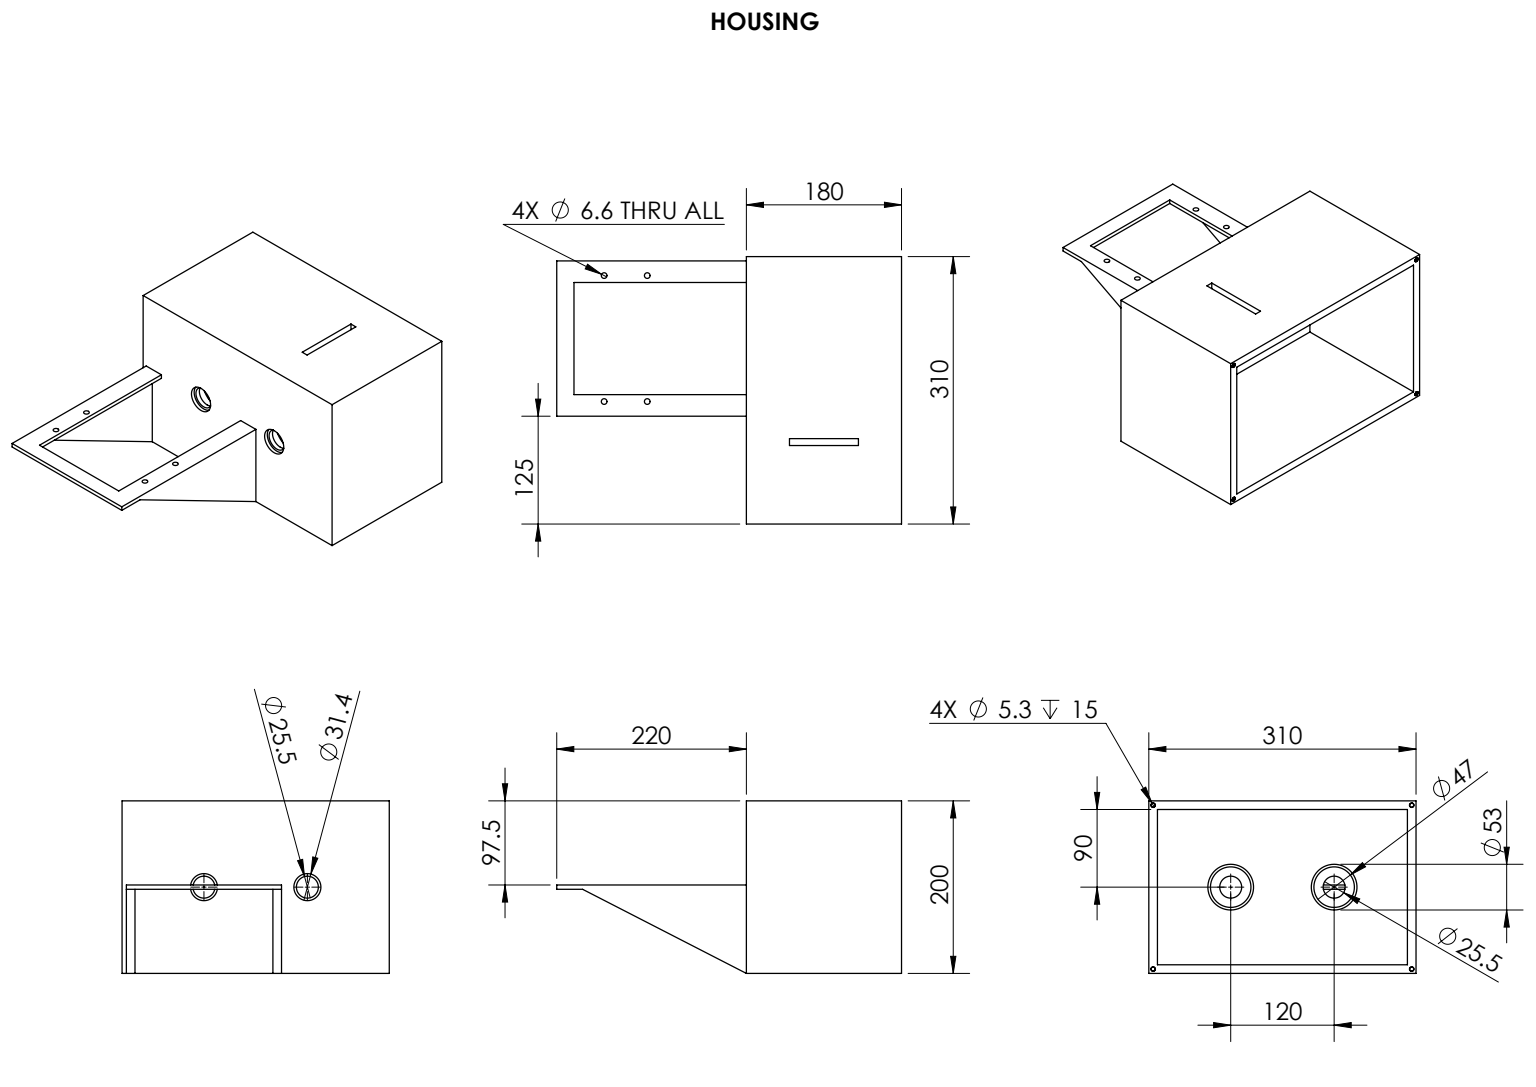
ISO-10303-21;
HEADER;
FILE_DESCRIPTION (('STEP AP214'),
    '1' );
FILE_NAME ('housing.step',
    '2026-10-08T09:53:37',
    ( '' ),
    ( '' ),
    'SwSTEP 2.0',
    'SolidWorks 2026',
    '' );
FILE_SCHEMA (( 'AUTOMOTIVE_DESIGN' ));
ENDSEC;

DATA;
#1=ORIENTED_EDGE ( 'NONE', *, *, #51679, .F. ) ;
#2=CARTESIAN_POINT ( 'NONE',  ( -96.15314808468745866, -211.9973110713294489, 75.77864583420047495 ) ) ;
#6=DIRECTION ( 'NONE',  ( -0.000000000000000000, -0.000000000000000000, 1.000000000000000000 ) ) ;
#9=CARTESIAN_POINT ( 'NONE',  ( -92.34999999999999432, -209.9999999999999716, 90.00000000000000000 ) ) ;
#10=CARTESIAN_POINT ( 'NONE',  ( 96.15314808468748708, 91.99731107132950569, 84.98614583420047097 ) ) ;
#18=CARTESIAN_POINT ( 'NONE',  ( 99.99999999999998579, 90.00000000000000000, -90.00000000000000000 ) ) ;
#23=CARTESIAN_POINT ( 'NONE',  ( -92.69370383062505425, 91.33154071421968467, 89.37822916753378877 ) ) ;
#27=CARTESIAN_POINT ( 'NONE',  ( -93.07557990970633455, 88.17815826261617929, 75.00000000000001421 ) ) ;
#29=CARTESIAN_POINT ( 'NONE',  ( -92.35000000000005116, 91.52997821335253548, 77.03541666666666288 ) ) ;
#32=DIRECTION ( 'NONE',  ( 0.4565542962317865050, 0.000000000000000000, 0.8896955516311735312 ) ) ;
#37=CARTESIAN_POINT ( 'NONE',  ( 97.30629616937498838, -208.6684592857803011, 84.45697916753383083 ) ) ;
#47=CARTESIAN_POINT ( 'NONE',  ( 96.15314808468750130, -211.9973110713294489, 77.78947916753381264 ) ) ;
#49=CARTESIAN_POINT ( 'NONE',  ( 95.00000000000000000, -212.6630814284392557, 84.24531250086715772 ) ) ;
#52=ORIENTED_EDGE ( 'NONE', *, *, #54649, .T. ) ;
#53=CARTESIAN_POINT ( 'NONE',  ( -92.35000000000005116, -211.5299782133524786, 88.35958333333334735 ) ) ;
#54=ORIENTED_EDGE ( 'NONE', *, *, #5365, .T. ) ;
#56=CARTESIAN_POINT ( 'NONE',  ( -97.30629616937501680, 88.66845928578038638, 75.24947916753383481 ) ) ;
#60=CARTESIAN_POINT ( 'NONE',  ( 97.64999999999997726, -211.5299782133524502, 87.16895833506762870 ) ) ;
#78=CARTESIAN_POINT ( 'NONE',  ( 95.00000000000000000, -213.0599564267049857, 76.18874999999999886 ) ) ;
#79=CARTESIAN_POINT ( 'NONE',  ( -97.64999999960622290, -209.9999706925929672, 76.74344264316562203 ) ) ;
#80=CARTESIAN_POINT ( 'NONE',  ( -97.65000000000001990, 90.00000000000004263, 86.82500000000000284 ) ) ;
#85=LINE ( 'NONE', #57553, #61145 ) ;
#86=CARTESIAN_POINT ( 'NONE',  ( -92.69370383062498320, -209.9999999999999716, 84.88031250086713442 ) ) ;
#87=ORIENTED_EDGE ( 'NONE', *, *, #45061, .F. ) ;
#90=CARTESIAN_POINT ( 'NONE',  ( 93.89144186338218390, -212.3693961632864955, 74.97612907457772735 ) ) ;
#91=CARTESIAN_POINT ( 'NONE',  ( -2.499999999999970690, 73.00000000000001421, -201.6999999999999602 ) ) ;
#92=CARTESIAN_POINT ( 'NONE',  ( -97.30629616937497417, -208.6684592857803295, 76.25489583420049655 ) ) ;
#95=CARTESIAN_POINT ( 'NONE',  ( 94.99999999999998579, 90.00000000000002842, 90.00000000000000000 ) ) ;
#101=CARTESIAN_POINT ( 'NONE',  ( -96.15314808468752972, 91.99731107132950569, 78.74197916753381321 ) ) ;
#104=( BOUNDED_CURVE ( )  B_SPLINE_CURVE ( 2, ( #36888, #19593, #59840, #8323, #31250, #71460, #19961 ),
 .UNSPECIFIED., .F., .F. ) 
 B_SPLINE_CURVE_WITH_KNOTS ( ( 3, 2, 2, 3 ),
 ( 0.2291666666666663521, 0.2361111111111107719, 0.2430555555555551639, 0.2499999999999995837 ),
 .UNSPECIFIED. ) 
 CURVE ( )  GEOMETRIC_REPRESENTATION_ITEM ( )  RATIONAL_B_SPLINE_CURVE ( ( 1.000000000000005995, 0.8660254037844328234, 1.000000000000000000, 0.8660254037844387076, 1.000000000000000000, 0.8660254037844467012, 0.9999999999999920064 ) ) 
 REPRESENTATION_ITEM ( '' )  );
#106=DIRECTION ( 'NONE',  ( -1.000000000000000000, 0.000000000000000000, -0.000000000000000000 ) ) ;
#108=CARTESIAN_POINT ( 'NONE',  ( 97.64999999999999147, 90.00000015433757028, 79.60187500750917877 ) ) ;
#112=CARTESIAN_POINT ( 'NONE',  ( -93.84685191531248449, -208.0026889286704943, 80.06489583420048461 ) ) ;
#113=LINE ( 'NONE', #11332, #2116 ) ;
#129=CARTESIAN_POINT ( 'NONE',  ( 92.69370383062501162, -208.6684592857803295, 89.58989583420047609 ) ) ;
#134=EDGE_CURVE ( 'NONE', #23470, #67171, #321, .T. ) ;
#135=ORIENTED_EDGE ( 'NONE', *, *, #35787, .T. ) ;
#145=ORIENTED_EDGE ( 'NONE', *, *, #39730, .F. ) ;
#146=CYLINDRICAL_SURFACE ( 'NONE', #33227, 26.50000000000000355 ) ;
#156=CARTESIAN_POINT ( 'NONE',  ( 97.30629616937498838, 91.33154071421968467, 85.56822916753380071 ) ) ;
#157=EDGE_CURVE ( 'NONE', #60576, #23470, #28588, .T. ) ;
#159=CARTESIAN_POINT ( 'NONE',  ( 96.15314808468750130, -211.9973110713294489, 82.23447916753380582 ) ) ;
#163=CARTESIAN_POINT ( 'NONE',  ( -2.500000000000015543, -73.00000000000001421, -255.0000000000000000 ) ) ;
#164=CARTESIAN_POINT ( 'NONE',  ( -94.99999999999997158, -206.9400435732949575, 89.20624999999999716 ) ) ;
#165=CARTESIAN_POINT ( 'NONE',  ( -97.65000000000001990, 90.00000000000004263, 79.20499999999999829 ) ) ;
#166=CARTESIAN_POINT ( 'NONE',  ( 97.65000000000000568, 88.47002178664752137, 85.26395833506762756 ) ) ;
#167=CARTESIAN_POINT ( 'NONE',  ( -93.84685191531248449, -208.0026889286704943, 84.98614583420047097 ) ) ;
#168=CARTESIAN_POINT ( 'NONE',  ( -92.69370383062502583, 91.33154071421968467, 85.72697916753381264 ) ) ;
#169=EDGE_CURVE ( 'NONE', #3345, #5520, #11254, .T. ) ;
#171=CARTESIAN_POINT ( 'NONE',  ( 96.15314808468748708, 91.99731107132950569, 84.98614583420047097 ) ) ;
#172=CARTESIAN_POINT ( 'NONE',  ( -95.00000000000002842, 92.66308142843932671, 85.03906250086714635 ) ) ;
#175=CARTESIAN_POINT ( 'NONE',  ( 96.32499999999998863, -212.2949673200287179, 76.32104166840096582 ) ) ;
#178=CARTESIAN_POINT ( 'NONE',  ( -96.15314808468745866, -211.9973110713294489, 86.57364583420047666 ) ) ;
#187=CARTESIAN_POINT ( 'NONE',  ( -97.65000000000001990, 90.00000000000004263, 77.29999999999999716 ) ) ;
#188=LINE ( 'NONE', #23080, #53533 ) ;
#190=LINE ( 'NONE', #46749, #7538 ) ;
#191=CARTESIAN_POINT ( 'NONE',  ( -92.35000000000000853, -208.4700217866474929, 89.73541666666663730 ) ) ;
#193=ORIENTED_EDGE ( 'NONE', *, *, #19096, .F. ) ;
#194=CARTESIAN_POINT ( 'NONE',  ( -97.30629616937501680, 88.66845928578038638, 76.99572916753380980 ) ) ;
#205=CARTESIAN_POINT ( 'NONE',  ( 97.30629616937498838, 90.00000000000002842, 78.68906250086715204 ) ) ;
#206=ADVANCED_FACE ( 'NONE', ( #58175 ), #28481, .T. ) ;
#207=CARTESIAN_POINT ( 'NONE',  ( -97.30629616937497417, -211.3315407142195852, 79.05947916753382287 ) ) ;
#211=CARTESIAN_POINT ( 'NONE',  ( -93.09170270117411405, -211.8387227684710012, 74.99909419456534465 ) ) ;
#214=EDGE_CURVE ( 'NONE', #50169, #71079, #46057, .T. ) ;
#216=CARTESIAN_POINT ( 'NONE',  ( -92.69370383062505425, 91.33154071421968467, 76.20197916753382117 ) ) ;
#217=CARTESIAN_POINT ( 'NONE',  ( 97.30629616937498838, -208.6684592857803011, 81.75822916753381264 ) ) ;
#219=CARTESIAN_POINT ( 'NONE',  ( -93.67500000000003979, 92.29496732002878900, 75.18333333333332291 ) ) ;
#221=ADVANCED_FACE ( 'NONE', ( #63104 ), #33867, .F. ) ;
#222=CYLINDRICAL_SURFACE ( 'NONE', #63992, 2.649999999999999467 ) ;
#228=ORIENTED_EDGE ( 'NONE', *, *, #5227, .F. ) ;
#230=EDGE_LOOP ( 'NONE', ( #33493, #51216, #41523, #73402, #35685 ) ) ;
#234=CARTESIAN_POINT ( 'NONE',  ( 94.99999999999998579, 92.66308142843935514, 83.92781250086716227 ) ) ;
#243=EDGE_CURVE ( 'NONE', #20441, #46588, #25658, .T. ) ;
#250=VECTOR ( 'NONE', #46862, 1000.000000000000000 ) ;
#251=FACE_OUTER_BOUND ( 'NONE', #1348, .T. ) ;
#255=CARTESIAN_POINT ( 'NONE',  ( -96.32499999999996021, -212.2949673200287179, 82.56520833506762358 ) ) ;
#256=ORIENTED_EDGE ( 'NONE', *, *, #21571, .T. ) ;
#260=CARTESIAN_POINT ( 'NONE',  ( 93.67499999999998295, 92.29496732002878900, 80.44854166840097776 ) ) ;
#261=CARTESIAN_POINT ( 'NONE',  ( -97.65000000000001990, 90.00000000000004263, 81.18937500173430521 ) ) ;
#263=CARTESIAN_POINT ( 'NONE',  ( 92.69370383062498320, 90.00000000000002842, 81.54656250086715374 ) ) ;
#269=CARTESIAN_POINT ( 'NONE',  ( -97.65000000000001990, 90.00000000000004263, 80.47499999999999432 ) ) ;
#273=ORIENTED_EDGE ( 'NONE', *, *, #31155, .T. ) ;
#276=FACE_OUTER_BOUND ( 'NONE', #73498, .T. ) ;
#277=CARTESIAN_POINT ( 'NONE',  ( -92.69370383062498320, -208.6684592857803011, 80.01197916753380923 ) ) ;
#284=CARTESIAN_POINT ( 'NONE',  ( 93.84685191531248449, 91.99731107132950569, 74.93197916753379673 ) ) ;
#288=DIRECTION ( 'NONE',  ( -0.000000000000000000, -0.000000000000000000, 1.000000000000000000 ) ) ;
#293=CARTESIAN_POINT ( 'NONE',  ( 97.30629616937498838, 88.66845928578035796, 88.79614583420048746 ) ) ;
#295=CARTESIAN_POINT ( 'NONE',  ( 94.99999999999998579, 86.94004357329502852, 82.53874999999999318 ) ) ;
#298=CARTESIAN_POINT ( 'NONE',  ( -95.00000000000002842, 92.66308142843932671, 81.22906250086714408 ) ) ;
#306=( BOUNDED_CURVE ( )  B_SPLINE_CURVE ( 2, ( #42487, #60161, #54139, #60884, #2672, #20658, #32290, #43244, #36830 ),
 .UNSPECIFIED., .F., .F. ) 
 B_SPLINE_CURVE_WITH_KNOTS ( ( 3, 2, 2, 2, 3 ),
 ( 0.3810111478265176821, 0.3810113392076479033, 0.3880671047485306224, 0.3951228702894133971, 0.4021785743327781493 ),
 .UNSPECIFIED. ) 
 CURVE ( )  GEOMETRIC_REPRESENTATION_ITEM ( )  RATIONAL_B_SPLINE_CURVE ( ( 0.9999927323225166198, 0.9999963660626911555, 1.000000000000000000, 0.8660254037844387076, 1.000000000000000000, 0.8660254037844387076, 1.000000000000000000, 0.8660265714968713446, 0.9999976645954902210 ) ) 
 REPRESENTATION_ITEM ( '' )  );
#307=CARTESIAN_POINT ( 'NONE',  ( 92.34999999999999432, 90.00000000000002842, 90.00000000000000000 ) ) ;
#314=ORIENTED_EDGE ( 'NONE', *, *, #27692, .F. ) ;
#316=CARTESIAN_POINT ( 'NONE',  ( 97.30629616937498838, -208.6684592857803295, 81.28197916753381946 ) ) ;
#321=( BOUNDED_CURVE ( )  B_SPLINE_CURVE ( 2, ( #16099, #50676, #20629, #43944, #66860, #72847, #67236, #38290, #61237 ),
 .UNSPECIFIED., .F., .F. ) 
 B_SPLINE_CURVE_WITH_KNOTS ( ( 3, 2, 2, 2, 3 ),
 ( 0.3386766260338263668, 0.3386767459623536980, 0.3457325115032360840, 0.3527882770441184701, 0.3598440426530882807 ),
 .UNSPECIFIED. ) 
 CURVE ( )  GEOMETRIC_REPRESENTATION_ITEM ( )  RATIONAL_B_SPLINE_CURVE ( ( 0.9999954456811732673, 0.9999977228018805953, 1.000000000000000000, 0.8660254037844387076, 1.000000000000000000, 0.8660254037844387076, 1.000000000000000000, 0.8660254037844387076, 1.000000000000000000 ) ) 
 REPRESENTATION_ITEM ( '' )  );
#322=CARTESIAN_POINT ( 'NONE',  ( 92.35000000049315361, 89.99996796133687837, 83.73041644179049570 ) ) ;
#324=CARTESIAN_POINT ( 'NONE',  ( 97.64999999999999147, -209.9999999999999716, 87.77749999999998920 ) ) ;
#329=ORIENTED_EDGE ( 'NONE', *, *, #65370, .T. ) ;
#331=EDGE_CURVE ( 'NONE', #62654, #68271, #27501, .T. ) ;
#333=CARTESIAN_POINT ( 'NONE',  ( -96.15314808468752972, 91.99731107132950569, 89.06072916753382174 ) ) ;
#336=CARTESIAN_POINT ( 'NONE',  ( 92.35000000000000853, -209.9999999999999716, 75.47437500173430180 ) ) ;
#337=CARTESIAN_POINT ( 'NONE',  ( 92.34999999999999432, 90.00000000000002842, 79.83999999999998920 ) ) ;
#338=EDGE_LOOP ( 'NONE', ( #19478, #31271, #53427, #16608 ) ) ;
#343=ORIENTED_EDGE ( 'NONE', *, *, #47596, .F. ) ;
#344=CARTESIAN_POINT ( 'NONE',  ( -97.65000000000001990, 91.52997821335253548, 89.39145833506763950 ) ) ;
#346=CARTESIAN_POINT ( 'NONE',  ( -97.30629616937501680, 91.33154071421968467, 82.76364583420048859 ) ) ;
#347=CARTESIAN_POINT ( 'NONE',  ( 94.99999999999998579, 92.66308142843935514, 89.64281250086715147 ) ) ;
#351=CARTESIAN_POINT ( 'NONE',  ( 96.32499999999998863, -212.2949673200287179, 85.76666666666665151 ) ) ;
#357=CARTESIAN_POINT ( 'NONE',  ( -92.69370383062498320, -209.9999999999999716, 77.89531250086714920 ) ) ;
#360=DIRECTION ( 'NONE',  ( -0.000000000000000000, -0.000000000000000000, 1.000000000000000000 ) ) ;
#362=CARTESIAN_POINT ( 'NONE',  ( 92.34999999999990905, 88.47002178664757821, 77.98791666666667766 ) ) ;
#363=CARTESIAN_POINT ( 'NONE',  ( -96.32499999999996021, -212.2949673200287179, 78.04083333333333883 ) ) ;
#365=CARTESIAN_POINT ( 'NONE',  ( -96.15314808468745866, -211.9973110713294489, 75.14364583420046984 ) ) ;
#373=CARTESIAN_POINT ( 'NONE',  ( 92.69370383062498320, 91.33154071421968467, 83.23989583420048177 ) ) ;
#397=DIRECTION ( 'NONE',  ( -0.000000000000000000, -0.000000000000000000, 1.000000000000000000 ) ) ;
#400=CARTESIAN_POINT ( 'NONE',  ( 95.00000000000000000, -207.3369185715606307, 85.83281250086714920 ) ) ;
#405=CARTESIAN_POINT ( 'NONE',  ( -97.64999999999996305, -209.9999999999999716, 86.18999999999999773 ) ) ;
#408=CARTESIAN_POINT ( 'NONE',  ( 95.00000000000000000, -212.6630814284392557, 76.46656250086712703 ) ) ;
#409=ORIENTED_EDGE ( 'NONE', *, *, #48240, .T. ) ;
#410=CARTESIAN_POINT ( 'NONE',  ( 93.84685191531249870, -208.0026889286704943, 83.98072916753382344 ) ) ;
#413=ORIENTED_EDGE ( 'NONE', *, *, #7216, .F. ) ;
#414=EDGE_LOOP ( 'NONE', ( #16035, #20964, #13795, #59926 ) ) ;
#418=DIRECTION ( 'NONE',  ( 1.000000000000000000, 0.000000000000000000, 0.000000000000000000 ) ) ;
#419=CARTESIAN_POINT ( 'NONE',  ( 97.64999999999997726, -211.5299782133524502, 86.53395833506763779 ) ) ;
#422=VECTOR ( 'NONE', #39738, 1000.000000000000000 ) ;
#423=VERTEX_POINT ( 'NONE', #26756 ) ;
#428=VERTEX_POINT ( 'NONE', #4227 ) ;
#429=CARTESIAN_POINT ( 'NONE',  ( -92.35001786638896704, -211.5299885285169523, 78.27895762153575276 ) ) ;
#437=CARTESIAN_POINT ( 'NONE',  ( 94.99999999999998579, 93.05995642670504253, 81.58624999999999261 ) ) ;
#438=CARTESIAN_POINT ( 'NONE',  ( -93.67500000000003979, 92.29496732002878900, 85.97833333333332462 ) ) ;
#443=DIRECTION ( 'NONE',  ( -1.000000000000000000, 0.000000000000000000, 0.000000000000000000 ) ) ;
#444=CARTESIAN_POINT ( 'NONE',  ( -96.15314808468745866, -211.9973110713294489, 86.57364583420047666 ) ) ;
#448=CARTESIAN_POINT ( 'NONE',  ( 94.70433044324006744, -212.6272429001183752, 74.99300273738302280 ) ) ;
#449=CARTESIAN_POINT ( 'NONE',  ( 97.64999999999999147, -209.9999999999999716, 87.77749999999998920 ) ) ;
#450=CARTESIAN_POINT ( 'NONE',  ( -94.99999999999997158, -212.6630814284392557, 77.10156250086711793 ) ) ;
#460=CARTESIAN_POINT ( 'NONE',  ( 94.99999999999998579, 86.94004357329502852, 88.25374999999999659 ) ) ;
#461=CARTESIAN_POINT ( 'NONE',  ( -96.15314808468751551, 88.00268892867056536, 78.31864583420048120 ) ) ;
#465=CARTESIAN_POINT ( 'NONE',  ( -97.64998201403183486, -208.4700114024439301, 80.50145761676010636 ) ) ;
#466=ADVANCED_FACE ( 'NONE', ( #10577, #5342 ), #11324, .T. ) ;
#472=CARTESIAN_POINT ( 'NONE',  ( -97.30629616937497417, -211.3315407142195852, 77.15447916753382174 ) ) ;
#475=ORIENTED_EDGE ( 'NONE', *, *, #13669, .T. ) ;
#491=CARTESIAN_POINT ( 'NONE',  ( 92.69370383062501162, -209.9999999999999716, 87.73781250086713612 ) ) ;
#492=CARTESIAN_POINT ( 'NONE',  ( -96.32499999999996021, -207.7050326799711968, 83.62354166840097491 ) ) ;
#496=CARTESIAN_POINT ( 'NONE',  ( 92.35000000000000853, -209.9999999999999716, 89.36499999999999488 ) ) ;
#502=CARTESIAN_POINT ( 'NONE',  ( -96.15314808468752972, 91.99731107132950569, 80.80572916753382628 ) ) ;
#508=ORIENTED_EDGE ( 'NONE', *, *, #49231, .F. ) ;
#510=B_SPLINE_CURVE_WITH_KNOTS ( 'NONE', 3,
 ( #3394, #26294, #49227, #66535, #39824, #742 ),
 .UNSPECIFIED., .F., .F.,
 ( 4, 2, 4 ),
 ( 0.7528176110416364697, 0.8153862273022683960, 0.8779548435629003222 ),
 .UNSPECIFIED. ) ;
#513=VECTOR ( 'NONE', #18864, 1000.000000000000000 ) ;
#515=CARTESIAN_POINT ( 'NONE',  ( 97.30629616937498838, 88.66845928578037217, 84.19239583420046813 ) ) ;
#517=CARTESIAN_POINT ( 'NONE',  ( 92.69370383062501162, -208.6684592857803011, 82.60489583420047666 ) ) ;
#519=CARTESIAN_POINT ( 'NONE',  ( -94.99999999999997158, -213.0599564267049857, 81.34812500173430294 ) ) ;
#520=CARTESIAN_POINT ( 'NONE',  ( -93.33265519076724104, -212.0887925413172184, 75.00000000000000000 ) ) ;
#525=CARTESIAN_POINT ( 'NONE',  ( -96.15314808468747287, -208.0026889286704943, 83.82197916753381151 ) ) ;
#526=CARTESIAN_POINT ( 'NONE',  ( -92.69370383062502583, 88.66845928578038638, 81.17614583420048291 ) ) ;
#528=CARTESIAN_POINT ( 'NONE',  ( 94.99999999999998579, 92.66308142843935514, 83.76906250086713612 ) ) ;
#529=( BOUNDED_CURVE ( )  B_SPLINE_CURVE ( 2, ( #47805, #72207, #66588, #9060, #20711, #13586, #71832, #43301, #43665 ),
 .UNSPECIFIED., .F., .F. ) 
 B_SPLINE_CURVE_WITH_KNOTS ( ( 3, 2, 2, 2, 3 ),
 ( 0.5291824299508934848, 0.5362381811070600079, 0.5432939466479423940, 0.5503497121888247801, 0.5503499107226622611 ),
 .UNSPECIFIED. ) 
 CURVE ( )  GEOMETRIC_REPRESENTATION_ITEM ( )  RATIONAL_B_SPLINE_CURVE ( ( 1.000000000000000000, 0.8660254037844387076, 1.000000000000000000, 0.8660254037844387076, 1.000000000000000000, 0.8660254037844387076, 1.000000000000000000, 0.9999962302473691667, 0.9999924607068835236 ) ) 
 REPRESENTATION_ITEM ( '' )  );
#532=CARTESIAN_POINT ( 'NONE',  ( 97.64999999999602665, -210.0000045800691737, 76.42687486206342840 ) ) ;
#534=LINE ( 'NONE', #6511, #45287 ) ;
#535=CARTESIAN_POINT ( 'NONE',  ( -97.30629616937495996, -209.9999999999999716, 86.46781250086714010 ) ) ;
#541=ORIENTED_EDGE ( 'NONE', *, *, #46124, .F. ) ;
#545=CARTESIAN_POINT ( 'NONE',  ( -97.65000000000001990, 91.52997821335253548, 77.24708333333332178 ) ) ;
#555=CARTESIAN_POINT ( 'NONE',  ( -92.69370383062504004, 90.00000000000004263, 79.80031250086713612 ) ) ;
#556=ADVANCED_FACE ( 'NONE', ( #33503 ), #45931, .F. ) ;
#558=AXIS2_PLACEMENT_3D ( 'NONE', #43819, #60369, #66736 ) ;
#561=CARTESIAN_POINT ( 'NONE',  ( 92.35000000039373447, 90.00002930740642171, 76.74344264317738862 ) ) ;
#563=CARTESIAN_POINT ( 'NONE',  ( -96.15314808468745866, -211.9973110713294489, 87.36739583420049371 ) ) ;
#566=CARTESIAN_POINT ( 'NONE',  ( 97.30629616937498838, 88.66845928578035796, 76.73114583420048973 ) ) ;
#568=CARTESIAN_POINT ( 'NONE',  ( -96.15314808468747287, -208.0026889286704943, 78.90072916753382515 ) ) ;
#570=ORIENTED_EDGE ( 'NONE', *, *, #37192, .T. ) ;
#572=DIRECTION ( 'NONE',  ( -0.000000000000000000, -0.000000000000000000, 1.000000000000000000 ) ) ;
#573=CYLINDRICAL_SURFACE ( 'NONE', #58202, 2.649999999999985700 ) ;
#575=CARTESIAN_POINT ( 'NONE',  ( 97.30629616937498838, -208.6684592857803011, 78.58322916753381548 ) ) ;
#577=EDGE_CURVE ( 'NONE', #43302, #35704, #70298, .T. ) ;
#578=EDGE_CURVE ( 'NONE', #23298, #25333, #62669, .T. ) ;
#587=ORIENTED_EDGE ( 'NONE', *, *, #27135, .F. ) ;
#589=CARTESIAN_POINT ( 'NONE',  ( 96.92442009029420547, -211.8218417373832096, 75.00000000000001421 ) ) ;
#593=CARTESIAN_POINT ( 'NONE',  ( 97.30629616937498838, 90.00000000000002842, 83.76906250086716454 ) ) ;
#596=CARTESIAN_POINT ( 'NONE',  ( 96.32499999999998863, -212.2949673200287179, 76.24166666666666003 ) ) ;
#597=ORIENTED_EDGE ( 'NONE', *, *, #35391, .T. ) ;
#603=CARTESIAN_POINT ( 'NONE',  ( -92.34999999999999432, -209.9999999999999716, 85.23749999999999716 ) ) ;
#605=CYLINDRICAL_SURFACE ( 'NONE', #65079, 2.649999999999985700 ) ;
#610=ORIENTED_EDGE ( 'NONE', *, *, #1325, .T. ) ;
#611=CARTESIAN_POINT ( 'NONE',  ( -93.67499999999998295, -212.2949673200287179, 79.49604166840096298 ) ) ;
#617=CARTESIAN_POINT ( 'NONE',  ( 94.99999999999998579, 86.94004357329500010, 80.71312500173431204 ) ) ;
#618=CARTESIAN_POINT ( 'NONE',  ( -95.00000000000002842, 93.05995642670501411, 81.03062500173430749 ) ) ;
#619=ORIENTED_EDGE ( 'NONE', *, *, #26416, .F. ) ;
#620=CARTESIAN_POINT ( 'NONE',  ( 97.30629616937498838, 91.33154071421968467, 79.37697916753381833 ) ) ;
#621=CARTESIAN_POINT ( 'NONE',  ( -93.67499999999998295, -207.7050326799711968, 82.16833333333332234 ) ) ;
#625=CYLINDRICAL_SURFACE ( 'NONE', #23007, 2.649999999999999467 ) ;
#626=CARTESIAN_POINT ( 'NONE',  ( 92.35000000000000853, -209.9999999999999716, 84.28499999999999659 ) ) ;
#628=CARTESIAN_POINT ( 'NONE',  ( -92.35000000000003695, 90.00000000000004263, 80.15749999999999886 ) ) ;
#636=FACE_OUTER_BOUND ( 'NONE', #73794, .T. ) ;
#638=CARTESIAN_POINT ( 'NONE',  ( -92.69370383062498320, -208.6684592857803011, 76.20197916753382117 ) ) ;
#644=FACE_BOUND ( 'NONE', #53061, .T. ) ;
#645=CARTESIAN_POINT ( 'NONE',  ( 94.99999999999998579, 87.33691857156068750, 75.83156250086715033 ) ) ;
#655=CARTESIAN_POINT ( 'NONE',  ( 97.30629616937498838, 88.66845928578035796, 85.62114583420047609 ) ) ;
#659=ORIENTED_EDGE ( 'NONE', *, *, #57378, .T. ) ;
#661=CARTESIAN_POINT ( 'NONE',  ( -92.69370383062505425, 88.66845928578038638, 81.01739583420048518 ) ) ;
#666=CARTESIAN_POINT ( 'NONE',  ( 97.30629616937498838, -209.9999999999999716, 86.78531250086714977 ) ) ;
#668=ORIENTED_EDGE ( 'NONE', *, *, #18506, .T. ) ;
#669=CARTESIAN_POINT ( 'NONE',  ( -92.35000000000003695, 89.99999996655868983, 87.85687500050293863 ) ) ;
#672=ORIENTED_EDGE ( 'NONE', *, *, #52995, .F. ) ;
#673=EDGE_CURVE ( 'NONE', #53082, #50612, #29711, .T. ) ;
#674=CARTESIAN_POINT ( 'NONE',  ( 7.103376864691351012E-17, -120.0000000000000000, -64.00000000000000000 ) ) ;
#678=ORIENTED_EDGE ( 'NONE', *, *, #36155, .F. ) ;
#679=CARTESIAN_POINT ( 'NONE',  ( 97.30629616937498838, -209.9999999999999716, 81.86406250086714920 ) ) ;
#680=CYLINDRICAL_SURFACE ( 'NONE', #59674, 2.649999999999985700 ) ;
#681=DIRECTION ( 'NONE',  ( -0.000000000000000000, -0.000000000000000000, 1.000000000000000000 ) ) ;
#683=CARTESIAN_POINT ( 'NONE',  ( 97.64999999989933599, 90.00002309722570715, 83.41187580057898288 ) ) ;
#685=CARTESIAN_POINT ( 'NONE',  ( 95.00000000000000000, -206.9400435732949575, 84.12625000000001307 ) ) ;
#693=CARTESIAN_POINT ( 'NONE',  ( -93.84685191531252713, 88.00268892867056536, 88.74322916753382628 ) ) ;
#696=CARTESIAN_POINT ( 'NONE',  ( 92.35000000000000853, -209.9999999999999716, 76.74437500173429783 ) ) ;
#697=CARTESIAN_POINT ( 'NONE',  ( 97.64999999999997726, 91.52997821335252127, 78.30541666666668732 ) ) ;
#698=ORIENTED_EDGE ( 'NONE', *, *, #67370, .F. ) ;
#699=CARTESIAN_POINT ( 'NONE',  ( -93.67499999999998295, -207.7050326799711968, 89.23270833506762756 ) ) ;
#700=ORIENTED_EDGE ( 'NONE', *, *, #70526, .F. ) ;
#702=ORIENTED_EDGE ( 'NONE', *, *, #35715, .T. ) ;
#703=CARTESIAN_POINT ( 'NONE',  ( -97.65000000000001990, 90.00000000000004263, 88.17437500173430465 ) ) ;
#704=CARTESIAN_POINT ( 'NONE',  ( -92.69370383062505425, 88.66845928578038638, 82.44614583420049314 ) ) ;
#705=CARTESIAN_POINT ( 'NONE',  ( 97.30629616937498838, 91.33154071421968467, 76.04322916753380923 ) ) ;
#710=CARTESIAN_POINT ( 'NONE',  ( 95.00000000000000000, -213.0599564267049857, 85.71374999999999034 ) ) ;
#715=AXIS2_PLACEMENT_3D ( 'NONE', #66827, #15314, #46127 ) ;
#716=CARTESIAN_POINT ( 'NONE',  ( -97.30629616937497417, -208.6684592857803011, 76.88989583420047325 ) ) ;
#721=CARTESIAN_POINT ( 'NONE',  ( 97.64999999946594755, 90.00005320149050192, 78.96687695417308817 ) ) ;
#724=ORIENTED_EDGE ( 'NONE', *, *, #39012, .T. ) ;
#728=CARTESIAN_POINT ( 'NONE',  ( -97.30629616937497417, -211.3315407142195852, 87.94947916753382344 ) ) ;
#730=CARTESIAN_POINT ( 'NONE',  ( 97.64999999994533653, 89.99998298270493535, 88.49187441316099978 ) ) ;
#732=ORIENTED_EDGE ( 'NONE', *, *, #49373, .F. ) ;
#735=CARTESIAN_POINT ( 'NONE',  ( -97.65000000000001990, 90.00000000000004263, 83.72937500173429726 ) ) ;
#738=CARTESIAN_POINT ( 'NONE',  ( 94.99999999999998579, 87.33691857156068750, 85.99156250086714692 ) ) ;
#742=CARTESIAN_POINT ( 'NONE',  ( 96.90829729882862864, -211.8387227684681591, 74.99954709728268654 ) ) ;
#745=CARTESIAN_POINT ( 'NONE',  ( 95.00000000000000000, -213.0599564267049857, 87.69812500173429726 ) ) ;
#747=( BOUNDED_CURVE ( )  B_SPLINE_CURVE ( 2, ( #24289, #12255, #25012, #14741, #18627, #40847, #41566, #47953, #70870 ),
 .UNSPECIFIED., .F., .F. ) 
 B_SPLINE_CURVE_WITH_KNOTS ( ( 3, 2, 2, 2, 3 ),
 ( 0.2751748541917909407, 0.2822306216366805010, 0.2892863871775971929, 0.2963421527185139959, 0.2963422021995995026 ),
 .UNSPECIFIED. ) 
 CURVE ( )  GEOMETRIC_REPRESENTATION_ITEM ( )  RATIONAL_B_SPLINE_CURVE ( ( 1.000000000000000000, 0.8660254037844387076, 1.000000000000000000, 0.8660254037844387076, 1.000000000000000000, 0.8660254037844387076, 1.000000000000000000, 0.9999990604551106665, 0.9999981209233991253 ) ) 
 REPRESENTATION_ITEM ( '' )  );
#756=( BOUNDED_CURVE ( )  B_SPLINE_CURVE ( 2, ( #59486, #48574, #47465, #64762, #25279, #41816, #36176, #7978, #48203 ),
 .UNSPECIFIED., .F., .F. ) 
 B_SPLINE_CURVE_WITH_KNOTS ( ( 3, 2, 2, 2, 3 ),
 ( 0.4021785743347534581, 0.4021786358322713695, 0.4092344013731880059, 0.4162901669141046423, 0.4233457466706606609 ),
 .UNSPECIFIED. ) 
 CURVE ( )  GEOMETRIC_REPRESENTATION_ITEM ( )  RATIONAL_B_SPLINE_CURVE ( ( 0.9999976645954944399, 0.9999988322875694724, 1.000000000000000000, 0.8660254037844387076, 1.000000000000000000, 0.8660254037844387076, 1.000000000000000000, 0.8660289314505091873, 0.9999929448536319931 ) ) 
 REPRESENTATION_ITEM ( '' )  );
#757=DIRECTION ( 'NONE',  ( 0.000000000000000000, 0.000000000000000000, 1.000000000000000000 ) ) ;
#761=CARTESIAN_POINT ( 'NONE',  ( -93.67500000000003979, 87.70503267997129626, 77.59104166840097605 ) ) ;
#764=CARTESIAN_POINT ( 'NONE',  ( 96.15314808468748708, -208.0026889286704943, 83.87489583420048689 ) ) ;
#769=VERTEX_POINT ( 'NONE', #31569 ) ;
#773=CARTESIAN_POINT ( 'NONE',  ( 96.15314808468748708, -208.0026889286704943, 75.46114583420047950 ) ) ;
#775=CARTESIAN_POINT ( 'NONE',  ( 92.69370383062501162, -208.6684592857803011, 80.85864583420048746 ) ) ;
#785=CARTESIAN_POINT ( 'NONE',  ( 96.32499999999998863, -207.7050326799711968, 87.96270833506763154 ) ) ;
#786=ORIENTED_EDGE ( 'NONE', *, *, #5639, .T. ) ;
#791=EDGE_CURVE ( 'NONE', #29550, #48269, #72525, .T. ) ;
#792=CARTESIAN_POINT ( 'NONE',  ( 97.64999999999997726, 91.52997821335252127, 87.27479166840096525 ) ) ;
#805=FACE_OUTER_BOUND ( 'NONE', #65981, .T. ) ;
#806=ADVANCED_FACE ( 'NONE', ( #54514 ), #43981, .F. ) ;
#807=CARTESIAN_POINT ( 'NONE',  ( -95.00000000000002842, 86.94004357329504273, 86.98374999999998636 ) ) ;
#812=CARTESIAN_POINT ( 'NONE',  ( -96.15314808468747287, -208.0026889286704943, 85.72697916753379843 ) ) ;
#815=CARTESIAN_POINT ( 'NONE',  ( -97.64999999992174651, -209.9999869687493685, 79.28395951166956479 ) ) ;
#819=CARTESIAN_POINT ( 'NONE',  ( -93.84685191531248449, -208.0026889286704943, 74.82614583420047438 ) ) ;
#826=DIRECTION ( 'NONE',  ( -0.000000000000000000, -0.000000000000000000, 1.000000000000000000 ) ) ;
#827=ADVANCED_FACE ( 'NONE', ( #55624 ), #60537, .F. ) ;
#829=EDGE_CURVE ( 'NONE', #43747, #51185, #3600, .T. ) ;
#830=CARTESIAN_POINT ( 'NONE',  ( -96.15314808468752972, 91.99731107132950569, 77.47197916753380298 ) ) ;
#844=CARTESIAN_POINT ( 'NONE',  ( -96.15314808468747287, -208.0026889286704943, 76.99572916753382401 ) ) ;
#845=FACE_OUTER_BOUND ( 'NONE', #61404, .T. ) ;
#856=CARTESIAN_POINT ( 'NONE',  ( 97.30629616937498838, -208.6684592857803295, 83.66322916753381378 ) ) ;
#865=CARTESIAN_POINT ( 'NONE',  ( -92.69370383062502583, 91.33154071421968467, 80.01197916753380923 ) ) ;
#869=EDGE_CURVE ( 'NONE', #18817, #10724, #10128, .T. ) ;
#871=( BOUNDED_CURVE ( )  B_SPLINE_CURVE ( 2, ( #24028, #46957, #18006, #63886, #69869, #12357, #35300 ),
 .UNSPECIFIED., .F., .F. ) 
 B_SPLINE_CURVE_WITH_KNOTS ( ( 3, 2, 2, 3 ),
 ( 0.8333333333333334814, 0.8402777777777779011, 0.8472222222222222099, 0.8541666666666666297 ),
 .UNSPECIFIED. ) 
 CURVE ( )  GEOMETRIC_REPRESENTATION_ITEM ( )  RATIONAL_B_SPLINE_CURVE ( ( 0.9999999999999978906, 0.8660254037844408170, 1.000000000000000000, 0.8660254037844387076, 1.000000000000000000, 0.8660254037844387076, 1.000000000000000000 ) ) 
 REPRESENTATION_ITEM ( '' )  );
#881=CARTESIAN_POINT ( 'NONE',  ( 96.32499999999998863, -212.2949673200287179, 80.76604166840097321 ) ) ;
#886=CARTESIAN_POINT ( 'NONE',  ( 96.15314808468750130, -211.9973110713294489, 81.59947916753381492 ) ) ;
#891=CARTESIAN_POINT ( 'NONE',  ( 97.64999999999999147, 89.99999999755287661, 75.15687493081163950 ) ) ;
#893=CARTESIAN_POINT ( 'NONE',  ( -97.65000000000003411, -208.4700217866475214, 89.31208333333333371 ) ) ;
#895=CARTESIAN_POINT ( 'NONE',  ( 96.32499999999998863, -207.7050326799711968, 76.45333333333333314 ) ) ;
#896=CARTESIAN_POINT ( 'NONE',  ( -97.30629616937497417, -211.3315407142195852, 85.88572916753382458 ) ) ;
#898=CARTESIAN_POINT ( 'NONE',  ( -96.15314808468751551, 88.00268892867056536, 82.28739583420048120 ) ) ;
#900=CARTESIAN_POINT ( 'NONE',  ( 97.30629616937498838, 88.66845928578037217, 85.46239583420047836 ) ) ;
#907=CARTESIAN_POINT ( 'NONE',  ( -94.99999999999997158, -212.6630814284392557, 85.35656250086714181 ) ) ;
#911=CARTESIAN_POINT ( 'NONE',  ( 92.35000000000005116, 91.52997821335254969, 80.42208333333330472 ) ) ;
#912=ORIENTED_EDGE ( 'NONE', *, *, #73582, .T. ) ;
#914=CARTESIAN_POINT ( 'NONE',  ( -93.67500000000003979, 87.70503267997129626, 78.78166666666666629 ) ) ;
#918=CARTESIAN_POINT ( 'NONE',  ( -97.30629616937501680, 91.33154071421968467, 87.68489583420047495 ) ) ;
#919=CARTESIAN_POINT ( 'NONE',  ( 97.64999999999999147, -209.9999999999999716, 80.79249999999998977 ) ) ;
#922=CARTESIAN_POINT ( 'NONE',  ( 97.65000000000000568, -208.4700217866474645, 77.74979166840097378 ) ) ;
#925=CARTESIAN_POINT ( 'NONE',  ( -97.30629616937501680, 91.33154071421968467, 76.88989583420047325 ) ) ;
#928=FACE_OUTER_BOUND ( 'NONE', #18946, .T. ) ;
#933=CARTESIAN_POINT ( 'NONE',  ( -94.99999999999997158, -212.6630814284392557, 84.88031250086714863 ) ) ;
#935=CARTESIAN_POINT ( 'NONE',  ( 97.64999999946594755, -209.9999467985095976, 78.96687695417307395 ) ) ;
#936=CARTESIAN_POINT ( 'NONE',  ( 92.69370383062498320, 90.00000000000002842, 76.46656250086715545 ) ) ;
#937=CARTESIAN_POINT ( 'NONE',  ( -97.30629616937497417, -211.3315407142195852, 75.24947916753383481 ) ) ;
#945=CARTESIAN_POINT ( 'NONE',  ( 97.30629616937498838, -211.3315407142195852, 77.20739583420046870 ) ) ;
#948=EDGE_CURVE ( 'NONE', #66194, #44844, #36716, .T. ) ;
#951=DIRECTION ( 'NONE',  ( 1.000000000000000000, 0.000000000000000000, 0.000000000000000000 ) ) ;
#953=CARTESIAN_POINT ( 'NONE',  ( -92.35000000053409508, 90.00005320149026034, 78.96687695417308817 ) ) ;
#954=EDGE_LOOP ( 'NONE', ( #39042, #25241, #27298, #50210 ) ) ;
#962=( BOUNDED_CURVE ( )  B_SPLINE_CURVE ( 2, ( #1157, #42080, #42445, #59365, #65383, #65016, #54102 ),
 .UNSPECIFIED., .F., .F. ) 
 B_SPLINE_CURVE_WITH_KNOTS ( ( 3, 2, 2, 3 ),
 ( 0.4583333333333335924, 0.4652777777777780122, 0.4722222222222224319, 0.4791666666666668517 ),
 .UNSPECIFIED. ) 
 CURVE ( )  GEOMETRIC_REPRESENTATION_ITEM ( )  RATIONAL_B_SPLINE_CURVE ( ( 0.9999999999999946709, 0.8660254037844440367, 1.000000000000000000, 0.8660254037844387076, 1.000000000000000000, 0.8660254037844354880, 1.000000000000003109 ) ) 
 REPRESENTATION_ITEM ( '' )  );
#963=CARTESIAN_POINT ( 'NONE',  ( 94.99999999999998579, 92.66308142843935514, 83.29281250086717137 ) ) ;
#977=CARTESIAN_POINT ( 'NONE',  ( -92.34999999999999432, -208.4700217866474645, 75.20979166840096752 ) ) ;
#981=CARTESIAN_POINT ( 'NONE',  ( 92.35000000039364920, -209.9999706968037287, 82.45844277051352833 ) ) ;
#985=CARTESIAN_POINT ( 'NONE',  ( -93.67499999999998295, -207.7050326799711968, 77.80270833506763495 ) ) ;
#989=CARTESIAN_POINT ( 'NONE',  ( 92.34999999999999432, 91.52997821335252127, 79.86645833506761960 ) ) ;
#990=CARTESIAN_POINT ( 'NONE',  ( -97.65000000000001990, 88.47002178664754979, 78.70229166840096013 ) ) ;
#992=CARTESIAN_POINT ( 'NONE',  ( 92.69370383062498320, 90.00000000000002842, 78.37156250086715659 ) ) ;
#995=CARTESIAN_POINT ( 'NONE',  ( -92.35000000000003695, 89.99999997928479445, 80.87187500099602744 ) ) ;
#999=CARTESIAN_POINT ( 'NONE',  ( 92.35000000000003695, -208.4700217866474929, 77.24708333333332178 ) ) ;
#1001=ORIENTED_EDGE ( 'NONE', *, *, #65099, .T. ) ;
#1008=DIRECTION ( 'NONE',  ( -0.000000000000000000, -0.000000000000000000, 1.000000000000000000 ) ) ;
#1010=CARTESIAN_POINT ( 'NONE',  ( -93.84685191531247028, -211.9973110713294489, 77.94822916753382458 ) ) ;
#1013=ORIENTED_EDGE ( 'NONE', *, *, #51838, .T. ) ;
#1021=CARTESIAN_POINT ( 'NONE',  ( 92.34999999999999432, 90.00000000000002842, 86.26937500173430351 ) ) ;
#1024=AXIS2_PLACEMENT_3D ( 'NONE', #8514, #65658, #64924 ) ;
#1025=CARTESIAN_POINT ( 'NONE',  ( 92.69370383062498320, 88.66845928578035796, 87.94947916753382344 ) ) ;
#1028=CARTESIAN_POINT ( 'NONE',  ( -96.15314808468745866, -211.9973110713294489, 86.09739583420049769 ) ) ;
#1030=ORIENTED_EDGE ( 'NONE', *, *, #64700, .F. ) ;
#1031=CARTESIAN_POINT ( 'NONE',  ( -97.65000000000006253, 91.52997821335252127, 81.69208333333332916 ) ) ;
#1032=CARTESIAN_POINT ( 'NONE',  ( -92.34999999999999432, -208.4700217866474645, 80.21041666666666003 ) ) ;
#1033=CARTESIAN_POINT ( 'NONE',  ( -93.26027265873601380, 91.51405112163766375, 74.79348190356853365 ) ) ;
#1034=AXIS2_PLACEMENT_3D ( 'NONE', #51639, #52754, #57661 ) ;
#1036=CARTESIAN_POINT ( 'NONE',  ( 92.69370383062501162, -209.9999999999999716, 86.46781250086714010 ) ) ;
#1041=DIRECTION ( 'NONE',  ( -0.000000000000000000, -0.000000000000000000, -1.000000000000000000 ) ) ;
#1051=CARTESIAN_POINT ( 'NONE',  ( 97.30629616937498838, -208.6684592857803295, 80.64697916753382856 ) ) ;
#1053=CYLINDRICAL_SURFACE ( 'NONE', #39955, 2.649999999999985700 ) ;
#1054=COLOUR_RGB ( '', 0.66274510, 0.83137255, 0.94901961) ;
#1058=CARTESIAN_POINT ( 'NONE',  ( 95.00000000000000000, -206.9400435732949575, 86.03125000000000000 ) ) ;
#1066=CARTESIAN_POINT ( 'NONE',  ( -95.00000000000002842, 92.66308142843932671, 87.73781250086715033 ) ) ;
#1069=CARTESIAN_POINT ( 'NONE',  ( 93.67500000000001137, -207.7050326799711968, 74.73354166840096013 ) ) ;
#1070=CARTESIAN_POINT ( 'NONE',  ( 96.32499999999998863, 87.70503267997126784, 77.51166666666665606 ) ) ;
#1072=CARTESIAN_POINT ( 'NONE',  ( -97.64999999999994884, -211.5299782133524502, 88.22729166840096582 ) ) ;
#1074=CARTESIAN_POINT ( 'NONE',  ( -97.64999999999999147, -211.5299782133525071, 84.97291666666667709 ) ) ;
#1077=CARTESIAN_POINT ( 'NONE',  ( -95.00000000000002842, 86.94004357329504273, 88.33312500173428816 ) ) ;
#1078=CARTESIAN_POINT ( 'NONE',  ( -93.84685191531254134, 91.99731107132950569, 82.60489583420049087 ) ) ;
#1080=CARTESIAN_POINT ( 'NONE',  ( 97.30629616937498838, 90.00000000000002842, 74.72031250086713783 ) ) ;
#1086=DIRECTION ( 'NONE',  ( 0.000000000000000000, -0.000000000000000000, -1.000000000000000000 ) ) ;
#1088=CARTESIAN_POINT ( 'NONE',  ( -97.64999999999996305, -209.9999999999999716, 86.26937500173430351 ) ) ;
#1091=EDGE_CURVE ( 'NONE', #44704, #27953, #35640, .T. ) ;
#1099=CARTESIAN_POINT ( 'NONE',  ( -92.34999999999999432, -209.9999999999999716, 89.04749999999999943 ) ) ;
#1102=CARTESIAN_POINT ( 'NONE',  ( -93.84685191531248449, -208.0026889286704943, 87.04989583420048405 ) ) ;
#1106=ORIENTED_EDGE ( 'NONE', *, *, #17167, .T. ) ;
#1107=AXIS2_PLACEMENT_3D ( 'NONE', #20105, #19733, #37790 ) ;
#1112=CARTESIAN_POINT ( 'NONE',  ( 92.69370383062498320, 88.66845928578035796, 81.44072916753380298 ) ) ;
#1115=CARTESIAN_POINT ( 'NONE',  ( -96.32500000000001705, 92.29496732002878900, 85.44916666666665606 ) ) ;
#1120=CARTESIAN_POINT ( 'NONE',  ( 94.99999999999998579, 90.00000000000002842, 90.00000000000000000 ) ) ;
#1122=CARTESIAN_POINT ( 'NONE',  ( -92.69370383062505425, 91.33154071421968467, 88.10822916753380696 ) ) ;
#1123=LINE ( 'NONE', #17998, #61089 ) ;
#1126=VERTEX_POINT ( 'NONE', #23638 ) ;
#1130=CARTESIAN_POINT ( 'NONE',  ( 92.35000000046503033, 89.99996900126896548, 83.09538598081184091 ) ) ;
#1131=AXIS2_PLACEMENT_3D ( 'NONE', #52664, #1217, #24110 ) ;
#1135=CARTESIAN_POINT ( 'NONE',  ( 96.15314808468750130, -211.9973110713294489, 81.12322916753382174 ) ) ;
#1137=EDGE_CURVE ( 'NONE', #25853, #74080, #3155, .T. ) ;
#1143=CARTESIAN_POINT ( 'NONE',  ( 95.00000000000000000, -206.9400435732949575, 88.57124999999999204 ) ) ;
#1147=CARTESIAN_POINT ( 'NONE',  ( 95.00000000000000000, -207.3369185715606307, 80.75281250086715090 ) ) ;
#1151=CARTESIAN_POINT ( 'NONE',  ( 97.64999999999999147, 89.99999990163419739, 80.23687499810812085 ) ) ;
#1157=CARTESIAN_POINT ( 'NONE',  ( -97.65000000000001990, 90.00000000000004263, 83.01499999999998636 ) ) ;
#1161=CARTESIAN_POINT ( 'NONE',  ( 92.35000000000000853, -209.9999999999999716, 86.26937500173430351 ) ) ;
#1162=CARTESIAN_POINT ( 'NONE',  ( 94.99999999999998579, 86.94004357329500010, 87.61875000000000568 ) ) ;
#1165=CARTESIAN_POINT ( 'NONE',  ( 92.35001072950491618, 91.52998440803509084, 84.94645790656223028 ) ) ;
#1169=CARTESIAN_POINT ( 'NONE',  ( -97.30629616937501680, 90.00000000000004263, 89.80156250086714920 ) ) ;
#1171=CARTESIAN_POINT ( 'NONE',  ( 97.64999999999997726, 88.47002178664753558, 86.53395833506763779 ) ) ;
#1178=ORIENTED_EDGE ( 'NONE', *, *, #31971, .T. ) ;
#1180=EDGE_LOOP ( 'NONE', ( #3896, #18215, #17497, #47321 ) ) ;
#1183=CARTESIAN_POINT ( 'NONE',  ( -92.35000000000005116, 88.47002178664754979, 88.35958333333333314 ) ) ;
#1185=ADVANCED_FACE ( 'NONE', ( #52568 ), #1489, .F. ) ;
#1187=( BOUNDED_CURVE ( )  B_SPLINE_CURVE ( 2, ( #53628, #31794, #37083, #54740, #54373, #2170, #25056 ),
 .UNSPECIFIED., .F., .F. ) 
 B_SPLINE_CURVE_WITH_KNOTS ( ( 3, 2, 2, 3 ),
 ( 0.1905056698846566698, 0.1975614351456765616, 0.2046172006865936144, 0.2116728463017078510 ),
 .UNSPECIFIED. ) 
 CURVE ( )  GEOMETRIC_REPRESENTATION_ITEM ( )  RATIONAL_B_SPLINE_CURVE ( ( 1.000000000000000000, 0.8660254037844387076, 1.000000000000000000, 0.8660254037844387076, 1.000000000000000000, 0.8660276809308252721, 0.9999954457846356171 ) ) 
 REPRESENTATION_ITEM ( '' )  );
#1191=CARTESIAN_POINT ( 'NONE',  ( -97.30629616937497417, -208.6684592857803011, 82.60489583420047666 ) ) ;
#1195=CARTESIAN_POINT ( 'NONE',  ( 93.74200686866063847, -212.2877248121147034, 74.97309184317512631 ) ) ;
#1197=CARTESIAN_POINT ( 'NONE',  ( -92.69370383062498320, -211.3315407142195852, 77.84239583420047381 ) ) ;
#1200=VECTOR ( 'NONE', #13246, 1000.000000000000000 ) ;
#1207=CARTESIAN_POINT ( 'NONE',  ( -95.00000000000002842, 87.33691857156074434, 77.10156250086711793 ) ) ;
#1213=CARTESIAN_POINT ( 'NONE',  ( 97.65000000000000568, -208.4700217866474645, 89.17979166840096639 ) ) ;
#1217=DIRECTION ( 'NONE',  ( -0.000000000000000000, -0.000000000000000000, 1.000000000000000000 ) ) ;
#1220=CARTESIAN_POINT ( 'NONE',  ( -97.30629616937495996, -209.9999999999999716, 77.10156250086714635 ) ) ;
#1223=DIRECTION ( 'NONE',  ( 1.000000000000000000, 0.000000000000000000, -0.000000000000000000 ) ) ;
#1226=LINE ( 'NONE', #70684, #62292 ) ;
#1227=CARTESIAN_POINT ( 'NONE',  ( -97.65000000000001990, 90.00000000000004263, 90.00000000000000000 ) ) ;
#1237=CARTESIAN_POINT ( 'NONE',  ( 93.84685191531249870, -208.0026889286704943, 86.36197916753381776 ) ) ;
#1238=CARTESIAN_POINT ( 'NONE',  ( -92.35000000010064980, -209.9999769027738239, 83.41187580057901130 ) ) ;
#1239=ORIENTED_EDGE ( 'NONE', *, *, #62083, .F. ) ;
#1240=CARTESIAN_POINT ( 'NONE',  ( -92.35000000000005116, 91.52997821335253548, 79.57541666666666913 ) ) ;
#1242=ORIENTED_EDGE ( 'NONE', *, *, #57164, .F. ) ;
#1245=CARTESIAN_POINT ( 'NONE',  ( -97.30629616937501680, 88.66845928578038638, 80.96447916753382401 ) ) ;
#1252=DIRECTION ( 'NONE',  ( -0.000000000000000000, -0.000000000000000000, 1.000000000000000000 ) ) ;
#1262=VERTEX_POINT ( 'NONE', #37880 ) ;
#1263=CARTESIAN_POINT ( 'NONE',  ( 93.84685191531251292, -211.9973110713294489, 82.76364583420047438 ) ) ;
#1265=ADVANCED_FACE ( 'NONE', ( #71698 ), #68476, .F. ) ;
#1271=CARTESIAN_POINT ( 'NONE',  ( 92.35000000000000853, -209.9999999999999716, 79.20499999999999829 ) ) ;
#1272=CARTESIAN_POINT ( 'NONE',  ( -97.64999999999996305, -209.9999999999999716, 89.36499999999999488 ) ) ;
#1274=VECTOR ( 'NONE', #31612, 1000.000000000000000 ) ;
#1277=CARTESIAN_POINT ( 'NONE',  ( -97.30629616937495996, -209.9999999999999716, 85.83281250086714920 ) ) ;
#1278=CARTESIAN_POINT ( 'NONE',  ( -92.69370383062504004, 90.00000000000004263, 81.22906250086715829 ) ) ;
#1280=CARTESIAN_POINT ( 'NONE',  ( 93.84685191531248449, 91.99731107132950569, 82.55197916753380127 ) ) ;
#1282=CARTESIAN_POINT ( 'NONE',  ( -95.00000000000002842, 86.94004357329504273, 78.80812500173429669 ) ) ;
#1287=CARTESIAN_POINT ( 'NONE',  ( -92.69370383062498320, -211.3315407142195852, 88.00239583420047040 ) ) ;
#1293=ORIENTED_EDGE ( 'NONE', *, *, #14537, .T. ) ;
#1295=CARTESIAN_POINT ( 'NONE',  ( -97.65000000000001990, 88.47002178664754979, 78.62291666666668277 ) ) ;
#1297=CARTESIAN_POINT ( 'NONE',  ( -97.30629616937501680, 90.00000000000004263, 89.00781250086714635 ) ) ;
#1299=CARTESIAN_POINT ( 'NONE',  ( 92.34999999999999432, 90.00000000000002842, 76.66499999999999204 ) ) ;
#1302=ORIENTED_EDGE ( 'NONE', *, *, #61731, .T. ) ;
#1307=CARTESIAN_POINT ( 'NONE',  ( -97.64999999999996305, -209.9999999999999716, 90.00000000000000000 ) ) ;
#1310=CARTESIAN_POINT ( 'NONE',  ( -94.99999999999997158, -212.6630814284392557, 87.42031250086715488 ) ) ;
#1312=EDGE_CURVE ( 'NONE', #51311, #11086, #32593, .T. ) ;
#1317=CARTESIAN_POINT ( 'NONE',  ( -96.15314808468745866, -211.9973110713294489, 75.30239583420048177 ) ) ;
#1325=EDGE_CURVE ( 'NONE', #15992, #50254, #26586, .T. ) ;
#1326=AXIS2_PLACEMENT_3D ( 'NONE', #48969, #48614, #71528 ) ;
#1327=CARTESIAN_POINT ( 'NONE',  ( -92.69370383062504004, 90.00000000000004263, 75.51406250086715488 ) ) ;
#1328=CARTESIAN_POINT ( 'NONE',  ( 95.00000000000000000, -212.6630814284392557, 76.46656250086712703 ) ) ;
#1333=EDGE_CURVE ( 'NONE', #6700, #65764, #21417, .T. ) ;
#1345=CARTESIAN_POINT ( 'NONE',  ( 92.69370383062498320, 91.33154071421968467, 84.66864583420047552 ) ) ;
#1347=CARTESIAN_POINT ( 'NONE',  ( 97.64999999999997726, -211.5299782133524502, 76.29458333333333542 ) ) ;
#1348=EDGE_LOOP ( 'NONE', ( #12482, #25821, #42433, #73861 ) ) ;
#1356=CARTESIAN_POINT ( 'NONE',  ( -97.64999999999996305, -210.0000123297513142, 75.47437542817786493 ) ) ;
#1360=CYLINDRICAL_SURFACE ( 'NONE', #49182, 2.649999999999985700 ) ;
#1362=CARTESIAN_POINT ( 'NONE',  ( -92.34999999999999432, -208.4700217866474645, 80.28979166840098003 ) ) ;
#1366=CARTESIAN_POINT ( 'NONE',  ( 96.32499999999998863, 87.70503267997126784, 80.13104166840095388 ) ) ;
#1367=CARTESIAN_POINT ( 'NONE',  ( -97.65000000000001990, 88.47002178664754979, 75.52729166840099140 ) ) ;
#1368=ORIENTED_EDGE ( 'NONE', *, *, #26702, .T. ) ;
#1369=CARTESIAN_POINT ( 'NONE',  ( 92.69370383062498320, 90.00000000000002842, 80.27656250086714351 ) ) ;
#1383=CYLINDRICAL_SURFACE ( 'NONE', #67856, 2.649999999999999467 ) ;
#1385=CARTESIAN_POINT ( 'NONE',  ( -97.30629616937495996, -209.9999999999999716, 78.37156250086715659 ) ) ;
#1389=CARTESIAN_POINT ( 'NONE',  ( -94.99999999999997158, -209.9999999999999716, 90.00000000000000000 ) ) ;
#1390=CARTESIAN_POINT ( 'NONE',  ( -92.34999999999999432, -209.9999999999999716, 90.00000000000000000 ) ) ;
#1399=DIRECTION ( 'NONE',  ( -0.000000000000000000, -0.000000000000000000, 1.000000000000000000 ) ) ;
#1400=CARTESIAN_POINT ( 'NONE',  ( 93.84685191531248449, 88.00268892867053694, 86.09739583420049769 ) ) ;
#1402=CARTESIAN_POINT ( 'NONE',  ( -92.69370383062498320, -211.3315407142195852, 86.25614583420048120 ) ) ;
#1404=VECTOR ( 'NONE', #49786, 1000.000000000000000 ) ;
#1405=CARTESIAN_POINT ( 'NONE',  ( 96.32499999999998863, -212.2949673200287179, 83.30604166840096525 ) ) ;
#1407=CARTESIAN_POINT ( 'NONE',  ( -92.34999999999999432, -208.4700217866474645, 82.75041666666665208 ) ) ;
#1408=CARTESIAN_POINT ( 'NONE',  ( -92.69370383062505425, 88.66845928578038638, 77.20739583420046870 ) ) ;
#1411=CARTESIAN_POINT ( 'NONE',  ( 95.00000000000000000, -207.3369185715606307, 85.67406250086715147 ) ) ;
#1415=( BOUNDED_CURVE ( )  B_SPLINE_CURVE ( 2, ( #55247, #62014, #10879, #21026, #50342, #61269, #73272 ),
 .UNSPECIFIED., .F., .F. ) 
 B_SPLINE_CURVE_WITH_KNOTS ( ( 3, 2, 2, 3 ),
 ( 0.8125000000000002220, 0.8194444444444446418, 0.8263888888888889506, 0.8333333333333334814 ),
 .UNSPECIFIED. ) 
 CURVE ( )  GEOMETRIC_REPRESENTATION_ITEM ( )  RATIONAL_B_SPLINE_CURVE ( ( 0.9999999999999956701, 0.8660254037844430375, 1.000000000000000000, 0.8660254037844387076, 1.000000000000000000, 0.8660254037844365982, 1.000000000000002220 ) ) 
 REPRESENTATION_ITEM ( '' )  );
#1421=CARTESIAN_POINT ( 'NONE',  ( 97.64999999999999147, 90.00000000000002842, 90.00000000000000000 ) ) ;
#1424=ORIENTED_EDGE ( 'NONE', *, *, #33606, .T. ) ;
#1425=CARTESIAN_POINT ( 'NONE',  ( 95.00000000000000000, -207.3369185715606307, 83.29281250086715715 ) ) ;
#1435=CARTESIAN_POINT ( 'NONE',  ( 93.67500000000001137, -212.2949673200287179, 85.02583333333332405 ) ) ;
#1441=CARTESIAN_POINT ( 'NONE',  ( -97.30629616937501680, 90.00000000000004263, 88.53156250086716739 ) ) ;
#1442=CARTESIAN_POINT ( 'NONE',  ( -0.0004442498525516064278, 0.001194404164626844313, -80.00000000000000000 ) ) ;
#1443=CARTESIAN_POINT ( 'NONE',  ( 97.65000000000000568, -210.0000154727341055, 78.33187446658581621 ) ) ;
#1444=CARTESIAN_POINT ( 'NONE',  ( 93.84685191531249870, -208.0026889286704943, 88.90197916753380980 ) ) ;
#1445=CARTESIAN_POINT ( 'NONE',  ( 97.64999999999997726, 88.47002178664753558, 79.46958333333333258 ) ) ;
#1447=CARTESIAN_POINT ( 'NONE',  ( -97.64999999999996305, -209.9999999999999716, 89.44437500173430067 ) ) ;
#1451=CARTESIAN_POINT ( 'NONE',  ( -92.35000000000005116, 91.52997821335253548, 87.27479166840096525 ) ) ;
#1452=CARTESIAN_POINT ( 'NONE',  ( 94.99999999999998579, 87.33691857156068750, 75.19656250086714522 ) ) ;
#1456=DIRECTION ( 'NONE',  ( 0.000000000000000000, 0.000000000000000000, 1.000000000000000000 ) ) ;
#1461=CARTESIAN_POINT ( 'NONE',  ( -94.99999999999997158, -207.3369185715606307, 75.51406250086714067 ) ) ;
#1469=CARTESIAN_POINT ( 'NONE',  ( -97.30629616937497417, -208.6684592857803011, 86.57364583420047666 ) ) ;
#1470=ORIENTED_EDGE ( 'NONE', *, *, #28367, .T. ) ;
#1478=CARTESIAN_POINT ( 'NONE',  ( 94.99999999999998579, 92.66308142843932671, 81.86406250086713499 ) ) ;
#1483=CYLINDRICAL_SURFACE ( 'NONE', #12026, 2.649999999999999467 ) ;
#1486=EDGE_CURVE ( 'NONE', #13338, #50169, #7947, .T. ) ;
#1489=CYLINDRICAL_SURFACE ( 'NONE', #8409, 2.649999999999999467 ) ;
#1490=EDGE_CURVE ( 'NONE', #73251, #73292, #52095, .T. ) ;
#1492=CARTESIAN_POINT ( 'NONE',  ( -93.84685191531252713, 88.00268892867056536, 87.94947916753380923 ) ) ;
#1497=CARTESIAN_POINT ( 'NONE',  ( 97.64999999999987779, -208.4700217866473793, 83.38541666666667140 ) ) ;
#1501=STYLED_ITEM ( 'NONE', ( #59364 ), #59777 ) ;
#1504=CARTESIAN_POINT ( 'NONE',  ( 97.30629616937498838, -208.6684592857803011, 83.18697916753382060 ) ) ;
#1517=CARTESIAN_POINT ( 'NONE',  ( 96.15314808468750130, -211.9973110713294489, 80.48822916753381662 ) ) ;
#1525=FILL_AREA_STYLE ('',( #52986 ) ) ;
#1529=CARTESIAN_POINT ( 'NONE',  ( 97.64999999999997726, -211.5299782133524502, 83.35895833506762642 ) ) ;
#1530=CARTESIAN_POINT ( 'NONE',  ( 92.34999999999999432, 90.00000000000002842, 90.00000000000000000 ) ) ;
#1533=CARTESIAN_POINT ( 'NONE',  ( -92.35000000000003695, 90.00000000000004263, 78.88750000000000284 ) ) ;
#1538=CARTESIAN_POINT ( 'NONE',  ( 92.34999999999999432, 88.47002178664753558, 87.59229166840096070 ) ) ;
#1548=CARTESIAN_POINT ( 'NONE',  ( -97.65000000000001990, 90.00000000000004263, 86.18999999999999773 ) ) ;
#1554=CARTESIAN_POINT ( 'NONE',  ( -92.69370383062498320, -208.6684592857803011, 82.39322916753381776 ) ) ;
#1558=CARTESIAN_POINT ( 'NONE',  ( 93.67499999999998295, 92.29496732002878900, 89.33854166840096411 ) ) ;
#1566=CARTESIAN_POINT ( 'NONE',  ( 96.85456758451090309, -211.3788240028427765, 74.79348190356850523 ) ) ;
#1571=CARTESIAN_POINT ( 'NONE',  ( -96.15314808468752972, 91.99731107132950569, 79.37697916753380412 ) ) ;
#1575=DIRECTION ( 'NONE',  ( 0.000000000000000000, -0.000000000000000000, -1.000000000000000000 ) ) ;
#1582=CARTESIAN_POINT ( 'NONE',  ( 95.00000000000000000, -209.9999999999999716, 90.00000000000000000 ) ) ;
#1583=CARTESIAN_POINT ( 'NONE',  ( -92.69370383062498320, -210.9303121318040155, 74.84209103131394158 ) ) ;
#1586=ORIENTED_EDGE ( 'NONE', *, *, #57493, .F. ) ;
#1594=CARTESIAN_POINT ( 'NONE',  ( 97.64999999999999147, 90.00001154861291752, 83.41187540116095533 ) ) ;
#1595=EDGE_LOOP ( 'NONE', ( #4910, #24656 ) ) ;
#1596=DIRECTION ( 'NONE',  ( -0.000000000000000000, -0.000000000000000000, 1.000000000000000000 ) ) ;
#1600=CARTESIAN_POINT ( 'NONE',  ( 93.84685191531251292, -211.9973110713294489, 85.93864583420048575 ) ) ;
#1601=CARTESIAN_POINT ( 'NONE',  ( 92.69370383062501162, -209.9999999999999716, 87.89656250086714806 ) ) ;
#1609=CARTESIAN_POINT ( 'NONE',  ( -93.84685191531254134, 91.99731107132950569, 81.33489583420049485 ) ) ;
#1613=CYLINDRICAL_SURFACE ( 'NONE', #24485, 3.299999999999969624 ) ;
#1617=ORIENTED_EDGE ( 'NONE', *, *, #51959, .T. ) ;
#1619=AXIS2_PLACEMENT_3D ( 'NONE', #13758, #25425, #3623 ) ;
#1621=( BOUNDED_CURVE ( )  B_SPLINE_CURVE ( 2, ( #67884, #27269, #44959, #20901, #21253, #16375, #39317 ),
 .UNSPECIFIED., .F., .F. ) 
 B_SPLINE_CURVE_WITH_KNOTS ( ( 3, 2, 2, 3 ),
 ( 0.06350193517771154927, 0.07055765540916983380, 0.07761342095008726127, 0.08466915177933910519 ),
 .UNSPECIFIED. ) 
 CURVE ( )  GEOMETRIC_REPRESENTATION_ITEM ( )  RATIONAL_B_SPLINE_CURVE ( ( 0.9999982793426236416, 0.8660262641186515786, 1.000000000000000000, 0.8660254037844387076, 1.000000000000000000, 0.8660260628881676359, 0.9999986817990271781 ) ) 
 REPRESENTATION_ITEM ( '' )  );
#1622=CARTESIAN_POINT ( 'NONE',  ( 94.70433044323989691, 87.37275709988163896, 74.99300273738302280 ) ) ;
#1628=CARTESIAN_POINT ( 'NONE',  ( 95.00000000000000000, -212.6630814284392557, 82.18156250086714465 ) ) ;
#1632=LINE ( 'NONE', #2734, #4166 ) ;
#1636=DIRECTION ( 'NONE',  ( 0.4565542962317865050, 0.000000000000000000, 0.8896955516311735312 ) ) ;
#1637=CARTESIAN_POINT ( 'NONE',  ( -96.15314808468745866, -211.9973110713294489, 85.93864583420048575 ) ) ;
#1638=CARTESIAN_POINT ( 'NONE',  ( -95.00000000000002842, 92.66308142843932671, 83.29281250086717137 ) ) ;
#1640=CARTESIAN_POINT ( 'NONE',  ( 92.69370383062498320, 88.66845928578037217, 79.53572916753380184 ) ) ;
#1647=CARTESIAN_POINT ( 'NONE',  ( -97.30629616937495996, -209.9999999999999716, 84.56281250086713897 ) ) ;
#1649=EDGE_CURVE ( 'NONE', #6687, #39397, #29244, .T. ) ;
#1650=CARTESIAN_POINT ( 'NONE',  ( 92.35000000003287823, 90.00000839536618003, 84.99910573348789455 ) ) ;
#1658=CARTESIAN_POINT ( 'NONE',  ( -97.65000000000001990, 91.52997821335253548, 75.97708333333333997 ) ) ;
#1660=CARTESIAN_POINT ( 'NONE',  ( -97.30629616937501680, 90.00000000000004263, 88.37281250086715545 ) ) ;
#1666=ORIENTED_EDGE ( 'NONE', *, *, #39550, .T. ) ;
#1667=CARTESIAN_POINT ( 'NONE',  ( -95.00000000000002842, 87.33691857156074434, 75.83156250086715033 ) ) ;
#1670=CARTESIAN_POINT ( 'NONE',  ( 93.67500000000001137, -207.7050326799711968, 84.25854166840096582 ) ) ;
#1671=CARTESIAN_POINT ( 'NONE',  ( -15.70000000000000284, -120.0000000000000000, -90.00000000000000000 ) ) ;
#1672=CARTESIAN_POINT ( 'NONE',  ( -92.69370383062498320, -209.9999999999999716, 85.67406250086715147 ) ) ;
#1678=CARTESIAN_POINT ( 'NONE',  ( 2.500000000000029754, 73.00000000000001421, -258.2999999999999545 ) ) ;
#1679=CARTESIAN_POINT ( 'NONE',  ( -97.30629616937495996, -209.9999999999999716, 77.73656250086715147 ) ) ;
#1680=CARTESIAN_POINT ( 'NONE',  ( 93.67499999999998295, 92.29496732002878900, 88.62416666666665321 ) ) ;
#1684=CARTESIAN_POINT ( 'NONE',  ( 96.32499999999997442, 92.29496732002878900, 85.42270833506762528 ) ) ;
#1686=VECTOR ( 'NONE', #33317, 1000.000000000000000 ) ;
#1689=CARTESIAN_POINT ( 'NONE',  ( 92.69370383062501162, -209.9999999999999716, 77.57781250086713953 ) ) ;
#1697=CARTESIAN_POINT ( 'NONE',  ( -97.64998344411506537, 91.52998777189718282, 79.23145767387349281 ) ) ;
#1701=CARTESIAN_POINT ( 'NONE',  ( -97.64999999996712177, 90.00000839536629371, 84.99910573348492449 ) ) ;
#1702=ORIENTED_EDGE ( 'NONE', *, *, #65557, .T. ) ;
#1705=CARTESIAN_POINT ( 'NONE',  ( 92.69370383062498320, 91.33154071421968467, 79.58864583420047722 ) ) ;
#1711=DIRECTION ( 'NONE',  ( -0.000000000000000000, -0.000000000000000000, 1.000000000000000000 ) ) ;
#1718=CARTESIAN_POINT ( 'NONE',  ( -0.0004442498525516064278, 0.001194404164626844313, -90.00000000000000000 ) ) ;
#1720=CARTESIAN_POINT ( 'NONE',  ( 94.99999999999998579, 93.05995642670504253, 77.77624999999999034 ) ) ;
#1721=CARTESIAN_POINT ( 'NONE',  ( -94.99999999999997158, -206.9400435732949575, 79.76062500173429726 ) ) ;
#1724=CARTESIAN_POINT ( 'NONE',  ( 92.69370383062498320, 90.00000000000002842, 89.64281250086713726 ) ) ;
#1725=CARTESIAN_POINT ( 'NONE',  ( -95.00000000000002842, 86.94004357329504273, 75.63312500173429953 ) ) ;
#1728=CARTESIAN_POINT ( 'NONE',  ( 94.99999999999998579, 87.33691857156068750, 79.80031250086715033 ) ) ;
#1729=VECTOR ( 'NONE', #24933, 1000.000000000000000 ) ;
#1730=CARTESIAN_POINT ( 'NONE',  ( -97.64999999999996305, -209.9999999999999716, 82.37999999999999545 ) ) ;
#1741=ORIENTED_EDGE ( 'NONE', *, *, #25450, .T. ) ;
#1742=EDGE_CURVE ( 'NONE', #2166, #43747, #62203, .T. ) ;
#1744=EDGE_CURVE ( 'NONE', #52184, #4841, #67009, .T. ) ;
#1749=CARTESIAN_POINT ( 'NONE',  ( -93.84685191531248449, -208.0026889286704943, 77.52489583420047836 ) ) ;
#1759=CYLINDRICAL_SURFACE ( 'NONE', #69719, 2.649999999999999467 ) ;
#1761=FACE_OUTER_BOUND ( 'NONE', #45328, .T. ) ;
#1766=CARTESIAN_POINT ( 'NONE',  ( 97.30629616937498838, 91.33154071421968467, 85.09197916753380753 ) ) ;
#1767=CARTESIAN_POINT ( 'NONE',  ( -92.69370383062498320, -208.6684592857803295, 86.99697916753382287 ) ) ;
#1770=CARTESIAN_POINT ( 'NONE',  ( -96.32500000000001705, 92.29496732002878900, 81.63916666666666799 ) ) ;
#1771=CARTESIAN_POINT ( 'NONE',  ( -97.64999999999996305, -209.9999999999999716, 81.10999999999999943 ) ) ;
#1772=CARTESIAN_POINT ( 'NONE',  ( -97.30629616937501680, 90.00000000000004263, 76.30781250086714351 ) ) ;
#1776=CARTESIAN_POINT ( 'NONE',  ( 97.30629616937498838, -211.3315407142195852, 86.73239583420047438 ) ) ;
#1787=VERTEX_POINT ( 'NONE', #50807 ) ;
#1790=CARTESIAN_POINT ( 'NONE',  ( 92.69370383062501162, -208.6684592857803295, 82.12864583420048348 ) ) ;
#1792=CARTESIAN_POINT ( 'NONE',  ( 92.34999999999999432, 90.00000000000002842, 81.10999999999999943 ) ) ;
#1795=CARTESIAN_POINT ( 'NONE',  ( 92.35000000000000853, -209.9999999999999716, 85.55499999999999261 ) ) ;
#1798=ORIENTED_EDGE ( 'NONE', *, *, #2824, .T. ) ;
#1800=VERTEX_POINT ( 'NONE', #51930 ) ;
#1802=CARTESIAN_POINT ( 'NONE',  ( -93.84685191531252713, 88.00268892867056536, 88.10822916753382117 ) ) ;
#1806=CARTESIAN_POINT ( 'NONE',  ( 93.84685191531251292, -211.9973110713294489, 87.84364583420047268 ) ) ;
#1807=CARTESIAN_POINT ( 'NONE',  ( 93.67499999999999716, 87.70503267997126784, 79.31083333333333485 ) ) ;
#1810=CARTESIAN_POINT ( 'NONE',  ( -96.32499999999996021, -207.7050326799711968, 88.06854166840095388 ) ) ;
#1814=CARTESIAN_POINT ( 'NONE',  ( -97.65000000000001990, 88.47002178664754979, 86.32229166840097889 ) ) ;
#1815=CARTESIAN_POINT ( 'NONE',  ( 93.84685191531248449, 91.99731107132950569, 89.69572916753382685 ) ) ;
#1818=ADVANCED_FACE ( 'NONE', ( #69598 ), #6092, .F. ) ;
#1820=CARTESIAN_POINT ( 'NONE',  ( 95.00000000000000000, -209.9999999999999716, 90.00000000000000000 ) ) ;
#1824=CARTESIAN_POINT ( 'NONE',  ( -97.64999999993855795, 90.00001182123732235, 81.82400613091868991 ) ) ;
#1825=AXIS2_PLACEMENT_3D ( 'NONE', #50580, #21252, #39316 ) ;
#1831=CARTESIAN_POINT ( 'NONE',  ( -97.30629616937497417, -211.3315407142195852, 88.58447916753382856 ) ) ;
#1834=EDGE_CURVE ( 'NONE', #56117, #3345, #113, .T. ) ;
#1843=CARTESIAN_POINT ( 'NONE',  ( 93.84685191531248449, 91.99731107132950569, 80.01197916753380923 ) ) ;
#1853=( BOUNDED_CURVE ( )  B_SPLINE_CURVE ( 2, ( #56734, #57097, #61995, #5234, #68384, #362, #28133 ),
 .UNSPECIFIED., .F., .F. ) 
 B_SPLINE_CURVE_WITH_KNOTS ( ( 3, 2, 2, 3 ),
 ( 0.7708333333333328152, 0.7777777777777775681, 0.7847222222222222099, 0.7916666666666669627 ),
 .UNSPECIFIED. ) 
 CURVE ( )  GEOMETRIC_REPRESENTATION_ITEM ( )  RATIONAL_B_SPLINE_CURVE ( ( 1.000000000000010658, 0.8660254037844280495, 1.000000000000000000, 0.8660254037844387076, 1.000000000000000000, 0.8660254037844322683, 1.000000000000006439 ) ) 
 REPRESENTATION_ITEM ( '' )  );
#1859=CARTESIAN_POINT ( 'NONE',  ( -96.15314808468751551, 88.00268892867056536, 87.20864583420046756 ) ) ;
#1869=CARTESIAN_POINT ( 'NONE',  ( 96.15314808468748708, -208.0026889286704943, 81.96989583420048575 ) ) ;
#1871=ORIENTED_EDGE ( 'NONE', *, *, #11857, .F. ) ;
#1873=DIRECTION ( 'NONE',  ( -0.000000000000000000, -0.000000000000000000, -1.000000000000000000 ) ) ;
#1875=CARTESIAN_POINT ( 'NONE',  ( 92.35000000000000853, -209.9999999999999716, 88.73000000000000398 ) ) ;
#1876=CARTESIAN_POINT ( 'NONE',  ( 92.69370383062501162, -208.6684592857803295, 76.25489583420049655 ) ) ;
#1878=ORIENTED_EDGE ( 'NONE', *, *, #4867, .T. ) ;
#1880=CARTESIAN_POINT ( 'NONE',  ( 95.00000000000000000, -212.6630814284392557, 79.80031250086715033 ) ) ;
#1886=CARTESIAN_POINT ( 'NONE',  ( 97.65000000000000568, -208.4700217866474645, 86.63979166840096013 ) ) ;
#1888=ADVANCED_FACE ( 'NONE', ( #34637 ), #56842, .F. ) ;
#1891=CARTESIAN_POINT ( 'NONE',  ( 93.67500000000001137, -207.7050326799711968, 83.62354166840097491 ) ) ;
#1892=CARTESIAN_POINT ( 'NONE',  ( 94.99999999999998579, 93.05995642670504253, 89.20624999999999716 ) ) ;
#1899=ORIENTED_EDGE ( 'NONE', *, *, #7386, .T. ) ;
#1900=CARTESIAN_POINT ( 'NONE',  ( -92.69370383062505425, 88.66845928578038638, 89.43114583420049257 ) ) ;
#1901=CARTESIAN_POINT ( 'NONE',  ( 94.99999999999998579, 87.33691857156068750, 84.08656250086713158 ) ) ;
#1904=CARTESIAN_POINT ( 'NONE',  ( 96.32499999999998863, 87.70503267997126784, 87.11604166840096752 ) ) ;
#1915=CARTESIAN_POINT ( 'NONE',  ( 92.34999999999999432, 91.52997821335252127, 75.42145833506764063 ) ) ;
#1916=CARTESIAN_POINT ( 'NONE',  ( -97.65000000000001990, 88.47002178664754979, 84.97291666666666288 ) ) ;
#1919=DIRECTION ( 'NONE',  ( 1.000000000000000000, 0.000000000000000000, 0.000000000000000000 ) ) ;
#1922=CARTESIAN_POINT ( 'NONE',  ( -96.15314808468747287, -208.0026889286704943, 83.82197916753381151 ) ) ;
#1923=ORIENTED_EDGE ( 'NONE', *, *, #36567, .F. ) ;
#1927=CARTESIAN_POINT ( 'NONE',  ( -92.35000000000003695, 90.00000000000004263, 90.00000000000000000 ) ) ;
#1929=CARTESIAN_POINT ( 'NONE',  ( 97.64999999999447766, 89.99999459739470353, 81.50687481489491404 ) ) ;
#1937=CARTESIAN_POINT ( 'NONE',  ( -92.69370383062504004, 90.00000000000004263, 89.48406250086715374 ) ) ;
#1940=ADVANCED_FACE ( 'NONE', ( #845 ), #22253, .F. ) ;
#1950=CARTESIAN_POINT ( 'NONE',  ( -96.15314808468747287, -208.0026889286704943, 76.36072916753381890 ) ) ;
#1962=ORIENTED_EDGE ( 'NONE', *, *, #51424, .T. ) ;
#1964=CARTESIAN_POINT ( 'NONE',  ( 93.84685191531251292, -211.9973110713294489, 86.57364583420047666 ) ) ;
#1965=CARTESIAN_POINT ( 'NONE',  ( 92.69370383062501162, -208.6684592857803295, 89.74864583420048803 ) ) ;
#1967=ADVANCED_FACE ( 'NONE', ( #36117 ), #41392, .F. ) ;
#1970=CARTESIAN_POINT ( 'NONE',  ( -92.34999999999999432, -209.9999999999999716, 80.79249999999998977 ) ) ;
#1972=CARTESIAN_POINT ( 'NONE',  ( -92.69370383062504004, 90.00000000000004263, 81.22906250086715829 ) ) ;
#1976=DIRECTION ( 'NONE',  ( -1.000000000000000000, -0.000000000000000000, -0.000000000000000000 ) ) ;
#1982=ORIENTED_EDGE ( 'NONE', *, *, #9744, .F. ) ;
#1986=ADVANCED_FACE ( 'NONE', ( #71421 ), #24117, .F. ) ;
#1987=ORIENTED_EDGE ( 'NONE', *, *, #10454, .T. ) ;
#1989=CARTESIAN_POINT ( 'NONE',  ( 95.00000000000000000, -207.3369185715606307, 79.95906250086713385 ) ) ;
#1993=LINE ( 'NONE', #8337, #11259 ) ;
#2000=CARTESIAN_POINT ( 'NONE',  ( -94.99999999999997158, -212.6630814284392557, 80.27656250086714351 ) ) ;
#2001=CARTESIAN_POINT ( 'NONE',  ( -95.00000000000002842, 87.33691857156074434, 80.43531250086715545 ) ) ;
#2005=CARTESIAN_POINT ( 'NONE',  ( 97.30629616937498838, 90.00000000000002842, 82.34031250086714238 ) ) ;
#2014=CARTESIAN_POINT ( 'NONE',  ( -94.99999999999997158, -207.3369185715606307, 82.49906250086715431 ) ) ;
#2026=CARTESIAN_POINT ( 'NONE',  ( -95.00000000000002842, 87.33691857156074434, 85.99156250086714692 ) ) ;
#2032=CARTESIAN_POINT ( 'NONE',  ( -97.30629616937501680, 90.00000000000004263, 75.67281250086713840 ) ) ;
#2039=CARTESIAN_POINT ( 'NONE',  ( -93.84685191531248449, -208.0026889286704943, 86.41489583420049314 ) ) ;
#2044=CARTESIAN_POINT ( 'NONE',  ( -96.15314808468747287, -208.0026889286704943, 76.36072916753381890 ) ) ;
#2048=CARTESIAN_POINT ( 'NONE',  ( -97.64999999999996305, -209.9999999999999716, 81.82437500173429612 ) ) ;
#2049=CARTESIAN_POINT ( 'NONE',  ( 92.34999999999990905, 91.52997821335249284, 75.97708333333333997 ) ) ;
#2050=CARTESIAN_POINT ( 'NONE',  ( 97.64999999999990621, 90.00000071509185773, 85.31687502647973531 ) ) ;
#2054=CARTESIAN_POINT ( 'NONE',  ( 96.15314808468750130, -211.9973110713294489, 76.51947916753380241 ) ) ;
#2060=( BOUNDED_CURVE ( )  B_SPLINE_CURVE ( 2, ( #61830, #44538, #55436, #21584, #72349, #38141, #38891 ),
 .UNSPECIFIED., .F., .F. ) 
 B_SPLINE_CURVE_WITH_KNOTS ( ( 3, 2, 2, 3 ),
 ( 0.2708333333333337034, 0.2777777777777781232, 0.2847222222222224874, 0.2916666666666669072 ),
 .UNSPECIFIED. ) 
 CURVE ( )  GEOMETRIC_REPRESENTATION_ITEM ( )  RATIONAL_B_SPLINE_CURVE ( ( 0.9999999999999924505, 0.8660254037844462571, 1.000000000000000000, 0.8660254037844387076, 1.000000000000000000, 0.8660254037844343777, 1.000000000000004219 ) ) 
 REPRESENTATION_ITEM ( '' )  );
#2064=DIRECTION ( 'NONE',  ( -0.000000000000000000, 0.000000000000000000, 1.000000000000000000 ) ) ;
#2069=ADVANCED_FACE ( 'NONE', ( #30464 ), #53413, .F. ) ;
#2071=FACE_OUTER_BOUND ( 'NONE', #69092, .T. ) ;
#2073=ORIENTED_EDGE ( 'NONE', *, *, #17898, .F. ) ;
#2075=CARTESIAN_POINT ( 'NONE',  ( 93.84685191531248449, 91.99731107132950569, 80.17072916753382117 ) ) ;
#2076=CARTESIAN_POINT ( 'NONE',  ( 97.64999999964365429, -210.0000434577794408, 89.12687334326047051 ) ) ;
#2080=VERTEX_POINT ( 'NONE', #31216 ) ;
#2088=DIRECTION ( 'NONE',  ( 1.000000000000000000, 0.000000000000000000, 0.000000000000000000 ) ) ;
#2091=CARTESIAN_POINT ( 'NONE',  ( -97.64999999999996305, -209.9999999999999716, 80.55437500173430010 ) ) ;
#2093=CARTESIAN_POINT ( 'NONE',  ( 94.99999999999998579, 93.05995642670504253, 75.95062500173428077 ) ) ;
#2094=CARTESIAN_POINT ( 'NONE',  ( -93.67500000000003979, 92.29496732002878900, 74.62770833506762358 ) ) ;
#2096=CARTESIAN_POINT ( 'NONE',  ( 92.69370383062498320, 91.33154071421968467, 75.14364583420049826 ) ) ;
#2115=PLANE ( 'NONE',  #73532 ) ;
#2116=VECTOR ( 'NONE', #18095, 1000.000000000000000 ) ;
#2118=CARTESIAN_POINT ( 'NONE',  ( -93.67499999999998295, -207.7050326799711968, 75.81833333333332803 ) ) ;
#2119=CARTESIAN_POINT ( 'NONE',  ( -92.69370383062498320, -209.9999999999999716, 76.78406250086715090 ) ) ;
#2120=VERTEX_POINT ( 'NONE', #32682 ) ;
#2133=CARTESIAN_POINT ( 'NONE',  ( 93.84685191531248449, 91.99731107132950569, 85.25072916753381946 ) ) ;
#2134=CARTESIAN_POINT ( 'NONE',  ( -97.30629616937495996, -209.9999999999999716, 87.26156250086715715 ) ) ;
#2138=CARTESIAN_POINT ( 'NONE',  ( -92.34999999999999432, -209.9999999999999716, 82.06250000000000000 ) ) ;
#2139=CARTESIAN_POINT ( 'NONE',  ( -96.15314808468752972, 91.99731107132950569, 75.56697916753381605 ) ) ;
#2140=CARTESIAN_POINT ( 'NONE',  ( 92.69370383062501162, -208.6684592857803011, 85.77989583420048803 ) ) ;
#2151=EDGE_CURVE ( 'NONE', #37629, #51617, #36609, .T. ) ;
#2157=CARTESIAN_POINT ( 'NONE',  ( 96.15314808468750130, -211.9973110713294489, 77.31322916753381946 ) ) ;
#2164=CARTESIAN_POINT ( 'NONE',  ( 95.00000000000000000, -213.0599564267049857, 83.17374999999999829 ) ) ;
#2166=VERTEX_POINT ( 'NONE', #31947 ) ;
#2170=CARTESIAN_POINT ( 'NONE',  ( -97.64997399525502431, -211.5299932271988723, 86.32229270695523837 ) ) ;
#2172=CARTESIAN_POINT ( 'NONE',  ( -96.15314808468752972, 91.99731107132950569, 84.61572916753381435 ) ) ;
#2179=DIRECTION ( 'NONE',  ( -1.000000000000000000, -0.000000000000000000, -0.000000000000000000 ) ) ;
#2180=ORIENTED_EDGE ( 'NONE', *, *, #58720, .T. ) ;
#2184=CARTESIAN_POINT ( 'NONE',  ( -96.32500000000001705, 92.29496732002878900, 86.79854166840097207 ) ) ;
#2186=CARTESIAN_POINT ( 'NONE',  ( 96.15314808468748708, 91.99731107132950569, 86.41489583420049314 ) ) ;
#2187=PLANE ( 'NONE',  #44209 ) ;
#2191=ORIENTED_EDGE ( 'NONE', *, *, #47228, .T. ) ;
#2200=CARTESIAN_POINT ( 'NONE',  ( -97.65000000000001990, 90.00000000000004263, 75.47437500173430180 ) ) ;
#2201=CARTESIAN_POINT ( 'NONE',  ( -92.69370383062498320, -208.6684592857803011, 88.26697916753381890 ) ) ;
#2207=VECTOR ( 'NONE', #33319, 1000.000000000000000 ) ;
#2210=CARTESIAN_POINT ( 'NONE',  ( 94.99999999999998579, 93.05995642670504253, 86.66624999999999091 ) ) ;
#2213=CARTESIAN_POINT ( 'NONE',  ( 97.30629616937498838, 90.00000000000002842, 82.97531250086714749 ) ) ;
#2216=DIRECTION ( 'NONE',  ( -0.000000000000000000, -0.000000000000000000, 1.000000000000000000 ) ) ;
#2218=CARTESIAN_POINT ( 'NONE',  ( -92.35000000000005116, 88.47002178664754979, 77.00895833506763211 ) ) ;
#2220=DIRECTION ( 'NONE',  ( 1.000000000000000000, 0.000000000000000000, 0.000000000000000000 ) ) ;
#2221=CARTESIAN_POINT ( 'NONE',  ( 92.35000000000000853, -208.4700217866474645, 85.58145833506763722 ) ) ;
#2223=ORIENTED_EDGE ( 'NONE', *, *, #63704, .T. ) ;
#2224=CARTESIAN_POINT ( 'NONE',  ( -93.84685191531254134, 91.99731107132950569, 86.89114583420047211 ) ) ;
#2225=DIRECTION ( 'NONE',  ( -1.000000000000000000, -0.000000000000000000, -0.000000000000000000 ) ) ;
#2226=ADVANCED_FACE ( 'NONE', ( #72533 ), #60186, .F. ) ;
#2229=EDGE_CURVE ( 'NONE', #46998, #14970, #33054, .T. ) ;
#2231=EDGE_CURVE ( 'NONE', #25802, #52184, #66907, .T. ) ;
#2237=EDGE_CURVE ( 'NONE', #44790, #71356, #42871, .T. ) ;
#2238=CARTESIAN_POINT ( 'NONE',  ( 93.84685191531251292, -211.9973110713294489, 83.55739583420049144 ) ) ;
#2242=CYLINDRICAL_SURFACE ( 'NONE', #47591, 2.649999999999985700 ) ;
#2245=DIRECTION ( 'NONE',  ( -0.000000000000000000, -0.000000000000000000, 1.000000000000000000 ) ) ;
#2249=CARTESIAN_POINT ( 'NONE',  ( 92.69370383062501162, -209.9999999999999716, 79.64156250086715261 ) ) ;
#2250=VECTOR ( 'NONE', #24283, 1000.000000000000000 ) ;
#2253=CARTESIAN_POINT ( 'NONE',  ( 96.32499999999998863, 87.70503267997126784, 79.41666666666665719 ) ) ;
#2258=CARTESIAN_POINT ( 'NONE',  ( 96.32499999999998863, -207.7050326799711968, 80.26333333333332121 ) ) ;
#2259=ORIENTED_EDGE ( 'NONE', *, *, #58765, .T. ) ;
#2260=CARTESIAN_POINT ( 'NONE',  ( -96.32500000000001705, 92.29496732002878900, 84.17916666666666003 ) ) ;
#2261=CARTESIAN_POINT ( 'NONE',  ( 97.64999999999997726, -208.4700217866474645, 82.82979166840095786 ) ) ;
#2262=CARTESIAN_POINT ( 'NONE',  ( 94.99999999999998579, 93.05995642670504253, 84.12625000000001307 ) ) ;
#2269=VERTEX_POINT ( 'NONE', #23284 ) ;
#2270=CARTESIAN_POINT ( 'NONE',  ( -97.30629616937501680, 91.33154071421968467, 89.11364583420049712 ) ) ;
#2271=CARTESIAN_POINT ( 'NONE',  ( 92.69370383062498320, 88.66845928578037217, 81.44072916753381719 ) ) ;
#2273=CARTESIAN_POINT ( 'NONE',  ( 97.64999999999997726, 88.47002178664753558, 85.89895833506764689 ) ) ;
#2279=ORIENTED_EDGE ( 'NONE', *, *, #8294, .F. ) ;
#2282=CARTESIAN_POINT ( 'NONE',  ( 96.32499999999997442, 92.29496732002878900, 75.26270833506764291 ) ) ;
#2285=CARTESIAN_POINT ( 'NONE',  ( -95.00000000000002842, 93.05995642670501411, 83.49125000000000796 ) ) ;
#2287=CARTESIAN_POINT ( 'NONE',  ( 96.73972734126401463, 91.51405112163766375, 74.79348190356853365 ) ) ;
#2291=( BOUNDED_CURVE ( )  B_SPLINE_CURVE ( 2, ( #27012, #72860, #38309, #31916, #49574, #20265, #44324 ),
 .UNSPECIFIED., .F., .F. ) 
 B_SPLINE_CURVE_WITH_KNOTS ( ( 3, 2, 2, 3 ),
 ( 0.5503499107253647660, 0.5574054777324447540, 0.5644612432733617791, 0.5715170088694363493 ),
 .UNSPECIFIED. ) 
 CURVE ( )  GEOMETRIC_REPRESENTATION_ITEM ( )  RATIONAL_B_SPLINE_CURVE ( ( 0.9999924607068964022, 0.8660291735370631017, 1.000000000000000000, 0.8660254037844387076, 1.000000000000000000, 0.8660254037844387076, 1.000000000000000000 ) ) 
 REPRESENTATION_ITEM ( '' )  );
#2293=CARTESIAN_POINT ( 'NONE',  ( -92.69370383062498320, -211.3315407142195852, 83.55739583420047722 ) ) ;
#2294=VERTEX_POINT ( 'NONE', #16906 ) ;
#2301=CARTESIAN_POINT ( 'NONE',  ( 97.01450244679210755, -211.1324117838501877, 74.79348190356851944 ) ) ;
#2306=CARTESIAN_POINT ( 'NONE',  ( -97.30629616937501680, 90.00000000000004263, 76.30781250086714351 ) ) ;
#2316=CARTESIAN_POINT ( 'NONE',  ( 92.35000000000000853, -209.9999999999999716, 77.29999999999999716 ) ) ;
#2318=CARTESIAN_POINT ( 'NONE',  ( 97.64999999999999147, 90.00000000000002842, 90.00000000000000000 ) ) ;
#2319=CARTESIAN_POINT ( 'NONE',  ( -92.34999999999999432, -211.5299782133524502, 89.62958333333332916 ) ) ;
#2323=DIRECTION ( 'NONE',  ( -0.000000000000000000, -0.000000000000000000, 1.000000000000000000 ) ) ;
#2327=CARTESIAN_POINT ( 'NONE',  ( 97.64999999999999147, -209.9999999999999716, 76.34749999999999659 ) ) ;
#2341=CARTESIAN_POINT ( 'NONE',  ( 93.84685191531249870, -208.0026889286704943, 83.18697916753382060 ) ) ;
#2342=CARTESIAN_POINT ( 'NONE',  ( 97.30629616937498838, -209.9999999999999716, 87.57906250086715261 ) ) ;
#2343=EDGE_CURVE ( 'NONE', #62638, #43916, #41555, .T. ) ;
#2348=CARTESIAN_POINT ( 'NONE',  ( -95.00000000000002842, 87.33691857156074434, 77.26031250086714408 ) ) ;
#2356=VERTEX_POINT ( 'NONE', #5634 ) ;
#2357=PLANE ( 'NONE',  #10599 ) ;
#2368=CARTESIAN_POINT ( 'NONE',  ( 93.84685191531249870, -208.0026889286704943, 76.83697916753381207 ) ) ;
#2376=CARTESIAN_POINT ( 'NONE',  ( -92.34999999999999432, -209.9999999999999716, 75.71250000000000568 ) ) ;
#2379=CARTESIAN_POINT ( 'NONE',  ( -92.69370383062498320, -211.3315407142195852, 80.38239583420049428 ) ) ;
#2380=CARTESIAN_POINT ( 'NONE',  ( -92.69370383062502583, 91.33154071421968467, 79.37697916753381833 ) ) ;
#2382=CARTESIAN_POINT ( 'NONE',  ( 94.99999999999998579, 92.66308142843935514, 80.59406250086715318 ) ) ;
#2384=CARTESIAN_POINT ( 'NONE',  ( 93.67499999999998295, 92.29496732002878900, 78.54354166840096241 ) ) ;
#2389=CARTESIAN_POINT ( 'NONE',  ( -93.84685191531247028, -211.9973110713294489, 83.50447916753381605 ) ) ;
#2403=CARTESIAN_POINT ( 'NONE',  ( -96.15314808468751551, 88.00268892867056536, 86.57364583420047666 ) ) ;
#2408=CARTESIAN_POINT ( 'NONE',  ( -92.69370383062504004, 90.00000000000004263, 74.72031250086713783 ) ) ;
#2409=EDGE_CURVE ( 'NONE', #19936, #50232, #5563, .T. ) ;
#2414=CARTESIAN_POINT ( 'NONE',  ( -97.64999999999996305, -209.9999999999999716, 76.03000000000000114 ) ) ;
#2415=CARTESIAN_POINT ( 'NONE',  ( -93.84685191531247028, -211.9973110713294489, 82.39322916753381776 ) ) ;
#2417=EDGE_CURVE ( 'NONE', #23688, #40782, #10815, .T. ) ;
#2421=CARTESIAN_POINT ( 'NONE',  ( 94.99999999999998579, 92.66308142843932671, 75.03781250086714749 ) ) ;
#2422=AXIS2_PLACEMENT_3D ( 'NONE', #44885, #32469, #32835 ) ;
#2423=CARTESIAN_POINT ( 'NONE',  ( -92.69370383062498320, -208.6684592857803295, 76.20197916753382117 ) ) ;
#2433=CARTESIAN_POINT ( 'NONE',  ( 92.69370383062501162, -209.9999999999999716, 88.53156250086716739 ) ) ;
#2434=EDGE_LOOP ( 'NONE', ( #65330, #60143, #52415, #7736 ) ) ;
#2441=EDGE_CURVE ( 'NONE', #8621, #33107, #31119, .T. ) ;
#2445=CARTESIAN_POINT ( 'NONE',  ( 0.000000000000000000, 0.000000000000000000, -90.00000000000000000 ) ) ;
#2450=EDGE_LOOP ( 'NONE', ( #72929, #48162 ) ) ;
#2454=LINE ( 'NONE', #24953, #27482 ) ;
#2455=ADVANCED_FACE ( 'NONE', ( #13821 ), #70220, .F. ) ;
#2458=CARTESIAN_POINT ( 'NONE',  ( 97.30629616937498838, 90.00000000000002842, 80.59406250086715318 ) ) ;
#2471=CYLINDRICAL_SURFACE ( 'NONE', #41864, 2.649999999999985700 ) ;
#2472=CARTESIAN_POINT ( 'NONE',  ( -96.32499999999996021, -207.7050326799711968, 76.63854166840096127 ) ) ;
#2473=CARTESIAN_POINT ( 'NONE',  ( -97.30629616937501680, 90.00000000000004263, 89.80156250086714920 ) ) ;
#2474=CARTESIAN_POINT ( 'NONE',  ( 92.34999999999999432, 88.47002178664753558, 75.52729166840099140 ) ) ;
#2475=CARTESIAN_POINT ( 'NONE',  ( -96.32500000000001705, 87.70503267997129626, 76.21520833506762926 ) ) ;
#2478=CARTESIAN_POINT ( 'NONE',  ( 97.30629616937498838, 91.33154071421968467, 76.20197916753382117 ) ) ;
#2479=CARTESIAN_POINT ( 'NONE',  ( 93.67499999999998295, 92.29496732002878900, 82.27416666666665890 ) ) ;
#2486=CARTESIAN_POINT ( 'NONE',  ( -97.64999999999996305, -209.9999999999999716, 87.45999999999999375 ) ) ;
#2488=CYLINDRICAL_SURFACE ( 'NONE', #61222, 2.649999999999999467 ) ;
#2490=ORIENTED_EDGE ( 'NONE', *, *, #28162, .F. ) ;
#2497=CARTESIAN_POINT ( 'NONE',  ( -97.30629616937497417, -208.6684592857803011, 75.77864583420048916 ) ) ;
#2504=LINE ( 'NONE', #12977, #33234 ) ;
#2516=( BOUNDED_CURVE ( )  B_SPLINE_CURVE ( 2, ( #11798, #69329, #5825, #17096, #219, #23471, #21985 ),
 .UNSPECIFIED., .F., .F. ) 
 B_SPLINE_CURVE_WITH_KNOTS ( ( 3, 2, 2, 3 ),
 ( 0.9583333333333337034, 0.9652777777777781232, 0.9722222222222225430, 0.9791666666666669627 ),
 .UNSPECIFIED. ) 
 CURVE ( )  GEOMETRIC_REPRESENTATION_ITEM ( )  RATIONAL_B_SPLINE_CURVE ( ( 0.9999999999999935607, 0.8660254037844451469, 1.000000000000000000, 0.8660254037844387076, 1.000000000000000000, 0.8660254037844322683, 1.000000000000006439 ) ) 
 REPRESENTATION_ITEM ( '' )  );
#2517=CARTESIAN_POINT ( 'NONE',  ( 97.30629616937498838, 91.33154071421968467, 84.45697916753383083 ) ) ;
#2518=CARTESIAN_POINT ( 'NONE',  ( -94.99999999999997158, -207.3369185715606307, 86.46781250086714010 ) ) ;
#2523=CARTESIAN_POINT ( 'NONE',  ( -94.99999999999997158, -213.0599564267049857, 81.26874999999999716 ) ) ;
#2524=CARTESIAN_POINT ( 'NONE',  ( -92.69370383062505425, 88.66845928578038638, 76.57239583420046358 ) ) ;
#2525=CARTESIAN_POINT ( 'NONE',  ( 92.69370383062501162, -211.3315407142195852, 84.61572916753380014 ) ) ;
#2538=CARTESIAN_POINT ( 'NONE',  ( 95.00000000000000000, -212.6630814284392557, 78.53031250086715431 ) ) ;
#2542=CARTESIAN_POINT ( 'NONE',  ( 97.64999999999999147, -209.9999999999999716, 80.79249999999998977 ) ) ;
#2544=CARTESIAN_POINT ( 'NONE',  ( -95.00000000000002842, 86.94004357329504273, 83.25312500173430408 ) ) ;
#2545=CARTESIAN_POINT ( 'NONE',  ( 97.64999999999999147, -209.9999999999999716, 82.69749999999999091 ) ) ;
#2547=ORIENTED_EDGE ( 'NONE', *, *, #55991, .F. ) ;
#2550=CARTESIAN_POINT ( 'NONE',  ( 2.500000000000035083, 90.00000000000000000, -279.9999999999999432 ) ) ;
#2553=CARTESIAN_POINT ( 'NONE',  ( -93.84685191531252713, 88.00268892867056536, 83.66322916753382799 ) ) ;
#2554=CARTESIAN_POINT ( 'NONE',  ( -93.67499999999998295, -207.7050326799711968, 77.08833333333332405 ) ) ;
#2557=CARTESIAN_POINT ( 'NONE',  ( 96.32499999999998863, 87.70503267997126784, 75.60666666666665492 ) ) ;
#2559=CARTESIAN_POINT ( 'NONE',  ( -96.32499999999996021, -207.7050326799711968, 84.89354166840095672 ) ) ;
#2563=CARTESIAN_POINT ( 'NONE',  ( -92.35000000000003695, 90.00000000000004263, 87.22187500173430408 ) ) ;
#2564=CARTESIAN_POINT ( 'NONE',  ( 94.99999999999998579, 87.33691857156068750, 86.15031250086714465 ) ) ;
#2570=CARTESIAN_POINT ( 'NONE',  ( 94.99999999999998579, 90.00000000000002842, 90.00000000000000000 ) ) ;
#2576=CARTESIAN_POINT ( 'NONE',  ( -97.65000000000004832, -211.5299782133524218, 83.06791666666666174 ) ) ;
#2577=CARTESIAN_POINT ( 'NONE',  ( -97.30629616937497417, -208.6684592857803011, 85.30364583420048064 ) ) ;
#2587=CARTESIAN_POINT ( 'NONE',  ( 94.99999999999998579, 87.33691857156068750, 88.69031250086716511 ) ) ;
#2589=CARTESIAN_POINT ( 'NONE',  ( 92.69370383062498320, 91.33154071421968467, 82.60489583420049087 ) ) ;
#2595=CARTESIAN_POINT ( 'NONE',  ( -97.65000000000001990, 90.00003217427526181, 76.74437388893713319 ) ) ;
#2600=CARTESIAN_POINT ( 'NONE',  ( -97.64999999953592180, 89.99996903277666149, 77.38038495128051864 ) ) ;
#2602=CARTESIAN_POINT ( 'NONE',  ( -92.69370383062505425, 88.66845928578038638, 88.00239583420047040 ) ) ;
#2604=FACE_OUTER_BOUND ( 'NONE', #63993, .T. ) ;
#2606=VECTOR ( 'NONE', #50629, 1000.000000000000000 ) ;
#2612=CARTESIAN_POINT ( 'NONE',  ( -26.50000000000000355, -120.0000000000000000, -80.00000000000000000 ) ) ;
#2616=CARTESIAN_POINT ( 'NONE',  ( 96.15314808468748708, -208.0026889286704943, 80.69989583420047552 ) ) ;
#2625=CARTESIAN_POINT ( 'NONE',  ( 97.30629616937498838, -208.6684592857803011, 77.47197916753381719 ) ) ;
#2627=ORIENTED_EDGE ( 'NONE', *, *, #62325, .T. ) ;
#2629=VERTEX_POINT ( 'NONE', #20206 ) ;
#2636=CARTESIAN_POINT ( 'NONE',  ( 97.64999999999997726, -211.5299782133524502, 83.99395833506763154 ) ) ;
#2637=CARTESIAN_POINT ( 'NONE',  ( 97.64999999999999147, 90.00000000000002842, 83.96750000000000114 ) ) ;
#2644=CARTESIAN_POINT ( 'NONE',  ( -93.84685191531254134, 91.99731107132950569, 88.31989583420048007 ) ) ;
#2645=CARTESIAN_POINT ( 'NONE',  ( 94.99999999999998579, 87.33691857156068750, 80.27656250086714351 ) ) ;
#2647=CARTESIAN_POINT ( 'NONE',  ( 94.99999999999998579, 93.05995642670504253, 82.30062500173428930 ) ) ;
#2650=CARTESIAN_POINT ( 'NONE',  ( -92.34999999999999432, -209.9999999999999716, 86.50750000000000739 ) ) ;
#2659=CARTESIAN_POINT ( 'NONE',  ( -95.00000000000002842, 86.94004357329504273, 85.07874999999999943 ) ) ;
#2663=ORIENTED_EDGE ( 'NONE', *, *, #20184, .T. ) ;
#2665=CARTESIAN_POINT ( 'NONE',  ( -92.69370383062498320, -208.6684592857803011, 78.58322916753381548 ) ) ;
#2672=CARTESIAN_POINT ( 'NONE',  ( 93.67500000000001137, -207.7050326799711968, 83.62354166840097491 ) ) ;
#2678=EDGE_CURVE ( 'NONE', #23574, #16444, #67840, .T. ) ;
#2679=CARTESIAN_POINT ( 'NONE',  ( -95.00000000000002842, 87.33691857156074434, 89.32531250086715602 ) ) ;
#2688=CARTESIAN_POINT ( 'NONE',  ( 93.84685191531248449, 91.99731107132950569, 89.06072916753382174 ) ) ;
#2693=CARTESIAN_POINT ( 'NONE',  ( -92.34999999999999432, -209.9999999999999716, 88.41249999999999432 ) ) ;
#2701=CARTESIAN_POINT ( 'NONE',  ( 92.35001072685611234, -211.5299844065056902, 78.06729209680055703 ) ) ;
#2705=DIRECTION ( 'NONE',  ( 0.000000000000000000, -1.000000000000000000, 0.000000000000000000 ) ) ;
#2707=CARTESIAN_POINT ( 'NONE',  ( 95.00000000000000000, -207.3369185715606307, 82.49906250086715431 ) ) ;
#2708=CARTESIAN_POINT ( 'NONE',  ( 92.69370383062501162, -209.9999999999999716, 89.80156250086714920 ) ) ;
#2714=CARTESIAN_POINT ( 'NONE',  ( -96.15314808468752972, 91.99731107132950569, 78.26572916753382003 ) ) ;
#2724=( BOUNDED_CURVE ( )  B_SPLINE_CURVE ( 2, ( #35371, #52653, #41380, #460, #58665, #17703, #12062 ),
 .UNSPECIFIED., .F., .F. ) 
 B_SPLINE_CURVE_WITH_KNOTS ( ( 3, 2, 2, 3 ),
 ( 0.1041666666666670182, 0.1111111111111114103, 0.1180555555555558161, 0.1250000000000002220 ),
 .UNSPECIFIED. ) 
 CURVE ( )  GEOMETRIC_REPRESENTATION_ITEM ( )  RATIONAL_B_SPLINE_CURVE ( ( 0.9999999999999933387, 0.8660254037844453689, 1.000000000000000000, 0.8660254037844387076, 1.000000000000000000, 0.8660254037844343777, 1.000000000000004219 ) ) 
 REPRESENTATION_ITEM ( '' )  );
#2731=CARTESIAN_POINT ( 'NONE',  ( 92.69370383062501162, -209.9999999999999716, 78.21281250086714465 ) ) ;
#2734=CARTESIAN_POINT ( 'NONE',  ( 97.64999999999999147, 90.00000000000002842, 90.00000000000000000 ) ) ;
#2737=CARTESIAN_POINT ( 'NONE',  ( -92.34999999999999432, -211.5299782133524218, 78.91395833506763324 ) ) ;
#2740=CYLINDRICAL_SURFACE ( 'NONE', #69209, 2.649999999999999467 ) ;
#2744=CARTESIAN_POINT ( 'NONE',  ( -94.99999999999997158, -207.3369185715606307, 80.59406250086715318 ) ) ;
#2746=CARTESIAN_POINT ( 'NONE',  ( -92.69370383062502583, 88.66845928578038638, 80.54114583420049200 ) ) ;
#2749=CARTESIAN_POINT ( 'NONE',  ( 92.69370383062498320, 91.33154071421968467, 81.33489583420048064 ) ) ;
#2754=CARTESIAN_POINT ( 'NONE',  ( -96.32499999999996021, -212.2949673200287179, 76.77083333333332860 ) ) ;
#2757=CARTESIAN_POINT ( 'NONE',  ( -97.30629616937497417, -211.3315407142195852, 81.44072916753380298 ) ) ;
#2765=CARTESIAN_POINT ( 'NONE',  ( -97.65000000000001990, 88.47002178664754979, 75.44791666666667140 ) ) ;
#2767=CARTESIAN_POINT ( 'NONE',  ( -93.84685191531254134, 91.99731107132950569, 83.71614583420047495 ) ) ;
#2768=CARTESIAN_POINT ( 'NONE',  ( -97.19210266091309336, -208.8322938842643168, 74.89296886168689582 ) ) ;
#2773=CARTESIAN_POINT ( 'NONE',  ( -92.69370383062504004, 89.06968361095763953, 74.68334086212732359 ) ) ;
#2776=CYLINDRICAL_SURFACE ( 'NONE', #58571, 2.649999999999985700 ) ;
#2778=FACE_OUTER_BOUND ( 'NONE', #230, .T. ) ;
#2779=CARTESIAN_POINT ( 'NONE',  ( -92.69370383062498320, -209.9999999999999716, 81.22906250086715829 ) ) ;
#2793=CARTESIAN_POINT ( 'NONE',  ( 93.84685191531249870, -208.0026889286704943, 87.79072916753381151 ) ) ;
#2794=VERTEX_POINT ( 'NONE', #45392 ) ;
#2806=ORIENTED_EDGE ( 'NONE', *, *, #57155, .T. ) ;
#2809=ORIENTED_EDGE ( 'NONE', *, *, #26416, .T. ) ;
#2810=CARTESIAN_POINT ( 'NONE',  ( 93.84685191531248449, 88.00268892867053694, 79.74739583420048916 ) ) ;
#2813=ORIENTED_EDGE ( 'NONE', *, *, #40858, .F. ) ;
#2816=ORIENTED_EDGE ( 'NONE', *, *, #74295, .F. ) ;
#2818=ORIENTED_EDGE ( 'NONE', *, *, #7831, .F. ) ;
#2824=EDGE_CURVE ( 'NONE', #9802, #55839, #28443, .T. ) ;
#2827=CARTESIAN_POINT ( 'NONE',  ( -92.34999999999999432, -208.4700217866474645, 76.47979166840096354 ) ) ;
#2831=CARTESIAN_POINT ( 'NONE',  ( 94.99999999999998579, 93.05995642670504253, 76.58562500173430010 ) ) ;
#2832=CARTESIAN_POINT ( 'NONE',  ( -93.67500000000003979, 87.70503267997129626, 77.59104166840097605 ) ) ;
#2833=ORIENTED_EDGE ( 'NONE', *, *, #52136, .T. ) ;
#2834=CARTESIAN_POINT ( 'NONE',  ( 96.15314808468748708, 88.00268892867053694, 76.04322916753382344 ) ) ;
#2838=CARTESIAN_POINT ( 'NONE',  ( -96.32500000000001705, 92.29496732002878900, 78.54354166840096241 ) ) ;
#2840=EDGE_CURVE ( 'NONE', #58070, #55829, #4811, .T. ) ;
#2862=CARTESIAN_POINT ( 'NONE',  ( 97.64999999999999147, -210.0000000983658026, 80.23687499810812085 ) ) ;
#2863=CARTESIAN_POINT ( 'NONE',  ( -93.67499999999998295, -207.7050326799711968, 77.80270833506763495 ) ) ;
#2866=ADVANCED_FACE ( 'NONE', ( #16432 ), #65068, .F. ) ;
#2867=CARTESIAN_POINT ( 'NONE',  ( 92.69370383062498320, 90.00000000000002842, 85.35656250086715602 ) ) ;
#2869=CARTESIAN_POINT ( 'NONE',  ( -93.84685191531247028, -211.9973110713294489, 83.02822916753380866 ) ) ;
#2873=CARTESIAN_POINT ( 'NONE',  ( -96.32499999999996021, -212.2949673200287179, 76.77083333333332860 ) ) ;
#2875=CARTESIAN_POINT ( 'NONE',  ( 92.69370383062501162, -211.3315407142195852, 82.71072916753379900 ) ) ;
#2880=ORIENTED_EDGE ( 'NONE', *, *, #9602, .T. ) ;
#2887=CARTESIAN_POINT ( 'NONE',  ( 92.69370383062501162, -209.9999999999999716, 78.37156250086715659 ) ) ;
#2889=CARTESIAN_POINT ( 'NONE',  ( -96.32500000000001705, 92.29496732002878900, 76.63854166840096127 ) ) ;
#2890=EDGE_CURVE ( 'NONE', #61621, #67171, #39759, .T. ) ;
#2895=CARTESIAN_POINT ( 'NONE',  ( 97.64999999999999147, 89.99999999755287661, 75.15687493081163950 ) ) ;
#2896=CARTESIAN_POINT ( 'NONE',  ( 95.00000000000000000, -206.9400435732949575, 82.85625000000000284 ) ) ;
#2906=CARTESIAN_POINT ( 'NONE',  ( -92.69370383062502583, 88.66845928578038638, 82.44614583420049314 ) ) ;
#2910=CARTESIAN_POINT ( 'NONE',  ( 96.32499999999997442, 92.29496732002878900, 75.81833333333332803 ) ) ;
#2913=CARTESIAN_POINT ( 'NONE',  ( -97.64999999999994884, -211.5299782133524502, 86.32229166840097889 ) ) ;
#2916=ORIENTED_EDGE ( 'NONE', *, *, #5879, .T. ) ;
#2917=CARTESIAN_POINT ( 'NONE',  ( -93.67500000000003979, 87.70503267997129626, 85.21104166840096639 ) ) ;
#2919=CARTESIAN_POINT ( 'NONE',  ( 96.15314808468748708, 88.00268892867053694, 86.20322916753382003 ) ) ;
#2925=ORIENTED_EDGE ( 'NONE', *, *, #72549, .F. ) ;
#2928=VERTEX_POINT ( 'NONE', #61981 ) ;
#2935=( BOUNDED_CURVE ( )  B_SPLINE_CURVE ( 2, ( #23444, #41110, #34342, #46748, #18167, #12147, #919 ),
 .UNSPECIFIED., .F., .F. ) 
 B_SPLINE_CURVE_WITH_KNOTS ( ( 3, 2, 2, 3 ),
 ( 0.5833333333333329263, 0.5902777777777776791, 0.5972222222222223209, 0.6041666666666670737 ),
 .UNSPECIFIED. ) 
 CURVE ( )  GEOMETRIC_REPRESENTATION_ITEM ( )  RATIONAL_B_SPLINE_CURVE ( ( 1.000000000000008660, 0.8660254037844301589, 1.000000000000000000, 0.8660254037844387076, 1.000000000000000000, 0.8660254037844301589, 1.000000000000008660 ) ) 
 REPRESENTATION_ITEM ( '' )  );
#2936=CARTESIAN_POINT ( 'NONE',  ( -97.30629616937497417, -211.3315407142195852, 84.77447916753381207 ) ) ;
#2937=ORIENTED_EDGE ( 'NONE', *, *, #64890, .F. ) ;
#2938=DIRECTION ( 'NONE',  ( -0.000000000000000000, -0.000000000000000000, 1.000000000000000000 ) ) ;
#2940=ORIENTED_EDGE ( 'NONE', *, *, #44122, .T. ) ;
#2946=CARTESIAN_POINT ( 'NONE',  ( 93.84685191531248449, 91.99731107132950569, 76.83697916753381207 ) ) ;
#2950=CARTESIAN_POINT ( 'NONE',  ( 92.80789733908675032, 91.16770611573555527, 74.89296886168688161 ) ) ;
#2953=ADVANCED_FACE ( 'NONE', ( #68365 ), #22877, .F. ) ;
#2961=CARTESIAN_POINT ( 'NONE',  ( -93.84685191531252713, 88.00268892867056536, 82.86947916753379673 ) ) ;
#2971=CARTESIAN_POINT ( 'NONE',  ( 92.69370383062501162, -211.3315407142195852, 79.69447916753381378 ) ) ;
#2979=CARTESIAN_POINT ( 'NONE',  ( 96.15314808468748708, -208.0026889286704943, 75.61989583420049144 ) ) ;
#2991=CARTESIAN_POINT ( 'NONE',  ( 96.32499999999998863, -212.2949673200287179, 82.03604166840096923 ) ) ;
#2993=CARTESIAN_POINT ( 'NONE',  ( 94.99999999999998579, 93.05995642670504253, 86.03125000000000000 ) ) ;
#2997=CARTESIAN_POINT ( 'NONE',  ( -93.67499999999998295, -212.2949673200287179, 89.02104166840096866 ) ) ;
#3000=CARTESIAN_POINT ( 'NONE',  ( -93.84685191531254134, 91.99731107132950569, 89.58989583420049030 ) ) ;
#3002=CARTESIAN_POINT ( 'NONE',  ( 97.30629616937498838, 90.00000000000002842, 82.97531250086714749 ) ) ;
#3005=CARTESIAN_POINT ( 'NONE',  ( 92.34999999999999432, 91.52997821335252127, 81.13645833506764404 ) ) ;
#3013=ORIENTED_EDGE ( 'NONE', *, *, #7066, .F. ) ;
#3017=CARTESIAN_POINT ( 'NONE',  ( -95.00000000000002842, 86.94004357329504273, 85.71374999999997613 ) ) ;
#3020=AXIS2_PLACEMENT_3D ( 'NONE', #39598, #9160, #44501 ) ;
#3024=CARTESIAN_POINT ( 'NONE',  ( -92.69370383062498320, -209.9999999999999716, 78.53031250086714010 ) ) ;
#3033=ADVANCED_FACE ( 'NONE', ( #24341 ), #2187, .T. ) ;
#3035=CARTESIAN_POINT ( 'NONE',  ( 92.69370383062498320, 88.66845928578035796, 89.06072916753382174 ) ) ;
#3038=CARTESIAN_POINT ( 'NONE',  ( -92.34999999999999432, -208.4700217866474645, 86.63979166840096013 ) ) ;
#3039=CARTESIAN_POINT ( 'NONE',  ( -92.69370383062502583, 88.66845928578038638, 75.93739583420047268 ) ) ;
#3044=CARTESIAN_POINT ( 'NONE',  ( -93.67499999999998295, -212.2949673200287179, 84.57604166840096127 ) ) ;
#3048=CARTESIAN_POINT ( 'NONE',  ( 97.65000000000000568, 88.47002178664752137, 75.73895833506765030 ) ) ;
#3049=CARTESIAN_POINT ( 'NONE',  ( -93.67499999999998295, -212.2949673200287179, 88.94166666666666288 ) ) ;
#3062=FACE_OUTER_BOUND ( 'NONE', #13368, .T. ) ;
#3063=ORIENTED_EDGE ( 'NONE', *, *, #48240, .F. ) ;
#3064=CARTESIAN_POINT ( 'NONE',  ( 93.84685191531251292, -211.9973110713294489, 82.12864583420046927 ) ) ;
#3065=CARTESIAN_POINT ( 'NONE',  ( 92.69370383062501162, -208.6684592857803295, 89.11364583420049712 ) ) ;
#3067=VECTOR ( 'NONE', #17136, 1000.000000000000000 ) ;
#3068=CARTESIAN_POINT ( 'NONE',  ( 96.15314808468750130, -211.9973110713294489, 86.83822916753382515 ) ) ;
#3073=CARTESIAN_POINT ( 'NONE',  ( -97.30629616937501680, 90.00000000000004263, 77.10156250086714635 ) ) ;
#3074=EDGE_LOOP ( 'NONE', ( #36887, #53165, #62381, #13225 ) ) ;
#3079=VERTEX_POINT ( 'NONE', #23601 ) ;
#3086=CYLINDRICAL_SURFACE ( 'NONE', #33629, 2.649999999999985700 ) ;
#3091=CARTESIAN_POINT ( 'NONE',  ( 95.00000000000000000, -212.6630814284392557, 78.37156250086714238 ) ) ;
#3098=ORIENTED_EDGE ( 'NONE', *, *, #3316, .T. ) ;
#3102=CARTESIAN_POINT ( 'NONE',  ( -92.69370383062502583, 88.66845928578038638, 79.27114583420048177 ) ) ;
#3105=CARTESIAN_POINT ( 'NONE',  ( 96.15314808468748708, 91.99731107132950569, 78.63614583420047666 ) ) ;
#3112=CARTESIAN_POINT ( 'NONE',  ( -96.15314808468745866, -211.9973110713294489, 82.76364583420047438 ) ) ;
#3122=CARTESIAN_POINT ( 'NONE',  ( -96.32500000000001705, 92.29496732002878900, 75.92416666666666458 ) ) ;
#3123=CARTESIAN_POINT ( 'NONE',  ( -92.35000000000003695, 89.99999988321006583, 84.68187499741277691 ) ) ;
#3124=CARTESIAN_POINT ( 'NONE',  ( -97.30629616937501680, 88.66845928578038638, 84.61572916753380014 ) ) ;
#3135=CARTESIAN_POINT ( 'NONE',  ( 94.99999999999998579, 86.94004357329502852, 86.34874999999999545 ) ) ;
#3136=CARTESIAN_POINT ( 'NONE',  ( -92.69370383062498320, -211.3315407142195852, 82.44614583420049314 ) ) ;
#3139=( BOUNDED_CURVE ( )  B_SPLINE_CURVE ( 2, ( #61169, #31830, #50234, #73168, #26935, #3303, #72783 ),
 .UNSPECIFIED., .F., .F. ) 
 B_SPLINE_CURVE_WITH_KNOTS ( ( 3, 2, 2, 3 ),
 ( 0.5624999999999997780, 0.5694444444444440867, 0.5763888888888885065, 0.5833333333333329263 ),
 .UNSPECIFIED. ) 
 CURVE ( )  GEOMETRIC_REPRESENTATION_ITEM ( )  RATIONAL_B_SPLINE_CURVE ( ( 1.000000000000004219, 0.8660254037844343777, 1.000000000000000000, 0.8660254037844387076, 1.000000000000000000, 0.8660254037844472563, 0.9999999999999914513 ) ) 
 REPRESENTATION_ITEM ( '' )  );
#3148=DIRECTION ( 'NONE',  ( 1.000000000000000000, 0.000000000000000000, 0.000000000000000000 ) ) ;
#3155=( BOUNDED_CURVE ( )  B_SPLINE_CURVE ( 2, ( #18720, #47669, #41300, #2221, #24740, #58580, #64598, #11979, #36019 ),
 .UNSPECIFIED., .F., .F. ) 
 B_SPLINE_CURVE_WITH_KNOTS ( ( 3, 2, 2, 2, 3 ),
 ( 0.2540073681283129825, 0.2540075594717653429, 0.2610633250126476734, 0.2681190905535301150, 0.2751748541904411316 ),
 .UNSPECIFIED. ) 
 CURVE ( )  GEOMETRIC_REPRESENTATION_ITEM ( )  RATIONAL_B_SPLINE_CURVE ( ( 0.9999927337532901195, 0.9999963667781166521, 1.000000000000000000, 0.8660254037844387076, 1.000000000000000000, 0.8660254037844387076, 1.000000000000000000, 0.8660254037844387076, 1.000000000000000000 ) ) 
 REPRESENTATION_ITEM ( '' )  );
#3161=ORIENTED_EDGE ( 'NONE', *, *, #62752, .T. ) ;
#3162=AXIS2_PLACEMENT_3D ( 'NONE', #12087, #72814, #66832 ) ;
#3164=ORIENTED_EDGE ( 'NONE', *, *, #5446, .F. ) ;
#3166=ORIENTED_EDGE ( 'NONE', *, *, #69522, .F. ) ;
#3169=VERTEX_POINT ( 'NONE', #35609 ) ;
#3173=CARTESIAN_POINT ( 'NONE',  ( 94.99999999999998579, 92.66308142843935514, 75.67281250086716682 ) ) ;
#3178=ORIENTED_EDGE ( 'NONE', *, *, #39219, .F. ) ;
#3182=CARTESIAN_POINT ( 'NONE',  ( 95.00000000000000000, -212.6630814284392557, 87.89656250086713385 ) ) ;
#3187=DIRECTION ( 'NONE',  ( -0.000000000000000000, 0.000000000000000000, 1.000000000000000000 ) ) ;
#3190=CARTESIAN_POINT ( 'NONE',  ( -97.64999999999994884, -208.4700217866474645, 76.05645833506761733 ) ) ;
#3192=CARTESIAN_POINT ( 'NONE',  ( -95.00000000000002842, 92.66308142843932671, 89.00781250086716057 ) ) ;
#3195=CARTESIAN_POINT ( 'NONE',  ( 96.32499999999997442, 92.29496732002878900, 75.26270833506764291 ) ) ;
#3196=CARTESIAN_POINT ( 'NONE',  ( -96.15314808468752972, 91.99731107132950569, 88.90197916753380980 ) ) ;
#3197=B_SPLINE_CURVE_WITH_KNOTS ( 'NONE', 1,
 ( #32318, #48878 ),
 .UNSPECIFIED., .F., .F.,
 ( 2, 2 ),
 ( 0.000000000000000000, 1.000000000000000000 ),
 .UNSPECIFIED. ) ;
#3199=CARTESIAN_POINT ( 'NONE',  ( 96.15314808468748708, 91.99731107132950569, 74.98489583420048632 ) ) ;
#3201=DIRECTION ( 'NONE',  ( -1.000000000000000000, 0.000000000000000000, -0.000000000000000000 ) ) ;
#3206=CARTESIAN_POINT ( 'NONE',  ( -97.64999999999994884, -211.5299782133524218, 87.51291666666666913 ) ) ;
#3215=CARTESIAN_POINT ( 'NONE',  ( 92.35000000009272014, 90.00001381026685010, 80.55392363656929433 ) ) ;
#3216=CARTESIAN_POINT ( 'NONE',  ( -92.69370383062499741, -210.9303297190751891, 74.84209033237941355 ) ) ;
#3219=CARTESIAN_POINT ( 'NONE',  ( -95.00000000000002842, 92.66308142843932671, 82.49906250086714010 ) ) ;
#3222=CARTESIAN_POINT ( 'NONE',  ( -97.65000000000007674, 91.52997821335250705, 79.15208333333333712 ) ) ;
#3229=DIRECTION ( 'NONE',  ( -0.000000000000000000, -0.000000000000000000, 1.000000000000000000 ) ) ;
#3233=CARTESIAN_POINT ( 'NONE',  ( 97.30629616937498838, 88.66845928578035796, 84.98614583420047097 ) ) ;
#3234=CARTESIAN_POINT ( 'NONE',  ( -97.30629616937495996, -209.9999999999999716, 81.54656250086715374 ) ) ;
#3238=CARTESIAN_POINT ( 'NONE',  ( -92.34999999999999432, -211.5299782133524502, 78.83458333333334167 ) ) ;
#3242=CARTESIAN_POINT ( 'NONE',  ( 92.69370383062501162, -208.6684592857803011, 82.60489583420047666 ) ) ;
#3246=EDGE_LOOP ( 'NONE', ( #22765, #11489, #8962, #73622, #29290, #732 ) ) ;
#3251=CARTESIAN_POINT ( 'NONE',  ( -97.65000000000001990, 90.00001433786178495, 79.28437450583712121 ) ) ;
#3252=ORIENTED_EDGE ( 'NONE', *, *, #64700, .T. ) ;
#3253=CARTESIAN_POINT ( 'NONE',  ( 96.15314808468750130, -211.9973110713294489, 77.94822916753382458 ) ) ;
#3260=CARTESIAN_POINT ( 'NONE',  ( 93.67500000000001137, -207.7050326799711968, 81.63916666666666799 ) ) ;
#3262=ORIENTED_EDGE ( 'NONE', *, *, #15719, .T. ) ;
#3267=CARTESIAN_POINT ( 'NONE',  ( -93.84685191531254134, 91.99731107132950569, 83.87489583420048689 ) ) ;
#3268=AXIS2_PLACEMENT_3D ( 'NONE', #46731, #17775, #6153 ) ;
#3269=CARTESIAN_POINT ( 'NONE',  ( 97.64999999994533653, 89.99998298270493535, 88.49187441316099978 ) ) ;
#3272=( BOUNDED_CURVE ( )  B_SPLINE_CURVE ( 2, ( #8654, #66178, #71783, #55248, #21028, #66899, #38331 ),
 .UNSPECIFIED., .F., .F. ) 
 B_SPLINE_CURVE_WITH_KNOTS ( ( 3, 2, 2, 3 ),
 ( 0.9583333333333337034, 0.9652777777777781232, 0.9722222222222225430, 0.9791666666666669627 ),
 .UNSPECIFIED. ) 
 CURVE ( )  GEOMETRIC_REPRESENTATION_ITEM ( )  RATIONAL_B_SPLINE_CURVE ( ( 0.9999999999999935607, 0.8660254037844451469, 1.000000000000000000, 0.8660254037844387076, 1.000000000000000000, 0.8660254037844322683, 1.000000000000006439 ) ) 
 REPRESENTATION_ITEM ( '' )  );
#3273=CARTESIAN_POINT ( 'NONE',  ( 92.34999999999999432, 91.52997821335252127, 75.97708333333333997 ) ) ;
#3276=CARTESIAN_POINT ( 'NONE',  ( -97.64999999999994884, -211.5299782133524502, 87.59229166840096070 ) ) ;
#3278=VERTEX_POINT ( 'NONE', #48374 ) ;
#3281=EDGE_LOOP ( 'NONE', ( #56265, #48763, #11453, #36038 ) ) ;
#3282=CARTESIAN_POINT ( 'NONE',  ( -97.65000000000001990, 91.52997821335253548, 82.40645833506762585 ) ) ;
#3285=CARTESIAN_POINT ( 'NONE',  ( 97.30629616937498838, 90.00000000000002842, 88.21406250086714351 ) ) ;
#3288=CARTESIAN_POINT ( 'NONE',  ( -97.64995850092664398, 88.46999782714635785, 83.78229332575388355 ) ) ;
#3291=ORIENTED_EDGE ( 'NONE', *, *, #48064, .T. ) ;
#3292=CARTESIAN_POINT ( 'NONE',  ( 95.00000000000000000, -206.9400435732949575, 77.77624999999999034 ) ) ;
#3296=ORIENTED_EDGE ( 'NONE', *, *, #13435, .F. ) ;
#3301=CARTESIAN_POINT ( 'NONE',  ( -93.84685191531248449, -208.0026889286704943, 85.14489583420048291 ) ) ;
#3303=CARTESIAN_POINT ( 'NONE',  ( 92.35000000000012221, -211.5299782133525071, 81.16291666666667481 ) ) ;
#3306=CARTESIAN_POINT ( 'NONE',  ( 93.84685191531248449, 88.00268892867053694, 89.27239583420049485 ) ) ;
#3308=CARTESIAN_POINT ( 'NONE',  ( 94.99999999999998579, 87.33691857156068750, 76.46656250086712703 ) ) ;
#3316=EDGE_CURVE ( 'NONE', #56423, #51311, #48011, .T. ) ;
#3320=CARTESIAN_POINT ( 'NONE',  ( 92.34999999999999432, 90.00000000000002842, 89.36499999999999488 ) ) ;
#3322=CARTESIAN_POINT ( 'NONE',  ( -92.69370383062504004, 90.00000000000004263, 81.70531250086713726 ) ) ;
#3335=CARTESIAN_POINT ( 'NONE',  ( 96.15314808468750130, -211.9973110713294489, 79.85322916753381151 ) ) ;
#3345=VERTEX_POINT ( 'NONE', #42375 ) ;
#3346=CARTESIAN_POINT ( 'NONE',  ( 93.84685191531249870, -208.0026889286704943, 75.72572916753382799 ) ) ;
#3349=ORIENTED_EDGE ( 'NONE', *, *, #46529, .F. ) ;
#3356=CARTESIAN_POINT ( 'NONE',  ( 95.00000000000000000, -213.0599564267049857, 79.44312500173428759 ) ) ;
#3357=CARTESIAN_POINT ( 'NONE',  ( 94.99999999999998579, 86.94004357329500010, 85.07874999999999943 ) ) ;
#3364=( BOUNDED_CURVE ( )  B_SPLINE_CURVE ( 2, ( #47605, #11536, #51773, #53613, #37070, #42712, #26143 ),
 .UNSPECIFIED., .F., .F. ) 
 B_SPLINE_CURVE_WITH_KNOTS ( ( 3, 2, 2, 3 ),
 ( 0.5833333333333329263, 0.5902777777777776791, 0.5972222222222223209, 0.6041666666666670737 ),
 .UNSPECIFIED. ) 
 CURVE ( )  GEOMETRIC_REPRESENTATION_ITEM ( )  RATIONAL_B_SPLINE_CURVE ( ( 1.000000000000008660, 0.8660254037844301589, 1.000000000000000000, 0.8660254037844387076, 1.000000000000000000, 0.8660254037844301589, 1.000000000000008660 ) ) 
 REPRESENTATION_ITEM ( '' )  );
#3365=CARTESIAN_POINT ( 'NONE',  ( -92.69370383062504004, 90.00000000000004263, 88.84906250086716284 ) ) ;
#3366=CARTESIAN_POINT ( 'NONE',  ( 93.84685191531248449, 88.00268892867053694, 82.76364583420047438 ) ) ;
#3371=ORIENTED_EDGE ( 'NONE', *, *, #21136, .T. ) ;
#3372=ORIENTED_EDGE ( 'NONE', *, *, #26905, .F. ) ;
#3380=CARTESIAN_POINT ( 'NONE',  ( -96.15314808468747287, -208.0026889286704943, 78.74197916753381321 ) ) ;
#3382=DIRECTION ( 'NONE',  ( -0.000000000000000000, -0.000000000000000000, 1.000000000000000000 ) ) ;
#3384=CARTESIAN_POINT ( 'NONE',  ( 97.64999999999997726, 89.99997826787402744, 89.12687425009507081 ) ) ;
#3389=CARTESIAN_POINT ( 'NONE',  ( 94.99999999999998579, 92.66308142843932671, 86.94406250086714749 ) ) ;
#3394=CARTESIAN_POINT ( 'NONE',  ( 95.04693102382874770, -212.6495843973424940, 75.00000002508419072 ) ) ;
#3396=CARTESIAN_POINT ( 'NONE',  ( -92.35000000000000853, -210.0000001051137701, 86.58687499784845443 ) ) ;
#3400=DIRECTION ( 'NONE',  ( -0.000000000000000000, -0.000000000000000000, 1.000000000000000000 ) ) ;
#3401=CARTESIAN_POINT ( 'NONE',  ( 97.64999999999821512, 90.00000306648260562, 75.79187510780352000 ) ) ;
#3405=CARTESIAN_POINT ( 'NONE',  ( 97.30629616937498838, 90.00000000000002842, 89.48406250086715374 ) ) ;
#3407=EDGE_CURVE ( 'NONE', #14315, #53082, #7509, .T. ) ;
#3409=CARTESIAN_POINT ( 'NONE',  ( -94.99999999999997158, -213.0599564267049857, 88.88875000000000171 ) ) ;
#3410=EDGE_CURVE ( 'NONE', #58605, #30791, #29028, .T. ) ;
#3413=EDGE_LOOP ( 'NONE', ( #10470, #25244, #45684, #45485 ) ) ;
#3425=CARTESIAN_POINT ( 'NONE',  ( 97.30629616937498838, -208.6684592857803295, 82.39322916753381776 ) ) ;
#3426=CARTESIAN_POINT ( 'NONE',  ( 95.00000000000000000, -207.3369185715606307, 83.92781250086716227 ) ) ;
#3428=CARTESIAN_POINT ( 'NONE',  ( 92.69370383062501162, -211.3315407142195852, 85.40947916753380298 ) ) ;
#3433=EDGE_CURVE ( 'NONE', #52810, #22408, #54512, .T. ) ;
#3435=CARTESIAN_POINT ( 'NONE',  ( -97.30629616937501680, 91.33154071421968467, 78.31864583420050963 ) ) ;
#3444=CARTESIAN_POINT ( 'NONE',  ( -92.35000000010070664, 90.00002309722640348, 83.41187580057902551 ) ) ;
#3447=DIRECTION ( 'NONE',  ( -0.000000000000000000, -0.000000000000000000, 1.000000000000000000 ) ) ;
#3450=FACE_OUTER_BOUND ( 'NONE', #20245, .T. ) ;
#3454=CARTESIAN_POINT ( 'NONE',  ( 92.69370383062501162, -208.6684592857803011, 78.15989583420048348 ) ) ;
#3459=CARTESIAN_POINT ( 'NONE',  ( -94.99999999999997158, -213.0599564267049857, 84.44374999999999432 ) ) ;
#3461=CARTESIAN_POINT ( 'NONE',  ( -93.84685191531254134, 91.99731107132950569, 78.15989583420049769 ) ) ;
#3463=CARTESIAN_POINT ( 'NONE',  ( 94.99999999999998579, 87.33691857156068750, 76.46656250086712703 ) ) ;
#3466=CARTESIAN_POINT ( 'NONE',  ( -96.15314808468747287, -208.0026889286704943, 89.53697916753381492 ) ) ;
#3467=AXIS2_PLACEMENT_3D ( 'NONE', #13316, #1711, #24598 ) ;
#3470=DIRECTION ( 'NONE',  ( -0.000000000000000000, -0.000000000000000000, 1.000000000000000000 ) ) ;
#3471=CARTESIAN_POINT ( 'NONE',  ( -94.99999999999997158, -207.3369185715606307, 79.32406250086714294 ) ) ;
#3482=CARTESIAN_POINT ( 'NONE',  ( -92.69370383062504004, 90.00000000000004263, 85.51531250086713953 ) ) ;
#3490=CARTESIAN_POINT ( 'NONE',  ( -97.64999999999996305, -209.9999999999999716, 90.00000000000000000 ) ) ;
#3496=CARTESIAN_POINT ( 'NONE',  ( -93.84685191531248449, -208.0026889286704943, 82.60489583420049087 ) ) ;
#3502=EDGE_CURVE ( 'NONE', #31031, #23968, #72707, .T. ) ;
#3505=FACE_OUTER_BOUND ( 'NONE', #33164, .T. ) ;
#3506=ORIENTED_EDGE ( 'NONE', *, *, #243, .F. ) ;
#3510=DIRECTION ( 'NONE',  ( -0.000000000000000000, -0.000000000000000000, 1.000000000000000000 ) ) ;
#3511=ADVANCED_FACE ( 'NONE', ( #73892 ), #39706, .F. ) ;
#3515=CARTESIAN_POINT ( 'NONE',  ( -93.67500000000003979, 92.29496732002878900, 75.89770833506763381 ) ) ;
#3532=ORIENTED_EDGE ( 'NONE', *, *, #62824, .T. ) ;
#3538=CARTESIAN_POINT ( 'NONE',  ( 92.69370383062498320, 91.33154071421968467, 77.04864583420048518 ) ) ;
#3545=CARTESIAN_POINT ( 'NONE',  ( 97.30629616937498838, 91.33154071421968467, 87.47322916753381605 ) ) ;
#3547=CARTESIAN_POINT ( 'NONE',  ( 95.00000000000000000, -212.6630814284392557, 89.16656250086712987 ) ) ;
#3553=CARTESIAN_POINT ( 'NONE',  ( 94.99999999999998579, 93.05995642670504253, 77.85562500173431033 ) ) ;
#3554=CARTESIAN_POINT ( 'NONE',  ( -92.34999999999999432, -208.4700217866474645, 84.09979166840098230 ) ) ;
#3555=FACE_OUTER_BOUND ( 'NONE', #56420, .T. ) ;
#3558=CARTESIAN_POINT ( 'NONE',  ( -96.32499999999996021, -212.2949673200287179, 76.85020833506763438 ) ) ;
#3559=CARTESIAN_POINT ( 'NONE',  ( -92.69370383062502583, 91.33154071421968467, 88.26697916753381890 ) ) ;
#3561=CARTESIAN_POINT ( 'NONE',  ( 93.84685191531248449, 91.99731107132950569, 88.26697916753380468 ) ) ;
#3562=CARTESIAN_POINT ( 'NONE',  ( -93.84685191531252713, 88.00268892867056536, 87.94947916753380923 ) ) ;
#3566=CYLINDRICAL_SURFACE ( 'NONE', #43922, 2.649999999999985700 ) ;
#3567=FACE_OUTER_BOUND ( 'NONE', #46877, .T. ) ;
#3572=ORIENTED_EDGE ( 'NONE', *, *, #2231, .F. ) ;
#3573=ORIENTED_EDGE ( 'NONE', *, *, #24608, .F. ) ;
#3574=CARTESIAN_POINT ( 'NONE',  ( -96.32500000000001705, 92.29496732002878900, 82.90916666666666401 ) ) ;
#3581=( BOUNDED_CURVE ( )  B_SPLINE_CURVE ( 2, ( #8612, #61597, #2997, #25889, #72845, #21344, #20627 ),
 .UNSPECIFIED., .F., .F. ) 
 B_SPLINE_CURVE_WITH_KNOTS ( ( 3, 2, 2, 3 ),
 ( 0.02116741234835334273, 0.02822306216366812434, 0.03527882770458510425, 0.04233441017615420521 ),
 .UNSPECIFIED. ) 
 CURVE ( )  GEOMETRIC_REPRESENTATION_ITEM ( )  RATIONAL_B_SPLINE_CURVE ( ( 0.9999956052857933431, 0.8660276011775827065, 1.000000000000000000, 0.8660254037844387076, 1.000000000000000000, 0.8660288798979544067, 0.9999930479533516436 ) ) 
 REPRESENTATION_ITEM ( '' )  );
#3586=CARTESIAN_POINT ( 'NONE',  ( -92.69370383062502583, 91.33154071421968467, 83.02822916753379445 ) ) ;
#3587=EDGE_CURVE ( 'NONE', #51903, #72660, #70099, .T. ) ;
#3589=CARTESIAN_POINT ( 'NONE',  ( 92.34999999999999432, 90.00000000000002842, 82.45937500173430124 ) ) ;
#3599=EDGE_CURVE ( 'NONE', #30760, #39726, #45765, .T. ) ;
#3600=( BOUNDED_CURVE ( )  B_SPLINE_CURVE ( 2, ( #32303, #38333, #61271, #9760, #61641, #27034, #3401 ),
 .UNSPECIFIED., .F., .F. ) 
 B_SPLINE_CURVE_WITH_KNOTS ( ( 3, 2, 2, 3 ),
 ( 0.8890265259358468564, 0.8960822236920598094, 0.9031379892329426395, 0.9101937466091534201 ),
 .UNSPECIFIED. ) 
 CURVE ( )  GEOMETRIC_REPRESENTATION_ITEM ( )  RATIONAL_B_SPLINE_CURVE ( ( 0.9999974258394828119, 0.8660266908770624106, 1.000000000000000000, 0.8660254037844387076, 1.000000000000000000, 0.8660254037844387076, 1.000000000000000000 ) ) 
 REPRESENTATION_ITEM ( '' )  );
#3601=EDGE_CURVE ( 'NONE', #22350, #20056, #59793, .T. ) ;
#3602=CARTESIAN_POINT ( 'NONE',  ( 92.69370383062498320, 90.00000000000002842, 80.91156250086716284 ) ) ;
#3603=CARTESIAN_POINT ( 'NONE',  ( -92.69370383062498320, -211.3315407142195852, 82.44614583420049314 ) ) ;
#3604=CARTESIAN_POINT ( 'NONE',  ( 97.64999999999999147, 90.00000000000002842, 90.00000000000000000 ) ) ;
#3608=CARTESIAN_POINT ( 'NONE',  ( -97.64999999999994884, -211.5299782133524502, 77.35291666666665833 ) ) ;
#3612=CARTESIAN_POINT ( 'NONE',  ( 92.69370383062501162, -208.6684592857803011, 83.87489583420047268 ) ) ;
#3613=ADVANCED_FACE ( 'NONE', ( #69014 ), #6599, .T. ) ;
#3617=VERTEX_POINT ( 'NONE', #6240 ) ;
#3621=CARTESIAN_POINT ( 'NONE',  ( 92.69370383062501162, -211.3315407142195852, 77.15447916753382174 ) ) ;
#3623=DIRECTION ( 'NONE',  ( 1.000000000000000000, 0.000000000000000000, 0.000000000000000000 ) ) ;
#3624=CARTESIAN_POINT ( 'NONE',  ( -95.79297114439312111, 87.49569407151190603, 74.98272308147875265 ) ) ;
#3625=CARTESIAN_POINT ( 'NONE',  ( 92.69370383062498320, 88.66845928578037217, 87.94947916753382344 ) ) ;
#3627=CARTESIAN_POINT ( 'NONE',  ( 92.35000000000002274, -208.4700217866474645, 82.96208333333333940 ) ) ;
#3635=CARTESIAN_POINT ( 'NONE',  ( -93.84685191531252713, 88.00268892867056536, 84.29822916753381890 ) ) ;
#3636=FACE_OUTER_BOUND ( 'NONE', #71266, .T. ) ;
#3639=CARTESIAN_POINT ( 'NONE',  ( 92.34999999999999432, 91.52997821335252127, 76.61208333333333087 ) ) ;
#3642=CARTESIAN_POINT ( 'NONE',  ( -93.67499999999998295, -207.7050326799711968, 86.05770833506763040 ) ) ;
#3643=ORIENTED_EDGE ( 'NONE', *, *, #24107, .F. ) ;
#3645=ORIENTED_EDGE ( 'NONE', *, *, #8579, .F. ) ;
#3646=CARTESIAN_POINT ( 'NONE',  ( -96.32500000000001705, 92.29496732002878900, 81.71854166840095957 ) ) ;
#3648=CARTESIAN_POINT ( 'NONE',  ( 94.99999999999998579, 87.33691857156068750, 88.05531250086716000 ) ) ;
#3652=CARTESIAN_POINT ( 'NONE',  ( -93.67500000000003979, 87.70503267997129626, 83.94104166840097037 ) ) ;
#3655=CARTESIAN_POINT ( 'NONE',  ( -94.99999999999997158, -209.9999999999999716, 90.00000000000000000 ) ) ;
#3657=CARTESIAN_POINT ( 'NONE',  ( -93.67500000000003979, 92.29496732002878900, 80.97770833506763211 ) ) ;
#3660=VECTOR ( 'NONE', #51991, 1000.000000000000000 ) ;
#3670=CARTESIAN_POINT ( 'NONE',  ( -92.35000000000003695, 89.99999999755290503, 75.15687493081163950 ) ) ;
#3671=CARTESIAN_POINT ( 'NONE',  ( -97.30629616937495996, -209.9999999999999716, 84.08656250086716000 ) ) ;
#3679=CARTESIAN_POINT ( 'NONE',  ( 97.30629616937498838, 91.33154071421968467, 77.31322916753380525 ) ) ;
#3683=CARTESIAN_POINT ( 'NONE',  ( 94.99999999999998579, 90.00000000000002842, 90.00000000000000000 ) ) ;
#3690=CARTESIAN_POINT ( 'NONE',  ( -92.69370383062505425, 91.33154071421968467, 83.02822916753379445 ) ) ;
#3695=EDGE_CURVE ( 'NONE', #35038, #69246, #13220, .T. ) ;
#3704=FACE_OUTER_BOUND ( 'NONE', #37853, .T. ) ;
#3705=CARTESIAN_POINT ( 'NONE',  ( 96.15314808468748708, -208.0026889286704943, 77.52489583420047836 ) ) ;
#3709=( BOUNDED_CURVE ( )  B_SPLINE_CURVE ( 2, ( #41441, #19244, #12856, #52347, #895, #42196, #41086 ),
 .UNSPECIFIED., .F., .F. ) 
 B_SPLINE_CURVE_WITH_KNOTS ( ( 3, 2, 2, 3 ),
 ( 0.8749999999999997780, 0.8819444444444441977, 0.8888888888888886175, 0.8958333333333331483 ),
 .UNSPECIFIED. ) 
 CURVE ( )  GEOMETRIC_REPRESENTATION_ITEM ( )  RATIONAL_B_SPLINE_CURVE ( ( 1.000000000000004219, 0.8660254037844343777, 1.000000000000000000, 0.8660254037844387076, 1.000000000000000000, 0.8660254037844430375, 0.9999999999999956701 ) ) 
 REPRESENTATION_ITEM ( '' )  );
#3715=CARTESIAN_POINT ( 'NONE',  ( 96.15314808468750130, -211.9973110713294489, 75.40822916753381833 ) ) ;
#3716=ORIENTED_EDGE ( 'NONE', *, *, #32088, .F. ) ;
#3717=CARTESIAN_POINT ( 'NONE',  ( -92.34999999999999432, -209.9999999999999716, 87.77749999999998920 ) ) ;
#3722=EDGE_LOOP ( 'NONE', ( #73607, #73304, #12847, #40772 ) ) ;
#3724=CARTESIAN_POINT ( 'NONE',  ( 97.64999999999997726, -211.5299782133524502, 80.81895833506764859 ) ) ;
#3725=CARTESIAN_POINT ( 'NONE',  ( 92.34999999999999432, 90.00000000000002842, 86.82500000000000284 ) ) ;
#3730=CARTESIAN_POINT ( 'NONE',  ( -97.30629616937501680, 88.66845928578038638, 84.13947916753383538 ) ) ;
#3731=CARTESIAN_POINT ( 'NONE',  ( 93.84685191531248449, 91.99731107132950569, 83.18697916753382060 ) ) ;
#3732=ORIENTED_EDGE ( 'NONE', *, *, #10251, .T. ) ;
#3733=EDGE_CURVE ( 'NONE', #71136, #42455, #6009, .T. ) ;
#3737=VERTEX_POINT ( 'NONE', #60694 ) ;
#3739=AXIS2_PLACEMENT_3D ( 'NONE', #53575, #25001, #63769 ) ;
#3747=CARTESIAN_POINT ( 'NONE',  ( 96.32499999999997442, 92.29496732002878900, 88.59770833506763665 ) ) ;
#3750=CARTESIAN_POINT ( 'NONE',  ( -93.84685191531247028, -211.9973110713294489, 78.42447916753381776 ) ) ;
#3757=ADVANCED_FACE ( 'NONE', ( #25365 ), #8809, .F. ) ;
#3761=CARTESIAN_POINT ( 'NONE',  ( -96.32500000000001705, 87.70503267997129626, 89.47083333333333144 ) ) ;
#3762=CARTESIAN_POINT ( 'NONE',  ( 97.30629616937498838, 88.66845928578035796, 87.36739583420047950 ) ) ;
#3766=CARTESIAN_POINT ( 'NONE',  ( -93.67500000000003979, 87.70503267997129626, 87.03666666666666174 ) ) ;
#3769=CARTESIAN_POINT ( 'NONE',  ( -97.64999999998390479, 89.99999393654049129, 88.17456390440148084 ) ) ;
#3777=CARTESIAN_POINT ( 'NONE',  ( -92.34999999999999432, -209.9999999999999716, 89.04749999999999943 ) ) ;
#3788=VECTOR ( 'NONE', #44721, 1000.000000000000000 ) ;
#3795=( BOUNDED_CURVE ( )  B_SPLINE_CURVE ( 2, ( #4462, #21725, #44681, #39028, #46899, #63823, #70167, #1443, #17572 ),
 .UNSPECIFIED., .F., .F. ) 
 B_SPLINE_CURVE_WITH_KNOTS ( ( 3, 2, 2, 2, 3 ),
 ( 0.7196881748034549275, 0.7267438507108832102, 0.7337996162517648191, 0.7408553817926463170, 0.7408554641864679713 ),
 .UNSPECIFIED. ) 
 CURVE ( )  GEOMETRIC_REPRESENTATION_ITEM ( )  RATIONAL_B_SPLINE_CURVE ( ( 0.9999965961303334261, 0.8660271057408929218, 1.000000000000000000, 0.8660254037844387076, 1.000000000000000000, 0.8660254037844387076, 1.000000000000000000, 0.9999984355093834987, 0.9999968710553057694 ) ) 
 REPRESENTATION_ITEM ( '' )  );
#3796=CARTESIAN_POINT ( 'NONE',  ( 92.69370383062501162, -211.3315407142195852, 81.44072916753380298 ) ) ;
#3797=CARTESIAN_POINT ( 'NONE',  ( 95.00000000000000000, -212.6630814284392557, 83.61031250086715261 ) ) ;
#3799=CARTESIAN_POINT ( 'NONE',  ( 97.30629616937498838, -211.3315407142195852, 84.98614583420047097 ) ) ;
#3804=CARTESIAN_POINT ( 'NONE',  ( -93.84685191531254134, 91.99731107132950569, 76.88989583420048746 ) ) ;
#3805=VECTOR ( 'NONE', #34128, 1000.000000000000000 ) ;
#3807=ORIENTED_EDGE ( 'NONE', *, *, #11540, .T. ) ;
#3813=ORIENTED_EDGE ( 'NONE', *, *, #56366, .T. ) ;
#3817=EDGE_LOOP ( 'NONE', ( #39411, #48534, #33782, #25634 ) ) ;
#3821=CARTESIAN_POINT ( 'NONE',  ( 92.69370383062501162, -208.6684592857803011, 74.98489583420048632 ) ) ;
#3822=FACE_OUTER_BOUND ( 'NONE', #9408, .T. ) ;
#3823=ORIENTED_EDGE ( 'NONE', *, *, #1137, .F. ) ;
#3830=CARTESIAN_POINT ( 'NONE',  ( -96.15314808468752972, 91.99731107132950569, 76.36072916753381890 ) ) ;
#3832=CARTESIAN_POINT ( 'NONE',  ( 97.30629616937498838, 90.00000000000002842, 75.99031250086714806 ) ) ;
#3839=CARTESIAN_POINT ( 'NONE',  ( -96.15314808468745866, -211.9973110713294489, 80.22364583420046813 ) ) ;
#3842=CARTESIAN_POINT ( 'NONE',  ( 97.64999999999999147, -209.9999999999999716, 90.00000000000000000 ) ) ;
#3849=DIRECTION ( 'NONE',  ( 0.000000000000000000, -1.000000000000000000, 0.000000000000000000 ) ) ;
#3851=CARTESIAN_POINT ( 'NONE',  ( -96.15314808468751551, 88.00268892867056536, 82.76364583420047438 ) ) ;
#3863=CARTESIAN_POINT ( 'NONE',  ( -92.34999999999999432, -209.9999999999999716, 90.00000000000000000 ) ) ;
#3866=CARTESIAN_POINT ( 'NONE',  ( -92.35003071824209542, -208.4700040514621264, 79.01979289519869099 ) ) ;
#3867=CARTESIAN_POINT ( 'NONE',  ( -94.99999999999997158, -207.3369185715606307, 83.29281250086717137 ) ) ;
#3871=ORIENTED_EDGE ( 'NONE', *, *, #25873, .T. ) ;
#3884=CARTESIAN_POINT ( 'NONE',  ( -92.35000000000012221, 90.00000071509187194, 85.31687502647973531 ) ) ;
#3890=ORIENTED_EDGE ( 'NONE', *, *, #10454, .F. ) ;
#3894=ORIENTED_EDGE ( 'NONE', *, *, #59094, .F. ) ;
#3896=ORIENTED_EDGE ( 'NONE', *, *, #65370, .F. ) ;
#3902=CARTESIAN_POINT ( 'NONE',  ( 92.69370383062498320, 91.33154071421968467, 76.41364583420049428 ) ) ;
#3903=CARTESIAN_POINT ( 'NONE',  ( 96.32499999999998863, -212.2949673200287179, 89.02104166840096866 ) ) ;
#3909=CARTESIAN_POINT ( 'NONE',  ( 92.69370383062498320, 90.00000000000002842, 89.64281250086713726 ) ) ;
#3912=CARTESIAN_POINT ( 'NONE',  ( 93.84685191531251292, -211.9973110713294489, 85.30364583420046642 ) ) ;
#3917=CYLINDRICAL_SURFACE ( 'NONE', #6593, 2.649999999999985700 ) ;
#3918=DIRECTION ( 'NONE',  ( -0.000000000000000000, -0.000000000000000000, 1.000000000000000000 ) ) ;
#3923=ADVANCED_FACE ( 'NONE', ( #5415 ), #50876, .F. ) ;
#3924=CARTESIAN_POINT ( 'NONE',  ( -93.67499999999998295, -212.2949673200287179, 76.32104166840096582 ) ) ;
#3928=CARTESIAN_POINT ( 'NONE',  ( 96.15314808468748708, 91.99731107132950569, 88.79614583420047325 ) ) ;
#3929=CARTESIAN_POINT ( 'NONE',  ( -95.00000000000002842, 92.66308142843932671, 87.57906250086713840 ) ) ;
#3942=EDGE_CURVE ( 'NONE', #37865, #23298, #67465, .T. ) ;
#3943=CARTESIAN_POINT ( 'NONE',  ( -93.67500000000003979, 92.29496732002878900, 82.80333333333332746 ) ) ;
#3951=CARTESIAN_POINT ( 'NONE',  ( -96.15314808468752972, 91.99731107132950569, 80.64697916753381435 ) ) ;
#3958=DIRECTION ( 'NONE',  ( -0.000000000000000000, -0.000000000000000000, 1.000000000000000000 ) ) ;
#3964=CARTESIAN_POINT ( 'NONE',  ( 92.69370383062498320, 90.00000000000002842, 80.27656250086714351 ) ) ;
#3965=CARTESIAN_POINT ( 'NONE',  ( -93.84685191531247028, -211.9973110713294489, 82.39322916753381776 ) ) ;
#3967=ORIENTED_EDGE ( 'NONE', *, *, #55706, .T. ) ;
#3968=CARTESIAN_POINT ( 'NONE',  ( 97.64999999999999147, -210.0000000207152198, 80.87187500099602744 ) ) ;
#3969=CARTESIAN_POINT ( 'NONE',  ( -97.64999999999994884, -208.4700217866474645, 78.51708333333334622 ) ) ;
#3973=CARTESIAN_POINT ( 'NONE',  ( -97.30629616937501680, 88.66845928578038638, 77.78947916753381264 ) ) ;
#3974=CARTESIAN_POINT ( 'NONE',  ( 97.30629616937498838, -209.9999999999999716, 83.61031250086713840 ) ) ;
#3980=CARTESIAN_POINT ( 'NONE',  ( -92.35000000000010800, -208.4700217866473793, 83.38541666666667140 ) ) ;
#3984=CARTESIAN_POINT ( 'NONE',  ( 95.00000000000000000, -209.9999999999999716, 90.00000000000000000 ) ) ;
#3987=CARTESIAN_POINT ( 'NONE',  ( 96.15314808468748708, 91.99731107132950569, 88.31989583420048007 ) ) ;
#3988=CARTESIAN_POINT ( 'NONE',  ( -96.32500000000001705, 87.70503267997129626, 83.20020833506764291 ) ) ;
#3989=CARTESIAN_POINT ( 'NONE',  ( 96.32499999999998863, -212.2949673200287179, 82.59166666666665435 ) ) ;
#3996=ORIENTED_EDGE ( 'NONE', *, *, #50257, .T. ) ;
#4003=CARTESIAN_POINT ( 'NONE',  ( 97.64999322989702080, -211.5299821220732213, 82.72395806468929891 ) ) ;
#4008=CARTESIAN_POINT ( 'NONE',  ( -97.64999999999994884, -211.5299782133524502, 85.68729166840097378 ) ) ;
#4009=VERTEX_POINT ( 'NONE', #6150 ) ;
#4012=CARTESIAN_POINT ( 'NONE',  ( -97.65000000000001990, 91.52997821335253548, 84.31145833506762699 ) ) ;
#4014=( BOUNDED_CURVE ( )  B_SPLINE_CURVE ( 2, ( #14802, #64844, #65958, #36624, #54301, #70448, #71570 ),
 .UNSPECIFIED., .F., .F. ) 
 B_SPLINE_CURVE_WITH_KNOTS ( ( 3, 2, 2, 3 ),
 ( 0.7708333333333328152, 0.7777777777777775681, 0.7847222222222222099, 0.7916666666666669627 ),
 .UNSPECIFIED. ) 
 CURVE ( )  GEOMETRIC_REPRESENTATION_ITEM ( )  RATIONAL_B_SPLINE_CURVE ( ( 1.000000000000010658, 0.8660254037844280495, 1.000000000000000000, 0.8660254037844387076, 1.000000000000000000, 0.8660254037844322683, 1.000000000000006439 ) ) 
 REPRESENTATION_ITEM ( '' )  );
#4015=EDGE_CURVE ( 'NONE', #55000, #14315, #42727, .T. ) ;
#4017=CARTESIAN_POINT ( 'NONE',  ( 92.69370383062498320, 91.33154071421968467, 84.66864583420047552 ) ) ;
#4020=CARTESIAN_POINT ( 'NONE',  ( -97.64999999999996305, -209.9999999999999716, 75.39499999999999602 ) ) ;
#4022=LINE ( 'NONE', #20916, #29433 ) ;
#4026=CARTESIAN_POINT ( 'NONE',  ( -97.64999999947052345, 90.00003365185393989, 81.18829462297244959 ) ) ;
#4028=CONICAL_SURFACE ( 'NONE', #24450, 2.649999999999999467, 1.029744258676654312 ) ;
#4037=CARTESIAN_POINT ( 'NONE',  ( -97.30629616937495996, -209.9999999999999716, 84.72156250086715090 ) ) ;
#4046=CARTESIAN_POINT ( 'NONE',  ( 92.69370383062498320, 88.66845928578035796, 79.53572916753380184 ) ) ;
#4057=CARTESIAN_POINT ( 'NONE',  ( -95.00000000000002842, 87.33691857156074434, 84.72156250086713669 ) ) ;
#4069=VECTOR ( 'NONE', #43982, 1000.000000000000000 ) ;
#4070=CARTESIAN_POINT ( 'NONE',  ( 92.69370383062501162, -211.3315407142195852, 77.15447916753382174 ) ) ;
#4073=ORIENTED_EDGE ( 'NONE', *, *, #21116, .T. ) ;
#4074=EDGE_CURVE ( 'NONE', #428, #4451, #59340, .T. ) ;
#4075=CARTESIAN_POINT ( 'NONE',  ( 97.25633982090076302, -209.4495095149827364, 74.79348190356850523 ) ) ;
#4077=EDGE_CURVE ( 'NONE', #61415, #47972, #12865, .T. ) ;
#4081=CARTESIAN_POINT ( 'NONE',  ( 95.00000000000000000, -207.3369185715606307, 77.57781250086715374 ) ) ;
#4086=ORIENTED_EDGE ( 'NONE', *, *, #48411, .T. ) ;
#4093=CARTESIAN_POINT ( 'NONE',  ( 96.32499999999998863, -212.2949673200287179, 79.49604166840096298 ) ) ;
#4094=CARTESIAN_POINT ( 'NONE',  ( 94.99999999999998579, 93.05995642670504253, 80.31624999999998238 ) ) ;
#4102=CARTESIAN_POINT ( 'NONE',  ( -97.30629616937501680, 90.00000000000004263, 83.45156250086715488 ) ) ;
#4104=CARTESIAN_POINT ( 'NONE',  ( 93.84685191531248449, 88.00268892867053694, 79.58864583420047722 ) ) ;
#4106=CARTESIAN_POINT ( 'NONE',  ( -94.99999999999997158, -213.0599564267049857, 78.80812500173429669 ) ) ;
#4110=CARTESIAN_POINT ( 'NONE',  ( -94.99999999999997158, -207.3369185715606307, 79.32406250086714294 ) ) ;
#4122=CARTESIAN_POINT ( 'NONE',  ( -92.69370383062498320, -209.9999999999999716, 79.16531250086714522 ) ) ;
#4133=CARTESIAN_POINT ( 'NONE',  ( 93.67500000000001137, -207.7050326799711968, 82.35354166840096468 ) ) ;
#4134=CARTESIAN_POINT ( 'NONE',  ( 96.15314808468748708, 88.00268892867053694, 89.21947916753380525 ) ) ;
#4139=CARTESIAN_POINT ( 'NONE',  ( -96.32500000000001705, 87.70503267997129626, 87.64520833506762187 ) ) ;
#4142=DIRECTION ( 'NONE',  ( 1.000000000000000000, 0.000000000000000000, 0.000000000000000000 ) ) ;
#4146=CARTESIAN_POINT ( 'NONE',  ( -97.64999999999996305, -209.9999999999999716, 83.01499999999998636 ) ) ;
#4154=CARTESIAN_POINT ( 'NONE',  ( 92.69370383062501162, -211.3315407142195852, 87.94947916753382344 ) ) ;
#4162=CARTESIAN_POINT ( 'NONE',  ( 93.84685191531251292, -211.9973110713294489, 77.68364583420047609 ) ) ;
#4163=CARTESIAN_POINT ( 'NONE',  ( 92.69370383062501162, -211.3315407142195852, 83.50447916753383026 ) ) ;
#4166=VECTOR ( 'NONE', #8705, 1000.000000000000000 ) ;
#4167=CARTESIAN_POINT ( 'NONE',  ( 96.15314808468748708, -208.0026889286704943, 87.68489583420048916 ) ) ;
#4168=EDGE_CURVE ( 'NONE', #19312, #6682, #16079, .T. ) ;
#4180=CARTESIAN_POINT ( 'NONE',  ( 96.32499999999998863, -207.7050326799711968, 89.23270833506762756 ) ) ;
#4191=CARTESIAN_POINT ( 'NONE',  ( 95.00000000000000000, -207.3369185715606307, 74.87906250086713555 ) ) ;
#4196=CARTESIAN_POINT ( 'NONE',  ( -92.34999999999996589, -211.5299782133524502, 84.54958333333334508 ) ) ;
#4197=CARTESIAN_POINT ( 'NONE',  ( -92.34999999999990905, -208.4700217866474929, 88.46541666666664128 ) ) ;
#4198=CARTESIAN_POINT ( 'NONE',  ( -96.15314808468751551, 88.00268892867056536, 75.93739583420048689 ) ) ;
#4199=EDGE_CURVE ( 'NONE', #32740, #72643, #756, .T. ) ;
#4201=EDGE_LOOP ( 'NONE', ( #10088, #15057 ) ) ;
#4202=CARTESIAN_POINT ( 'NONE',  ( 92.69370383062498320, 88.66845928578037217, 77.63072916753380071 ) ) ;
#4205=CARTESIAN_POINT ( 'NONE',  ( -93.84685191531248449, -208.0026889286704943, 88.79614583420047325 ) ) ;
#4211=CARTESIAN_POINT ( 'NONE',  ( -93.84685191531248449, -208.0026889286704943, 78.63614583420047666 ) ) ;
#4214=CARTESIAN_POINT ( 'NONE',  ( -97.64999999999996305, -209.9999999999999716, 84.28499999999999659 ) ) ;
#4215=EDGE_LOOP ( 'NONE', ( #56432, #33445, #45255, #50926 ) ) ;
#4220=DIRECTION ( 'NONE',  ( -0.000000000000000000, -0.000000000000000000, 1.000000000000000000 ) ) ;
#4221=CARTESIAN_POINT ( 'NONE',  ( -95.00000000000002842, 92.66308142843932671, 82.49906250086714010 ) ) ;
#4227=CARTESIAN_POINT ( 'NONE',  ( 97.64999999999602665, -210.0000045800691737, 76.42687486206342840 ) ) ;
#4232=CARTESIAN_POINT ( 'NONE',  ( 93.67500000000001137, -207.7050326799711968, 88.70354166840097321 ) ) ;
#4233=CARTESIAN_POINT ( 'NONE',  ( -93.84685191531248449, -208.0026889286704943, 79.42989583420049371 ) ) ;
#4235=CARTESIAN_POINT ( 'NONE',  ( -92.34999999999999432, -209.9999999999999716, 87.22187500173430408 ) ) ;
#4237=( BOUNDED_CURVE ( )  B_SPLINE_CURVE ( 2, ( #23300, #40581, #34562, #46226, #39102, #63529, #62427 ),
 .UNSPECIFIED., .F., .F. ) 
 B_SPLINE_CURVE_WITH_KNOTS ( ( 3, 2, 2, 3 ),
 ( 0.6350190250602294473, 0.6420746642234487211, 0.6491304297643658572, 0.6561861948943049638 ),
 .UNSPECIFIED. ) 
 CURVE ( )  GEOMETRIC_REPRESENTATION_ITEM ( )  RATIONAL_B_SPLINE_CURVE ( ( 0.9999952007765371409, 0.8660278034391509783, 1.000000000000000000, 0.8660254037844387076, 1.000000000000000000, 0.8660254037844387076, 1.000000000000000000 ) ) 
 REPRESENTATION_ITEM ( '' )  );
#4241=EDGE_CURVE ( 'NONE', #66971, #59392, #8403, .T. ) ;
#4247=EDGE_CURVE ( 'NONE', #42384, #68050, #23768, .T. ) ;
#4254=CARTESIAN_POINT ( 'NONE',  ( -92.35000000000003695, 90.00000000000004263, 80.15749999999999886 ) ) ;
#4256=VERTEX_POINT ( 'NONE', #62466 ) ;
#4262=CARTESIAN_POINT ( 'NONE',  ( 26.50000000000000355, -120.0000000000000000, -64.00000000000000000 ) ) ;
#4263=ORIENTED_EDGE ( 'NONE', *, *, #22560, .F. ) ;
#4270=CARTESIAN_POINT ( 'NONE',  ( 97.30629616937498838, 91.33154071421968467, 74.93197916753381094 ) ) ;
#4279=CARTESIAN_POINT ( 'NONE',  ( 92.69370383062498320, 91.33154071421968467, 89.58989583420047609 ) ) ;
#4280=EDGE_CURVE ( 'NONE', #62636, #53174, #70531, .T. ) ;
#4283=CARTESIAN_POINT ( 'NONE',  ( 97.30629616937498838, -211.3315407142195852, 86.73239583420047438 ) ) ;
#4286=CARTESIAN_POINT ( 'NONE',  ( -96.32499999999996021, -207.7050326799711968, 80.36916666666665776 ) ) ;
#4290=CARTESIAN_POINT ( 'NONE',  ( -92.34999999999999432, -209.9999999999999716, 82.69749999999999091 ) ) ;
#4292=CARTESIAN_POINT ( 'NONE',  ( -94.99999999999997158, -207.3369185715606307, 87.57906250086713840 ) ) ;
#4293=CARTESIAN_POINT ( 'NONE',  ( -93.84685191531252713, 88.00268892867056536, 84.29822916753381890 ) ) ;
#4296=CARTESIAN_POINT ( 'NONE',  ( 94.99999999999998579, 87.33691857156068750, 89.16656250086712987 ) ) ;
#4297=CARTESIAN_POINT ( 'NONE',  ( -95.00000000000002842, 92.66308142843932671, 86.94406250086714749 ) ) ;
#4300=CARTESIAN_POINT ( 'NONE',  ( 97.30629616937498838, 89.06967028092473981, 74.84209033237942776 ) ) ;
#4303=CARTESIAN_POINT ( 'NONE',  ( -95.00000000000002842, 90.00000000000004263, 90.00000000000000000 ) ) ;
#4306=CARTESIAN_POINT ( 'NONE',  ( -96.15314808468745866, -211.9973110713294489, 89.11364583420048291 ) ) ;
#4308=CARTESIAN_POINT ( 'NONE',  ( -95.00000000000002842, 90.00000000000004263, 90.00000000000000000 ) ) ;
#4313=CARTESIAN_POINT ( 'NONE',  ( -97.65000000000001990, 90.00000000000004263, 80.47499999999999432 ) ) ;
#4315=CARTESIAN_POINT ( 'NONE',  ( 97.64999999999989200, -208.4700217866474077, 75.76541666666668107 ) ) ;
#4322=CARTESIAN_POINT ( 'NONE',  ( -96.15314808468752972, 91.99731107132950569, 81.91697916753381037 ) ) ;
#4328=CARTESIAN_POINT ( 'NONE',  ( -93.84685191531247028, -211.9973110713294489, 89.37822916753381719 ) ) ;
#4330=CARTESIAN_POINT ( 'NONE',  ( 96.15314808468748708, 88.00268892867053694, 79.21822916753382060 ) ) ;
#4331=CARTESIAN_POINT ( 'NONE',  ( -92.69370383062498320, -209.9999999999999716, 83.13406250086715943 ) ) ;
#4335=CARTESIAN_POINT ( 'NONE',  ( -97.64999999999994884, -211.5299782133524502, 77.98791666666664923 ) ) ;
#4340=CIRCLE ( 'NONE', #30712, 2.649999999999985700 ) ;
#4341=EDGE_CURVE ( 'NONE', #69813, #62636, #18489, .T. ) ;
#4342=CARTESIAN_POINT ( 'NONE',  ( -97.30629616937501680, 88.66845928578038638, 79.05947916753382287 ) ) ;
#4343=CARTESIAN_POINT ( 'NONE',  ( 93.84685191531249870, -208.0026889286704943, 80.64697916753381435 ) ) ;
#4344=VERTEX_POINT ( 'NONE', #50783 ) ;
#4348=EDGE_LOOP ( 'NONE', ( #29664, #31807, #63172, #69094 ) ) ;
#4349=FACE_OUTER_BOUND ( 'NONE', #73662, .T. ) ;
#4352=ORIENTED_EDGE ( 'NONE', *, *, #36729, .F. ) ;
#4353=CARTESIAN_POINT ( 'NONE',  ( 92.69370383062501162, -208.6684592857803295, 76.41364583420049428 ) ) ;
#4357=CARTESIAN_POINT ( 'NONE',  ( 97.30629616937498838, 91.33154071421968467, 86.99697916753382287 ) ) ;
#4358=CARTESIAN_POINT ( 'NONE',  ( 2.499999999999988454, -65.00000000000000000, -290.0000000000000568 ) ) ;
#4359=CARTESIAN_POINT ( 'NONE',  ( 95.00000000000000000, -213.0599564267049857, 76.82374999999998977 ) ) ;
#4361=ORIENTED_EDGE ( 'NONE', *, *, #67415, .T. ) ;
#4370=CARTESIAN_POINT ( 'NONE',  ( 95.00000000000000000, -213.0599564267049857, 82.61812500173428475 ) ) ;
#4374=CARTESIAN_POINT ( 'NONE',  ( -94.99999999999997158, -213.0599564267049857, 81.34812500173430294 ) ) ;
#4379=CARTESIAN_POINT ( 'NONE',  ( 93.67499999999999716, 87.70503267997126784, 82.56520833506762358 ) ) ;
#4380=CARTESIAN_POINT ( 'NONE',  ( -96.32500000000001705, 92.29496732002878900, 83.62354166840097491 ) ) ;
#4382=CARTESIAN_POINT ( 'NONE',  ( 96.15314808468748708, 91.99731107132950569, 84.50989583420049200 ) ) ;
#4393=ORIENTED_EDGE ( 'NONE', *, *, #68628, .F. ) ;
#4401=CARTESIAN_POINT ( 'NONE',  ( -97.65000000000001990, 90.00000000000004263, 79.91937500173429498 ) ) ;
#4403=CARTESIAN_POINT ( 'NONE',  ( -93.84685191531248449, -208.0026889286704943, 81.33489583420049485 ) ) ;
#4406=ORIENTED_EDGE ( 'NONE', *, *, #30646, .T. ) ;
#4407=CARTESIAN_POINT ( 'NONE',  ( -92.35000000000000853, -209.9999996502046429, 77.69687501385436690 ) ) ;
#4411=CARTESIAN_POINT ( 'NONE',  ( 96.15314808468748708, 91.99731107132950569, 78.00114583420048575 ) ) ;
#4412=CARTESIAN_POINT ( 'NONE',  ( 97.64999999999999147, -209.9999999999999716, 90.00000000000000000 ) ) ;
#4417=CARTESIAN_POINT ( 'NONE',  ( 93.67500000000001137, -212.2949673200287179, 84.39083333333333314 ) ) ;
#4420=CARTESIAN_POINT ( 'NONE',  ( 94.99999999999998579, 86.94004357329502852, 76.90312500173429555 ) ) ;
#4423=CARTESIAN_POINT ( 'NONE',  ( -97.30629616937501680, 90.00000000000004263, 82.65781250086713783 ) ) ;
#4426=EDGE_CURVE ( 'NONE', #43916, #51617, #15649, .T. ) ;
#4430=DIRECTION ( 'NONE',  ( -0.000000000000000000, -0.000000000000000000, 1.000000000000000000 ) ) ;
#4431=CARTESIAN_POINT ( 'NONE',  ( 99.99999999999998579, 95.00000000000002842, -90.00000000000000000 ) ) ;
#4436=CARTESIAN_POINT ( 'NONE',  ( 93.84685191531251292, -211.9973110713294489, 77.20739583420048291 ) ) ;
#4444=DIRECTION ( 'NONE',  ( -0.000000000000000000, -0.000000000000000000, 1.000000000000000000 ) ) ;
#4445=( BOUNDED_CURVE ( )  B_SPLINE_CURVE ( 2, ( #30532, #911, #12141, #46738, #53115, #29791, #11758 ),
 .UNSPECIFIED., .F., .T. ) 
 B_SPLINE_CURVE_WITH_KNOTS ( ( 3, 2, 2, 3 ),
 ( 0.6250000000000003331, 0.6319444444444446418, 0.6388888888888890616, 0.6458333333333334814 ),
 .UNSPECIFIED. ) 
 CURVE ( )  GEOMETRIC_REPRESENTATION_ITEM ( )  RATIONAL_B_SPLINE_CURVE ( ( 0.9999999999999935607, 0.8660254037844451469, 1.000000000000000000, 0.8660254037844387076, 1.000000000000000000, 0.8660254037844365982, 1.000000000000002220 ) ) 
 REPRESENTATION_ITEM ( '' )  );
#4450=CARTESIAN_POINT ( 'NONE',  ( 95.00000000000000000, -213.0599564267049857, 86.98374999999998636 ) ) ;
#4451=VERTEX_POINT ( 'NONE', #11667 ) ;
#4457=EDGE_CURVE ( 'NONE', #8687, #55876, #23340, .T. ) ;
#4462=CARTESIAN_POINT ( 'NONE',  ( 92.35000000010806787, -209.9999848944895007, 78.64888723592486031 ) ) ;
#4463=CARTESIAN_POINT ( 'NONE',  ( 92.35000000000000853, -209.9999999999999716, 80.55437500173430010 ) ) ;
#4464=CARTESIAN_POINT ( 'NONE',  ( 93.67499999999998295, 92.29496732002878900, 82.27416666666665890 ) ) ;
#4471=CARTESIAN_POINT ( 'NONE',  ( -97.30629616937501680, 88.66845928578038638, 82.86947916753379673 ) ) ;
#4472=CARTESIAN_POINT ( 'NONE',  ( 93.84685191531248449, 88.00268892867053694, 77.68364583420047609 ) ) ;
#4480=CARTESIAN_POINT ( 'NONE',  ( -94.99999999999997158, -207.3369185715606307, 81.86406250086714920 ) ) ;
#4483=DIRECTION ( 'NONE',  ( 0.000000000000000000, -0.000000000000000000, -1.000000000000000000 ) ) ;
#4488=CARTESIAN_POINT ( 'NONE',  ( -92.69370383062498320, -208.6684592857803011, 74.77322916753379900 ) ) ;
#4498=CARTESIAN_POINT ( 'NONE',  ( -97.65000000000001990, 90.00000000000004263, 89.36499999999999488 ) ) ;
#4499=CARTESIAN_POINT ( 'NONE',  ( 92.69370383062498320, 88.66845928578035796, 88.42572916753381662 ) ) ;
#4501=VECTOR ( 'NONE', #45288, 1000.000000000000000 ) ;
#4503=CARTESIAN_POINT ( 'NONE',  ( 96.32499999999998863, 87.70503267997126784, 81.40104166840096411 ) ) ;
#4506=EDGE_CURVE ( 'NONE', #71815, #43675, #27859, .T. ) ;
#4519=CARTESIAN_POINT ( 'NONE',  ( -97.64999999999994884, -211.5299782133524502, 84.97291666666666288 ) ) ;
#4526=CARTESIAN_POINT ( 'NONE',  ( 97.64999999999999147, -209.9999999999999716, 85.23749999999999716 ) ) ;
#4527=CARTESIAN_POINT ( 'NONE',  ( 93.84685191531249870, -208.0026889286704943, 89.69572916753382685 ) ) ;
#4536=CARTESIAN_POINT ( 'NONE',  ( 92.69370383062501162, -209.9999999999999716, 78.84781250086714977 ) ) ;
#4537=VECTOR ( 'NONE', #73302, 1000.000000000000000 ) ;
#4539=CARTESIAN_POINT ( 'NONE',  ( 97.30629616937498838, -209.9999999999999716, 86.30906250086715659 ) ) ;
#4541=ORIENTED_EDGE ( 'NONE', *, *, #18001, .F. ) ;
#4544=CARTESIAN_POINT ( 'NONE',  ( -92.69370383062502583, 88.66845928578038638, 75.46114583420049371 ) ) ;
#4550=CARTESIAN_POINT ( 'NONE',  ( -97.65000000000001990, 90.00000000000004263, 77.29999999999999716 ) ) ;
#4551=CARTESIAN_POINT ( 'NONE',  ( 93.67500000000001137, -207.7050326799711968, 88.70354166840097321 ) ) ;
#4559=CARTESIAN_POINT ( 'NONE',  ( 95.00000000000000000, -207.3369185715606307, 75.51406250086714067 ) ) ;
#4568=DIRECTION ( 'NONE',  ( -0.000000000000000000, -1.000000000000000000, -0.000000000000000000 ) ) ;
#4569=AXIS2_PLACEMENT_3D ( 'NONE', #6286, #1041, #34845 ) ;
#4571=CARTESIAN_POINT ( 'NONE',  ( -93.33920801875069628, 88.39975876321990711, 74.80065669543250806 ) ) ;
#4573=VERTEX_POINT ( 'NONE', #25186 ) ;
#4574=CARTESIAN_POINT ( 'NONE',  ( 97.30629616937498838, 91.33154071421968467, 78.58322916753381548 ) ) ;
#4581=CARTESIAN_POINT ( 'NONE',  ( -92.34999999999999432, -210.0000000255707278, 84.04687500080852658 ) ) ;
#4582=CARTESIAN_POINT ( 'NONE',  ( -97.30629616937497417, -208.6684592857803295, 79.42989583420047950 ) ) ;
#4589=EDGE_CURVE ( 'NONE', #32411, #35173, #59400, .T. ) ;
#4590=CARTESIAN_POINT ( 'NONE',  ( 93.67499999999998295, 92.29496732002878900, 84.81416666666666515 ) ) ;
#4592=CARTESIAN_POINT ( 'NONE',  ( 92.69400202757779539, -209.0535479562711600, 74.89836836546776055 ) ) ;
#4593=CARTESIAN_POINT ( 'NONE',  ( -93.84685191531252713, 88.00268892867056536, 80.32947916753380468 ) ) ;
#4596=VECTOR ( 'NONE', #57520, 1000.000000000000000 ) ;
#4600=ADVANCED_FACE ( 'NONE', ( #41727 ), #43237, .F. ) ;
#4603=DIRECTION ( 'NONE',  ( -0.000000000000000000, -0.000000000000000000, 1.000000000000000000 ) ) ;
#4607=CARTESIAN_POINT ( 'NONE',  ( -93.67499999999998295, -207.7050326799711968, 79.07270833506763097 ) ) ;
#4608=CARTESIAN_POINT ( 'NONE',  ( -92.69370383062498320, -209.9999999999999716, 78.05406250086716113 ) ) ;
#4614=CARTESIAN_POINT ( 'NONE',  ( -96.32500000000001705, 87.70503267997129626, 80.66020833506763665 ) ) ;
#4627=LINE ( 'NONE', #33531, #46307 ) ;
#4630=CARTESIAN_POINT ( 'NONE',  ( 93.84685191531251292, -211.9973110713294489, 87.84364583420047268 ) ) ;
#4639=ORIENTED_EDGE ( 'NONE', *, *, #25137, .F. ) ;
#4644=CARTESIAN_POINT ( 'NONE',  ( 94.99999999999998579, 87.33691857156068750, 77.26031250086714408 ) ) ;
#4646=CARTESIAN_POINT ( 'NONE',  ( 95.00000000000000000, -209.9999999999999716, 90.00000000000000000 ) ) ;
#4652=CARTESIAN_POINT ( 'NONE',  ( 94.99999999999998579, 92.66308142843935514, 88.21406250086714351 ) ) ;
#4654=CARTESIAN_POINT ( 'NONE',  ( 96.15314808468748708, -208.0026889286704943, 84.98614583420047097 ) ) ;
#4657=CARTESIAN_POINT ( 'NONE',  ( -93.67500000000003979, 92.29496732002878900, 77.16770833506762983 ) ) ;
#4663=CARTESIAN_POINT ( 'NONE',  ( -97.30629616937497417, -208.6684592857803011, 87.04989583420048405 ) ) ;
#4664=CARTESIAN_POINT ( 'NONE',  ( -97.30629616937501680, 91.33154071421968467, 85.93864583420048575 ) ) ;
#4666=CARTESIAN_POINT ( 'NONE',  ( 97.30629616937498838, 91.33154071421968467, 89.37822916753381719 ) ) ;
#4667=CARTESIAN_POINT ( 'NONE',  ( -97.30629616937501680, 91.33154071421968467, 85.77989583420048803 ) ) ;
#4670=CARTESIAN_POINT ( 'NONE',  ( -92.34999999999999432, -211.5299782133524218, 80.81895833506763438 ) ) ;
#4673=CARTESIAN_POINT ( 'NONE',  ( -92.69370383062498320, -209.9999999999999716, 88.69031250086715090 ) ) ;
#4674=CARTESIAN_POINT ( 'NONE',  ( -97.65000000000001990, 90.00000000000004263, 90.00000000000000000 ) ) ;
#4675=EDGE_CURVE ( 'NONE', #52450, #18128, #7523, .T. ) ;
#4683=CARTESIAN_POINT ( 'NONE',  ( -95.00000000000002842, 93.05995642670501411, 82.22124999999999773 ) ) ;
#4685=FACE_OUTER_BOUND ( 'NONE', #13111, .T. ) ;
#4692=( BOUNDED_CURVE ( )  B_SPLINE_CURVE ( 2, ( #58874, #6981, #64145, #14093, #37043, #70128, #19371 ),
 .UNSPECIFIED., .F., .F. ) 
 B_SPLINE_CURVE_WITH_KNOTS ( ( 3, 2, 2, 3 ),
 ( 0.8958333333333331483, 0.9027777777777775681, 0.9097222222222218768, 0.9166666666666662966 ),
 .UNSPECIFIED. ) 
 CURVE ( )  GEOMETRIC_REPRESENTATION_ITEM ( )  RATIONAL_B_SPLINE_CURVE ( ( 1.000000000000004219, 0.8660254037844343777, 1.000000000000000000, 0.8660254037844387076, 1.000000000000000000, 0.8660254037844451469, 0.9999999999999935607 ) ) 
 REPRESENTATION_ITEM ( '' )  );
#4694=CARTESIAN_POINT ( 'NONE',  ( -92.69370383062502583, 91.33154071421968467, 80.48822916753383083 ) ) ;
#4701=CARTESIAN_POINT ( 'NONE',  ( -93.84685191531248449, -208.0026889286704943, 88.95489583420049939 ) ) ;
#4706=CARTESIAN_POINT ( 'NONE',  ( 92.69370383062498320, 91.33154071421968467, 80.85864583420048746 ) ) ;
#4710=CARTESIAN_POINT ( 'NONE',  ( -93.84685191531248449, -208.0026889286704943, 78.79489583420048859 ) ) ;
#4718=CARTESIAN_POINT ( 'NONE',  ( -92.69370383062504004, 90.00000000000004263, 78.05406250086716113 ) ) ;
#4719=CARTESIAN_POINT ( 'NONE',  ( 97.30629616937498838, -211.3315407142195852, 80.38239583420049428 ) ) ;
#4724=DIRECTION ( 'NONE',  ( 1.000000000000000000, 0.000000000000000000, 0.000000000000000000 ) ) ;
#4725=ORIENTED_EDGE ( 'NONE', *, *, #35646, .T. ) ;
#4727=CARTESIAN_POINT ( 'NONE',  ( -97.65000000000004832, -208.4700217866475214, 83.59708333333334451 ) ) ;
#4734=CARTESIAN_POINT ( 'NONE',  ( 93.84685191531249870, -208.0026889286704943, 76.36072916753381890 ) ) ;
#4739=CARTESIAN_POINT ( 'NONE',  ( 97.30629616937498838, 91.33154071421968467, 86.36197916753383197 ) ) ;
#4741=CARTESIAN_POINT ( 'NONE',  ( 92.35000000000002274, -208.4700217866474645, 78.51708333333334622 ) ) ;
#4753=CARTESIAN_POINT ( 'NONE',  ( -97.64999999999996305, -209.9999999999999716, 81.18937500173430521 ) ) ;
#4757=CARTESIAN_POINT ( 'NONE',  ( 97.64999999999997726, 91.52997821335252127, 84.09979166840095388 ) ) ;
#4758=CARTESIAN_POINT ( 'NONE',  ( -97.65000000000001990, 90.00000000000004263, 83.72937500173429726 ) ) ;
#4761=CARTESIAN_POINT ( 'NONE',  ( 92.69370383062498320, 88.66845928578037217, 83.50447916753383026 ) ) ;
#4762=CARTESIAN_POINT ( 'NONE',  ( -96.32499999999996021, -207.7050326799711968, 86.71916666666666629 ) ) ;
#4764=CARTESIAN_POINT ( 'NONE',  ( -89.99999999999998579, -124.0000000000000142, -40.00000000000002132 ) ) ;
#4767=CARTESIAN_POINT ( 'NONE',  ( -95.00000000000002842, 90.00000000000004263, 90.00000000000000000 ) ) ;
#4768=CARTESIAN_POINT ( 'NONE',  ( 97.65000000000000568, 91.52997821335252127, 81.55979166840097605 ) ) ;
#4774=DIRECTION ( 'NONE',  ( 1.000000000000000000, 0.000000000000000000, 0.000000000000000000 ) ) ;
#4777=ORIENTED_EDGE ( 'NONE', *, *, #38167, .T. ) ;
#4778=EDGE_CURVE ( 'NONE', #22408, #58433, #16125, .T. ) ;
#4781=DIRECTION ( 'NONE',  ( -0.000000000000000000, -0.000000000000000000, 1.000000000000000000 ) ) ;
#4782=CARTESIAN_POINT ( 'NONE',  ( -96.32500000000001705, 87.70503267997129626, 80.02520833506763154 ) ) ;
#4785=CARTESIAN_POINT ( 'NONE',  ( -97.30629616937497417, -211.3315407142195852, 81.59947916753381492 ) ) ;
#4788=ORIENTED_EDGE ( 'NONE', *, *, #64050, .T. ) ;
#4800=CARTESIAN_POINT ( 'NONE',  ( 2.499999999999984457, -73.00000000000001421, -208.2999999999999261 ) ) ;
#4806=CARTESIAN_POINT ( 'NONE',  ( 92.34999999999993747, 91.52997821335250705, 89.31208333333333371 ) ) ;
#4808=CARTESIAN_POINT ( 'NONE',  ( -92.69370383062504004, 90.00000000000004263, 79.80031250086713612 ) ) ;
#4809=EDGE_CURVE ( 'NONE', #30790, #33107, #61758, .T. ) ;
#4811=LINE ( 'NONE', #44653, #21320 ) ;
#4820=CARTESIAN_POINT ( 'NONE',  ( 97.64999999999999147, -210.0000000198592716, 85.95187500101400246 ) ) ;
#4821=CARTESIAN_POINT ( 'NONE',  ( 97.30629616937498838, -209.9999999999999716, 76.14906250086716000 ) ) ;
#4826=CARTESIAN_POINT ( 'NONE',  ( -97.64999999950698850, -210.0000320324311076, 85.63541623677365067 ) ) ;
#4830=CARTESIAN_POINT ( 'NONE',  ( 96.32499999999998863, -207.7050326799711968, 87.88333333333332575 ) ) ;
#4832=CARTESIAN_POINT ( 'NONE',  ( 92.34999999999999432, 90.00000000000002842, 90.00000000000000000 ) ) ;
#4840=AXIS2_PLACEMENT_3D ( 'NONE', #39585, #62532, #67026 ) ;
#4841=VERTEX_POINT ( 'NONE', #33787 ) ;
#4842=CARTESIAN_POINT ( 'NONE',  ( -92.34999999999999432, -210.0000000983656605, 80.23687499810813506 ) ) ;
#4843=CARTESIAN_POINT ( 'NONE',  ( 95.00000000000000000, -206.9400435732949575, 80.39562500173431658 ) ) ;
#4844=CARTESIAN_POINT ( 'NONE',  ( 94.99999999999998579, 86.94004357329500010, 81.26874999999999716 ) ) ;
#4852=CARTESIAN_POINT ( 'NONE',  ( -95.00000000000002842, 87.33691857156074434, 84.88031250086713442 ) ) ;
#4853=CARTESIAN_POINT ( 'NONE',  ( 96.15314808468748708, 91.99731107132950569, 79.90614583420047268 ) ) ;
#4862=CARTESIAN_POINT ( 'NONE',  ( -96.15314808468747287, -208.0026889286704943, 76.83697916753381207 ) ) ;
#4866=CARTESIAN_POINT ( 'NONE',  ( 92.34999999999996589, 88.47002178664753558, 79.89291666666666458 ) ) ;
#4867=EDGE_CURVE ( 'NONE', #23574, #50963, #22895, .T. ) ;
#4873=CARTESIAN_POINT ( 'NONE',  ( -97.30629616937497417, -208.6684592857803011, 77.52489583420046415 ) ) ;
#4875=CARTESIAN_POINT ( 'NONE',  ( 94.99999999999998579, 93.05995642670504253, 88.65062500173428361 ) ) ;
#4884=CARTESIAN_POINT ( 'NONE',  ( 97.30629616937498838, 90.00000000000002842, 84.24531250086714351 ) ) ;
#4886=CARTESIAN_POINT ( 'NONE',  ( -92.34999999999999432, -209.9999998456625860, 79.60187500750915035 ) ) ;
#4898=AXIS2_PLACEMENT_3D ( 'NONE', #60949, #15833, #20359 ) ;
#4899=EDGE_CURVE ( 'NONE', #26229, #19675, #35399, .T. ) ;
#4902=CARTESIAN_POINT ( 'NONE',  ( -96.32499999999996021, -207.7050326799711968, 84.81416666666666515 ) ) ;
#4904=( BOUNDED_CURVE ( )  B_SPLINE_CURVE ( 2, ( #65978, #20083, #66346, #49025, #59969, #3206, #2486 ),
 .UNSPECIFIED., .F., .F. ) 
 B_SPLINE_CURVE_WITH_KNOTS ( ( 3, 2, 2, 3 ),
 ( 0.1458333333333334536, 0.1527777777777778734, 0.1597222222222222654, 0.1666666666666666852 ),
 .UNSPECIFIED. ) 
 CURVE ( )  GEOMETRIC_REPRESENTATION_ITEM ( )  RATIONAL_B_SPLINE_CURVE ( ( 0.9999999999999978906, 0.8660254037844408170, 1.000000000000000000, 0.8660254037844387076, 1.000000000000000000, 0.8660254037844381525, 1.000000000000000444 ) ) 
 REPRESENTATION_ITEM ( '' )  );
#4908=CARTESIAN_POINT ( 'NONE',  ( 93.84685191531251292, -211.9973110713294489, 87.36739583420049371 ) ) ;
#4910=ORIENTED_EDGE ( 'NONE', *, *, #42193, .T. ) ;
#4914=CARTESIAN_POINT ( 'NONE',  ( 97.30629616937498838, -211.3315407142195852, 78.47739583420047893 ) ) ;
#4915=ORIENTED_EDGE ( 'NONE', *, *, #55685, .F. ) ;
#4916=CARTESIAN_POINT ( 'NONE',  ( 96.15314808468750130, -211.9973110713294489, 83.66322916753382799 ) ) ;
#4918=ORIENTED_EDGE ( 'NONE', *, *, #41592, .F. ) ;
#4936=CARTESIAN_POINT ( 'NONE',  ( 93.84685191531249870, -208.0026889286704943, 75.56697916753381605 ) ) ;
#4949=CARTESIAN_POINT ( 'NONE',  ( -95.00000000000002842, 87.33691857156074434, 75.99031250086716227 ) ) ;
#4951=EDGE_LOOP ( 'NONE', ( #55296, #68665, #38832, #49643 ) ) ;
#4953=CARTESIAN_POINT ( 'NONE',  ( -94.99999999999997158, -207.3369185715606307, 85.03906250086714635 ) ) ;
#4954=EDGE_CURVE ( 'NONE', #32656, #47166, #58903, .T. ) ;
#4956=CARTESIAN_POINT ( 'NONE',  ( 96.91640186574987581, -211.8303114255586479, 74.99954695036826990 ) ) ;
#4958=CARTESIAN_POINT ( 'NONE',  ( -97.30629616937495996, -209.9999999999999716, 78.84781250086714977 ) ) ;
#4966=DIRECTION ( 'NONE',  ( -0.000000000000000000, -0.000000000000000000, 1.000000000000000000 ) ) ;
#4967=EDGE_CURVE ( 'NONE', #72633, #23298, #55048, .T. ) ;
#4968=CARTESIAN_POINT ( 'NONE',  ( -97.30629616937501680, 91.33154071421968467, 80.69989583420048973 ) ) ;
#4975=DIRECTION ( 'NONE',  ( -3.061616997868382648E-16, -1.000000000000000000, 0.000000000000000000 ) ) ;
#4978=CARTESIAN_POINT ( 'NONE',  ( -97.65000000000001990, 90.00000000000004263, 90.00000000000000000 ) ) ;
#4980=CARTESIAN_POINT ( 'NONE',  ( 97.64999999994533653, -210.0000170172949367, 88.49187441316098557 ) ) ;
#4981=CARTESIAN_POINT ( 'NONE',  ( -93.84685191531248449, -208.0026889286704943, 80.69989583420047552 ) ) ;
#4984=CARTESIAN_POINT ( 'NONE',  ( -93.07557990970633455, 88.17815826261617929, 75.00000000000001421 ) ) ;
#4988=CARTESIAN_POINT ( 'NONE',  ( 92.34999999999999432, 89.99996514701891215, 77.37937620717863751 ) ) ;
#4989=CARTESIAN_POINT ( 'NONE',  ( 92.35000000000000853, -209.9999999999999716, 84.92000000000000171 ) ) ;
#4992=LINE ( 'NONE', #9866, #20406 ) ;
#4994=CARTESIAN_POINT ( 'NONE',  ( -96.32500000000001705, 92.29496732002878900, 76.00354166840097037 ) ) ;
#4998=CARTESIAN_POINT ( 'NONE',  ( 92.69370383062501162, -211.3315407142195852, 88.42572916753381662 ) ) ;
#5007=ORIENTED_EDGE ( 'NONE', *, *, #29761, .F. ) ;
#5016=CARTESIAN_POINT ( 'NONE',  ( 92.34999999999999432, 90.00000000000002842, 87.45999999999999375 ) ) ;
#5023=CARTESIAN_POINT ( 'NONE',  ( 97.30629616937498838, 90.00000000000002842, 88.69031250086715090 ) ) ;
#5025=CARTESIAN_POINT ( 'NONE',  ( 95.00000000000000000, -207.3369185715606307, 86.30906250086715659 ) ) ;
#5026=DIRECTION ( 'NONE',  ( -0.000000000000000000, -0.000000000000000000, 1.000000000000000000 ) ) ;
#5029=CARTESIAN_POINT ( 'NONE',  ( -95.00000000000002842, 93.05995642670504253, 77.85562500173431033 ) ) ;
#5033=CARTESIAN_POINT ( 'NONE',  ( -97.30629616937497417, -211.3315407142195852, 86.52072916753381548 ) ) ;
#5034=CARTESIAN_POINT ( 'NONE',  ( -95.00000000000002842, 92.66308142843932671, 84.56281250086716739 ) ) ;
#5035=AXIS2_PLACEMENT_3D ( 'NONE', #4767, #26919, #11123 ) ;
#5037=CARTESIAN_POINT ( 'NONE',  ( 92.69370383062498320, 91.33154071421968467, 86.41489583420047893 ) ) ;
#5038=CARTESIAN_POINT ( 'NONE',  ( -92.69370383062502583, 88.66845928578038638, 85.46239583420047836 ) ) ;
#5053=EDGE_LOOP ( 'NONE', ( #16686, #40975, #46032, #69757 ) ) ;
#5054=CARTESIAN_POINT ( 'NONE',  ( -95.00000000000002842, 93.05995642670501411, 82.85625000000000284 ) ) ;
#5056=CARTESIAN_POINT ( 'NONE',  ( -2.499999999999970690, 73.00000000000001421, -208.2999999999999545 ) ) ;
#5058=CYLINDRICAL_SURFACE ( 'NONE', #44187, 2.649999999999985700 ) ;
#5060=CARTESIAN_POINT ( 'NONE',  ( -93.67499999999998295, -212.2949673200287179, 76.95604166840095672 ) ) ;
#5063=CARTESIAN_POINT ( 'NONE',  ( -94.99999999999997158, -206.9400435732949575, 79.68124999999999147 ) ) ;
#5066=CARTESIAN_POINT ( 'NONE',  ( -96.15314808468751551, 88.00268892867056536, 78.95364583420047211 ) ) ;
#5072=CARTESIAN_POINT ( 'NONE',  ( -92.69370383062498320, -209.9999999999999716, 89.48406250086715374 ) ) ;
#5075=CARTESIAN_POINT ( 'NONE',  ( 96.15314808468748708, 88.00268892867053694, 80.48822916753381662 ) ) ;
#5076=CARTESIAN_POINT ( 'NONE',  ( -92.69370383062498320, -211.3315407142195852, 78.63614583420046245 ) ) ;
#5080=CARTESIAN_POINT ( 'NONE',  ( -97.65000000000001990, 90.00000000000004263, 86.90437500173429441 ) ) ;
#5081=VECTOR ( 'NONE', #56739, 1000.000000000000000 ) ;
#5085=CARTESIAN_POINT ( 'NONE',  ( -93.84685191531252713, 88.00268892867056536, 78.58322916753382970 ) ) ;
#5086=CARTESIAN_POINT ( 'NONE',  ( 97.30629616937498838, -209.9999999999999716, 79.16531250086714522 ) ) ;
#5092=VERTEX_POINT ( 'NONE', #49033 ) ;
#5101=CARTESIAN_POINT ( 'NONE',  ( 96.66078148566039374, -211.6002521295064867, 74.80065602173002048 ) ) ;
#5106=CARTESIAN_POINT ( 'NONE',  ( 96.15314808468748708, 91.99731107132950569, 87.68489583420048916 ) ) ;
#5108=CARTESIAN_POINT ( 'NONE',  ( 95.00000000000000000, -213.0599564267049857, 79.36374999999999602 ) ) ;
#5115=LINE ( 'NONE', #73130, #69154 ) ;
#5119=CARTESIAN_POINT ( 'NONE',  ( 94.99999999999998579, 86.94004357329502852, 83.88812500173429498 ) ) ;
#5121=CARTESIAN_POINT ( 'NONE',  ( -92.34999999999999432, -211.5299782133524502, 83.35895833506762642 ) ) ;
#5124=CARTESIAN_POINT ( 'NONE',  ( 94.99999999999998579, 93.05995642670504253, 83.57062500173429953 ) ) ;
#5125=CARTESIAN_POINT ( 'NONE',  ( -93.67500000000003979, 92.29496732002878900, 79.07270833506763097 ) ) ;
#5126=( BOUNDED_CURVE ( )  B_SPLINE_CURVE ( 2, ( #20494, #43808, #21208, #31755, #14844, #65620, #44160 ),
 .UNSPECIFIED., .F., .F. ) 
 B_SPLINE_CURVE_WITH_KNOTS ( ( 3, 2, 2, 3 ),
 ( 0.1666666666666666852, 0.1736111111111111049, 0.1805555555555554970, 0.1874999999999999167 ),
 .UNSPECIFIED. ) 
 CURVE ( )  GEOMETRIC_REPRESENTATION_ITEM ( )  RATIONAL_B_SPLINE_CURVE ( ( 0.9999999999999994449, 0.8660254037844392627, 1.000000000000000000, 0.8660254037844387076, 1.000000000000000000, 0.8660254037844402619, 0.9999999999999984457 ) ) 
 REPRESENTATION_ITEM ( '' )  );
#5128=CARTESIAN_POINT ( 'NONE',  ( 97.30629616937498838, 90.00000000000002842, 82.49906250086715431 ) ) ;
#5130=CARTESIAN_POINT ( 'NONE',  ( 92.34999999999989484, 91.52997821335247863, 83.59708333333334451 ) ) ;
#5132=CYLINDRICAL_SURFACE ( 'NONE', #5035, 2.649999999999985700 ) ;
#5135=ORIENTED_EDGE ( 'NONE', *, *, #26144, .T. ) ;
#5142=FACE_OUTER_BOUND ( 'NONE', #14590, .T. ) ;
#5150=CARTESIAN_POINT ( 'NONE',  ( -97.30629616937497417, -208.6684592857803011, 82.76364583420048859 ) ) ;
#5157=CARTESIAN_POINT ( 'NONE',  ( -97.50728577674108521, -210.3406226724060559, 74.92458348457978445 ) ) ;
#5159=CARTESIAN_POINT ( 'NONE',  ( 95.00000000000000000, -209.9999999999999716, 90.00000000000000000 ) ) ;
#5168=CARTESIAN_POINT ( 'NONE',  ( -93.84685191531248449, -208.0026889286704943, 89.58989583420049030 ) ) ;
#5172=CARTESIAN_POINT ( 'NONE',  ( -96.15314808468751551, 88.00268892867056536, 79.58864583420047722 ) ) ;
#5178=LINE ( 'NONE', #22082, #11985 ) ;
#5182=CARTESIAN_POINT ( 'NONE',  ( 92.69370383062501162, -211.3315407142195852, 75.88447916753382572 ) ) ;
#5188=CARTESIAN_POINT ( 'NONE',  ( -92.34999999999999432, -208.4700217866474645, 81.55979166840097605 ) ) ;
#5191=CARTESIAN_POINT ( 'NONE',  ( 92.34999999999999432, 90.00000000000002842, 90.00000000000000000 ) ) ;
#5195=CARTESIAN_POINT ( 'NONE',  ( 95.00000000000000000, -206.9400435732949575, 89.20624999999999716 ) ) ;
#5202=DIRECTION ( 'NONE',  ( 1.000000000000000000, 0.000000000000000000, 0.000000000000000000 ) ) ;
#5203=AXIS2_PLACEMENT_3D ( 'NONE', #62774, #10490, #33409 ) ;
#5208=CARTESIAN_POINT ( 'NONE',  ( 93.67500000000001137, -207.7050326799711968, 76.63854166840096127 ) ) ;
#5209=CARTESIAN_POINT ( 'NONE',  ( 93.67499999999998295, 92.29496732002878900, 82.90916666666666401 ) ) ;
#5214=ADVANCED_FACE ( 'NONE', ( #4685 ), #56920, .F. ) ;
#5216=CARTESIAN_POINT ( 'NONE',  ( -97.65000000000001990, 88.47002178664754979, 88.86229166840097093 ) ) ;
#5217=CARTESIAN_POINT ( 'NONE',  ( -96.15314808468751551, 88.00268892867056536, 84.19239583420049655 ) ) ;
#5218=CARTESIAN_POINT ( 'NONE',  ( 97.30629616937498838, 91.33154071421968467, 77.31322916753380525 ) ) ;
#5222=CYLINDRICAL_SURFACE ( 'NONE', #54450, 2.649999999999985700 ) ;
#5227=EDGE_CURVE ( 'NONE', #55546, #26437, #7918, .T. ) ;
#5228=CARTESIAN_POINT ( 'NONE',  ( -94.99999999999997158, -212.6630814284392557, 78.37156250086714238 ) ) ;
#5234=CARTESIAN_POINT ( 'NONE',  ( 94.99999999999998579, 86.94004357329502852, 78.09374999999998579 ) ) ;
#5235=VECTOR ( 'NONE', #63781, 1000.000000000000000 ) ;
#5237=VERTEX_POINT ( 'NONE', #5056 ) ;
#5238=CARTESIAN_POINT ( 'NONE',  ( -97.30629616937495996, -209.9999999999999716, 89.80156250086714920 ) ) ;
#5241=CARTESIAN_POINT ( 'NONE',  ( -97.65000000000001990, 90.00000000000004263, 90.00000000000000000 ) ) ;
#5244=EDGE_CURVE ( 'NONE', #40498, #64759, #54337, .T. ) ;
#5248=CARTESIAN_POINT ( 'NONE',  ( 93.84685191531248449, 88.00268892867053694, 84.03364583420047040 ) ) ;
#5263=VECTOR ( 'NONE', #37232, 1000.000000000000000 ) ;
#5266=CARTESIAN_POINT ( 'NONE',  ( -97.64999999999994884, -208.4700217866474645, 85.50208333333331723 ) ) ;
#5275=CARTESIAN_POINT ( 'NONE',  ( 93.84685191531249870, -208.0026889286704943, 85.88572916753381037 ) ) ;
#5282=VERTEX_POINT ( 'NONE', #73067 ) ;
#5285=CARTESIAN_POINT ( 'NONE',  ( 97.30629616937498838, -209.9999999999999716, 76.62531250086713897 ) ) ;
#5287=CARTESIAN_POINT ( 'NONE',  ( 93.84685191531251292, -211.9973110713294489, 82.92239583420048632 ) ) ;
#5293=CARTESIAN_POINT ( 'NONE',  ( -97.30629616937501680, 91.33154071421968467, 75.14364583420049826 ) ) ;
#5298=CARTESIAN_POINT ( 'NONE',  ( 97.64999999999997726, -208.4700217866474645, 85.36979166840096411 ) ) ;
#5305=VECTOR ( 'NONE', #19744, 1000.000000000000000 ) ;
#5310=CARTESIAN_POINT ( 'NONE',  ( 92.69370383062501162, -209.9999999999999716, 75.03781250086713328 ) ) ;
#5315=ORIENTED_EDGE ( 'NONE', *, *, #26233, .F. ) ;
#5318=LINE ( 'NONE', #67708, #47931 ) ;
#5319=CARTESIAN_POINT ( 'NONE',  ( -97.30629616937501680, 91.33154071421968467, 75.77864583420048916 ) ) ;
#5321=CARTESIAN_POINT ( 'NONE',  ( 96.15314808468748708, 88.00268892867053694, 75.24947916753380639 ) ) ;
#5324=CARTESIAN_POINT ( 'NONE',  ( -94.99999999999997158, -212.6630814284392557, 84.72156250086713669 ) ) ;
#5329=CARTESIAN_POINT ( 'NONE',  ( -93.84685191531248449, -208.0026889286704943, 76.09614583420047040 ) ) ;
#5334=CARTESIAN_POINT ( 'NONE',  ( -97.65000000000001990, 90.00000000000004263, 76.66499999999999204 ) ) ;
#5335=CARTESIAN_POINT ( 'NONE',  ( 93.65592807507104567, -207.9734350352808860, 74.86703477254889094 ) ) ;
#5336=CARTESIAN_POINT ( 'NONE',  ( -92.69370383062502583, 91.33154071421968467, 82.39322916753381776 ) ) ;
#5340=( BOUNDED_CURVE ( )  B_SPLINE_CURVE ( 2, ( #27654, #4003, #32906, #4370, #29127, #64103, #6939, #17487, #981 ),
 .UNSPECIFIED., .F., .F. ) 
 B_SPLINE_CURVE_WITH_KNOTS ( ( 3, 2, 2, 2, 3 ),
 ( 0.4445132602971393343, 0.4515689946164714308, 0.4586247601573539279, 0.4656805256982364249, 0.4656806970056959760 ),
 .UNSPECIFIED. ) 
 CURVE ( )  GEOMETRIC_REPRESENTATION_ITEM ( )  RATIONAL_B_SPLINE_CURVE ( ( 0.9999988143381259853, 0.8660259966179989499, 1.000000000000000000, 0.8660254037844387076, 1.000000000000000000, 0.8660254037844387076, 1.000000000000000000, 0.9999967472207530461, 0.9999934945994550795 ) ) 
 REPRESENTATION_ITEM ( '' )  );
#5341=ORIENTED_EDGE ( 'NONE', *, *, #13557, .T. ) ;
#5342=FACE_OUTER_BOUND ( 'NONE', #18332, .T. ) ;
#5345=VECTOR ( 'NONE', #36420, 1000.000000000000000 ) ;
#5349=CARTESIAN_POINT ( 'NONE',  ( -97.30629616937497417, -208.6684592857803011, 80.22364583420048234 ) ) ;
#5365=EDGE_CURVE ( 'NONE', #70250, #6931, #61320, .T. ) ;
#5367=LINE ( 'NONE', #56855, #23554 ) ;
#5371=CARTESIAN_POINT ( 'NONE',  ( 95.00000000000000000, -212.6630814284392557, 87.89656250086713385 ) ) ;
#5379=CARTESIAN_POINT ( 'NONE',  ( 97.64999999999999147, -209.9999999999999716, 82.06250000000000000 ) ) ;
#5382=ORIENTED_EDGE ( 'NONE', *, *, #63596, .T. ) ;
#5388=CARTESIAN_POINT ( 'NONE',  ( 93.67499999999999716, 87.70503267997126784, 86.93083333333332519 ) ) ;
#5389=CARTESIAN_POINT ( 'NONE',  ( -92.35000000000003695, 90.00000000000004263, 90.00000000000000000 ) ) ;
#5394=CARTESIAN_POINT ( 'NONE',  ( 92.69370383062498320, 91.33154071421968467, 84.50989583420046358 ) ) ;
#5396=CARTESIAN_POINT ( 'NONE',  ( 97.30629616937498838, -211.3315407142195852, 86.09739583420048348 ) ) ;
#5398=EDGE_CURVE ( 'NONE', #49261, #48383, #188, .T. ) ;
#5407=CARTESIAN_POINT ( 'NONE',  ( -93.84685191531248449, -208.0026889286704943, 87.52614583420047722 ) ) ;
#5408=CARTESIAN_POINT ( 'NONE',  ( -93.84685191531254134, 91.99731107132950569, 85.77989583420048803 ) ) ;
#5410=CARTESIAN_POINT ( 'NONE',  ( 96.15314808468748708, 88.00268892867053694, 84.13947916753380696 ) ) ;
#5411=CARTESIAN_POINT ( 'NONE',  ( -97.30629616937501680, 90.00000000000004263, 83.92781250086714806 ) ) ;
#5415=FACE_OUTER_BOUND ( 'NONE', #14412, .T. ) ;
#5416=DIRECTION ( 'NONE',  ( -0.000000000000000000, -0.000000000000000000, 1.000000000000000000 ) ) ;
#5418=CARTESIAN_POINT ( 'NONE',  ( -95.00000000000002842, 93.05995642670504253, 86.66624999999999091 ) ) ;
#5426=CARTESIAN_POINT ( 'NONE',  ( -95.00000000000002842, 93.05995642670501411, 78.41125000000000966 ) ) ;
#5430=CARTESIAN_POINT ( 'NONE',  ( -97.64999999999996305, -208.4700217866474645, 89.94708333333332462 ) ) ;
#5431=CARTESIAN_POINT ( 'NONE',  ( -96.32500000000001705, 87.70503267997129626, 86.37520833506764006 ) ) ;
#5434=CARTESIAN_POINT ( 'NONE',  ( -92.69370383062502583, 91.33154071421968467, 78.58322916753381548 ) ) ;
#5441=DIRECTION ( 'NONE',  ( -0.000000000000000000, -0.000000000000000000, 1.000000000000000000 ) ) ;
#5442=DIRECTION ( 'NONE',  ( 1.000000000000000000, 0.000000000000000000, 0.000000000000000000 ) ) ;
#5446=EDGE_CURVE ( 'NONE', #72954, #36972, #33416, .T. ) ;
#5447=CARTESIAN_POINT ( 'NONE',  ( 96.15314808468748708, 91.99731107132950569, 78.15989583420049769 ) ) ;
#5449=CARTESIAN_POINT ( 'NONE',  ( -94.99999999999997158, -212.6630814284392557, 78.53031250086715431 ) ) ;
#5453=CARTESIAN_POINT ( 'NONE',  ( -93.67499999999998295, -207.7050326799711968, 75.81833333333332803 ) ) ;
#5457=CARTESIAN_POINT ( 'NONE',  ( -96.15314808468752972, 91.99731107132950569, 76.99572916753382401 ) ) ;
#5458=CARTESIAN_POINT ( 'NONE',  ( 96.15314808468750130, -211.9973110713294489, 80.96447916753380980 ) ) ;
#5463=EDGE_CURVE ( 'NONE', #23087, #53667, #60875, .T. ) ;
#5464=CARTESIAN_POINT ( 'NONE',  ( -97.64999999999996305, -208.4700217866474645, 88.12145833506765769 ) ) ;
#5469=ORIENTED_EDGE ( 'NONE', *, *, #17302, .T. ) ;
#5472=CARTESIAN_POINT ( 'NONE',  ( 95.00000000000000000, -212.6630814284392557, 76.62531250086715318 ) ) ;
#5478=CARTESIAN_POINT ( 'NONE',  ( 92.69370383062498320, 91.33154071421968467, 82.76364583420048859 ) ) ;
#5479=CARTESIAN_POINT ( 'NONE',  ( 96.32499999999998863, -207.7050326799711968, 77.72333333333332916 ) ) ;
#5485=CARTESIAN_POINT ( 'NONE',  ( 2.500000000000029754, 73.00000000000001421, -204.9999999999999716 ) ) ;
#5492=ORIENTED_EDGE ( 'NONE', *, *, #26971, .T. ) ;
#5493=CARTESIAN_POINT ( 'NONE',  ( -96.32499999999996021, -212.2949673200287179, 83.83520833506763381 ) ) ;
#5494=ORIENTED_EDGE ( 'NONE', *, *, #45595, .T. ) ;
#5497=CARTESIAN_POINT ( 'NONE',  ( 92.34999999999999432, 91.52997821335252127, 79.23145833506762870 ) ) ;
#5498=CARTESIAN_POINT ( 'NONE',  ( -97.65000000000001990, 91.52997821335253548, 81.13645833506764404 ) ) ;
#5499=ORIENTED_EDGE ( 'NONE', *, *, #59426, .T. ) ;
#5500=CARTESIAN_POINT ( 'NONE',  ( 92.69370383062498320, 91.33154071421968467, 82.76364583420048859 ) ) ;
#5504=CARTESIAN_POINT ( 'NONE',  ( 94.99999999999998579, 93.05995642670504253, 81.66562500173431260 ) ) ;
#5517=CARTESIAN_POINT ( 'NONE',  ( -97.30629616937497417, -208.6684592857803011, 80.85864583420048746 ) ) ;
#5520=VERTEX_POINT ( 'NONE', #30540 ) ;
#5523=CARTESIAN_POINT ( 'NONE',  ( -96.25799313130249857, -212.2877248121365312, 74.97309184317589370 ) ) ;
#5526=FACE_OUTER_BOUND ( 'NONE', #28371, .T. ) ;
#5528=CARTESIAN_POINT ( 'NONE',  ( 92.35000000003357457, 89.99999234487445676, 78.01464417100922333 ) ) ;
#5530=CIRCLE ( 'NONE', #40283, 2.649999999999985700 ) ;
#5531=CARTESIAN_POINT ( 'NONE',  ( -97.64999999999996305, -209.9999999999999716, 79.20499999999999829 ) ) ;
#5532=CARTESIAN_POINT ( 'NONE',  ( 95.00000000000000000, -209.9999999999999716, 75.00000000000000000 ) ) ;
#5538=CARTESIAN_POINT ( 'NONE',  ( 92.69370383062498320, 88.66845928578035796, 86.67947916753382742 ) ) ;
#5540=CARTESIAN_POINT ( 'NONE',  ( -92.69370383062498320, -209.9999999999999716, 88.84906250086716284 ) ) ;
#5541=CARTESIAN_POINT ( 'NONE',  ( 93.67499999999999716, 87.70503267997126784, 82.48583333333333201 ) ) ;
#5545=CARTESIAN_POINT ( 'NONE',  ( -97.30629616937501680, 88.66845928578038638, 78.26572916753380582 ) ) ;
#5549=( BOUNDED_CURVE ( )  B_SPLINE_CURVE ( 2, ( #61613, #27010, #21003, #62372, #33389, #10100, #33022 ),
 .UNSPECIFIED., .F., .F. ) 
 B_SPLINE_CURVE_WITH_KNOTS ( ( 3, 2, 2, 3 ),
 ( 0.7083333333333331483, 0.7152777777777775681, 0.7222222222222220989, 0.7291666666666665186 ),
 .UNSPECIFIED. ) 
 CURVE ( )  GEOMETRIC_REPRESENTATION_ITEM ( )  RATIONAL_B_SPLINE_CURVE ( ( 1.000000000000004219, 0.8660254037844343777, 1.000000000000000000, 0.8660254037844387076, 1.000000000000000000, 0.8660254037844408170, 0.9999999999999978906 ) ) 
 REPRESENTATION_ITEM ( '' )  );
#5554=CARTESIAN_POINT ( 'NONE',  ( -92.35000000000000853, -208.4700217866474929, 84.65541666666669585 ) ) ;
#5558=CARTESIAN_POINT ( 'NONE',  ( 93.84685191531251292, -211.9973110713294489, 86.73239583420048859 ) ) ;
#5560=CARTESIAN_POINT ( 'NONE',  ( -93.67499999999998295, -207.7050326799711968, 81.61270833506763722 ) ) ;
#5563=( BOUNDED_CURVE ( )  B_SPLINE_CURVE ( 2, ( #27799, #28531, #74027, #68780, #62411, #63147, #28170 ),
 .UNSPECIFIED., .F., .F. ) 
 B_SPLINE_CURVE_WITH_KNOTS ( ( 3, 2, 2, 3 ),
 ( 0.2708333333333337034, 0.2777777777777781232, 0.2847222222222224874, 0.2916666666666669072 ),
 .UNSPECIFIED. ) 
 CURVE ( )  GEOMETRIC_REPRESENTATION_ITEM ( )  RATIONAL_B_SPLINE_CURVE ( ( 0.9999999999999924505, 0.8660254037844462571, 1.000000000000000000, 0.8660254037844387076, 1.000000000000000000, 0.8660254037844343777, 1.000000000000004219 ) ) 
 REPRESENTATION_ITEM ( '' )  );
#5566=AXIS2_PLACEMENT_3D ( 'NONE', #4303, #5416, #16675 ) ;
#5567=CARTESIAN_POINT ( 'NONE',  ( 96.32499999999998863, -212.2949673200287179, 82.03604166840096923 ) ) ;
#5568=CARTESIAN_POINT ( 'NONE',  ( 96.32499999999998863, -212.2949673200287179, 89.57666666666666799 ) ) ;
#5574=VECTOR ( 'NONE', #24030, 1000.000000000000000 ) ;
#5576=LINE ( 'NONE', #16091, #72540 ) ;
#5577=CARTESIAN_POINT ( 'NONE',  ( 96.32499999999998863, -212.2949673200287179, 78.22604166840096696 ) ) ;
#5578=CARTESIAN_POINT ( 'NONE',  ( 97.64999999999997726, 91.52997821335252127, 80.84541666666666515 ) ) ;
#5579=VERTEX_POINT ( 'NONE', #71130 ) ;
#5587=CARTESIAN_POINT ( 'NONE',  ( -92.69370383062504004, 90.00000000000004263, 81.86406250086714920 ) ) ;
#5588=CARTESIAN_POINT ( 'NONE',  ( 96.15314808468748708, 91.99731107132950569, 76.73114583420047552 ) ) ;
#5592=CARTESIAN_POINT ( 'NONE',  ( 100.0000000000000000, -214.9999999999999716, -90.00000000000000000 ) ) ;
#5596=CARTESIAN_POINT ( 'NONE',  ( -93.84685191531248449, -208.0026889286704943, 78.63614583420047666 ) ) ;
#5599=ORIENTED_EDGE ( 'NONE', *, *, #20574, .T. ) ;
#5600=CARTESIAN_POINT ( 'NONE',  ( -97.65000000000001990, 90.00000000000004263, 90.00000000000000000 ) ) ;
#5601=EDGE_LOOP ( 'NONE', ( #12654, #65551, #24404, #58922 ) ) ;
#5605=CARTESIAN_POINT ( 'NONE',  ( -96.15314808468745866, -211.9973110713294489, 77.68364583420047609 ) ) ;
#5611=CARTESIAN_POINT ( 'NONE',  ( -96.32500000000001705, 87.70503267997129626, 81.21583333333333599 ) ) ;
#5614=CARTESIAN_POINT ( 'NONE',  ( 93.84685191531248449, 91.99731107132950569, 84.45697916753380241 ) ) ;
#5616=CARTESIAN_POINT ( 'NONE',  ( -92.35000000000003695, 90.00000000000004263, 88.41249999999999432 ) ) ;
#5617=ADVANCED_FACE ( 'NONE', ( #14372 ), #36929, .F. ) ;
#5624=CARTESIAN_POINT ( 'NONE',  ( -93.67500000000003979, 92.29496732002878900, 75.81833333333332803 ) ) ;
#5627=EDGE_CURVE ( 'NONE', #55850, #68978, #21476, .T. ) ;
#5632=CARTESIAN_POINT ( 'NONE',  ( -96.32499999999996021, -207.7050326799711968, 82.27416666666665890 ) ) ;
#5634=CARTESIAN_POINT ( 'NONE',  ( 92.35000000000000853, -209.9999999999999716, 89.44437500173430067 ) ) ;
#5638=CARTESIAN_POINT ( 'NONE',  ( -97.65000000000000568, 91.52997821335254969, 77.24708333333332178 ) ) ;
#5639=EDGE_CURVE ( 'NONE', #5801, #42810, #34541, .T. ) ;
#5640=EDGE_CURVE ( 'NONE', #26437, #55546, #13967, .T. ) ;
#5643=LINE ( 'NONE', #22930, #53416 ) ;
#5645=CARTESIAN_POINT ( 'NONE',  ( 95.00000000000000000, -207.3369185715606307, 86.46781250086716852 ) ) ;
#5646=AXIS2_PLACEMENT_3D ( 'NONE', #13104, #1873, #7839 ) ;
#5650=EDGE_CURVE ( 'NONE', #58605, #55390, #56076, .T. ) ;
#5654=CARTESIAN_POINT ( 'NONE',  ( 92.69370383062501162, -211.3315407142195852, 78.90072916753381094 ) ) ;
#5655=EDGE_LOOP ( 'NONE', ( #59713, #37490, #46615, #34093 ) ) ;
#5656=CARTESIAN_POINT ( 'NONE',  ( 97.30629616937498838, -211.3315407142195852, 81.81114583420048803 ) ) ;
#5659=ORIENTED_EDGE ( 'NONE', *, *, #29268, .F. ) ;
#5664=CARTESIAN_POINT ( 'NONE',  ( 93.67500000000001137, -207.7050326799711968, 87.43354166840096298 ) ) ;
#5670=VERTEX_POINT ( 'NONE', #39533 ) ;
#5672=CARTESIAN_POINT ( 'NONE',  ( -97.64999999996638280, -210.0000076551254722, 78.01464417100379478 ) ) ;
#5673=CARTESIAN_POINT ( 'NONE',  ( -97.65000000000001990, 90.00000000000004263, 78.57000000000000739 ) ) ;
#5675=ORIENTED_EDGE ( 'NONE', *, *, #66295, .F. ) ;
#5680=( BOUNDED_CURVE ( )  B_SPLINE_CURVE ( 2, ( #72344, #43438, #59596, #8828, #71593, #66715, #31005 ),
 .UNSPECIFIED., .F., .F. ) 
 B_SPLINE_CURVE_WITH_KNOTS ( ( 3, 2, 2, 3 ),
 ( 0.3541666666666665741, 0.3611111111111109939, 0.3680555555555554137, 0.3749999999999998335 ),
 .UNSPECIFIED. ) 
 CURVE ( )  GEOMETRIC_REPRESENTATION_ITEM ( )  RATIONAL_B_SPLINE_CURVE ( ( 1.000000000000002220, 0.8660254037844365982, 1.000000000000000000, 0.8660254037844387076, 1.000000000000000000, 0.8660254037844419273, 0.9999999999999967804 ) ) 
 REPRESENTATION_ITEM ( '' )  );
#5682=CARTESIAN_POINT ( 'NONE',  ( -92.35000000000005116, 88.47002178664754979, 87.08958333333333712 ) ) ;
#5685=AXIS2_PLACEMENT_3D ( 'NONE', #35734, #52670, #70310 ) ;
#5687=DIRECTION ( 'NONE',  ( -0.000000000000000000, -0.000000000000000000, -1.000000000000000000 ) ) ;
#5688=CARTESIAN_POINT ( 'NONE',  ( -97.30629616937495996, -209.9999999999999716, 87.10281250086714522 ) ) ;
#5693=CARTESIAN_POINT ( 'NONE',  ( -92.69370383062498320, -211.3315407142195852, 76.57239583420046358 ) ) ;
#5694=ADVANCED_FACE ( 'NONE', ( #55332 ), #27495, .T. ) ;
#5704=CARTESIAN_POINT ( 'NONE',  ( -97.30629616937501680, 91.33154071421968467, 77.52489583420046415 ) ) ;
#5708=ORIENTED_EDGE ( 'NONE', *, *, #50132, .T. ) ;
#5709=CARTESIAN_POINT ( 'NONE',  ( 96.32499999999998863, 87.70503267997126784, 79.49604166840096298 ) ) ;
#5711=CARTESIAN_POINT ( 'NONE',  ( 97.64999999999999147, -210.0000217321284879, 89.12687425009498554 ) ) ;
#5716=CARTESIAN_POINT ( 'NONE',  ( -97.30629616937495996, -209.9999999999999716, 78.37156250086715659 ) ) ;
#5718=APPLICATION_CONTEXT ( 'automotive_design' ) ;
#5722=EDGE_CURVE ( 'NONE', #12189, #59848, #69430, .T. ) ;
#5735=CARTESIAN_POINT ( 'NONE',  ( 92.35000000000000853, -209.9999999999999716, 79.83999999999998920 ) ) ;
#5739=DIRECTION ( 'NONE',  ( -1.000000000000000000, -0.000000000000000000, -0.000000000000000000 ) ) ;
#5749=FACE_OUTER_BOUND ( 'NONE', #52429, .T. ) ;
#5751=EDGE_LOOP ( 'NONE', ( #16213, #49673, #409, #17324 ) ) ;
#5757=ORIENTED_EDGE ( 'NONE', *, *, #9397, .T. ) ;
#5758=CARTESIAN_POINT ( 'NONE',  ( 92.69370383062498320, 88.66845928578037217, 85.88572916753382458 ) ) ;
#5760=CARTESIAN_POINT ( 'NONE',  ( 97.30629616937498838, -208.6684592857803011, 80.48822916753383083 ) ) ;
#5762=CARTESIAN_POINT ( 'NONE',  ( -92.35000000000003695, -208.4700217866474077, 76.40041666666667197 ) ) ;
#5763=CARTESIAN_POINT ( 'NONE',  ( -97.64999999999999147, 88.47002178664753558, 84.33791666666667197 ) ) ;
#5768=CARTESIAN_POINT ( 'NONE',  ( -92.69370383062498320, -209.9999999999999716, 89.32531250086714181 ) ) ;
#5769=CARTESIAN_POINT ( 'NONE',  ( -92.69370383062504004, 90.00000000000004263, 86.94406250086716170 ) ) ;
#5771=CARTESIAN_POINT ( 'NONE',  ( 97.30629616937498838, 90.00000000000002842, 85.51531250086713953 ) ) ;
#5772=CARTESIAN_POINT ( 'NONE',  ( -95.00000000000002842, 92.66308142843932671, 86.30906250086715659 ) ) ;
#5773=( BOUNDED_CURVE ( )  B_SPLINE_CURVE ( 2, ( #2076, #24958, #3903, #19314, #8422, #13675, #26804 ),
 .UNSPECIFIED., .F., .F. ) 
 B_SPLINE_CURVE_WITH_KNOTS ( ( 3, 2, 2, 3 ),
 ( 0.02116741234828206988, 0.02822306216352941585, 0.03527882770441186089, 0.04233441017594471306 ),
 .UNSPECIFIED. ) 
 CURVE ( )  GEOMETRIC_REPRESENTATION_ITEM ( )  RATIONAL_B_SPLINE_CURVE ( ( 0.9999956052845440091, 0.8660276011782074290, 1.000000000000000000, 0.8660254037844387076, 1.000000000000000000, 0.8660288798979868252, 0.9999930479532868066 ) ) 
 REPRESENTATION_ITEM ( '' )  );
#5780=CARTESIAN_POINT ( 'NONE',  ( -97.30629616937495996, -209.9999999999999716, 87.10281250086714522 ) ) ;
#5783=DIRECTION ( 'NONE',  ( -0.000000000000000000, -0.000000000000000000, 1.000000000000000000 ) ) ;
#5784=CARTESIAN_POINT ( 'NONE',  ( -95.00000000000002842, 86.94004357329504273, 88.96812500173430749 ) ) ;
#5785=B_SPLINE_CURVE_WITH_KNOTS ( 'NONE', 3,
 ( #57282, #6523, #28701, #69299, #17428, #63302, #51996, #52371, #63679, #20387, #19268, #54241, #71501, #7623, #65519, #43342, #37687, #2768, #13991, #37321, #42958, #14375, #24911, #25294 ),
 .UNSPECIFIED., .F., .F.,
 ( 4, 2, 2, 2, 2, 2, 2, 2, 2, 2, 2, 4 ),
 ( -0.009991285189197379041, -0.009254074025163634351, -0.008516862861129889661, -0.007779651697096144104, -0.007411046115079250943, -0.007042440533062358649, -0.006673834951045466354, -0.006305229369028574060, -0.005568018204994787737, -0.004830807040961002281, -0.004462201458944102181, -0.004093595876927202080 ),
 .UNSPECIFIED. ) ;
#5793=CARTESIAN_POINT ( 'NONE',  ( -97.65000000000001990, 88.47002178664754979, 79.25791666666665947 ) ) ;
#5801=VERTEX_POINT ( 'NONE', #12428 ) ;
#5802=CARTESIAN_POINT ( 'NONE',  ( -93.84685191531252713, 88.00268892867056536, 77.15447916753380753 ) ) ;
#5809=CARTESIAN_POINT ( 'NONE',  ( -97.30629616937495996, -209.9999999999999716, 89.16656250086715829 ) ) ;
#5813=CARTESIAN_POINT ( 'NONE',  ( 97.30629616937498838, 90.00000000000002842, 76.78406250086715090 ) ) ;
#5814=CARTESIAN_POINT ( 'NONE',  ( -97.30629616937497417, -211.3315407142195852, 80.96447916753382401 ) ) ;
#5823=CARTESIAN_POINT ( 'NONE',  ( 92.69370383062501162, -211.3315407142195852, 79.53572916753380184 ) ) ;
#5825=CARTESIAN_POINT ( 'NONE',  ( -96.32500000000001705, 92.29496732002878900, 75.28916666666665947 ) ) ;
#5828=CARTESIAN_POINT ( 'NONE',  ( 92.35000000019411459, 89.99998015682159291, 84.36502760998348549 ) ) ;
#5841=CARTESIAN_POINT ( 'NONE',  ( 96.15314808468748708, 88.00268892867053694, 84.29822916753381890 ) ) ;
#5842=CARTESIAN_POINT ( 'NONE',  ( 92.35000000000000853, -209.9999999999999716, 77.29999999999999716 ) ) ;
#5843=ORIENTED_EDGE ( 'NONE', *, *, #67054, .T. ) ;
#5851=LINE ( 'NONE', #12938, #60296 ) ;
#5852=DIRECTION ( 'NONE',  ( -0.000000000000000000, -0.000000000000000000, 1.000000000000000000 ) ) ;
#5853=CARTESIAN_POINT ( 'NONE',  ( 97.64999999999999147, -209.9999999999999716, 87.22187500173430408 ) ) ;
#5859=CARTESIAN_POINT ( 'NONE',  ( -96.32499999999996021, -207.7050326799711968, 83.62354166840097491 ) ) ;
#5863=CARTESIAN_POINT ( 'NONE',  ( 93.67499999999999716, 87.70503267997126784, 79.39020833506762642 ) ) ;
#5864=CARTESIAN_POINT ( 'NONE',  ( -97.65000000000001990, 91.52997821335253548, 77.96145833506763267 ) ) ;
#5867=CARTESIAN_POINT ( 'NONE',  ( 97.30629616937498838, 91.33154071421968467, 81.28197916753381946 ) ) ;
#5873=LINE ( 'NONE', #40433, #3067 ) ;
#5875=DIRECTION ( 'NONE',  ( -0.000000000000000000, -0.000000000000000000, 1.000000000000000000 ) ) ;
#5879=EDGE_CURVE ( 'NONE', #8621, #51903, #2724, .T. ) ;
#5885=CYLINDRICAL_SURFACE ( 'NONE', #38911, 2.649999999999985700 ) ;
#5886=CARTESIAN_POINT ( 'NONE',  ( -92.69370383062498320, -208.6684592857803011, 80.64697916753382856 ) ) ;
#5895=CARTESIAN_POINT ( 'NONE',  ( 97.30629616937498838, 90.00000000000002842, 75.99031250086714806 ) ) ;
#5900=CARTESIAN_POINT ( 'NONE',  ( 7.103376864691351012E-17, -120.0000000000000000, -64.00000000000000000 ) ) ;
#5905=CARTESIAN_POINT ( 'NONE',  ( 96.15314808468748708, 88.00268892867053694, 88.10822916753382117 ) ) ;
#5912=CARTESIAN_POINT ( 'NONE',  ( -97.30629616937501680, 88.66845928578038638, 80.80572916753379786 ) ) ;
#5922=CARTESIAN_POINT ( 'NONE',  ( 96.15314808468748708, -208.0026889286704943, 76.88989583420048746 ) ) ;
#5927=CARTESIAN_POINT ( 'NONE',  ( 95.00000000000000000, -212.6630814284392557, 84.24531250086717193 ) ) ;
#5930=CARTESIAN_POINT ( 'NONE',  ( 97.65000000000003411, 91.52997821335250705, 82.75041666666666629 ) ) ;
#5934=CARTESIAN_POINT ( 'NONE',  ( 92.35000000000002274, -208.4700217866474645, 88.04208333333332348 ) ) ;
#5937=ORIENTED_EDGE ( 'NONE', *, *, #59928, .F. ) ;
#5944=CARTESIAN_POINT ( 'NONE',  ( -92.69370383062502583, 88.66845928578038638, 87.52614583420049144 ) ) ;
#5949=CARTESIAN_POINT ( 'NONE',  ( 95.00000000000000000, -206.9400435732949575, 75.95062500173428077 ) ) ;
#5950=CARTESIAN_POINT ( 'NONE',  ( 92.34999999999999432, 88.47002178664753558, 78.62291666666668277 ) ) ;
#5952=VERTEX_POINT ( 'NONE', #7897 ) ;
#5955=CYLINDRICAL_SURFACE ( 'NONE', #24245, 2.649999999999985700 ) ;
#5958=CARTESIAN_POINT ( 'NONE',  ( -96.15314808468751551, 88.00268892867056536, 81.01739583420049939 ) ) ;
#5959=CARTESIAN_POINT ( 'NONE',  ( 93.84685191531248449, 91.99731107132950569, 74.93197916753379673 ) ) ;
#5962=EDGE_CURVE ( 'NONE', #4841, #69024, #40677, .T. ) ;
#5971=CARTESIAN_POINT ( 'NONE',  ( -96.15314808468747287, -208.0026889286704943, 78.10697916753380809 ) ) ;
#5972=VERTEX_POINT ( 'NONE', #30816 ) ;
#5981=CARTESIAN_POINT ( 'NONE',  ( -97.30629616937497417, -208.6684592857803011, 76.25489583420049655 ) ) ;
#5986=FACE_OUTER_BOUND ( 'NONE', #954, .T. ) ;
#5989=CARTESIAN_POINT ( 'NONE',  ( 97.30629616937498838, 91.33154071421968467, 86.20322916753380582 ) ) ;
#5990=CARTESIAN_POINT ( 'NONE',  ( -96.32499999999996021, -212.2949673200287179, 83.75583333333332803 ) ) ;
#5991=CARTESIAN_POINT ( 'NONE',  ( -96.32500000000001705, 87.70503267997129626, 88.20083333333332121 ) ) ;
#5992=CARTESIAN_POINT ( 'NONE',  ( 96.32499999999998863, -207.7050326799711968, 86.61333333333332973 ) ) ;
#5996=CARTESIAN_POINT ( 'NONE',  ( 92.35000000030107969, -209.9999754409356854, 87.53856274002261273 ) ) ;
#5999=( BOUNDED_CURVE ( )  B_SPLINE_CURVE ( 2, ( #28432, #17164, #67929, #34443, #10783, #40097, #44636 ),
 .UNSPECIFIED., .F., .F. ) 
 B_SPLINE_CURVE_WITH_KNOTS ( ( 3, 2, 2, 3 ),
 ( 0.8466920362409167122, 0.8537476304509593605, 0.8608033959918763856, 0.8678591737257297378 ),
 .UNSPECIFIED. ) 
 CURVE ( )  GEOMETRIC_REPRESENTATION_ITEM ( )  RATIONAL_B_SPLINE_CURVE ( ( 0.9999934937103009958, 0.8660286570082842417, 1.000000000000000000, 0.8660254037844387076, 1.000000000000000000, 0.8660254037844387076, 1.000000000000000000 ) ) 
 REPRESENTATION_ITEM ( '' )  );
#6000=EDGE_CURVE ( 'NONE', #24873, #63128, #57246, .T. ) ;
#6005=CARTESIAN_POINT ( 'NONE',  ( -96.15314808468752972, 91.99731107132950569, 88.26697916753380468 ) ) ;
#6009=( BOUNDED_CURVE ( )  B_SPLINE_CURVE ( 2, ( #66695, #53941, #2479, #36268, #70839, #36632, #43418 ),
 .UNSPECIFIED., .F., .F. ) 
 B_SPLINE_CURVE_WITH_KNOTS ( ( 3, 2, 2, 3 ),
 ( 0.5000000000000000000, 0.5069444444444444198, 0.5138888888888887285, 0.5208333333333332593 ),
 .UNSPECIFIED. ) 
 CURVE ( )  GEOMETRIC_REPRESENTATION_ITEM ( )  RATIONAL_B_SPLINE_CURVE ( ( 1.000000000000000000, 0.8660254037844387076, 1.000000000000000000, 0.8660254037844387076, 1.000000000000000000, 0.8660254037844408170, 0.9999999999999978906 ) ) 
 REPRESENTATION_ITEM ( '' )  );
#6010=CARTESIAN_POINT ( 'NONE',  ( -96.32500000000001705, 92.29496732002878900, 77.19416666666666060 ) ) ;
#6016=AXIS2_PLACEMENT_3D ( 'NONE', #27678, #11131, #4774 ) ;
#6017=CARTESIAN_POINT ( 'NONE',  ( 96.15314808468748708, -208.0026889286704943, 87.04989583420048405 ) ) ;
#6020=ORIENTED_EDGE ( 'NONE', *, *, #7544, .F. ) ;
#6025=CARTESIAN_POINT ( 'NONE',  ( 96.48680242707320076, -208.1953243530631994, 74.81083481226637844 ) ) ;
#6027=CARTESIAN_POINT ( 'NONE',  ( 97.30629616937498838, -208.6684592857803011, 82.55197916753382970 ) ) ;
#6029=VERTEX_POINT ( 'NONE', #66174 ) ;
#6038=CARTESIAN_POINT ( 'NONE',  ( 97.64999999999999147, -209.9999999999999716, 86.58687500173429896 ) ) ;
#6046=EDGE_CURVE ( 'NONE', #32186, #27271, #20016, .T. ) ;
#6049=ORIENTED_EDGE ( 'NONE', *, *, #70578, .T. ) ;
#6052=ORIENTED_EDGE ( 'NONE', *, *, #29797, .F. ) ;
#6053=ORIENTED_EDGE ( 'NONE', *, *, #51264, .T. ) ;
#6055=ORIENTED_EDGE ( 'NONE', *, *, #46328, .F. ) ;
#6058=CARTESIAN_POINT ( 'NONE',  ( -96.32500000000001705, 92.29496732002878900, 86.08416666666666117 ) ) ;
#6060=DIRECTION ( 'NONE',  ( -0.000000000000000000, -0.000000000000000000, 1.000000000000000000 ) ) ;
#6061=VERTEX_POINT ( 'NONE', #21775 ) ;
#6063=CARTESIAN_POINT ( 'NONE',  ( -92.69370383062498320, -208.6684592857803011, 86.83822916753381094 ) ) ;
#6064=EDGE_LOOP ( 'NONE', ( #1293, #7957, #7204, #69285 ) ) ;
#6069=CARTESIAN_POINT ( 'NONE',  ( -97.30629616937497417, -211.3315407142195852, 76.36072916753381890 ) ) ;
#6077=CARTESIAN_POINT ( 'NONE',  ( -96.32500000000001705, 92.29496732002878900, 76.55916666666666970 ) ) ;
#6080=CARTESIAN_POINT ( 'NONE',  ( -97.30629616937501680, 91.33154071421968467, 78.15989583420048348 ) ) ;
#6085=CARTESIAN_POINT ( 'NONE',  ( 94.99999999999998579, 86.94004357329502852, 79.44312500173430180 ) ) ;
#6087=CARTESIAN_POINT ( 'NONE',  ( 97.64999999999999147, -210.0000001051138270, 86.58687499784845443 ) ) ;
#6090=CARTESIAN_POINT ( 'NONE',  ( -92.35000000000005116, 91.52997821335253548, 85.36979166840096411 ) ) ;
#6091=CARTESIAN_POINT ( 'NONE',  ( -94.99999999999997158, -207.3369185715606307, 75.67281250086716682 ) ) ;
#6092=CYLINDRICAL_SURFACE ( 'NONE', #6844, 2.649999999999985700 ) ;
#6095=CARTESIAN_POINT ( 'NONE',  ( -97.64999999990727986, 90.00001381026693537, 80.55392363656929433 ) ) ;
#6106=CARTESIAN_POINT ( 'NONE',  ( 95.00000000000000000, -207.3369185715606307, 88.84906250086713442 ) ) ;
#6120=DIRECTION ( 'NONE',  ( -0.000000000000000000, -0.000000000000000000, 1.000000000000000000 ) ) ;
#6127=ORIENTED_EDGE ( 'NONE', *, *, #14016, .F. ) ;
#6128=CARTESIAN_POINT ( 'NONE',  ( 92.48632958231164025, 89.99999999999990052, 74.91808492278045151 ) ) ;
#6132=CARTESIAN_POINT ( 'NONE',  ( 92.69370383062498320, 90.00000000000002842, 83.92781250086714806 ) ) ;
#6134=CARTESIAN_POINT ( 'NONE',  ( 93.84685191531249870, -208.0026889286704943, 83.18697916753382060 ) ) ;
#6136=CARTESIAN_POINT ( 'NONE',  ( -92.35000000000547971, -210.0000054026037049, 81.50687481489497088 ) ) ;
#6137=CARTESIAN_POINT ( 'NONE',  ( -97.65000000000001990, 90.00000000000004263, 84.28499999999999659 ) ) ;
#6142=CARTESIAN_POINT ( 'NONE',  ( -93.84685191531247028, -211.9973110713294489, 84.77447916753381207 ) ) ;
#6143=CARTESIAN_POINT ( 'NONE',  ( -92.69370383062502583, 91.33154071421968467, 83.18697916753382060 ) ) ;
#6146=CARTESIAN_POINT ( 'NONE',  ( 92.69370383062498320, 91.33154071421968467, 83.23989583420046756 ) ) ;
#6147=CARTESIAN_POINT ( 'NONE',  ( -97.30629616937501680, 88.66845928578038638, 83.98072916753380923 ) ) ;
#6150=CARTESIAN_POINT ( 'NONE',  ( 92.35000000000000853, -209.9999999999999716, 79.20499999999999829 ) ) ;
#6153=DIRECTION ( 'NONE',  ( 1.000000000000000000, 0.000000000000000000, 0.000000000000000000 ) ) ;
#6154=CARTESIAN_POINT ( 'NONE',  ( -97.30629616937495996, -209.9999999999999716, 87.73781250086713612 ) ) ;
#6158=CARTESIAN_POINT ( 'NONE',  ( -94.99999999999997158, -209.9999999999999716, 90.00000000000000000 ) ) ;
#6165=CARTESIAN_POINT ( 'NONE',  ( -92.35000000000005116, 91.52997821335253548, 79.57541666666665492 ) ) ;
#6166=CARTESIAN_POINT ( 'NONE',  ( 93.67500000000001137, -212.2949673200287179, 88.83583333333334053 ) ) ;
#6169=CARTESIAN_POINT ( 'NONE',  ( 93.67499999999998295, 92.29496732002878900, 76.55916666666666970 ) ) ;
#6171=CARTESIAN_POINT ( 'NONE',  ( -2.500000000000015543, -73.00000000000001421, -204.9999999999999716 ) ) ;
#6172=ORIENTED_EDGE ( 'NONE', *, *, #4168, .F. ) ;
#6173=CARTESIAN_POINT ( 'NONE',  ( -92.69370383062502583, 91.33154071421968467, 77.94822916753381037 ) ) ;
#6182=CARTESIAN_POINT ( 'NONE',  ( -97.30629616937497417, -211.3315407142195852, 86.04447916753382231 ) ) ;
#6184=CARTESIAN_POINT ( 'NONE',  ( 96.15314808468748708, 91.99731107132950569, 76.25489583420049655 ) ) ;
#6185=CARTESIAN_POINT ( 'NONE',  ( -96.15314808468745866, -211.9973110713294489, 79.11239583420048405 ) ) ;
#6186=CARTESIAN_POINT ( 'NONE',  ( -97.64998927049497013, 91.52998440803517610, 84.94645790656221607 ) ) ;
#6188=CARTESIAN_POINT ( 'NONE',  ( 92.34999999999998010, 90.00002803130637119, 87.53937403222812463 ) ) ;
#6191=CARTESIAN_POINT ( 'NONE',  ( -97.30629616937501680, 88.66845928578038638, 75.88447916753382572 ) ) ;
#6192=CARTESIAN_POINT ( 'NONE',  ( 92.69370383062501162, -208.6684592857803011, 77.52489583420046415 ) ) ;
#6209=CARTESIAN_POINT ( 'NONE',  ( 92.35002740377132113, -208.4700059650727155, 79.86645724064028684 ) ) ;
#6213=( BOUNDED_CURVE ( )  B_SPLINE_CURVE ( 2, ( #33639, #73481, #56955, #5464, #44935, #67857, #69331, #40390, #68972 ),
 .UNSPECIFIED., .F., .F. ) 
 B_SPLINE_CURVE_WITH_KNOTS ( ( 3, 2, 2, 2, 3 ),
 ( 0.08466915177933910519, 0.08466918649100467487, 0.09172495203192151947, 0.09878071757283837795, 0.1058364832028025337 ),
 .UNSPECIFIED. ) 
 CURVE ( )  GEOMETRIC_REPRESENTATION_ITEM ( )  RATIONAL_B_SPLINE_CURVE ( ( 0.9999986817990271781, 0.9999993408962710717, 1.000000000000000000, 0.8660254037844387076, 1.000000000000000000, 0.8660254037844387076, 1.000000000000000000, 0.8660254037844387076, 1.000000000000000000 ) ) 
 REPRESENTATION_ITEM ( '' )  );
#6214=CARTESIAN_POINT ( 'NONE',  ( 92.69370383062498320, 90.00000000000002842, 82.18156250086715886 ) ) ;
#6215=CARTESIAN_POINT ( 'NONE',  ( 93.67500000000001137, -212.2949673200287179, 75.50083333333331836 ) ) ;
#6223=CARTESIAN_POINT ( 'NONE',  ( -96.32500000000001705, 87.70503267997129626, 87.56583333333333030 ) ) ;
#6224=CARTESIAN_POINT ( 'NONE',  ( 15.69955575014744831, 0.001194404164628767254, -90.00000000000000000 ) ) ;
#6230=CARTESIAN_POINT ( 'NONE',  ( 97.64999999999999147, 89.99999997442942856, 84.04687500080852658 ) ) ;
#6232=CARTESIAN_POINT ( 'NONE',  ( -97.64999999999994884, -211.5299782133524502, 80.60729166840097548 ) ) ;
#6235=EDGE_LOOP ( 'NONE', ( #48527, #66152, #48103, #64168 ) ) ;
#6236=CARTESIAN_POINT ( 'NONE',  ( 94.99999999999998579, 86.94004357329500010, 78.80812500173429669 ) ) ;
#6237=CARTESIAN_POINT ( 'NONE',  ( -97.65000000000001990, 88.47002178664754979, 79.97229166840095615 ) ) ;
#6239=CARTESIAN_POINT ( 'NONE',  ( 92.69370383062498320, 91.33154071421968467, 81.49364583420047836 ) ) ;
#6240=CARTESIAN_POINT ( 'NONE',  ( -92.34999999999999432, -209.9999999999999716, 80.79249999999998977 ) ) ;
#6245=CARTESIAN_POINT ( 'NONE',  ( -92.35000000000000853, 91.52997821335252127, 80.21041666666666003 ) ) ;
#6251=EDGE_LOOP ( 'NONE', ( #47646, #57508, #45544, #63264, #49651, #8413, #41828, #63640, #58565, #38533, #35267, #71307, #3161, #46051, #61590, #59356, #50128, #31007, #69791, #24334, #20566, #25496, #16925, #36521, #71280, #2627, #39672, #33216, #55725, #23896, #71919, #31164, #40056, #24597, #73407, #48906, #62536, #69634, #15059, #61128, #54822, #55603, #73999, #70879, #50272, #23849, #48908, #2259, #4788, #72488 ) ) ;
#6254=CARTESIAN_POINT ( 'NONE',  ( -94.99999999999997158, -206.9400435732949575, 75.87125000000000341 ) ) ;
#6255=CARTESIAN_POINT ( 'NONE',  ( -97.30629616937495996, -209.9999999999999716, 76.46656250086715545 ) ) ;
#6263=CARTESIAN_POINT ( 'NONE',  ( 92.69370383062498320, 88.66845928578035796, 75.09072916753380866 ) ) ;
#6271=CARTESIAN_POINT ( 'NONE',  ( 96.15314808468748708, 91.99731107132950569, 85.77989583420048803 ) ) ;
#6273=CARTESIAN_POINT ( 'NONE',  ( -96.32499999999996021, -212.2949673200287179, 75.58020833506763836 ) ) ;
#6275=CARTESIAN_POINT ( 'NONE',  ( 97.64999999999999147, -209.9999884513868551, 83.41187540116096955 ) ) ;
#6276=CARTESIAN_POINT ( 'NONE',  ( -97.30629616937501680, 88.66845928578038638, 80.17072916753380696 ) ) ;
#6279=CARTESIAN_POINT ( 'NONE',  ( 92.69370383062501162, -211.3315407142195852, 86.52072916753381548 ) ) ;
#6281=CARTESIAN_POINT ( 'NONE',  ( 97.64999999999999147, -210.0000000983658026, 80.23687499810812085 ) ) ;
#6286=CARTESIAN_POINT ( 'NONE',  ( -0.0004442498525516064278, 0.001194404164626844313, -85.59999999999999432 ) ) ;
#6292=CARTESIAN_POINT ( 'NONE',  ( 95.00000000000000000, -207.3369185715606307, 80.11781250086714579 ) ) ;
#6299=CARTESIAN_POINT ( 'NONE',  ( 95.00000000000000000, -206.9400435732949575, 84.76125000000000398 ) ) ;
#6307=CARTESIAN_POINT ( 'NONE',  ( -95.00000000000002842, 92.66308142843932671, 85.83281250086714920 ) ) ;
#6309=LINE ( 'NONE', #29571, #17346 ) ;
#6310=CARTESIAN_POINT ( 'NONE',  ( 97.64999999999999147, -209.9999999999999716, 78.33187500173430351 ) ) ;
#6311=CARTESIAN_POINT ( 'NONE',  ( 93.67499999999999716, 87.70503267997126784, 79.94583333333332575 ) ) ;
#6320=CARTESIAN_POINT ( 'NONE',  ( 92.35000000001612364, -210.0000060634596082, 88.17456390440206349 ) ) ;
#6321=CARTESIAN_POINT ( 'NONE',  ( -92.69370383062505425, 91.33154071421968467, 80.01197916753382344 ) ) ;
#6322=CARTESIAN_POINT ( 'NONE',  ( 97.30629616937498838, 88.66845928578037217, 75.93739583420047268 ) ) ;
#6334=CARTESIAN_POINT ( 'NONE',  ( -96.15314808468745866, -211.9973110713294489, 77.68364583420047609 ) ) ;
#6340=CARTESIAN_POINT ( 'NONE',  ( 96.32499999999998863, 87.70503267997126784, 80.68666666666665321 ) ) ;
#6342=CARTESIAN_POINT ( 'NONE',  ( -97.30629616937495996, -209.9999999999999716, 87.89656250086714806 ) ) ;
#6344=CARTESIAN_POINT ( 'NONE',  ( 97.64999999999999147, 89.99999149135229004, 88.49187470744952577 ) ) ;
#6350=CARTESIAN_POINT ( 'NONE',  ( 93.84685191531248449, 88.00268892867053694, 84.66864583420047552 ) ) ;
#6352=CARTESIAN_POINT ( 'NONE',  ( -96.32500000000001705, 87.70503267997129626, 75.50083333333331836 ) ) ;
#6360=CARTESIAN_POINT ( 'NONE',  ( -23.50000000000000355, -120.0000000000000000, -64.00000000000000000 ) ) ;
#6371=DIRECTION ( 'NONE',  ( -0.000000000000000000, -0.000000000000000000, 1.000000000000000000 ) ) ;
#6377=CARTESIAN_POINT ( 'NONE',  ( 95.00000000000000000, -207.3369185715606307, 84.56281250086716739 ) ) ;
#6381=CARTESIAN_POINT ( 'NONE',  ( -92.34999999999999432, -209.9999999999999716, 85.87249999999998806 ) ) ;
#6382=ORIENTED_EDGE ( 'NONE', *, *, #54498, .F. ) ;
#6387=CARTESIAN_POINT ( 'NONE',  ( 97.30629616937498838, -211.3315407142195852, 84.35114583420049428 ) ) ;
#6389=CARTESIAN_POINT ( 'NONE',  ( 94.99999999999998579, 93.05995642670504253, 80.39562500173430237 ) ) ;
#6396=CARTESIAN_POINT ( 'NONE',  ( 96.32499999999998863, -207.7050326799711968, 86.69270833506763552 ) ) ;
#6402=VERTEX_POINT ( 'NONE', #47307 ) ;
#6405=CARTESIAN_POINT ( 'NONE',  ( 97.64999999999997726, 88.47002178664753558, 87.16895833506762870 ) ) ;
#6418=CARTESIAN_POINT ( 'NONE',  ( -92.35000000000003695, 90.00000000000004263, 87.14249999999999829 ) ) ;
#6420=CARTESIAN_POINT ( 'NONE',  ( 92.35000000000000853, -209.9999999999999716, 90.00000000000000000 ) ) ;
#6421=AXIS2_PLACEMENT_3D ( 'NONE', #34852, #681, #7396 ) ;
#6422=( BOUNDED_CURVE ( )  B_SPLINE_CURVE ( 2, ( #49550, #48810, #7852, #71728, #37549, #54826, #42079 ),
 .UNSPECIFIED., .F., .F. ) 
 B_SPLINE_CURVE_WITH_KNOTS ( ( 3, 2, 2, 3 ),
 ( 0.4656806970079900854, 0.4727362912414405649, 0.4797920567823575899, 0.4868478063952913493 ),
 .UNSPECIFIED. ) 
 CURVE ( )  GEOMETRIC_REPRESENTATION_ITEM ( )  RATIONAL_B_SPLINE_CURVE ( ( 0.9999934945991874047, 0.8660286565638194434, 1.000000000000000000, 0.8660254037844387076, 1.000000000000000000, 0.8660254037844387076, 1.000000000000000000 ) ) 
 REPRESENTATION_ITEM ( '' )  );
#6425=CARTESIAN_POINT ( 'NONE',  ( -97.30629616937497417, -208.6684592857803011, 85.77989583420048803 ) ) ;
#6428=CARTESIAN_POINT ( 'NONE',  ( -92.34999999999999432, -209.9999998456625860, 79.60187500750915035 ) ) ;
#6431=CARTESIAN_POINT ( 'NONE',  ( -94.99999999999997158, -212.6630814284392557, 76.46656250086712703 ) ) ;
#6439=CARTESIAN_POINT ( 'NONE',  ( -96.15314808468751551, 88.00268892867056536, 77.04864583420047097 ) ) ;
#6442=ORIENTED_EDGE ( 'NONE', *, *, #47596, .T. ) ;
#6449=CARTESIAN_POINT ( 'NONE',  ( -96.15314808468747287, -208.0026889286704943, 77.63072916753381492 ) ) ;
#6453=VECTOR ( 'NONE', #18628, 1000.000000000000000 ) ;
#6461=EDGE_CURVE ( 'NONE', #20380, #39507, #68579, .T. ) ;
#6468=CARTESIAN_POINT ( 'NONE',  ( 97.30629616937498838, -211.3315407142195852, 83.55739583420047722 ) ) ;
#6469=CARTESIAN_POINT ( 'NONE',  ( -2.500000000000015543, -73.00000000000001421, -251.7000000000000455 ) ) ;
#6479=CARTESIAN_POINT ( 'NONE',  ( -92.69370383062502583, 91.33154071421968467, 79.37697916753381833 ) ) ;
#6482=ORIENTED_EDGE ( 'NONE', *, *, #73234, .F. ) ;
#6483=CYLINDRICAL_SURFACE ( 'NONE', #11599, 2.649999999999985700 ) ;
#6489=CARTESIAN_POINT ( 'NONE',  ( 92.55058773059860755, 89.32071446497070610, 74.93153462041256319 ) ) ;
#6491=ORIENTED_EDGE ( 'NONE', *, *, #35957, .F. ) ;
#6495=CARTESIAN_POINT ( 'NONE',  ( 95.00000000000000000, -207.3369185715606307, 82.49906250086714010 ) ) ;
#6497=CARTESIAN_POINT ( 'NONE',  ( -92.35000000000003695, 90.00000000000004263, 84.60249999999999204 ) ) ;
#6499=CARTESIAN_POINT ( 'NONE',  ( -92.35000000000005116, -208.4700217866474361, 89.10041666666667481 ) ) ;
#6501=LINE ( 'NONE', #12124, #45536 ) ;
#6502=CARTESIAN_POINT ( 'NONE',  ( -92.69370383062498320, -211.3315407142195852, 83.55739583420047722 ) ) ;
#6503=CARTESIAN_POINT ( 'NONE',  ( -97.30629616937501680, 88.66845928578038638, 82.86947916753382515 ) ) ;
#6506=CARTESIAN_POINT ( 'NONE',  ( 93.84685191531248449, 88.00268892867053694, 84.03364583420047040 ) ) ;
#6509=CARTESIAN_POINT ( 'NONE',  ( 92.35000000000000853, -209.9999999999999716, 76.10937500173430692 ) ) ;
#6511=CARTESIAN_POINT ( 'NONE',  ( 92.35000000000000853, -209.9999999999999716, 90.00000000000000000 ) ) ;
#6512=CARTESIAN_POINT ( 'NONE',  ( -92.69370383062498320, -208.6684592857803295, 87.47322916753380184 ) ) ;
#6520=CARTESIAN_POINT ( 'NONE',  ( -97.65000000000001990, 88.47002178664754979, 76.71791666666666742 ) ) ;
#6522=CARTESIAN_POINT ( 'NONE',  ( -96.15314808468751551, 88.00268892867056536, 87.20864583420046756 ) ) ;
#6523=CARTESIAN_POINT ( 'NONE',  ( -93.41453557521617768, -208.2943803060621519, 74.79912739178799086 ) ) ;
#6524=CARTESIAN_POINT ( 'NONE',  ( 94.99999999999998579, 93.05995642670504253, 76.50624999999999432 ) ) ;
#6531=CARTESIAN_POINT ( 'NONE',  ( -96.15314808468752972, 91.99731107132950569, 76.83697916753381207 ) ) ;
#6538=CARTESIAN_POINT ( 'NONE',  ( -94.99999999999997158, -212.6630814284392557, 85.51531250086713953 ) ) ;
#6542=CARTESIAN_POINT ( 'NONE',  ( 97.30629616937498838, 90.00000000000002842, 75.51406250086715488 ) ) ;
#6544=CARTESIAN_POINT ( 'NONE',  ( -93.84685191531248449, -208.0026889286704943, 75.61989583420049144 ) ) ;
#6552=CARTESIAN_POINT ( 'NONE',  ( 96.15314808468748708, -208.0026889286704943, 77.36614583420046642 ) ) ;
#6566=EDGE_LOOP ( 'NONE', ( #35494, #23077, #26561, #32988 ) ) ;
#6567=CARTESIAN_POINT ( 'NONE',  ( 93.67500000000001137, -207.7050326799711968, 79.81354166840095843 ) ) ;
#6571=CARTESIAN_POINT ( 'NONE',  ( 96.15314808468748708, 88.00268892867053694, 83.66322916753382799 ) ) ;
#6583=CARTESIAN_POINT ( 'NONE',  ( 93.67499999999998295, 92.29496732002878900, 84.17916666666666003 ) ) ;
#6586=CARTESIAN_POINT ( 'NONE',  ( 92.35000000000000853, -211.5299782133524218, 86.95729166840096980 ) ) ;
#6590=CARTESIAN_POINT ( 'NONE',  ( -93.67499999999998295, -207.7050326799711968, 78.43770833506764006 ) ) ;
#6593=AXIS2_PLACEMENT_3D ( 'NONE', #21543, #67419, #26815 ) ;
#6595=CARTESIAN_POINT ( 'NONE',  ( 93.67499999999998295, 92.29496732002878900, 77.90854166840097150 ) ) ;
#6596=CARTESIAN_POINT ( 'NONE',  ( -93.67500000000003979, 92.29496732002878900, 78.43770833506764006 ) ) ;
#6598=CARTESIAN_POINT ( 'NONE',  ( 94.99999999999998579, 87.33691857156068750, 78.53031250086715431 ) ) ;
#6599=PLANE ( 'NONE',  #40966 ) ;
#6605=ORIENTED_EDGE ( 'NONE', *, *, #31892, .F. ) ;
#6610=CARTESIAN_POINT ( 'NONE',  ( -92.69370383062498320, -209.9999999999999716, 79.32406250086715715 ) ) ;
#6614=CARTESIAN_POINT ( 'NONE',  ( -97.01659045496313638, -211.6055158133294469, 74.95309847082374688 ) ) ;
#6620=FACE_OUTER_BOUND ( 'NONE', #46634, .T. ) ;
#6621=CYLINDRICAL_SURFACE ( 'NONE', #18433, 2.649999999999999467 ) ;
#6627=CARTESIAN_POINT ( 'NONE',  ( 97.30629616937498838, 91.33154071421968467, 88.26697916753381890 ) ) ;
#6628=CARTESIAN_POINT ( 'NONE',  ( -96.15314808468747287, -208.0026889286704943, 85.88572916753381037 ) ) ;
#6631=CARTESIAN_POINT ( 'NONE',  ( -92.69370383062505425, 91.33154071421968467, 77.31322916753380525 ) ) ;
#6634=CARTESIAN_POINT ( 'NONE',  ( 96.15314808468750130, -211.9973110713294489, 88.58447916753381435 ) ) ;
#6636=( BOUNDED_CURVE ( )  B_SPLINE_CURVE ( 2, ( #17610, #11962, #13349, #36279, #71963, #20091, #48675, #26103, #14078 ),
 .UNSPECIFIED., .F., .F. ) 
 B_SPLINE_CURVE_WITH_KNOTS ( ( 3, 2, 2, 2, 3 ),
 ( 0.2116728463006670724, 0.2116729662264710543, 0.2187287317673534404, 0.2257844973082357709, 0.2328402629019979686 ),
 .UNSPECIFIED. ) 
 CURVE ( )  GEOMETRIC_REPRESENTATION_ITEM ( )  RATIONAL_B_SPLINE_CURVE ( ( 0.9999954457845905420, 0.9999977228535908980, 1.000000000000000000, 0.8660254037844387076, 1.000000000000000000, 0.8660254037844387076, 1.000000000000000000, 0.8660254037844387076, 1.000000000000000000 ) ) 
 REPRESENTATION_ITEM ( '' )  );
#6647=CARTESIAN_POINT ( 'NONE',  ( 95.00000000000000000, -207.3369185715606307, 82.02281250086714692 ) ) ;
#6654=DIRECTION ( 'NONE',  ( -0.000000000000000000, -0.000000000000000000, 1.000000000000000000 ) ) ;
#6655=CARTESIAN_POINT ( 'NONE',  ( 92.35000000000000853, -209.9999999999999716, 83.65000000000000568 ) ) ;
#6656=EDGE_LOOP ( 'NONE', ( #66016, #59299, #19386, #34193 ) ) ;
#6657=EDGE_LOOP ( 'NONE', ( #60966, #45718, #50373, #12816 ) ) ;
#6663=CARTESIAN_POINT ( 'NONE',  ( -93.84685191531252713, 88.00268892867056536, 87.47322916753381605 ) ) ;
#6665=CYLINDRICAL_SURFACE ( 'NONE', #12611, 2.649999999999985700 ) ;
#6666=CARTESIAN_POINT ( 'NONE',  ( 93.67500000000001137, -207.7050326799711968, 77.90854166840097150 ) ) ;
#6667=CARTESIAN_POINT ( 'NONE',  ( 94.99999999999998579, 86.94004357329500010, 77.45874999999999488 ) ) ;
#6669=CARTESIAN_POINT ( 'NONE',  ( -96.32499999999996021, -212.2949673200287179, 88.91520833506763211 ) ) ;
#6673=DIRECTION ( 'NONE',  ( -0.000000000000000000, -0.000000000000000000, 1.000000000000000000 ) ) ;
#6674=CARTESIAN_POINT ( 'NONE',  ( -96.15314808468751551, 88.00268892867056536, 82.28739583420048120 ) ) ;
#6675=CARTESIAN_POINT ( 'NONE',  ( 97.30629616937498838, 91.33154071421968467, 74.77322916753379900 ) ) ;
#6676=VECTOR ( 'NONE', #3201, 1000.000000000000000 ) ;
#6681=CARTESIAN_POINT ( 'NONE',  ( -97.64999999999996305, -208.4700217866474645, 86.21645833506764234 ) ) ;
#6682=VERTEX_POINT ( 'NONE', #61925 ) ;
#6687=VERTEX_POINT ( 'NONE', #4800 ) ;
#6696=CARTESIAN_POINT ( 'NONE',  ( -92.69370383062498320, -209.9999999999999716, 87.57906250086715261 ) ) ;
#6700=VERTEX_POINT ( 'NONE', #67930 ) ;
#6702=CARTESIAN_POINT ( 'NONE',  ( -96.32500000000001705, 92.29496732002878900, 83.62354166840097491 ) ) ;
#6706=CARTESIAN_POINT ( 'NONE',  ( 97.30629616937498838, 90.00000000000002842, 82.34031250086714238 ) ) ;
#6708=CARTESIAN_POINT ( 'NONE',  ( -93.67500000000003979, 92.29496732002878900, 80.34270833506762699 ) ) ;
#6709=CARTESIAN_POINT ( 'NONE',  ( -99.99999999999997158, -214.9999999999999716, 90.00000000000000000 ) ) ;
#6718=CARTESIAN_POINT ( 'NONE',  ( -92.69370383062505425, 88.66845928578038638, 89.27239583420048064 ) ) ;
#6722=EDGE_CURVE ( 'NONE', #48440, #44941, #29532, .T. ) ;
#6723=VERTEX_POINT ( 'NONE', #28433 ) ;
#6725=CARTESIAN_POINT ( 'NONE',  ( 92.35000000000003695, 91.52997821335253548, 85.50208333333331723 ) ) ;
#6730=CIRCLE ( 'NONE', #18576, 26.50000000000000355 ) ;
#6733=CARTESIAN_POINT ( 'NONE',  ( 97.30629616937498838, -211.3315407142195852, 81.17614583420048291 ) ) ;
#6734=ORIENTED_EDGE ( 'NONE', *, *, #46028, .T. ) ;
#6739=AXIS2_PLACEMENT_3D ( 'NONE', #10957, #3849, #28233 ) ;
#6742=CARTESIAN_POINT ( 'NONE',  ( 95.00000000000000000, -207.3369185715606307, 75.51406250086714067 ) ) ;
#6744=CARTESIAN_POINT ( 'NONE',  ( 92.69370383062501162, -211.3315407142195852, 78.42447916753380355 ) ) ;
#6753=CARTESIAN_POINT ( 'NONE',  ( 97.64999999999997726, -211.5299782133524502, 85.89895833506764689 ) ) ;
#6754=CARTESIAN_POINT ( 'NONE',  ( 94.99999999999998579, 86.94004357329500010, 88.25374999999999659 ) ) ;
#6760=ORIENTED_EDGE ( 'NONE', *, *, #52004, .F. ) ;
#6761=CARTESIAN_POINT ( 'NONE',  ( 97.64999999999997726, 88.47002178664753558, 85.26395833506762756 ) ) ;
#6762=ORIENTED_EDGE ( 'NONE', *, *, #44931, .F. ) ;
#6763=ORIENTED_EDGE ( 'NONE', *, *, #46124, .T. ) ;
#6764=LINE ( 'NONE', #46253, #50066 ) ;
#6767=ORIENTED_EDGE ( 'NONE', *, *, #11183, .F. ) ;
#6772=CARTESIAN_POINT ( 'NONE',  ( -92.35000000000005116, 88.47002178664754979, 88.99458333333333826 ) ) ;
#6777=CARTESIAN_POINT ( 'NONE',  ( -92.69370383062498320, -211.3315407142195852, 81.65239583420049030 ) ) ;
#6778=ORIENTED_EDGE ( 'NONE', *, *, #59612, .T. ) ;
#6780=AXIS2_PLACEMENT_3D ( 'NONE', #73711, #9824, #22223 ) ;
#6782=CARTESIAN_POINT ( 'NONE',  ( 92.34999999999999432, 91.52997821335252127, 89.39145833506763950 ) ) ;
#6783=CARTESIAN_POINT ( 'NONE',  ( -94.99999999999997158, -207.3369185715606307, 77.41906250086714181 ) ) ;
#6785=EDGE_CURVE ( 'NONE', #28639, #34509, #17165, .T. ) ;
#6794=CARTESIAN_POINT ( 'NONE',  ( -92.69370383062502583, 91.33154071421968467, 77.31322916753380525 ) ) ;
#6801=DIRECTION ( 'NONE',  ( 1.000000000000000000, 0.000000000000000000, 0.000000000000000000 ) ) ;
#6806=CARTESIAN_POINT ( 'NONE',  ( -92.69370383062498320, -209.9999999999999716, 76.14906250086716000 ) ) ;
#6809=EDGE_CURVE ( 'NONE', #10929, #31307, #10786, .T. ) ;
#6813=LINE ( 'NONE', #1227, #65845 ) ;
#6815=AXIS2_PLACEMENT_3D ( 'NONE', #29220, #40150, #62736 ) ;
#6821=CARTESIAN_POINT ( 'NONE',  ( 97.30629616937498838, -211.3315407142195852, 86.73239583420047438 ) ) ;
#6825=CARTESIAN_POINT ( 'NONE',  ( 97.30629616937498838, -208.6684592857803011, 89.53697916753382913 ) ) ;
#6830=CARTESIAN_POINT ( 'NONE',  ( -96.15314808468751551, 88.00268892867056536, 80.38239583420048007 ) ) ;
#6831=ORIENTED_EDGE ( 'NONE', *, *, #16640, .T. ) ;
#6838=CARTESIAN_POINT ( 'NONE',  ( 97.64999999999999147, -209.9999999999999716, 79.52249999999999375 ) ) ;
#6844=AXIS2_PLACEMENT_3D ( 'NONE', #62874, #57949, #45574 ) ;
#6846=( BOUNDED_CURVE ( )  B_SPLINE_CURVE ( 2, ( #34877, #39782, #33368, #39406, #39033, #22488, #28111, #34493, #10835 ),
 .UNSPECIFIED., .F., .F. ) 
 B_SPLINE_CURVE_WITH_KNOTS ( ( 3, 2, 2, 2, 3 ),
 ( 0.9313609857393206903, 0.9313610513964741822, 0.9384168169373561241, 0.9454725824782379551, 0.9525283480321509177 ),
 .UNSPECIFIED. ) 
 CURVE ( )  GEOMETRIC_REPRESENTATION_ITEM ( )  RATIONAL_B_SPLINE_CURVE ( ( 0.9999975066323494310, 0.9999987533045736621, 1.000000000000000000, 0.8660254037844387076, 1.000000000000000000, 0.8660254037844387076, 1.000000000000000000, 0.8660254037844387076, 1.000000000000000000 ) ) 
 REPRESENTATION_ITEM ( '' )  );
#6847=CARTESIAN_POINT ( 'NONE',  ( 97.64999999999999147, -210.0000000207152198, 80.87187500099602744 ) ) ;
#6848=EDGE_LOOP ( 'NONE', ( #34742, #64084, #4073, #36549 ) ) ;
#6851=CARTESIAN_POINT ( 'NONE',  ( 95.00000000000000000, -212.6630814284392557, 80.91156250086714863 ) ) ;
#6853=CARTESIAN_POINT ( 'NONE',  ( -92.34999999999999432, -211.5299782133524218, 81.45395833506763950 ) ) ;
#6856=CARTESIAN_POINT ( 'NONE',  ( 92.34999999999999432, 90.00000000000002842, 84.92000000000000171 ) ) ;
#6858=EDGE_CURVE ( 'NONE', #16851, #32740, #40098, .T. ) ;
#6860=DIRECTION ( 'NONE',  ( -1.000000000000000000, 0.000000000000000000, 0.000000000000000000 ) ) ;
#6861=CARTESIAN_POINT ( 'NONE',  ( -97.30629616937495996, -209.9999999999999716, 84.56281250086713897 ) ) ;
#6863=CARTESIAN_POINT ( 'NONE',  ( -96.15314808468751551, 88.00268892867056536, 81.65239583420049030 ) ) ;
#6864=ORIENTED_EDGE ( 'NONE', *, *, #31795, .F. ) ;
#6865=CARTESIAN_POINT ( 'NONE',  ( 92.69370383062498320, 91.33154071421968467, 83.87489583420047268 ) ) ;
#6872=CARTESIAN_POINT ( 'NONE',  ( -92.69370383062498320, -211.3315407142195852, 85.46239583420044994 ) ) ;
#6880=CARTESIAN_POINT ( 'NONE',  ( -92.35000000000003695, 90.00000000000004263, 77.61749999999999261 ) ) ;
#6889=CARTESIAN_POINT ( 'NONE',  ( -92.69370383062502583, 88.66845928578038638, 75.93739583420047268 ) ) ;
#6893=CARTESIAN_POINT ( 'NONE',  ( 12.74955575014744547, 0.001194404164628405998, 127.4927882439603195 ) ) ;
#6897=CARTESIAN_POINT ( 'NONE',  ( -97.30629616937497417, -208.6684592857803011, 84.66864583420047552 ) ) ;
#6899=ADVANCED_FACE ( 'NONE', ( #1761 ), #59237, .F. ) ;
#6903=CARTESIAN_POINT ( 'NONE',  ( 96.15314808468748708, 88.00268892867053694, 78.58322916753382970 ) ) ;
#6904=CARTESIAN_POINT ( 'NONE',  ( -92.69370383062498320, -209.9999999999999716, 75.51406250086715488 ) ) ;
#6905=CARTESIAN_POINT ( 'NONE',  ( 97.64999999999999147, 90.00000000000002842, 88.41249999999999432 ) ) ;
#6906=EDGE_LOOP ( 'NONE', ( #63747, #29710, #40514, #15687 ) ) ;
#6908=CYLINDRICAL_SURFACE ( 'NONE', #32267, 2.649999999999985700 ) ;
#6910=CARTESIAN_POINT ( 'NONE',  ( -95.00000000000002842, 92.66308142843932671, 75.67281250086715261 ) ) ;
#6911=CARTESIAN_POINT ( 'NONE',  ( 92.69370383062501162, -211.3315407142195852, 77.63072916753380071 ) ) ;
#6924=CARTESIAN_POINT ( 'NONE',  ( 97.30629616937498838, 91.33154071421968467, 81.91697916753381037 ) ) ;
#6931=VERTEX_POINT ( 'NONE', #41567 ) ;
#6939=CARTESIAN_POINT ( 'NONE',  ( 92.35000000000000853, -209.9999999999999716, 82.45937500173430124 ) ) ;
#6940=EDGE_CURVE ( 'NONE', #39621, #7767, #66587, .T. ) ;
#6943=CARTESIAN_POINT ( 'NONE',  ( -92.34999999999999432, -208.4700217866474645, 79.01979166840095559 ) ) ;
#6945=EDGE_CURVE ( 'NONE', #27925, #50886, #4692, .T. ) ;
#6948=CARTESIAN_POINT ( 'NONE',  ( 92.34999999999999432, 90.00000000000002842, 80.55437500173430010 ) ) ;
#6949=CARTESIAN_POINT ( 'NONE',  ( -97.65000000000001990, 91.52997821335253548, 76.05645833506761733 ) ) ;
#6951=CARTESIAN_POINT ( 'NONE',  ( 97.30629616937498838, 90.00000000000002842, 80.59406250086715318 ) ) ;
#6954=DIRECTION ( 'NONE',  ( -0.000000000000000000, -0.000000000000000000, 1.000000000000000000 ) ) ;
#6970=CARTESIAN_POINT ( 'NONE',  ( -92.69370383062498320, -211.3315407142195852, 79.27114583420048177 ) ) ;
#6975=CARTESIAN_POINT ( 'NONE',  ( 97.64999999999999147, 90.00000000000002842, 82.06250000000000000 ) ) ;
#6978=CARTESIAN_POINT ( 'NONE',  ( -26.50000000000000355, -120.0000000000000000, -64.00000000000000000 ) ) ;
#6981=CARTESIAN_POINT ( 'NONE',  ( -92.34999999999993747, -211.5299782133523934, 76.29458333333333542 ) ) ;
#6983=EDGE_CURVE ( 'NONE', #64759, #64357, #35556, .T. ) ;
#6986=CARTESIAN_POINT ( 'NONE',  ( 92.69370383062498320, 91.33154071421968467, 87.84364583420048689 ) ) ;
#6988=CARTESIAN_POINT ( 'NONE',  ( -94.99999999999997158, -207.3369185715606307, 85.19781250086714408 ) ) ;
#6991=CARTESIAN_POINT ( 'NONE',  ( -92.35000000000003695, 90.00000000000004263, 81.42749999999999488 ) ) ;
#6992=CARTESIAN_POINT ( 'NONE',  ( -97.64999999999994884, -208.4700217866474645, 79.78708333333332803 ) ) ;
#6993=CARTESIAN_POINT ( 'NONE',  ( -92.69370383062504004, 90.00000000000004263, 77.89531250086714920 ) ) ;
#6996=CARTESIAN_POINT ( 'NONE',  ( 97.30629616937498838, -209.9999999999999716, 88.69031250086715090 ) ) ;
#7004=VERTEX_POINT ( 'NONE', #73083 ) ;
#7008=CARTESIAN_POINT ( 'NONE',  ( 92.69370383062501162, -211.3315407142195852, 81.59947916753382913 ) ) ;
#7011=( GEOMETRIC_REPRESENTATION_CONTEXT ( 3 ) GLOBAL_UNCERTAINTY_ASSIGNED_CONTEXT ( ( #19549 ) ) GLOBAL_UNIT_ASSIGNED_CONTEXT ( ( #25581, #48514, #8671 ) ) REPRESENTATION_CONTEXT ( 'NONE', 'WORKASPACE' ) );
#7013=CARTESIAN_POINT ( 'NONE',  ( 92.35000000000000853, -209.9999999999999716, 76.66499999999999204 ) ) ;
#7015=CARTESIAN_POINT ( 'NONE',  ( 97.64999999999999147, -209.9999999999999716, 83.96750000000000114 ) ) ;
#7019=ORIENTED_EDGE ( 'NONE', *, *, #13477, .T. ) ;
#7023=CARTESIAN_POINT ( 'NONE',  ( -95.00000000000002842, 87.33691857156074434, 86.15031250086714465 ) ) ;
#7026=DIRECTION ( 'NONE',  ( -0.000000000000000000, -0.000000000000000000, 1.000000000000000000 ) ) ;
#7027=CARTESIAN_POINT ( 'NONE',  ( 97.30629616937498838, -211.3315407142195852, 88.00239583420047040 ) ) ;
#7029=CARTESIAN_POINT ( 'NONE',  ( 96.32499999999998863, 87.70503267997126784, 78.14666666666667538 ) ) ;
#7030=ORIENTED_EDGE ( 'NONE', *, *, #65481, .T. ) ;
#7031=LINE ( 'NONE', #30328, #70757 ) ;
#7034=CARTESIAN_POINT ( 'NONE',  ( -95.00000000000002842, 93.05995642670501411, 87.38062500173430180 ) ) ;
#7036=CARTESIAN_POINT ( 'NONE',  ( 97.30629616937498838, 90.00000000000002842, 75.99031250086714806 ) ) ;
#7044=DIRECTION ( 'NONE',  ( -0.000000000000000000, -0.000000000000000000, 1.000000000000000000 ) ) ;
#7050=VERTEX_POINT ( 'NONE', #55815 ) ;
#7055=CARTESIAN_POINT ( 'NONE',  ( 92.35000000000000853, -209.9999999999999716, 87.45999999999999375 ) ) ;
#7057=CARTESIAN_POINT ( 'NONE',  ( -96.15314808468745866, -211.9973110713294489, 86.73239583420048859 ) ) ;
#7062=VECTOR ( 'NONE', #11047, 1000.000000000000000 ) ;
#7066=EDGE_CURVE ( 'NONE', #3169, #65641, #61463, .T. ) ;
#7070=CARTESIAN_POINT ( 'NONE',  ( 97.30629616937498838, 88.66845928578035796, 82.92239583420045790 ) ) ;
#7073=CARTESIAN_POINT ( 'NONE',  ( -93.67500000000003979, 92.29496732002878900, 80.89833333333332632 ) ) ;
#7081=( BOUNDED_CURVE ( )  B_SPLINE_CURVE ( 2, ( #23908, #59602, #35547, #18988, #13357, #46847, #7360 ),
 .UNSPECIFIED., .F., .F. ) 
 B_SPLINE_CURVE_WITH_KNOTS ( ( 3, 2, 2, 3 ),
 ( 0.2328402629019979686, 0.2398960283900005708, 0.2469517939308829568, 0.2540073681283125939 ),
 .UNSPECIFIED. ) 
 CURVE ( )  GEOMETRIC_REPRESENTATION_ITEM ( )  RATIONAL_B_SPLINE_CURVE ( ( 1.000000000000000000, 0.8660254037844387076, 1.000000000000000000, 0.8660254037844387076, 1.000000000000000000, 0.8660290370063296050, 0.9999927337532750204 ) ) 
 REPRESENTATION_ITEM ( '' )  );
#7085=CARTESIAN_POINT ( 'NONE',  ( -95.00000000000002842, 92.66308142843932671, 85.03906250086714635 ) ) ;
#7086=CARTESIAN_POINT ( 'NONE',  ( 97.64999999999999147, 90.00000000000002842, 83.33250000000001023 ) ) ;
#7087=AXIS2_PLACEMENT_3D ( 'NONE', #41807, #35065, #6860 ) ;
#7092=CARTESIAN_POINT ( 'NONE',  ( 97.64999999999821512, -209.9999969335172807, 75.79187510780352000 ) ) ;
#7097=CARTESIAN_POINT ( 'NONE',  ( 97.30629616937498838, -211.3315407142195852, 83.71614583420050337 ) ) ;
#7101=VERTEX_POINT ( 'NONE', #20497 ) ;
#7104=CARTESIAN_POINT ( 'NONE',  ( 97.65000000000004832, -208.4700217866474929, 88.46541666666664128 ) ) ;
#7105=CARTESIAN_POINT ( 'NONE',  ( 93.84685191531249870, -208.0026889286704943, 75.56697916753381605 ) ) ;
#7107=CARTESIAN_POINT ( 'NONE',  ( 93.84685191531249870, -208.0026889286704943, 80.17072916753382117 ) ) ;
#7108=VECTOR ( 'NONE', #72787, 1000.000000000000000 ) ;
#7109=VECTOR ( 'NONE', #36447, 1000.000000000000000 ) ;
#7114=ORIENTED_EDGE ( 'NONE', *, *, #25956, .T. ) ;
#7123=CARTESIAN_POINT ( 'NONE',  ( -92.35000000000012221, 91.52997821335257811, 84.02041666666666231 ) ) ;
#7124=CARTESIAN_POINT ( 'NONE',  ( 95.00000000000000000, -213.0599564267049857, 84.52312500173428589 ) ) ;
#7126=CARTESIAN_POINT ( 'NONE',  ( 92.34999999999999432, 90.00000000000002842, 89.36499999999999488 ) ) ;
#7137=CARTESIAN_POINT ( 'NONE',  ( 97.64999999999999147, 90.00000000000002842, 86.58687500173429896 ) ) ;
#7148=CARTESIAN_POINT ( 'NONE',  ( -96.32500000000001705, 92.29496732002878900, 87.35416666666665719 ) ) ;
#7154=CARTESIAN_POINT ( 'NONE',  ( -96.15314808468747287, -208.0026889286704943, 82.55197916753380127 ) ) ;
#7159=CARTESIAN_POINT ( 'NONE',  ( -97.64999999954989107, -210.0000310946949753, 88.81037122969127040 ) ) ;
#7164=EDGE_CURVE ( 'NONE', #73338, #3737, #71394, .T. ) ;
#7172=CARTESIAN_POINT ( 'NONE',  ( -93.84685191531252713, 88.00268892867056536, 77.78947916753381264 ) ) ;
#7174=CARTESIAN_POINT ( 'NONE',  ( 97.64999999999999147, 90.00000000000002842, 76.34749999999999659 ) ) ;
#7183=CARTESIAN_POINT ( 'NONE',  ( -92.69370383062498320, -208.6684592857803011, 74.93197916753381094 ) ) ;
#7185=VECTOR ( 'NONE', #757, 1000.000000000000000 ) ;
#7187=ORIENTED_EDGE ( 'NONE', *, *, #53215, .T. ) ;
#7198=CARTESIAN_POINT ( 'NONE',  ( 96.15314808468750130, -211.9973110713294489, 83.50447916753381605 ) ) ;
#7199=CARTESIAN_POINT ( 'NONE',  ( 93.84685191531251292, -211.9973110713294489, 88.63739583420048973 ) ) ;
#7200=ORIENTED_EDGE ( 'NONE', *, *, #11598, .F. ) ;
#7202=CARTESIAN_POINT ( 'NONE',  ( 96.15314808468750130, -211.9973110713294489, 88.74322916753382628 ) ) ;
#7204=ORIENTED_EDGE ( 'NONE', *, *, #70697, .F. ) ;
#7207=CARTESIAN_POINT ( 'NONE',  ( -95.00000000000002842, 92.66308142843932671, 80.75281250086715090 ) ) ;
#7216=EDGE_CURVE ( 'NONE', #73668, #50254, #41800, .T. ) ;
#7227=CARTESIAN_POINT ( 'NONE',  ( 97.30629616937498838, -208.6684592857803011, 82.39322916753381776 ) ) ;
#7230=AXIS2_PLACEMENT_3D ( 'NONE', #19717, #25374, #42663 ) ;
#7232=CARTESIAN_POINT ( 'NONE',  ( -92.35000000000000853, 88.47002178664756400, 82.00958333333333883 ) ) ;
#7233=CARTESIAN_POINT ( 'NONE',  ( -97.64999999999996305, -209.9999999999999716, 78.64937500173429896 ) ) ;
#7234=CARTESIAN_POINT ( 'NONE',  ( 92.34999999999998010, -208.4700217866475214, 79.15208333333333712 ) ) ;
#7235=CARTESIAN_POINT ( 'NONE',  ( -96.32499999999996021, -212.2949673200287179, 75.50083333333331836 ) ) ;
#7240=CARTESIAN_POINT ( 'NONE',  ( -96.15314808468747287, -208.0026889286704943, 83.18697916753382060 ) ) ;
#7242=CARTESIAN_POINT ( 'NONE',  ( -95.00000000000002842, 87.33691857156074434, 83.61031250086716682 ) ) ;
#7245=CARTESIAN_POINT ( 'NONE',  ( 92.69370383062498320, 88.66845928578037217, 80.80572916753382628 ) ) ;
#7246=ORIENTED_EDGE ( 'NONE', *, *, #40752, .F. ) ;
#7252=CARTESIAN_POINT ( 'NONE',  ( -93.84685191531247028, -211.9973110713294489, 85.40947916753380298 ) ) ;
#7263=CARTESIAN_POINT ( 'NONE',  ( -96.15314808468752972, 91.99731107132950569, 89.53697916753381492 ) ) ;
#7265=CARTESIAN_POINT ( 'NONE',  ( 97.64999999999993463, 91.52997821335253548, 76.40041666666667197 ) ) ;
#7274=CARTESIAN_POINT ( 'NONE',  ( 92.35000000019411459, -210.0000198431783929, 84.36502760998391182 ) ) ;
#7277=CARTESIAN_POINT ( 'NONE',  ( -92.69370383062498320, -209.9999999999999716, 86.30906250086715659 ) ) ;
#7280=EDGE_CURVE ( 'NONE', #44409, #59589, #57838, .T. ) ;
#7281=CARTESIAN_POINT ( 'NONE',  ( -92.69370383062496899, -210.9303121318039871, 74.84209103131394158 ) ) ;
#7286=CARTESIAN_POINT ( 'NONE',  ( 94.99999999999998579, 93.05995642670504253, 75.87125000000000341 ) ) ;
#7287=CARTESIAN_POINT ( 'NONE',  ( -92.35000000005469190, 89.99998298270445218, 88.49187441316097136 ) ) ;
#7290=EDGE_CURVE ( 'NONE', #30489, #63633, #66157, .T. ) ;
#7293=CARTESIAN_POINT ( 'NONE',  ( 93.84685191531249870, -208.0026889286704943, 75.56697916753381605 ) ) ;
#7298=( BOUNDED_CURVE ( )  B_SPLINE_CURVE ( 2, ( #8283, #3048, #24833, #71419, #20300, #19557, #42502 ),
 .UNSPECIFIED., .F., .F. ) 
 B_SPLINE_CURVE_WITH_KNOTS ( ( 3, 2, 2, 3 ),
 ( 0.9101937466091534201, 0.9172495203147085219, 0.9243052858555914630, 0.9313609857393204683 ),
 .UNSPECIFIED. ) 
 CURVE ( )  GEOMETRIC_REPRESENTATION_ITEM ( )  RATIONAL_B_SPLINE_CURVE ( ( 1.000000000000000000, 0.8660254037844387076, 1.000000000000000000, 0.8660254037844387076, 1.000000000000000000, 0.8660266504798714848, 0.9999975066323365525 ) ) 
 REPRESENTATION_ITEM ( '' )  );
#7304=ORIENTED_EDGE ( 'NONE', *, *, #26905, .T. ) ;
#7307=ORIENTED_EDGE ( 'NONE', *, *, #3695, .T. ) ;
#7309=CARTESIAN_POINT ( 'NONE',  ( 94.99999999999998579, 87.33691857156068750, 80.43531250086715545 ) ) ;
#7312=CARTESIAN_POINT ( 'NONE',  ( 96.32499999999998863, -212.2949673200287179, 75.60666666666665492 ) ) ;
#7325=CARTESIAN_POINT ( 'NONE',  ( 92.35000000003287823, -209.9999916080746516, 86.90410584365268676 ) ) ;
#7328=CARTESIAN_POINT ( 'NONE',  ( -94.99999999999997158, -206.9400435732949575, 80.39562500173431658 ) ) ;
#7333=CARTESIAN_POINT ( 'NONE',  ( 93.67499999999998295, 92.29496732002878900, 77.27354166840096639 ) ) ;
#7334=CARTESIAN_POINT ( 'NONE',  ( -96.32500000000001705, 87.70503267997129626, 77.48520833506763950 ) ) ;
#7337=CARTESIAN_POINT ( 'NONE',  ( 94.99999999999998579, 92.66308142843935514, 80.11781250086714579 ) ) ;
#7356=CARTESIAN_POINT ( 'NONE',  ( -94.99999999999997158, -212.6630814284392557, 77.89531250086714920 ) ) ;
#7357=ORIENTED_EDGE ( 'NONE', *, *, #59523, .T. ) ;
#7358=CARTESIAN_POINT ( 'NONE',  ( -95.00000000000002842, 90.00000000000004263, 90.00000000000000000 ) ) ;
#7359=CARTESIAN_POINT ( 'NONE',  ( 92.34999999999999432, 90.00000000000002842, 77.29999999999999716 ) ) ;
#7360=CARTESIAN_POINT ( 'NONE',  ( 92.35000000049295465, 89.99996796756887818, 85.63541623677173220 ) ) ;
#7365=DIRECTION ( 'NONE',  ( -0.000000000000000000, -0.000000000000000000, 1.000000000000000000 ) ) ;
#7368=CARTESIAN_POINT ( 'NONE',  ( 94.99999999999998579, 87.33691857156068750, 84.88031250086713442 ) ) ;
#7369=CARTESIAN_POINT ( 'NONE',  ( -94.99999999999997158, -207.3369185715606307, 87.73781250086715033 ) ) ;
#7374=CARTESIAN_POINT ( 'NONE',  ( -96.32499999999996021, -212.2949673200287179, 81.21583333333333599 ) ) ;
#7379=CARTESIAN_POINT ( 'NONE',  ( 96.15314808468750130, -211.9973110713294489, 87.31447916753380412 ) ) ;
#7386=EDGE_CURVE ( 'NONE', #33091, #15908, #10370, .T. ) ;
#7394=CARTESIAN_POINT ( 'NONE',  ( 92.69370383062501162, -209.9999999999999716, 81.54656250086715374 ) ) ;
#7396=DIRECTION ( 'NONE',  ( 1.000000000000000000, 0.000000000000000000, 0.000000000000000000 ) ) ;
#7401=CARTESIAN_POINT ( 'NONE',  ( 97.64999999999997726, -211.5299782133524502, 86.45458333333333201 ) ) ;
#7407=CARTESIAN_POINT ( 'NONE',  ( -96.15314808468752972, 91.99731107132950569, 86.52072916753382970 ) ) ;
#7410=CARTESIAN_POINT ( 'NONE',  ( 97.30629616937498838, -209.9999999999999716, 87.42031250086714067 ) ) ;
#7411=CARTESIAN_POINT ( 'NONE',  ( 92.34999999999999432, 91.52997821335252127, 77.24708333333332178 ) ) ;
#7413=CARTESIAN_POINT ( 'NONE',  ( -92.34999999999999432, -211.5299782133524502, 87.80395833506763381 ) ) ;
#7417=CARTESIAN_POINT ( 'NONE',  ( -97.64999999990727986, 90.00001381026693537, 80.55392363656929433 ) ) ;
#7420=CARTESIAN_POINT ( 'NONE',  ( -97.65000000000001990, 90.00000000000004263, 87.53937500173429953 ) ) ;
#7421=CARTESIAN_POINT ( 'NONE',  ( 92.69370383062498320, 91.33154071421968467, 89.74864583420048803 ) ) ;
#7422=EDGE_LOOP ( 'NONE', ( #49213, #71459, #35668, #9922 ) ) ;
#7427=AXIS2_PLACEMENT_3D ( 'NONE', #42846, #30437, #42117 ) ;
#7428=CARTESIAN_POINT ( 'NONE',  ( -94.99999999999997158, -206.9400435732949575, 86.11062500173430578 ) ) ;
#7431=CARTESIAN_POINT ( 'NONE',  ( -92.69370383062498320, -208.6684592857803011, 75.40822916753381833 ) ) ;
#7438=CARTESIAN_POINT ( 'NONE',  ( -92.69370383062498320, -211.3315407142195852, 86.89114583420050053 ) ) ;
#7446=CARTESIAN_POINT ( 'NONE',  ( 92.69370383062498320, 88.66845928578035796, 80.80572916753379786 ) ) ;
#7453=CYLINDRICAL_SURFACE ( 'NONE', #68721, 2.649999999999985700 ) ;
#7458=CARTESIAN_POINT ( 'NONE',  ( -95.00000000000002842, 87.33691857156074434, 85.99156250086714692 ) ) ;
#7459=CARTESIAN_POINT ( 'NONE',  ( 26.49955575014745079, 0.001194404164630089764, -80.00000000000000000 ) ) ;
#7471=CARTESIAN_POINT ( 'NONE',  ( 92.69370383062501162, -208.6684592857803011, 82.12864583420048348 ) ) ;
#7474=VERTEX_POINT ( 'NONE', #7055 ) ;
#7484=CARTESIAN_POINT ( 'NONE',  ( 97.30629616937498838, -209.9999999999999716, 80.59406250086715318 ) ) ;
#7491=CARTESIAN_POINT ( 'NONE',  ( 92.35001072511524001, -208.4700155944993014, 86.85145790673756494 ) ) ;
#7496=CARTESIAN_POINT ( 'NONE',  ( 96.32499999999998863, -212.2949673200287179, 85.21104166840096639 ) ) ;
#7497=CARTESIAN_POINT ( 'NONE',  ( 93.67499999999998295, 92.29496732002878900, 88.62416666666665321 ) ) ;
#7504=CARTESIAN_POINT ( 'NONE',  ( -97.30629616937501680, 88.66845928578038638, 86.67947916753382742 ) ) ;
#7505=CARTESIAN_POINT ( 'NONE',  ( 94.99999999999998579, 92.66308142843935514, 84.40406250086712703 ) ) ;
#7507=CARTESIAN_POINT ( 'NONE',  ( 92.34999999999999432, 88.47002178664753558, 84.41729166840097776 ) ) ;
#7509=B_SPLINE_CURVE_WITH_KNOTS ( 'NONE', 1,
 ( #16012, #10374 ),
 .UNSPECIFIED., .F., .F.,
 ( 2, 2 ),
 ( 0.000000000000000000, 1.000000000000000000 ),
 .UNSPECIFIED. ) ;
#7514=ORIENTED_EDGE ( 'NONE', *, *, #9602, .F. ) ;
#7516=CARTESIAN_POINT ( 'NONE',  ( -99.99999999999998579, -116.0000000000000000, -40.00000000000002132 ) ) ;
#7517=DIRECTION ( 'NONE',  ( 1.000000000000000000, 0.000000000000000000, 0.000000000000000000 ) ) ;
#7518=CARTESIAN_POINT ( 'NONE',  ( -92.35000000000005116, 88.47002178664754979, 85.81958333333331268 ) ) ;
#7523=( BOUNDED_CURVE ( )  B_SPLINE_CURVE ( 2, ( #67629, #10108, #62000, #9363, #43603, #37946, #38316 ),
 .UNSPECIFIED., .F., .F. ) 
 B_SPLINE_CURVE_WITH_KNOTS ( ( 3, 2, 2, 3 ),
 ( 0.2291666666666663521, 0.2361111111111107719, 0.2430555555555551639, 0.2499999999999995837 ),
 .UNSPECIFIED. ) 
 CURVE ( )  GEOMETRIC_REPRESENTATION_ITEM ( )  RATIONAL_B_SPLINE_CURVE ( ( 1.000000000000005995, 0.8660254037844328234, 1.000000000000000000, 0.8660254037844387076, 1.000000000000000000, 0.8660254037844467012, 0.9999999999999920064 ) ) 
 REPRESENTATION_ITEM ( '' )  );
#7525=CARTESIAN_POINT ( 'NONE',  ( -96.15314808468745866, -211.9973110713294489, 84.03364583420047040 ) ) ;
#7526=ORIENTED_EDGE ( 'NONE', *, *, #21115, .F. ) ;
#7534=CARTESIAN_POINT ( 'NONE',  ( -92.34999999999999432, -209.9999999999999716, 83.96750000000000114 ) ) ;
#7538=VECTOR ( 'NONE', #64409, 1000.000000000000000 ) ;
#7539=CARTESIAN_POINT ( 'NONE',  ( -92.69370383062502583, 91.33154071421968467, 89.53697916753382913 ) ) ;
#7543=CARTESIAN_POINT ( 'NONE',  ( -97.65000000000001990, 90.00000000000004263, 89.90078125043358170 ) ) ;
#7544=EDGE_CURVE ( 'NONE', #36799, #5972, #43546, .T. ) ;
#7549=CARTESIAN_POINT ( 'NONE',  ( 96.32499999999998863, -212.2949673200287179, 77.51166666666665606 ) ) ;
#7553=CARTESIAN_POINT ( 'NONE',  ( -97.30629616937497417, -208.6684592857803011, 75.14364583420049826 ) ) ;
#7554=ADVANCED_FACE ( 'NONE', ( #60794 ), #60428, .F. ) ;
#7568=CARTESIAN_POINT ( 'NONE',  ( 92.69370383062501162, -211.3315407142195852, 85.88572916753381037 ) ) ;
#7569=CARTESIAN_POINT ( 'NONE',  ( 92.69370383062501162, -209.9999999999999716, 89.16656250086715829 ) ) ;
#7571=CARTESIAN_POINT ( 'NONE',  ( 97.30629616937498838, -209.9999999999999716, 88.21406250086714351 ) ) ;
#7577=CARTESIAN_POINT ( 'NONE',  ( -97.30629616937501680, 91.33154071421968467, 79.58864583420047722 ) ) ;
#7580=CARTESIAN_POINT ( 'NONE',  ( -2.499999999999970690, 73.00000000000001421, -255.0000000000000000 ) ) ;
#7582=CARTESIAN_POINT ( 'NONE',  ( 92.35001072950502987, -208.4700155919648807, 84.94645790656225870 ) ) ;
#7586=EDGE_CURVE ( 'NONE', #16851, #19930, #50760, .T. ) ;
#7588=ORIENTED_EDGE ( 'NONE', *, *, #52692, .F. ) ;
#7591=ORIENTED_EDGE ( 'NONE', *, *, #51886, .F. ) ;
#7594=CARTESIAN_POINT ( 'NONE',  ( 96.15314808468750130, -211.9973110713294489, 79.69447916753379957 ) ) ;
#7604=CARTESIAN_POINT ( 'NONE',  ( -97.30629616937495996, -209.9999999999999716, 85.19781250086714408 ) ) ;
#7605=CARTESIAN_POINT ( 'NONE',  ( -96.15314808468752972, 91.99731107132950569, 83.34572916753383254 ) ) ;
#7607=CARTESIAN_POINT ( 'NONE',  ( 94.99999999999998579, 87.33691857156068750, 79.64156250086713840 ) ) ;
#7614=CARTESIAN_POINT ( 'NONE',  ( -97.30629616937497417, -208.6684592857803295, 83.23989583420048177 ) ) ;
#7620=CARTESIAN_POINT ( 'NONE',  ( -93.67500000000003979, 92.29496732002878900, 75.81833333333332803 ) ) ;
#7621=CARTESIAN_POINT ( 'NONE',  ( -93.67500000000003979, 87.70503267997129626, 84.57604166840096127 ) ) ;
#7623=CARTESIAN_POINT ( 'NONE',  ( -96.34407192492896854, -207.9734350352809429, 74.86703477254887673 ) ) ;
#7629=CARTESIAN_POINT ( 'NONE',  ( -92.69370383062504004, 90.00000000000004263, 75.35531250086714294 ) ) ;
#7635=CARTESIAN_POINT ( 'NONE',  ( 92.35000000000000853, -209.9999999999999716, 84.36437500173430237 ) ) ;
#7637=CARTESIAN_POINT ( 'NONE',  ( -96.15314808468745866, -211.9973110713294489, 86.73239583420048859 ) ) ;
#7644=CARTESIAN_POINT ( 'NONE',  ( -92.69370383062498320, -209.9999999999999716, 77.41906250086715602 ) ) ;
#7647=CARTESIAN_POINT ( 'NONE',  ( -92.35000000045951651, -209.9999506483816560, 87.22187670868756015 ) ) ;
#7648=DIRECTION ( 'NONE',  ( 1.000000000000000000, 0.000000000000000000, 0.000000000000000000 ) ) ;
#7653=CARTESIAN_POINT ( 'NONE',  ( 93.84685191531249870, -208.0026889286704943, 78.10697916753380809 ) ) ;
#7665=ORIENTED_EDGE ( 'NONE', *, *, #30644, .F. ) ;
#7672=CARTESIAN_POINT ( 'NONE',  ( 92.69370383062498320, 90.00000000000002842, 80.27656250086714351 ) ) ;
#7683=CARTESIAN_POINT ( 'NONE',  ( -97.64999999999996305, -209.9999999999999716, 77.29999999999999716 ) ) ;
#7689=CARTESIAN_POINT ( 'NONE',  ( -96.32499999999996021, -207.7050326799711968, 77.90854166840097150 ) ) ;
#7691=CARTESIAN_POINT ( 'NONE',  ( 93.67499999999999716, 87.70503267997126784, 76.85020833506763438 ) ) ;
#7692=CARTESIAN_POINT ( 'NONE',  ( -97.65000000000001990, 91.52997821335253548, 75.42145833506764063 ) ) ;
#7694=CARTESIAN_POINT ( 'NONE',  ( 92.69370383062498320, 91.33154071421968467, 78.31864583420050963 ) ) ;
#7696=DIRECTION ( 'NONE',  ( -0.000000000000000000, -0.000000000000000000, 1.000000000000000000 ) ) ;
#7699=DIRECTION ( 'NONE',  ( -0.000000000000000000, -0.000000000000000000, 1.000000000000000000 ) ) ;
#7711=CARTESIAN_POINT ( 'NONE',  ( 95.00000000000000000, -206.9400435732949575, 82.85625000000000284 ) ) ;
#7717=CARTESIAN_POINT ( 'NONE',  ( -92.69370383062498320, -211.3315407142195852, 77.36614583420048064 ) ) ;
#7718=ORIENTED_EDGE ( 'NONE', *, *, #69780, .F. ) ;
#7721=CARTESIAN_POINT ( 'NONE',  ( 95.00000000000000000, -209.9999999999999716, 90.00000000000000000 ) ) ;
#7731=( BOUNDED_CURVE ( )  B_SPLINE_CURVE ( 2, ( #39624, #68194, #50520, #44898, #21572, #15572, #27957 ),
 .UNSPECIFIED., .F., .F. ) 
 B_SPLINE_CURVE_WITH_KNOTS ( ( 3, 2, 2, 3 ),
 ( 0.7291666666666665186, 0.7361111111111109384, 0.7430555555555553582, 0.7499999999999996669 ),
 .UNSPECIFIED. ) 
 CURVE ( )  GEOMETRIC_REPRESENTATION_ITEM ( )  RATIONAL_B_SPLINE_CURVE ( ( 1.000000000000002220, 0.8660254037844365982, 1.000000000000000000, 0.8660254037844387076, 1.000000000000000000, 0.8660254037844451469, 0.9999999999999935607 ) ) 
 REPRESENTATION_ITEM ( '' )  );
#7733=CARTESIAN_POINT ( 'NONE',  ( 96.15314808468748708, 91.99731107132950569, 83.87489583420048689 ) ) ;
#7734=CARTESIAN_POINT ( 'NONE',  ( -92.69370383062498320, -211.3315407142195852, 84.98614583420047097 ) ) ;
#7736=ORIENTED_EDGE ( 'NONE', *, *, #55840, .F. ) ;
#7738=CARTESIAN_POINT ( 'NONE',  ( -93.67499999999998295, -207.7050326799711968, 79.62833333333333030 ) ) ;
#7739=CARTESIAN_POINT ( 'NONE',  ( -96.15314808468751551, 88.00268892867056536, 77.04864583420047097 ) ) ;
#7741=CARTESIAN_POINT ( 'NONE',  ( 93.84685191531249870, -208.0026889286704943, 88.26697916753380468 ) ) ;
#7742=ADVANCED_FACE ( 'NONE', ( #276 ), #73910, .F. ) ;
#7744=EDGE_CURVE ( 'NONE', #32195, #17108, #22805, .T. ) ;
#7747=AXIS2_PLACEMENT_3D ( 'NONE', #1442, #58917, #53267 ) ;
#7751=CARTESIAN_POINT ( 'NONE',  ( 97.64999999999999147, -209.9999999999999716, 75.71250000000000568 ) ) ;
#7758=CARTESIAN_POINT ( 'NONE',  ( 95.00000000000000000, -212.6630814284392557, 81.70531250086715147 ) ) ;
#7759=DIRECTION ( 'NONE',  ( 1.000000000000000000, 0.000000000000000000, 0.000000000000000000 ) ) ;
#7765=CARTESIAN_POINT ( 'NONE',  ( 96.32499999999998863, -212.2949673200287179, 83.22666666666665947 ) ) ;
#7767=VERTEX_POINT ( 'NONE', #44621 ) ;
#7768=ORIENTED_EDGE ( 'NONE', *, *, #55280, .F. ) ;
#7771=CARTESIAN_POINT ( 'NONE',  ( -95.00000000000002842, 87.33691857156074434, 85.51531250086713953 ) ) ;
#7774=CARTESIAN_POINT ( 'NONE',  ( 93.84685191531249870, -208.0026889286704943, 86.99697916753380866 ) ) ;
#7777=CARTESIAN_POINT ( 'NONE',  ( 93.67499999999998295, 92.29496732002878900, 79.73416666666666686 ) ) ;
#7778=EDGE_CURVE ( 'NONE', #56779, #27169, #34430, .T. ) ;
#7782=CARTESIAN_POINT ( 'NONE',  ( -95.00000000000002842, 93.05995642670501411, 84.84062500173429555 ) ) ;
#7783=CARTESIAN_POINT ( 'NONE',  ( 93.84685191531248449, 91.99731107132950569, 86.52072916753382970 ) ) ;
#7790=CARTESIAN_POINT ( 'NONE',  ( -93.84685191531247028, -211.9973110713294489, 75.88447916753381151 ) ) ;
#7793=EDGE_CURVE ( 'NONE', #31889, #25853, #38973, .T. ) ;
#7798=CARTESIAN_POINT ( 'NONE',  ( -97.30629616937495996, -209.9999999999999716, 88.53156250086716739 ) ) ;
#7801=CARTESIAN_POINT ( 'NONE',  ( -97.64999999999996305, -209.9999999999999716, 82.37999999999999545 ) ) ;
#7804=ADVANCED_FACE ( 'NONE', ( #63393 ), #5885, .F. ) ;
#7810=CARTESIAN_POINT ( 'NONE',  ( 93.84685191531248449, 91.99731107132950569, 81.28197916753380525 ) ) ;
#7811=CARTESIAN_POINT ( 'NONE',  ( -97.64999999999996305, -209.9999999999999716, 83.65000000000000568 ) ) ;
#7818=CARTESIAN_POINT ( 'NONE',  ( 94.99999999999998579, 86.94004357329502852, 83.80875000000000341 ) ) ;
#7824=CARTESIAN_POINT ( 'NONE',  ( -92.69370383062504004, 90.00000000000004263, 88.05531250086713158 ) ) ;
#7831=EDGE_CURVE ( 'NONE', #50886, #4344, #56035, .T. ) ;
#7835=VECTOR ( 'NONE', #71938, 1000.000000000000000 ) ;
#7836=CARTESIAN_POINT ( 'NONE',  ( 97.30629616937498838, -208.6684592857803011, 81.91697916753381037 ) ) ;
#7838=ORIENTED_EDGE ( 'NONE', *, *, #37171, .T. ) ;
#7839=DIRECTION ( 'NONE',  ( -1.000000000000000000, 0.000000000000000000, 0.000000000000000000 ) ) ;
#7846=CARTESIAN_POINT ( 'NONE',  ( 93.84685191531251292, -211.9973110713294489, 79.74739583420048916 ) ) ;
#7852=CARTESIAN_POINT ( 'NONE',  ( -96.32499999999996021, -207.7050326799711968, 82.35354166840096468 ) ) ;
#7853=CARTESIAN_POINT ( 'NONE',  ( 97.64999999946594755, 90.00005320149050192, 78.96687695417308817 ) ) ;
#7856=LINE ( 'NONE', #12750, #24479 ) ;
#7857=CARTESIAN_POINT ( 'NONE',  ( 97.64999999999997726, -208.4700217866474645, 83.46479166840096298 ) ) ;
#7858=CARTESIAN_POINT ( 'NONE',  ( 92.34999999999999432, 91.52997821335252127, 84.23208333333333542 ) ) ;
#7864=CARTESIAN_POINT ( 'NONE',  ( -97.30629616937501680, 88.66845928578038638, 87.94947916753382344 ) ) ;
#7865=CARTESIAN_POINT ( 'NONE',  ( 93.84685191531248449, 88.00268892867053694, 85.93864583420048575 ) ) ;
#7868=CARTESIAN_POINT ( 'NONE',  ( 93.67499999999998295, 92.29496732002878900, 85.52854166840096184 ) ) ;
#7870=ORIENTED_EDGE ( 'NONE', *, *, #51256, .T. ) ;
#7872=ORIENTED_EDGE ( 'NONE', *, *, #68849, .T. ) ;
#7876=CARTESIAN_POINT ( 'NONE',  ( -95.00000000000002842, 93.05995642670504253, 86.03125000000000000 ) ) ;
#7879=CARTESIAN_POINT ( 'NONE',  ( -96.32500000000001705, 92.29496732002878900, 84.81416666666666515 ) ) ;
#7881=EDGE_LOOP ( 'NONE', ( #66131, #49749, #72498, #39701 ) ) ;
#7882=CARTESIAN_POINT ( 'NONE',  ( 93.67499999999999716, 87.70503267997126784, 81.85083333333332689 ) ) ;
#7883=DIRECTION ( 'NONE',  ( -0.000000000000000000, -0.000000000000000000, 1.000000000000000000 ) ) ;
#7886=CARTESIAN_POINT ( 'NONE',  ( -94.99999999999997158, -212.6630814284392557, 82.81656250086713555 ) ) ;
#7896=CARTESIAN_POINT ( 'NONE',  ( 93.67499999999998295, 92.29496732002878900, 82.98854166840096980 ) ) ;
#7897=CARTESIAN_POINT ( 'NONE',  ( 97.30629616937500259, 90.00000000000002842, 74.79348190356851944 ) ) ;
#7898=CARTESIAN_POINT ( 'NONE',  ( -93.84685191531252713, 88.00268892867056536, 89.37822916753381719 ) ) ;
#7906=EDGE_CURVE ( 'NONE', #39489, #42628, #60348, .T. ) ;
#7908=CARTESIAN_POINT ( 'NONE',  ( 90.00000000000000000, 95.00000000000002842, 90.00000000000000000 ) ) ;
#7910=CARTESIAN_POINT ( 'NONE',  ( 95.73997229764715655, 87.43182282693489071, 75.00000000000000000 ) ) ;
#7911=CYLINDRICAL_SURFACE ( 'NONE', #29795, 26.50000000000000355 ) ;
#7913=CYLINDRICAL_SURFACE ( 'NONE', #48422, 2.649999999999985700 ) ;
#7914=CARTESIAN_POINT ( 'NONE',  ( -97.64999999999994884, -208.4700217866474645, 86.77208333333334167 ) ) ;
#7918=CIRCLE ( 'NONE', #15106, 12.75000000000000000 ) ;
#7922=SURFACE_STYLE_USAGE ( .BOTH. , #37249 ) ;
#7925=VERTEX_POINT ( 'NONE', #57750 ) ;
#7929=( BOUNDED_CURVE ( )  B_SPLINE_CURVE ( 2, ( #59769, #48480, #41367, #64666, #19161, #71395, #42843 ),
 .UNSPECIFIED., .F., .F. ) 
 B_SPLINE_CURVE_WITH_KNOTS ( ( 3, 2, 2, 3 ),
 ( 0.3125000000000001665, 0.3194444444444445308, 0.3263888888888890061, 0.3333333333333333703 ),
 .UNSPECIFIED. ) 
 CURVE ( )  GEOMETRIC_REPRESENTATION_ITEM ( )  RATIONAL_B_SPLINE_CURVE ( ( 0.9999999999999967804, 0.8660254037844419273, 1.000000000000000000, 0.8660254037844387076, 1.000000000000000000, 0.8660254037844375974, 1.000000000000001110 ) ) 
 REPRESENTATION_ITEM ( '' )  );
#7930=CARTESIAN_POINT ( 'NONE',  ( 93.84685191531251292, -211.9973110713294489, 84.03364583420047040 ) ) ;
#7931=CARTESIAN_POINT ( 'NONE',  ( 93.84685191531249870, -208.0026889286704943, 88.42572916753381662 ) ) ;
#7933=CARTESIAN_POINT ( 'NONE',  ( 97.30629616937498838, -211.3315407142195852, 89.43114583420049257 ) ) ;
#7937=CARTESIAN_POINT ( 'NONE',  ( -96.15314808468751551, 88.00268892867056536, 79.74739583420048916 ) ) ;
#7940=CARTESIAN_POINT ( 'NONE',  ( -96.32499999999996021, -212.2949673200287179, 87.64520833506762187 ) ) ;
#7947=( BOUNDED_CURVE ( )  B_SPLINE_CURVE ( 2, ( #27316, #56284, #50249, #58033, #73187, #21685, #61928 ),
 .UNSPECIFIED., .F., .F. ) 
 B_SPLINE_CURVE_WITH_KNOTS ( ( 3, 2, 2, 3 ),
 ( 0.4374999999999994449, 0.4444444444444441422, 0.4513888888888888951, 0.4583333333333335924 ),
 .UNSPECIFIED. ) 
 CURVE ( )  GEOMETRIC_REPRESENTATION_ITEM ( )  RATIONAL_B_SPLINE_CURVE ( ( 1.000000000000010658, 0.8660254037844280495, 1.000000000000000000, 0.8660254037844387076, 1.000000000000000000, 0.8660254037844333785, 1.000000000000005329 ) ) 
 REPRESENTATION_ITEM ( '' )  );
#7948=CARTESIAN_POINT ( 'NONE',  ( 92.35000000000000853, -209.9999999999999716, 90.00000000000000000 ) ) ;
#7954=CARTESIAN_POINT ( 'NONE',  ( 92.69370383062501162, -208.6684592857803011, 76.88989583420047325 ) ) ;
#7955=CARTESIAN_POINT ( 'NONE',  ( -95.00000000000002842, 93.05995642670504253, 83.49125000000000796 ) ) ;
#7957=ORIENTED_EDGE ( 'NONE', *, *, #1091, .T. ) ;
#7965=FACE_OUTER_BOUND ( 'NONE', #338, .T. ) ;
#7968=CARTESIAN_POINT ( 'NONE',  ( -97.30629616937495996, -209.9999999999999716, 80.75281250086715090 ) ) ;
#7969=CARTESIAN_POINT ( 'NONE',  ( -95.00000000000002842, 92.66308142843932671, 77.57781250086715374 ) ) ;
#7972=CARTESIAN_POINT ( 'NONE',  ( 92.69370383062498320, 90.00000000000002842, 82.65781250086713783 ) ) ;
#7974=EDGE_CURVE ( 'NONE', #2269, #44809, #15742, .T. ) ;
#7976=CARTESIAN_POINT ( 'NONE',  ( 92.35000000010803944, 90.00001510551041406, 78.64888723592453346 ) ) ;
#7978=CARTESIAN_POINT ( 'NONE',  ( -97.64995971452495382, -211.5300014721822208, 83.14729327728629471 ) ) ;
#7981=CARTESIAN_POINT ( 'NONE',  ( -97.30629616937497417, -211.3315407142195852, 84.61572916753380014 ) ) ;
#7990=CARTESIAN_POINT ( 'NONE',  ( 92.34999999999999432, 90.00000000000002842, 84.92000000000000171 ) ) ;
#7992=CARTESIAN_POINT ( 'NONE',  ( -96.15314808468751551, 88.00268892867056536, 85.30364583420046642 ) ) ;
#7995=CARTESIAN_POINT ( 'NONE',  ( -97.65000000000001990, 90.00000000000004263, 83.65000000000000568 ) ) ;
#7998=CARTESIAN_POINT ( 'NONE',  ( -97.30629616937501680, 88.66845928578038638, 76.36072916753381890 ) ) ;
#8003=CARTESIAN_POINT ( 'NONE',  ( -93.07557990970624928, -211.8218417373838065, 75.00000000000000000 ) ) ;
#8006=CARTESIAN_POINT ( 'NONE',  ( -92.69370383062498320, -209.9999999999999716, 82.49906250086715431 ) ) ;
#8012=CARTESIAN_POINT ( 'NONE',  ( -94.99999999999997158, -212.6630814284392557, 77.89531250086714920 ) ) ;
#8015=ORIENTED_EDGE ( 'NONE', *, *, #17175, .F. ) ;
#8017=CARTESIAN_POINT ( 'NONE',  ( 100.0000000000000000, -214.9999999999999716, 90.00000000000000000 ) ) ;
#8021=CARTESIAN_POINT ( 'NONE',  ( 97.30629616937498838, -208.6684592857803011, 74.77322916753379900 ) ) ;
#8027=ORIENTED_EDGE ( 'NONE', *, *, #50735, .T. ) ;
#8036=DIRECTION ( 'NONE',  ( -1.000000000000000000, -0.000000000000000000, -0.000000000000000000 ) ) ;
#8040=CARTESIAN_POINT ( 'NONE',  ( 92.69370383062498320, 88.66845928578037217, 81.59947916753381492 ) ) ;
#8051=CARTESIAN_POINT ( 'NONE',  ( -96.01774234934310925, 92.19538700400588027, 74.85985921673510290 ) ) ;
#8056=EDGE_CURVE ( 'NONE', #67503, #58433, #22451, .T. ) ;
#8057=CARTESIAN_POINT ( 'NONE',  ( -97.64999999999996305, -209.9999999999999716, 75.47437500173430180 ) ) ;
#8058=CARTESIAN_POINT ( 'NONE',  ( -96.15314808468752972, 91.99731107132950569, 87.79072916753381151 ) ) ;
#8059=CARTESIAN_POINT ( 'NONE',  ( 93.67499999999999716, 87.70503267997126784, 76.21520833506762926 ) ) ;
#8060=CARTESIAN_POINT ( 'NONE',  ( -92.35000000000003695, 90.00000000000004263, 75.15687500173430635 ) ) ;
#8062=CARTESIAN_POINT ( 'NONE',  ( 93.84685191531248449, 91.99731107132950569, 77.63072916753381492 ) ) ;
#8066=CARTESIAN_POINT ( 'NONE',  ( 92.35000000046409241, -210.0000309672231253, 77.38038495127494798 ) ) ;
#8077=DIRECTION ( 'NONE',  ( -0.000000000000000000, -0.000000000000000000, 1.000000000000000000 ) ) ;
#8079=DIRECTION ( 'NONE',  ( -0.000000000000000000, -0.000000000000000000, 1.000000000000000000 ) ) ;
#8092=CARTESIAN_POINT ( 'NONE',  ( -94.99999999999997158, -209.9999999999999716, 90.00000000000000000 ) ) ;
#8095=CARTESIAN_POINT ( 'NONE',  ( -97.64999999996638280, -210.0000076551254722, 78.01464417100379478 ) ) ;
#8098=CARTESIAN_POINT ( 'NONE',  ( 93.84685191531248449, 88.00268892867053694, 85.46239583420047836 ) ) ;
#8099=CARTESIAN_POINT ( 'NONE',  ( -97.30629616937497417, -211.3315407142195852, 86.67947916753382742 ) ) ;
#8102=DIRECTION ( 'NONE',  ( 1.000000000000000000, 0.000000000000000000, 0.000000000000000000 ) ) ;
#8103=CARTESIAN_POINT ( 'NONE',  ( -97.64999999999994884, -211.5299782133524502, 81.16291666666666060 ) ) ;
#8104=CARTESIAN_POINT ( 'NONE',  ( -96.15314808468752972, 91.99731107132950569, 74.93197916753379673 ) ) ;
#8105=CARTESIAN_POINT ( 'NONE',  ( 93.84685191531251292, -211.9973110713294489, 85.30364583420046642 ) ) ;
#8107=ORIENTED_EDGE ( 'NONE', *, *, #169, .F. ) ;
#8109=ORIENTED_EDGE ( 'NONE', *, *, #65150, .F. ) ;
#8115=ORIENTED_EDGE ( 'NONE', *, *, #3410, .F. ) ;
#8117=CARTESIAN_POINT ( 'NONE',  ( 92.69370383062501162, -208.6684592857803295, 78.95364583420045790 ) ) ;
#8121=DIRECTION ( 'NONE',  ( 1.000000000000000000, 0.000000000000000000, 0.000000000000000000 ) ) ;
#8122=DIRECTION ( 'NONE',  ( -0.000000000000000000, -0.000000000000000000, 1.000000000000000000 ) ) ;
#8123=CARTESIAN_POINT ( 'NONE',  ( 93.67500000000001137, -212.2949673200287179, 82.48583333333333201 ) ) ;
#8129=VERTEX_POINT ( 'NONE', #3215 ) ;
#8132=CARTESIAN_POINT ( 'NONE',  ( -92.69370383062504004, 90.00000000000004263, 84.40406250086715545 ) ) ;
#8134=CARTESIAN_POINT ( 'NONE',  ( 97.64999017507810208, 88.47001611422622602, 88.43895794268868826 ) ) ;
#8135=AXIS2_PLACEMENT_3D ( 'NONE', #57445, #68737, #16860 ) ;
#8137=CARTESIAN_POINT ( 'NONE',  ( 92.34999999999999432, 88.47002178664753558, 75.44791666666667140 ) ) ;
#8141=CARTESIAN_POINT ( 'NONE',  ( -93.67499999999998295, -207.7050326799711968, 87.32770833506762642 ) ) ;
#8145=CARTESIAN_POINT ( 'NONE',  ( -95.00000000000002842, 86.94004357329504273, 86.42812500173430124 ) ) ;
#8148=CARTESIAN_POINT ( 'NONE',  ( 93.84685191531248449, 88.00268892867053694, 88.00239583420048461 ) ) ;
#8150=CARTESIAN_POINT ( 'NONE',  ( -95.00000000000002842, 90.00000000000004263, 90.00000000000000000 ) ) ;
#8155=CARTESIAN_POINT ( 'NONE',  ( -97.30629616937495996, -209.9999999999999716, 75.67281250086713840 ) ) ;
#8156=ORIENTED_EDGE ( 'NONE', *, *, #46962, .F. ) ;
#8163=( BOUNDED_CURVE ( )  B_SPLINE_CURVE ( 2, ( #74048, #57152, #68436, #6389, #52597, #16926, #1151 ),
 .UNSPECIFIED., .F., .F. ) 
 B_SPLINE_CURVE_WITH_KNOTS ( ( 3, 2, 2, 3 ),
 ( 0.5926843883797353607, 0.5997400709749998171, 0.6067958365158829803, 0.6138516023186938453 ),
 .UNSPECIFIED. ) 
 CURVE ( )  GEOMETRIC_REPRESENTATION_ITEM ( )  RATIONAL_B_SPLINE_CURVE ( ( 0.9999968501007930888, 0.8660269787525570750, 1.000000000000000000, 0.8660254037844387076, 1.000000000000000000, 0.8660254037844387076, 1.000000000000000000 ) ) 
 REPRESENTATION_ITEM ( '' )  );
#8164=CARTESIAN_POINT ( 'NONE',  ( -97.30629616937497417, -208.6684592857803011, 84.03364583420049883 ) ) ;
#8167=ORIENTED_EDGE ( 'NONE', *, *, #19948, .F. ) ;
#8171=CARTESIAN_POINT ( 'NONE',  ( 97.30629616937498838, 88.66845928578037217, 88.79614583420050167 ) ) ;
#8174=CARTESIAN_POINT ( 'NONE',  ( 92.69370383062498320, 91.33154071421968467, 81.33489583420048064 ) ) ;
#8180=CARTESIAN_POINT ( 'NONE',  ( -96.32500000000001705, 87.70503267997129626, 76.85020833506763438 ) ) ;
#8182=CARTESIAN_POINT ( 'NONE',  ( -93.07889023459847522, -208.6943671794269335, 74.79348190356851944 ) ) ;
#8185=CARTESIAN_POINT ( 'NONE',  ( -97.30629616937501680, 90.00000000000004263, 86.46781250086714010 ) ) ;
#8190=DIRECTION ( 'NONE',  ( -0.000000000000000000, -0.000000000000000000, 1.000000000000000000 ) ) ;
#8193=CARTESIAN_POINT ( 'NONE',  ( 92.35000000000000853, -209.9999999999999716, 83.65000000000000568 ) ) ;
#8197=CARTESIAN_POINT ( 'NONE',  ( 92.69370383062501162, -211.3315407142195852, 81.59947916753381492 ) ) ;
#8202=CARTESIAN_POINT ( 'NONE',  ( 95.00000000000000000, -209.9999999999999716, 90.00000000000000000 ) ) ;
#8209=CARTESIAN_POINT ( 'NONE',  ( 93.84685191531251292, -211.9973110713294489, 75.93739583420048689 ) ) ;
#8212=EDGE_CURVE ( 'NONE', #42545, #51073, #21576, .T. ) ;
#8223=CARTESIAN_POINT ( 'NONE',  ( 95.00000000000000000, -213.0599564267049857, 83.25312500173430408 ) ) ;
#8224=CARTESIAN_POINT ( 'NONE',  ( 94.99999999999998579, 86.94004357329500010, 85.71374999999997613 ) ) ;
#8226=DIRECTION ( 'NONE',  ( -1.000000000000000000, 0.000000000000000000, 0.000000000000000000 ) ) ;
#8230=CARTESIAN_POINT ( 'NONE',  ( -92.69370383062505425, 88.66845928578038638, 88.79614583420048746 ) ) ;
#8232=CARTESIAN_POINT ( 'NONE',  ( 96.15314808468748708, 88.00268892867053694, 80.32947916753380468 ) ) ;
#8233=VERTEX_POINT ( 'NONE', #51262 ) ;
#8234=CARTESIAN_POINT ( 'NONE',  ( 93.67499999999998295, 92.29496732002878900, 82.35354166840096468 ) ) ;
#8242=CARTESIAN_POINT ( 'NONE',  ( -0.0004442498525516064278, 0.001194404164626844313, -85.60000000000000853 ) ) ;
#8246=CARTESIAN_POINT ( 'NONE',  ( -92.35000000000005116, 88.47002178664754979, 83.27958333333333485 ) ) ;
#8249=EDGE_CURVE ( 'NONE', #48511, #46834, #32968, .T. ) ;
#8250=DIRECTION ( 'NONE',  ( -1.000000000000000000, 0.000000000000000000, 0.000000000000000000 ) ) ;
#8255=CARTESIAN_POINT ( 'NONE',  ( -93.84685191531247028, -211.9973110713294489, 82.23447916753380582 ) ) ;
#8269=CARTESIAN_POINT ( 'NONE',  ( -93.84685191531254134, 91.99731107132950569, 74.82614583420047438 ) ) ;
#8282=DIRECTION ( 'NONE',  ( -1.000000000000000000, 0.000000000000000000, 0.000000000000000000 ) ) ;
#8283=CARTESIAN_POINT ( 'NONE',  ( 97.64999999999821512, 90.00000306648260562, 75.79187510780352000 ) ) ;
#8284=CARTESIAN_POINT ( 'NONE',  ( -97.64999999999994884, -211.5299782133524502, 89.41791666666667027 ) ) ;
#8285=AXIS2_PLACEMENT_3D ( 'NONE', #22170, #73285, #56004 ) ;
#8286=DIRECTION ( 'NONE',  ( 0.000000000000000000, 0.000000000000000000, 1.000000000000000000 ) ) ;
#8288=DIRECTION ( 'NONE',  ( -0.000000000000000000, -0.000000000000000000, 1.000000000000000000 ) ) ;
#8294=EDGE_CURVE ( 'NONE', #38969, #45116, #50524, .T. ) ;
#8305=CARTESIAN_POINT ( 'NONE',  ( 95.00000000000000000, -207.3369185715606307, 81.22906250086714408 ) ) ;
#8306=CARTESIAN_POINT ( 'NONE',  ( 97.30629616937498838, -211.3315407142195852, 86.89114583420048632 ) ) ;
#8308=CARTESIAN_POINT ( 'NONE',  ( -92.35000000000003695, 90.00000000000004263, 79.52249999999999375 ) ) ;
#8310=ORIENTED_EDGE ( 'NONE', *, *, #60357, .T. ) ;
#8313=CARTESIAN_POINT ( 'NONE',  ( -96.15314808468752972, 91.99731107132950569, 75.72572916753382799 ) ) ;
#8316=CARTESIAN_POINT ( 'NONE',  ( -94.99999999999997158, -213.0599564267049857, 87.69812500173429726 ) ) ;
#8321=FACE_OUTER_BOUND ( 'NONE', #28925, .T. ) ;
#8323=CARTESIAN_POINT ( 'NONE',  ( 95.00000000000000000, -213.0599564267049857, 86.34874999999999545 ) ) ;
#8330=ORIENTED_EDGE ( 'NONE', *, *, #16530, .F. ) ;
#8332=CARTESIAN_POINT ( 'NONE',  ( 97.30629616937498838, -211.3315407142195852, 79.74739583420047495 ) ) ;
#8337=CARTESIAN_POINT ( 'NONE',  ( 92.35000000000000853, -209.9999999999999716, 90.00000000000000000 ) ) ;
#8343=CARTESIAN_POINT ( 'NONE',  ( -93.84685191531248449, -208.0026889286704943, 80.54114583420046358 ) ) ;
#8344=CARTESIAN_POINT ( 'NONE',  ( -92.69370383062502583, 88.66845928578038638, 78.00114583420049996 ) ) ;
#8345=EDGE_CURVE ( 'NONE', #12034, #17937, #50513, .T. ) ;
#8347=EDGE_CURVE ( 'NONE', #27953, #70455, #53190, .T. ) ;
#8348=CARTESIAN_POINT ( 'NONE',  ( 93.84685191531248449, 91.99731107132950569, 80.64697916753381435 ) ) ;
#8355=CARTESIAN_POINT ( 'NONE',  ( -93.84685191531247028, -211.9973110713294489, 82.23447916753380582 ) ) ;
#8358=CARTESIAN_POINT ( 'NONE',  ( 96.32499999999998863, 87.70503267997126784, 87.03666666666666174 ) ) ;
#8363=CIRCLE ( 'NONE', #40838, 2.649999999999985700 ) ;
#8367=VECTOR ( 'NONE', #47323, 1000.000000000000000 ) ;
#8368=CARTESIAN_POINT ( 'NONE',  ( -95.00000000000002842, 93.05995642670501411, 75.87125000000000341 ) ) ;
#8370=CARTESIAN_POINT ( 'NONE',  ( -95.00000000000002842, 92.66308142843932671, 85.67406250086715147 ) ) ;
#8378=DIRECTION ( 'NONE',  ( -0.000000000000000000, -0.000000000000000000, 1.000000000000000000 ) ) ;
#8381=CARTESIAN_POINT ( 'NONE',  ( -93.84685191531248449, -208.0026889286704943, 81.33489583420049485 ) ) ;
#8384=( BOUNDED_CURVE ( )  B_SPLINE_CURVE ( 2, ( #17450, #67847, #17088, #40378, #63330, #11792, #29088, #73096, #38905, #61842, #10325 ),
 .UNSPECIFIED., .F., .F. ) 
 B_SPLINE_CURVE_WITH_KNOTS ( ( 3, 2, 2, 2, 2, 3 ),
 ( 0.6985206468843491168, 0.6985207885473545542, 0.7055765540882368292, 0.7126323196291192152, 0.7196880851700017123, 0.7196881748034549275 ),
 .UNSPECIFIED. ) 
 CURVE ( )  GEOMETRIC_REPRESENTATION_ITEM ( )  RATIONAL_B_SPLINE_CURVE ( ( 0.9999946203249591159, 0.9999973101084729254, 1.000000000000000000, 0.8660254037844387076, 1.000000000000000000, 0.8660254037844387076, 1.000000000000000000, 0.8660254037844387076, 1.000000000000000000, 0.9999982980435457858, 0.9999965961303334261 ) ) 
 REPRESENTATION_ITEM ( '' )  );
#8389=CARTESIAN_POINT ( 'NONE',  ( -92.35000000000003695, 90.00000000000004263, 89.04749999999999943 ) ) ;
#8391=CARTESIAN_POINT ( 'NONE',  ( -97.64999999996715019, 90.00000839192523472, 86.90410584365564262 ) ) ;
#8399=CARTESIAN_POINT ( 'NONE',  ( 97.30629616937498838, -209.9999999999999716, 89.48406250086715374 ) ) ;
#8403=( BOUNDED_CURVE ( )  B_SPLINE_CURVE ( 2, ( #71852, #43326, #14721 ),
 .UNSPECIFIED., .F., .F. ) 
 B_SPLINE_CURVE_WITH_KNOTS ( ( 3, 3 ),
 ( 0.000000000000000000, 2.334341054542201936E-05 ),
 .UNSPECIFIED. ) 
 CURVE ( )  GEOMETRIC_REPRESENTATION_ITEM ( )  RATIONAL_B_SPLINE_CURVE ( ( 0.9459494467533910989, 0.9464399322878964682, 0.9469490141588171594 ) ) 
 REPRESENTATION_ITEM ( '' )  );
#8408=FACE_BOUND ( 'NONE', #72335, .T. ) ;
#8409=AXIS2_PLACEMENT_3D ( 'NONE', #1120, #19097, #42044 ) ;
#8413=ORIENTED_EDGE ( 'NONE', *, *, #46782, .T. ) ;
#8421=CARTESIAN_POINT ( 'NONE',  ( 97.30629616937498838, 91.33154071421968467, 80.64697916753382856 ) ) ;
#8422=CARTESIAN_POINT ( 'NONE',  ( 93.67500000000001137, -212.2949673200287179, 88.91520833506763211 ) ) ;
#8424=CARTESIAN_POINT ( 'NONE',  ( -95.00000000000002842, 93.05995642670504253, 88.01562500173432113 ) ) ;
#8436=CARTESIAN_POINT ( 'NONE',  ( 97.64999999999996305, 90.00000034979572661, 77.69687501385438111 ) ) ;
#8439=FACE_OUTER_BOUND ( 'NONE', #58268, .T. ) ;
#8440=CARTESIAN_POINT ( 'NONE',  ( -92.34999999999999432, -208.4700217866474645, 75.84479166840098685 ) ) ;
#8443=CARTESIAN_POINT ( 'NONE',  ( 92.34999999999999432, 91.52997821335252127, 76.69145833506763665 ) ) ;
#8444=CARTESIAN_POINT ( 'NONE',  ( -95.00000000000002842, 93.05995642670501411, 77.85562500173429612 ) ) ;
#8446=CARTESIAN_POINT ( 'NONE',  ( 93.84685191531248449, 91.99731107132950569, 76.99572916753382401 ) ) ;
#8447=DIRECTION ( 'NONE',  ( 1.000000000000000000, 0.000000000000000000, 0.000000000000000000 ) ) ;
#8453=ORIENTED_EDGE ( 'NONE', *, *, #49611, .F. ) ;
#8458=EDGE_LOOP ( 'NONE', ( #46686, #65680, #11942, #3063 ) ) ;
#8462=CARTESIAN_POINT ( 'NONE',  ( 96.32499999999998863, -207.7050326799711968, 87.96270833506763154 ) ) ;
#8465=CARTESIAN_POINT ( 'NONE',  ( -92.69370383062498320, -209.9999999999999716, 75.51406250086715488 ) ) ;
#8470=CARTESIAN_POINT ( 'NONE',  ( -93.67500000000003979, 92.29496732002878900, 78.99333333333332519 ) ) ;
#8479=CARTESIAN_POINT ( 'NONE',  ( 92.69370383062498320, 88.66845928578035796, 84.77447916753381207 ) ) ;
#8480=CARTESIAN_POINT ( 'NONE',  ( -92.69370383062498320, -208.6684592857803295, 84.45697916753383083 ) ) ;
#8483=FACE_BOUND ( 'NONE', #18030, .T. ) ;
#8484=CARTESIAN_POINT ( 'NONE',  ( -97.64999999999994884, -208.4700217866474645, 77.88208333333332689 ) ) ;
#8490=CARTESIAN_POINT ( 'NONE',  ( 95.00000000000000000, -207.3369185715606307, 83.13406250086714522 ) ) ;
#8497=VECTOR ( 'NONE', #56924, 1000.000000000000000 ) ;
#8500=EDGE_CURVE ( 'NONE', #66667, #26840, #18062, .T. ) ;
#8502=CARTESIAN_POINT ( 'NONE',  ( 97.30629616937498838, -209.9999999999999716, 78.68906250086715204 ) ) ;
#8508=CARTESIAN_POINT ( 'NONE',  ( 97.64999999999997726, -211.5299782133524502, 81.37458333333333371 ) ) ;
#8514=CARTESIAN_POINT ( 'NONE',  ( -0.0004442498525516064278, 0.001194404164626844313, -64.00000000000000000 ) ) ;
#8520=CARTESIAN_POINT ( 'NONE',  ( -95.00000000000002842, 92.66308142843932671, 84.56281250086716739 ) ) ;
#8521=CARTESIAN_POINT ( 'NONE',  ( 92.34999999999999432, 90.00000000000002842, 89.44437500173430067 ) ) ;
#8526=DIRECTION ( 'NONE',  ( 1.000000000000000000, 0.000000000000000000, 0.000000000000000000 ) ) ;
#8528=CARTESIAN_POINT ( 'NONE',  ( -97.64999999999994884, -211.5299782133524502, 84.41729166840097776 ) ) ;
#8529=ORIENTED_EDGE ( 'NONE', *, *, #64256, .F. ) ;
#8531=ORIENTED_EDGE ( 'NONE', *, *, #65099, .F. ) ;
#8532=CARTESIAN_POINT ( 'NONE',  ( -95.00000000000002842, 86.94004357329504273, 85.15812500173430521 ) ) ;
#8534=CARTESIAN_POINT ( 'NONE',  ( 96.15314808468748708, 88.00268892867053694, 86.83822916753382515 ) ) ;
#8548=CARTESIAN_POINT ( 'NONE',  ( -92.69370383062498320, -208.6684592857803011, 85.72697916753381264 ) ) ;
#8553=VECTOR ( 'NONE', #71607, 1000.000000000000000 ) ;
#8557=CARTESIAN_POINT ( 'NONE',  ( 94.99999999999998579, 92.66308142843932671, 78.68906250086713783 ) ) ;
#8560=CARTESIAN_POINT ( 'NONE',  ( 92.35000000000000853, -209.9999999999999716, 90.00000000000000000 ) ) ;
#8561=CARTESIAN_POINT ( 'NONE',  ( 93.26435506835481704, 91.73956328105560942, 74.87701898318917415 ) ) ;
#8562=CARTESIAN_POINT ( 'NONE',  ( -97.65000000000001990, 88.47002178664754979, 76.79729166840095900 ) ) ;
#8570=CARTESIAN_POINT ( 'NONE',  ( -92.69370383062505425, 88.66845928578038638, 84.19239583420048234 ) ) ;
#8572=CARTESIAN_POINT ( 'NONE',  ( 92.35000000045006630, 89.99996890530464100, 88.81037122970248276 ) ) ;
#8579=EDGE_CURVE ( 'NONE', #16867, #50672, #70769, .T. ) ;
#8583=CARTESIAN_POINT ( 'NONE',  ( 97.30629616937498838, -208.6684592857803011, 78.10697916753383652 ) ) ;
#8589=FACE_OUTER_BOUND ( 'NONE', #69836, .T. ) ;
#8593=CARTESIAN_POINT ( 'NONE',  ( 92.69370383062501162, -208.6684592857803011, 77.04864583420048518 ) ) ;
#8607=CARTESIAN_POINT ( 'NONE',  ( 97.64999999999997726, -208.4700217866474645, 82.19479166840095274 ) ) ;
#8608=CARTESIAN_POINT ( 'NONE',  ( 92.34999999999999432, 88.47002178664753558, 84.33791666666667197 ) ) ;
#8612=CARTESIAN_POINT ( 'NONE',  ( -92.35000000035631729, -210.0000434577671911, 89.12687334326093946 ) ) ;
#8615=( BOUNDED_CURVE ( )  B_SPLINE_CURVE ( 2, ( #74164, #62157, #10644, #56894, #68162, #5029, #73788, #22679, #67042 ),
 .UNSPECIFIED., .F., .F. ) 
 B_SPLINE_CURVE_WITH_KNOTS ( ( 3, 2, 2, 2, 3 ),
 ( 0.7620226289464454572, 0.7620226784152968058, 0.7690784439561787478, 0.7761342094970608008, 0.7831899741065913023 ),
 .UNSPECIFIED. ) 
 CURVE ( )  GEOMETRIC_REPRESENTATION_ITEM ( )  RATIONAL_B_SPLINE_CURVE ( ( 0.9999981213879984843, 0.9999990606874136212, 1.000000000000000000, 0.8660254037844387076, 1.000000000000000000, 0.8660254037844387076, 1.000000000000000000, 0.8660254037844387076, 1.000000000000000000 ) ) 
 REPRESENTATION_ITEM ( '' )  );
#8616=CARTESIAN_POINT ( 'NONE',  ( -93.84685191531252713, 88.00268892867056536, 89.37822916753381719 ) ) ;
#8617=CARTESIAN_POINT ( 'NONE',  ( 97.30629616937498838, 88.66845928578037217, 82.92239583420045790 ) ) ;
#8619=CARTESIAN_POINT ( 'NONE',  ( 93.67499999999999716, 87.70503267997126784, 81.93020833506763267 ) ) ;
#8621=VERTEX_POINT ( 'NONE', #15013 ) ;
#8622=CARTESIAN_POINT ( 'NONE',  ( 93.67500000000001137, -207.7050326799711968, 87.43354166840096298 ) ) ;
#8624=ORIENTED_EDGE ( 'NONE', *, *, #62784, .T. ) ;
#8631=CARTESIAN_POINT ( 'NONE',  ( -93.67500000000003979, 87.70503267997129626, 84.49666666666666970 ) ) ;
#8633=FACE_OUTER_BOUND ( 'NONE', #50559, .T. ) ;
#8635=ORIENTED_EDGE ( 'NONE', *, *, #71085, .T. ) ;
#8637=CARTESIAN_POINT ( 'NONE',  ( -92.69370383062498320, -211.3315407142195852, 79.11239583420046984 ) ) ;
#8638=ORIENTED_EDGE ( 'NONE', *, *, #70802, .F. ) ;
#8646=EDGE_CURVE ( 'NONE', #3079, #8233, #74011, .T. ) ;
#8650=CARTESIAN_POINT ( 'NONE',  ( -96.15314808468752972, 91.99731107132950569, 76.20197916753380696 ) ) ;
#8653=EDGE_CURVE ( 'NONE', #50612, #55000, #43170, .T. ) ;
#8654=CARTESIAN_POINT ( 'NONE',  ( 92.35000000000000853, -209.9999999999999716, 75.39499999999999602 ) ) ;
#8665=CARTESIAN_POINT ( 'NONE',  ( -92.34999999999999432, -209.9999999999999716, 89.68250000000000455 ) ) ;
#8666=DIRECTION ( 'NONE',  ( 1.000000000000000000, 0.000000000000000000, 0.000000000000000000 ) ) ;
#8670=FACE_OUTER_BOUND ( 'NONE', #12643, .T. ) ;
#8671=( NAMED_UNIT ( * ) SI_UNIT ( $, .STERADIAN. ) SOLID_ANGLE_UNIT ( ) );
#8676=EDGE_CURVE ( 'NONE', #39802, #31963, #48348, .T. ) ;
#8681=CARTESIAN_POINT ( 'NONE',  ( 92.69370383062501162, -208.6684592857803295, 83.23989583420048177 ) ) ;
#8682=CARTESIAN_POINT ( 'NONE',  ( 93.84685191531249870, -208.0026889286704943, 87.79072916753381151 ) ) ;
#8684=CARTESIAN_POINT ( 'NONE',  ( 97.30629616937498838, -211.3315407142195852, 86.25614583420048120 ) ) ;
#8687=VERTEX_POINT ( 'NONE', #4886 ) ;
#8688=CARTESIAN_POINT ( 'NONE',  ( -97.30629616937501680, 91.33154071421968467, 77.68364583420047609 ) ) ;
#8696=CYLINDRICAL_SURFACE ( 'NONE', #58636, 2.649999999999985700 ) ;
#8698=ORIENTED_EDGE ( 'NONE', *, *, #49162, .F. ) ;
#8702=CARTESIAN_POINT ( 'NONE',  ( 96.15314808468750130, -211.9973110713294489, 77.15447916753380753 ) ) ;
#8705=DIRECTION ( 'NONE',  ( -0.000000000000000000, -0.000000000000000000, 1.000000000000000000 ) ) ;
#8709=DIRECTION ( 'NONE',  ( -0.000000000000000000, -0.000000000000000000, 1.000000000000000000 ) ) ;
#8713=CARTESIAN_POINT ( 'NONE',  ( -97.30629616937495996, -209.9999999999999716, 79.48281250086714067 ) ) ;
#8714=CARTESIAN_POINT ( 'NONE',  ( -92.69370383062502583, 88.66845928578038638, 78.63614583420049087 ) ) ;
#8718=CARTESIAN_POINT ( 'NONE',  ( 93.84685191531248449, 88.00268892867053694, 77.68364583420047609 ) ) ;
#8720=ORIENTED_EDGE ( 'NONE', *, *, #51959, .F. ) ;
#8722=CARTESIAN_POINT ( 'NONE',  ( -92.69370383062498320, -208.6684592857803011, 88.74322916753379786 ) ) ;
#8726=CARTESIAN_POINT ( 'NONE',  ( -94.99999999999997158, -207.3369185715606307, 84.40406250086714124 ) ) ;
#8739=CARTESIAN_POINT ( 'NONE',  ( -97.30629616937501680, 88.66845928578038638, 86.52072916753381548 ) ) ;
#8750=CARTESIAN_POINT ( 'NONE',  ( 97.64999999999997726, -208.4700217866474929, 84.65541666666669585 ) ) ;
#8752=CARTESIAN_POINT ( 'NONE',  ( -92.69370383062498320, -211.3315407142195852, 84.35114583420049428 ) ) ;
#8757=CARTESIAN_POINT ( 'NONE',  ( 97.64999999999999147, -209.9999999999999716, 90.00000000000000000 ) ) ;
#8758=CARTESIAN_POINT ( 'NONE',  ( -95.00000000000002842, 86.94004357329504273, 88.88875000000000171 ) ) ;
#8761=CARTESIAN_POINT ( 'NONE',  ( -92.35000000000017906, 91.52997821335260653, 78.30541666666667311 ) ) ;
#8764=CYLINDRICAL_SURFACE ( 'NONE', #69696, 2.649999999999999467 ) ;
#8766=EDGE_CURVE ( 'NONE', #32709, #59366, #9482, .T. ) ;
#8767=CARTESIAN_POINT ( 'NONE',  ( 92.34999999999998010, 90.00000928824103141, 86.90437468048608594 ) ) ;
#8782=ORIENTED_EDGE ( 'NONE', *, *, #47473, .F. ) ;
#8783=ORIENTED_EDGE ( 'NONE', *, *, #39012, .F. ) ;
#8784=CARTESIAN_POINT ( 'NONE',  ( 94.99999999999998579, 92.66308142843935514, 80.11781250086714579 ) ) ;
#8787=CARTESIAN_POINT ( 'NONE',  ( -92.35000000000003695, 89.99999996655868983, 87.85687500050293863 ) ) ;
#8790=ORIENTED_EDGE ( 'NONE', *, *, #30732, .T. ) ;
#8800=CARTESIAN_POINT ( 'NONE',  ( -97.64999999999994884, -208.4700217866474645, 74.78645833506763552 ) ) ;
#8801=CARTESIAN_POINT ( 'NONE',  ( -92.69370383062502583, 88.66845928578038638, 88.79614583420050167 ) ) ;
#8805=CARTESIAN_POINT ( 'NONE',  ( 93.67499999999998295, 92.29496732002878900, 74.73354166840096013 ) ) ;
#8806=CARTESIAN_POINT ( 'NONE',  ( -97.30629616937501680, 90.00000000000004263, 89.00781250086714635 ) ) ;
#8808=CARTESIAN_POINT ( 'NONE',  ( 92.69370383062498320, 90.00000000000002842, 75.83156250086716454 ) ) ;
#8809=CYLINDRICAL_SURFACE ( 'NONE', #24176, 2.649999999999985700 ) ;
#8810=CARTESIAN_POINT ( 'NONE',  ( 97.64999999999999147, -209.9999999999999716, 87.77749999999998920 ) ) ;
#8817=EDGE_LOOP ( 'NONE', ( #3291, #57455, #4393, #58189, #57552 ) ) ;
#8826=CARTESIAN_POINT ( 'NONE',  ( -92.35000000000005116, 88.47002178664754979, 76.37395833506761278 ) ) ;
#8827=( BOUNDED_CURVE ( )  B_SPLINE_CURVE ( 2, ( #9622, #15254, #26531, #20893, #73128, #22010, #56228 ),
 .UNSPECIFIED., .F., .F. ) 
 B_SPLINE_CURVE_WITH_KNOTS ( ( 3, 2, 2, 3 ),
 ( 0.04166666666666644231, 0.04861111111111085514, 0.05555555555555525410, 0.06249999999999966693 ),
 .UNSPECIFIED. ) 
 CURVE ( )  GEOMETRIC_REPRESENTATION_ITEM ( )  RATIONAL_B_SPLINE_CURVE ( ( 1.000000000000004219, 0.8660254037844343777, 1.000000000000000000, 0.8660254037844387076, 1.000000000000000000, 0.8660254037844451469, 0.9999999999999935607 ) ) 
 REPRESENTATION_ITEM ( '' )  );
#8828=CARTESIAN_POINT ( 'NONE',  ( 94.99999999999998579, 86.94004357329502852, 84.44374999999999432 ) ) ;
#8831=EDGE_CURVE ( 'NONE', #54767, #29022, #53616, .T. ) ;
#8841=DIRECTION ( 'NONE',  ( 0.000000000000000000, 0.000000000000000000, 1.000000000000000000 ) ) ;
#8843=CARTESIAN_POINT ( 'NONE',  ( -97.64999999998384794, -210.0000060634594661, 88.17456390440159453 ) ) ;
#8846=CARTESIAN_POINT ( 'NONE',  ( 92.69370383062498320, 88.66845928578035796, 82.86947916753379673 ) ) ;
#8848=CARTESIAN_POINT ( 'NONE',  ( -97.30629616937495996, -209.9999999999999716, 82.18156250086715886 ) ) ;
#8852=CARTESIAN_POINT ( 'NONE',  ( -97.64999999999994884, -208.4700217866474645, 79.15208333333332291 ) ) ;
#8855=CARTESIAN_POINT ( 'NONE',  ( 97.30629616937498838, -211.3315407142195852, 82.92239583420045790 ) ) ;
#8866=CARTESIAN_POINT ( 'NONE',  ( 97.30629616937498838, -211.3315407142195852, 77.36614583420048064 ) ) ;
#8868=CYLINDRICAL_SURFACE ( 'NONE', #1619, 2.649999999999985700 ) ;
#8872=CARTESIAN_POINT ( 'NONE',  ( -93.67500000000003979, 87.70503267997129626, 83.30604166840096525 ) ) ;
#8873=CARTESIAN_POINT ( 'NONE',  ( 92.35000000000002274, -211.5299782133524502, 83.06791666666664753 ) ) ;
#8875=ORIENTED_EDGE ( 'NONE', *, *, #56089, .F. ) ;
#8879=LINE ( 'NONE', #47618, #59863 ) ;
#8881=CARTESIAN_POINT ( 'NONE',  ( -93.84685191531254134, 91.99731107132950569, 82.60489583420049087 ) ) ;
#8887=CARTESIAN_POINT ( 'NONE',  ( -92.34999999999999432, -209.9999999999999716, 86.58687500173429896 ) ) ;
#8891=CARTESIAN_POINT ( 'NONE',  ( -96.32500000000001705, 87.70503267997129626, 82.56520833506762358 ) ) ;
#8893=CARTESIAN_POINT ( 'NONE',  ( 93.84685191531248449, 91.99731107132950569, 87.79072916753381151 ) ) ;
#8899=CARTESIAN_POINT ( 'NONE',  ( 97.65000000000006253, 88.47002178664757821, 88.99458333333333826 ) ) ;
#8908=DIRECTION ( 'NONE',  ( -3.061616997868382648E-16, -1.000000000000000000, 0.000000000000000000 ) ) ;
#8914=CARTESIAN_POINT ( 'NONE',  ( -96.15314808468745866, -211.9973110713294489, 85.46239583420047836 ) ) ;
#8916=DIRECTION ( 'NONE',  ( 1.000000000000000000, 0.000000000000000000, 0.000000000000000000 ) ) ;
#8922=CARTESIAN_POINT ( 'NONE',  ( 96.15314808468748708, 88.00268892867053694, 76.51947916753380241 ) ) ;
#8932=DIRECTION ( 'NONE',  ( -1.000000000000000000, 0.000000000000000000, -0.000000000000000000 ) ) ;
#8935=CARTESIAN_POINT ( 'NONE',  ( -92.69370383062505425, 91.33154071421968467, 81.75822916753381264 ) ) ;
#8938=ADVANCED_FACE ( 'NONE', ( #24734, #59318 ), #19457, .T. ) ;
#8942=EDGE_CURVE ( 'NONE', #16444, #57918, #44634, .T. ) ;
#8950=CARTESIAN_POINT ( 'NONE',  ( 92.69370383062501162, -208.6684592857803011, 80.22364583420048234 ) ) ;
#8958=CARTESIAN_POINT ( 'NONE',  ( 92.69370383062501162, -208.6684592857803011, 76.41364583420049428 ) ) ;
#8961=VERTEX_POINT ( 'NONE', #49871 ) ;
#8962=ORIENTED_EDGE ( 'NONE', *, *, #61110, .T. ) ;
#8963=CARTESIAN_POINT ( 'NONE',  ( -97.65000000000001990, 90.00000000000004263, 83.01499999999998636 ) ) ;
#8969=CARTESIAN_POINT ( 'NONE',  ( 93.67500000000001137, -212.2949673200287179, 81.29520833506762756 ) ) ;
#8970=CARTESIAN_POINT ( 'NONE',  ( 97.64999999999997726, 91.52997821335252127, 84.65541666666666742 ) ) ;
#8973=CARTESIAN_POINT ( 'NONE',  ( 2.499999999999979572, -90.00000000000000000, -310.0000000000000000 ) ) ;
#8976=CARTESIAN_POINT ( 'NONE',  ( -92.69370383062504004, 90.00000000000004263, 86.94406250086716170 ) ) ;
#8977=CARTESIAN_POINT ( 'NONE',  ( 97.30629616937498838, 91.33154071421968467, 81.75822916753381264 ) ) ;
#8978=VECTOR ( 'NONE', #50862, 1000.000000000000000 ) ;
#8980=CARTESIAN_POINT ( 'NONE',  ( 97.64999999999999147, 90.00000000000002842, 81.50687500173430067 ) ) ;
#8986=ORIENTED_EDGE ( 'NONE', *, *, #40752, .T. ) ;
#8992=CARTESIAN_POINT ( 'NONE',  ( -94.99999999999997158, -209.9999999999999716, 90.00000000000000000 ) ) ;
#8993=CARTESIAN_POINT ( 'NONE',  ( 96.32499999999997442, 92.29496732002878900, 87.96270833506763154 ) ) ;
#8996=CARTESIAN_POINT ( 'NONE',  ( -96.15314808468745866, -211.9973110713294489, 80.22364583420046813 ) ) ;
#9002=CARTESIAN_POINT ( 'NONE',  ( -92.34999999999998010, -210.0000217321222635, 89.12687425009517028 ) ) ;
#9006=CARTESIAN_POINT ( 'NONE',  ( 96.15314808468748708, 88.00268892867053694, 88.58447916753381435 ) ) ;
#9014=CARTESIAN_POINT ( 'NONE',  ( 94.99999999999998579, 86.94004357329502852, 76.18874999999999886 ) ) ;
#9015=DIRECTION ( 'NONE',  ( 1.000000000000000000, 0.000000000000000000, 0.000000000000000000 ) ) ;
#9016=DIRECTION ( 'NONE',  ( -0.000000000000000000, -0.000000000000000000, 1.000000000000000000 ) ) ;
#9017=DIRECTION ( 'NONE',  ( -0.000000000000000000, -0.000000000000000000, 1.000000000000000000 ) ) ;
#9018=DIRECTION ( 'NONE',  ( 1.000000000000000000, 0.000000000000000000, 0.000000000000000000 ) ) ;
#9020=EDGE_CURVE ( 'NONE', #56782, #32186, #28158, .T. ) ;
#9023=CARTESIAN_POINT ( 'NONE',  ( -96.32499999999996021, -212.2949673200287179, 88.83583333333334053 ) ) ;
#9039=( BOUNDED_CURVE ( )  B_SPLINE_CURVE ( 2, ( #44345, #32299, #20666, #55987, #4139, #43617, #15388, #9758, #56375 ),
 .UNSPECIFIED., .F., .F. ) 
 B_SPLINE_CURVE_WITH_KNOTS ( ( 3, 2, 2, 2, 3 ),
 ( 0.1058364832022826857, 0.1128922486541179271, 0.1199480141950002854, 0.1270037797358826437, 0.1270039290051391268 ),
 .UNSPECIFIED. ) 
 CURVE ( )  GEOMETRIC_REPRESENTATION_ITEM ( )  RATIONAL_B_SPLINE_CURVE ( ( 1.000000000000000000, 0.8660254037844387076, 1.000000000000000000, 0.8660254037844387076, 1.000000000000000000, 0.8660254037844387076, 1.000000000000000000, 0.9999971656812787213, 0.9999943314824810692 ) ) 
 REPRESENTATION_ITEM ( '' )  );
#9040=CARTESIAN_POINT ( 'NONE',  ( 95.00000000000000000, -212.6630814284392557, 82.81656250086712134 ) ) ;
#9041=CARTESIAN_POINT ( 'NONE',  ( 93.84685191531251292, -211.9973110713294489, 84.19239583420049655 ) ) ;
#9044=CARTESIAN_POINT ( 'NONE',  ( 97.30629616937498838, -209.9999999999999716, 86.94406250086716170 ) ) ;
#9045=EDGE_LOOP ( 'NONE', ( #64652, #1106, #70017 ) ) ;
#9047=ORIENTED_EDGE ( 'NONE', *, *, #73510, .F. ) ;
#9048=CARTESIAN_POINT ( 'NONE',  ( -96.15314808468751551, 88.00268892867056536, 76.57239583420049200 ) ) ;
#9051=ORIENTED_EDGE ( 'NONE', *, *, #52128, .F. ) ;
#9060=CARTESIAN_POINT ( 'NONE',  ( 95.00000000000000000, -213.0599564267049857, 81.34812500173430294 ) ) ;
#9065=CARTESIAN_POINT ( 'NONE',  ( 92.69370383062501162, -208.6684592857803011, 80.06489583420047040 ) ) ;
#9069=EDGE_LOOP ( 'NONE', ( #46542, #23231 ) ) ;
#9070=VERTEX_POINT ( 'NONE', #54786 ) ;
#9074=CARTESIAN_POINT ( 'NONE',  ( 97.64999999999999147, 90.00000000000002842, 90.00000000000000000 ) ) ;
#9076=CARTESIAN_POINT ( 'NONE',  ( -96.15314808468752972, 91.99731107132950569, 78.26572916753382003 ) ) ;
#9077=VERTEX_POINT ( 'NONE', #73179 ) ;
#9078=CARTESIAN_POINT ( 'NONE',  ( 93.84685191531248449, 91.99731107132950569, 78.10697916753380809 ) ) ;
#9087=CARTESIAN_POINT ( 'NONE',  ( -93.84685191531247028, -211.9973110713294489, 84.13947916753380696 ) ) ;
#9095=DIRECTION ( 'NONE',  ( -0.000000000000000000, -0.000000000000000000, 1.000000000000000000 ) ) ;
#9096=CARTESIAN_POINT ( 'NONE',  ( 96.32499999999997442, 92.29496732002878900, 84.70833333333332860 ) ) ;
#9100=CARTESIAN_POINT ( 'NONE',  ( -97.30629616937501680, 91.33154071421968467, 85.14489583420048291 ) ) ;
#9110=CARTESIAN_POINT ( 'NONE',  ( -94.99999999999997158, -209.9999999999999716, 90.00000000000000000 ) ) ;
#9113=CARTESIAN_POINT ( 'NONE',  ( -97.30629616937497417, -208.6684592857803011, 84.03364583420049883 ) ) ;
#9115=CARTESIAN_POINT ( 'NONE',  ( -92.34999999999999432, -211.5299782133524218, 87.16895833506762870 ) ) ;
#9117=CARTESIAN_POINT ( 'NONE',  ( 2.500000000000029754, 73.00000000000001421, -208.2999999999999261 ) ) ;
#9125=CARTESIAN_POINT ( 'NONE',  ( -97.64998530153629019, 91.52998669951453792, 76.05645774805350356 ) ) ;
#9128=CARTESIAN_POINT ( 'NONE',  ( 97.65000000000009095, -208.4700217866475214, 85.92541666666664923 ) ) ;
#9133=CARTESIAN_POINT ( 'NONE',  ( -2.500000000000015543, -73.00000000000001421, -201.6999999999999602 ) ) ;
#9147=CARTESIAN_POINT ( 'NONE',  ( 96.15314808468748708, 91.99731107132950569, 75.61989583420049144 ) ) ;
#9148=FACE_BOUND ( 'NONE', #9069, .T. ) ;
#9149=CARTESIAN_POINT ( 'NONE',  ( -100.0000000000000142, 85.00000000000002842, 90.00000000000000000 ) ) ;
#9154=FACE_OUTER_BOUND ( 'NONE', #32063, .T. ) ;
#9156=CARTESIAN_POINT ( 'NONE',  ( 97.64999999999999147, -211.0689600337108516, 74.48490336299447279 ) ) ;
#9160=DIRECTION ( 'NONE',  ( -0.000000000000000000, -0.000000000000000000, 1.000000000000000000 ) ) ;
#9165=CARTESIAN_POINT ( 'NONE',  ( -93.67499999999998295, -212.2949673200287179, 75.68604166840097491 ) ) ;
#9166=CARTESIAN_POINT ( 'NONE',  ( -92.69370383062502583, 91.33154071421968467, 88.90197916753382401 ) ) ;
#9169=CARTESIAN_POINT ( 'NONE',  ( 94.99999999999998579, 87.33691857156068750, 88.53156250086713897 ) ) ;
#9170=CARTESIAN_POINT ( 'NONE',  ( -97.30629616937501680, 88.66845928578038638, 88.42572916753380241 ) ) ;
#9172=CARTESIAN_POINT ( 'NONE',  ( 97.30629616937498838, 88.66845928578037217, 76.73114583420048973 ) ) ;
#9175=LINE ( 'NONE', #13698, #6676 ) ;
#9184=CARTESIAN_POINT ( 'NONE',  ( -95.00000000000002842, 86.94004357329504273, 80.63375000000000625 ) ) ;
#9190=CARTESIAN_POINT ( 'NONE',  ( 96.32499999999997442, 92.29496732002878900, 87.32770833506762642 ) ) ;
#9196=CARTESIAN_POINT ( 'NONE',  ( -97.30629616937501680, 90.00000000000004263, 81.38781250086714181 ) ) ;
#9197=CARTESIAN_POINT ( 'NONE',  ( 96.32499999999998863, 87.70503267997126784, 82.67104166840096013 ) ) ;
#9207=CARTESIAN_POINT ( 'NONE',  ( 96.15314808468748708, 91.99731107132950569, 80.69989583420047552 ) ) ;
#9208=CARTESIAN_POINT ( 'NONE',  ( -96.15314808468745866, -211.9973110713294489, 83.55739583420049144 ) ) ;
#9209=LINE ( 'NONE', #3604, #39821 ) ;
#9212=CARTESIAN_POINT ( 'NONE',  ( -93.67499999999998295, -207.7050326799711968, 76.45333333333333314 ) ) ;
#9215=CARTESIAN_POINT ( 'NONE',  ( 93.84685191531249870, -208.0026889286704943, 83.18697916753382060 ) ) ;
#9218=ORIENTED_EDGE ( 'NONE', *, *, #11370, .T. ) ;
#9225=CARTESIAN_POINT ( 'NONE',  ( 95.00000000000000000, -207.3369185715606307, 78.21281250086717307 ) ) ;
#9226=EDGE_CURVE ( 'NONE', #26794, #60251, #25747, .T. ) ;
#9227=FACE_OUTER_BOUND ( 'NONE', #59026, .T. ) ;
#9229=CARTESIAN_POINT ( 'NONE',  ( -97.20211296432958648, 88.68334238502464473, 74.94590613650809985 ) ) ;
#9230=CARTESIAN_POINT ( 'NONE',  ( 92.69370383062498320, 90.00000000000002842, 85.99156250086716113 ) ) ;
#9232=LINE ( 'NONE', #37824, #47790 ) ;
#9233=CARTESIAN_POINT ( 'NONE',  ( 92.35000000000000853, -209.9999999999999716, 82.37999999999999545 ) ) ;
#9238=ORIENTED_EDGE ( 'NONE', *, *, #54631, .F. ) ;
#9242=CARTESIAN_POINT ( 'NONE',  ( -97.30629616937501680, 88.66845928578038638, 84.77447916753381207 ) ) ;
#9244=LINE ( 'NONE', #20899, #59064 ) ;
#9248=CYLINDRICAL_SURFACE ( 'NONE', #68029, 2.649999999999985700 ) ;
#9250=CARTESIAN_POINT ( 'NONE',  ( -96.32499999999996021, -212.2949673200287179, 85.74020833506763495 ) ) ;
#9256=CARTESIAN_POINT ( 'NONE',  ( -93.67500000000003979, 87.70503267997129626, 82.03604166840096923 ) ) ;
#9257=( BOUNDED_CURVE ( )  B_SPLINE_CURVE ( 2, ( #67211, #41597, #57056, #46143, #51395, #64539, #7013 ),
 .UNSPECIFIED., .F., .F. ) 
 B_SPLINE_CURVE_WITH_KNOTS ( ( 3, 2, 2, 3 ),
 ( 0.8541666666666666297, 0.8611111111111110494, 0.8680555555555554692, 0.8749999999999997780 ),
 .UNSPECIFIED. ) 
 CURVE ( )  GEOMETRIC_REPRESENTATION_ITEM ( )  RATIONAL_B_SPLINE_CURVE ( ( 1.000000000000000000, 0.8660254037844387076, 1.000000000000000000, 0.8660254037844387076, 1.000000000000000000, 0.8660254037844430375, 0.9999999999999956701 ) ) 
 REPRESENTATION_ITEM ( '' )  );
#9259=CARTESIAN_POINT ( 'NONE',  ( 92.69370383062498320, 88.66845928578037217, 85.40947916753380298 ) ) ;
#9264=CARTESIAN_POINT ( 'NONE',  ( -92.98549755320794930, 88.86758821614978388, 74.79348190356850523 ) ) ;
#9269=DIRECTION ( 'NONE',  ( 0.4565542962317865050, 0.000000000000000000, 0.8896955516311735312 ) ) ;
#9277=CARTESIAN_POINT ( 'NONE',  ( -94.99999999999997158, -212.6630814284392557, 86.15031250086714465 ) ) ;
#9278=ORIENTED_EDGE ( 'NONE', *, *, #51679, .T. ) ;
#9279=DIRECTION ( 'NONE',  ( -0.000000000000000000, -0.000000000000000000, 1.000000000000000000 ) ) ;
#9284=CARTESIAN_POINT ( 'NONE',  ( 92.69370383062498320, 91.33154071421968467, 79.42989583420047950 ) ) ;
#9286=CARTESIAN_POINT ( 'NONE',  ( 15.70000000000000284, -120.0000000000000000, -85.59999999999999432 ) ) ;
#9288=CARTESIAN_POINT ( 'NONE',  ( 93.65592807507074724, 92.02656496471888659, 74.86703477254887673 ) ) ;
#9291=VECTOR ( 'NONE', #25091, 1000.000000000000000 ) ;
#9292=DIRECTION ( 'NONE',  ( -3.061616997868382648E-16, -1.000000000000000000, 0.000000000000000000 ) ) ;
#9297=CARTESIAN_POINT ( 'NONE',  ( -92.69370383062504004, 90.00000000000004263, 84.24531250086714351 ) ) ;
#9303=CARTESIAN_POINT ( 'NONE',  ( 92.35000000010806787, -209.9999848944895007, 78.64888723592486031 ) ) ;
#9307=CARTESIAN_POINT ( 'NONE',  ( -94.99999999999997158, -209.9999999999999716, 90.00000000000000000 ) ) ;
#9308=CARTESIAN_POINT ( 'NONE',  ( 93.84685191531251292, -211.9973110713294489, 77.84239583420048803 ) ) ;
#9312=EDGE_CURVE ( 'NONE', #39397, #32442, #63778, .T. ) ;
#9314=DIRECTION ( 'NONE',  ( -0.000000000000000000, -0.000000000000000000, 1.000000000000000000 ) ) ;
#9318=CARTESIAN_POINT ( 'NONE',  ( 97.30629616937498838, -209.9999999999999716, 75.51406250086715488 ) ) ;
#9321=CARTESIAN_POINT ( 'NONE',  ( -96.32499999999996021, -207.7050326799711968, 87.98916666666666231 ) ) ;
#9323=ORIENTED_EDGE ( 'NONE', *, *, #29189, .T. ) ;
#9329=CARTESIAN_POINT ( 'NONE',  ( 95.00000000000000000, -206.9400435732949575, 81.66562500173431260 ) ) ;
#9330=CARTESIAN_POINT ( 'NONE',  ( 93.67499999999998295, 92.29496732002878900, 85.44916666666665606 ) ) ;
#9331=ORIENTED_EDGE ( 'NONE', *, *, #49334, .T. ) ;
#9333=CARTESIAN_POINT ( 'NONE',  ( 99.99999999999997158, -80.00000000000001421, -90.00000000000014211 ) ) ;
#9337=CARTESIAN_POINT ( 'NONE',  ( -95.00000000000002842, 87.33691857156074434, 86.15031250086717307 ) ) ;
#9339=CARTESIAN_POINT ( 'NONE',  ( 94.99999999999998579, 87.33691857156068750, 82.81656250086713555 ) ) ;
#9361=CARTESIAN_POINT ( 'NONE',  ( -97.30629616937497417, -211.3315407142195852, 80.17072916753379275 ) ) ;
#9363=CARTESIAN_POINT ( 'NONE',  ( -95.00000000000002842, 86.94004357329504273, 86.34874999999999545 ) ) ;
#9371=CARTESIAN_POINT ( 'NONE',  ( 96.15314808468748708, 88.00268892867053694, 87.31447916753380412 ) ) ;
#9374=CARTESIAN_POINT ( 'NONE',  ( 92.34999999999999432, 90.00003728274771220, 81.18937371225271704 ) ) ;
#9376=CARTESIAN_POINT ( 'NONE',  ( -92.34999999999999432, -209.9999999999999716, 87.77749999999998920 ) ) ;
#9384=CARTESIAN_POINT ( 'NONE',  ( 94.99999999999998579, 90.00000000000002842, 90.00000000000000000 ) ) ;
#9386=CARTESIAN_POINT ( 'NONE',  ( -94.99999999999997158, -209.9999999999999716, 90.00000000000000000 ) ) ;
#9387=CARTESIAN_POINT ( 'NONE',  ( -92.34999999999999432, -208.4700217866474645, 89.10041666666667481 ) ) ;
#9391=CARTESIAN_POINT ( 'NONE',  ( 95.00000000000000000, -213.0599564267049857, 78.17312500173430578 ) ) ;
#9392=FILL_AREA_STYLE ('',( #72173 ) ) ;
#9397=EDGE_CURVE ( 'NONE', #34217, #44790, #58484, .T. ) ;
#9404=DIRECTION ( 'NONE',  ( 0.000000000000000000, -0.000000000000000000, -1.000000000000000000 ) ) ;
#9406=CARTESIAN_POINT ( 'NONE',  ( 97.30629616937498838, -208.6684592857803295, 83.02822916753379445 ) ) ;
#9407=CARTESIAN_POINT ( 'NONE',  ( 92.69370383062501162, -211.3315407142195852, 84.77447916753381207 ) ) ;
#9408=EDGE_LOOP ( 'NONE', ( #5675, #64520, #68726, #3996, #73997, #51818, #74117, #71005 ) ) ;
#9409=CARTESIAN_POINT ( 'NONE',  ( 97.30629616937498838, -208.6684592857803011, 87.63197916753382799 ) ) ;
#9412=CARTESIAN_POINT ( 'NONE',  ( 97.64999999994533653, 89.99998298270493535, 88.49187441316099978 ) ) ;
#9414=CARTESIAN_POINT ( 'NONE',  ( -92.69370383062504004, 90.00000000000004263, 77.41906250086715602 ) ) ;
#9430=CARTESIAN_POINT ( 'NONE',  ( 97.64999999999324132, 90.00000598221777182, 82.14187520865721126 ) ) ;
#9432=VERTEX_POINT ( 'NONE', #72354 ) ;
#9433=ORIENTED_EDGE ( 'NONE', *, *, #55879, .F. ) ;
#9435=EDGE_CURVE ( 'NONE', #38100, #25802, #5126, .T. ) ;
#9437=FACE_BOUND ( 'NONE', #57516, .T. ) ;
#9444=CARTESIAN_POINT ( 'NONE',  ( -93.84685191531252713, 88.00268892867056536, 80.48822916753381662 ) ) ;
#9446=CARTESIAN_POINT ( 'NONE',  ( 94.99999999999998579, 92.66308142843935514, 77.41906250086714181 ) ) ;
#9454=CARTESIAN_POINT ( 'NONE',  ( -94.99999999999997158, -207.3369185715606307, 80.59406250086715318 ) ) ;
#9461=ORIENTED_EDGE ( 'NONE', *, *, #29715, .T. ) ;
#9463=CIRCLE ( 'NONE', #8285, 23.50000000000000355 ) ;
#9466=CARTESIAN_POINT ( 'NONE',  ( -93.84685191531252713, 88.00268892867056536, 80.96447916753380980 ) ) ;
#9474=AXIS2_PLACEMENT_3D ( 'NONE', #37836, #60403, #43112 ) ;
#9477=FACE_OUTER_BOUND ( 'NONE', #4951, .T. ) ;
#9478=CARTESIAN_POINT ( 'NONE',  ( -97.30629616937497417, -211.3315407142195852, 82.86947916753382515 ) ) ;
#9480=CARTESIAN_POINT ( 'NONE',  ( -97.64999999999996305, -209.9999907117602618, 86.90437468048614278 ) ) ;
#9482=( BOUNDED_CURVE ( )  B_SPLINE_CURVE ( 2, ( #5616, #57477, #11590, #34530, #5991, #23268, #64973 ),
 .UNSPECIFIED., .F., .F. ) 
 B_SPLINE_CURVE_WITH_KNOTS ( ( 3, 2, 2, 3 ),
 ( 0.1041666666666670182, 0.1111111111111114103, 0.1180555555555558161, 0.1250000000000002220 ),
 .UNSPECIFIED. ) 
 CURVE ( )  GEOMETRIC_REPRESENTATION_ITEM ( )  RATIONAL_B_SPLINE_CURVE ( ( 0.9999999999999933387, 0.8660254037844453689, 1.000000000000000000, 0.8660254037844387076, 1.000000000000000000, 0.8660254037844343777, 1.000000000000004219 ) ) 
 REPRESENTATION_ITEM ( '' )  );
#9483=ORIENTED_EDGE ( 'NONE', *, *, #59406, .F. ) ;
#9512=VERTEX_POINT ( 'NONE', #71231 ) ;
#9518=EDGE_CURVE ( 'NONE', #19568, #25068, #51446, .T. ) ;
#9522=CARTESIAN_POINT ( 'NONE',  ( 92.69370383062498320, 91.33154071421968467, 75.77864583420048916 ) ) ;
#9523=CARTESIAN_POINT ( 'NONE',  ( 0.000000000000000000, 0.000000000000000000, 90.00000000000000000 ) ) ;
#9531=CARTESIAN_POINT ( 'NONE',  ( 96.15314808468748708, -208.0026889286704943, 89.43114583420047836 ) ) ;
#9534=EDGE_CURVE ( 'NONE', #47366, #69481, #74267, .T. ) ;
#9537=CARTESIAN_POINT ( 'NONE',  ( -97.65000000000000568, 89.99996514701868477, 77.37937620717865173 ) ) ;
#9544=CARTESIAN_POINT ( 'NONE',  ( -93.67499999999998295, -207.7050326799711968, 75.89770833506763381 ) ) ;
#9547=CARTESIAN_POINT ( 'NONE',  ( 96.15314808468748708, 88.00268892867053694, 89.21947916753380525 ) ) ;
#9548=CARTESIAN_POINT ( 'NONE',  ( -97.30629616937501680, 88.66845928578038638, 87.15572916753380639 ) ) ;
#9550=CARTESIAN_POINT ( 'NONE',  ( 97.65000000000000568, -211.5299782133524218, 84.62895833506763665 ) ) ;
#9560=CARTESIAN_POINT ( 'NONE',  ( -92.35000000000005116, 88.47002178664754979, 81.37458333333333371 ) ) ;
#9562=CARTESIAN_POINT ( 'NONE',  ( 92.35001423713265467, -211.5299864331648223, 75.52729223699087413 ) ) ;
#9568=CARTESIAN_POINT ( 'NONE',  ( -97.30629616937501680, 90.00000000000004263, 80.75281250086715090 ) ) ;
#9572=CARTESIAN_POINT ( 'NONE',  ( 92.34999999999999432, 88.47002178664752137, 82.51229166840094820 ) ) ;
#9584=CARTESIAN_POINT ( 'NONE',  ( 94.99999999999998579, 87.33691857156068750, 81.07031250086716057 ) ) ;
#9586=CARTESIAN_POINT ( 'NONE',  ( -96.15314808468747287, -208.0026889286704943, 83.34572916753383254 ) ) ;
#9589=EDGE_LOOP ( 'NONE', ( #64936, #724, #69789, #22005 ) ) ;
#9591=CARTESIAN_POINT ( 'NONE',  ( -93.67499999999998295, -212.2949673200287179, 77.51166666666665606 ) ) ;
#9597=CARTESIAN_POINT ( 'NONE',  ( -92.69370383062504004, 90.00000000000004263, 76.78406250086715090 ) ) ;
#9598=CARTESIAN_POINT ( 'NONE',  ( 96.15314808468750130, -211.9973110713294489, 82.23447916753380582 ) ) ;
#9601=ORIENTED_EDGE ( 'NONE', *, *, #9955, .T. ) ;
#9602=EDGE_CURVE ( 'NONE', #50254, #18134, #62968, .T. ) ;
#9606=CARTESIAN_POINT ( 'NONE',  ( 92.69370383062501162, -209.9999999999999716, 75.83156250086716454 ) ) ;
#9607=ADVANCED_FACE ( 'NONE', ( #63317 ), #67836, .F. ) ;
#9610=CARTESIAN_POINT ( 'NONE',  ( -97.64999999960629395, 90.00002930740643592, 76.74344264317980446 ) ) ;
#9612=CARTESIAN_POINT ( 'NONE',  ( 92.69370383062498320, 90.00000000000002842, 87.26156250086715715 ) ) ;
#9616=CARTESIAN_POINT ( 'NONE',  ( 97.64999999999999147, -209.9999999999999716, 81.42749999999999488 ) ) ;
#9622=CARTESIAN_POINT ( 'NONE',  ( 92.35000000000000853, -209.9999999999999716, 89.36499999999999488 ) ) ;
#9624=CARTESIAN_POINT ( 'NONE',  ( 92.69370383062498320, 90.00000000000002842, 89.64281250086713726 ) ) ;
#9629=CARTESIAN_POINT ( 'NONE',  ( -92.34999999999999432, -211.5299782133524502, 86.53395833506763779 ) ) ;
#9633=CARTESIAN_POINT ( 'NONE',  ( -92.35000000000003695, 90.00000000000004263, 81.50687500173430067 ) ) ;
#9635=CARTESIAN_POINT ( 'NONE',  ( 97.30629616937498838, 91.33154071421968467, 83.18697916753382060 ) ) ;
#9643=CARTESIAN_POINT ( 'NONE',  ( 94.99999999999998579, 90.00000000000002842, 90.00000000000000000 ) ) ;
#9644=AXIS2_PLACEMENT_3D ( 'NONE', #56434, #38395, #37662 ) ;
#9650=ADVANCED_FACE ( 'NONE', ( #45290 ), #41127, .F. ) ;
#9654=CARTESIAN_POINT ( 'NONE',  ( -94.99999999999997158, -207.3369185715606307, 85.19781250086714408 ) ) ;
#9659=DIRECTION ( 'NONE',  ( -0.000000000000000000, -0.000000000000000000, -1.000000000000000000 ) ) ;
#9661=CARTESIAN_POINT ( 'NONE',  ( 97.30629616937498838, 91.33154071421968467, 77.94822916753381037 ) ) ;
#9665=DIRECTION ( 'NONE',  ( -0.000000000000000000, -0.000000000000000000, 1.000000000000000000 ) ) ;
#9666=CARTESIAN_POINT ( 'NONE',  ( 93.55421244156863736, 91.96030971134655374, 74.86947676125078033 ) ) ;
#9672=CARTESIAN_POINT ( 'NONE',  ( 92.35000000000000853, -209.9999999999999716, 78.57000000000000739 ) ) ;
#9673=CARTESIAN_POINT ( 'NONE',  ( 92.35000000000000853, 90.00003217427531865, 76.74437388893713319 ) ) ;
#9676=CARTESIAN_POINT ( 'NONE',  ( -97.30629616937501680, 90.00000000000004263, 82.02281250086714692 ) ) ;
#9681=CYLINDRICAL_SURFACE ( 'NONE', #66678, 2.649999999999999467 ) ;
#9686=CARTESIAN_POINT ( 'NONE',  ( 94.99999999999998579, 86.94004357329502852, 83.25312500173430408 ) ) ;
#9687=CARTESIAN_POINT ( 'NONE',  ( 92.69370383062501162, -208.6684592857803011, 78.31864583420050963 ) ) ;
#9697=( BOUNDED_CURVE ( )  B_SPLINE_CURVE ( 2, ( #53096, #41806, #65862, #54213, #12855, #19976, #42931, #71476, #14347, #59477, #36530 ),
 .UNSPECIFIED., .F., .F. ) 
 B_SPLINE_CURVE_WITH_KNOTS ( ( 3, 2, 2, 2, 2, 3 ),
 ( 0.04233441017615420521, 0.04233459324550207376, 0.04939035878641885591, 0.05644612432733563112, 0.06350188986825240633, 0.06350193517771154927 ),
 .UNSPECIFIED. ) 
 CURVE ( )  GEOMETRIC_REPRESENTATION_ITEM ( )  RATIONAL_B_SPLINE_CURVE ( ( 0.9999930479533516436, 0.9999965238864843009, 1.000000000000000000, 0.8660254037844387076, 1.000000000000000000, 0.8660254037844387076, 1.000000000000000000, 0.8660254037844387076, 1.000000000000000000, 0.9999991396657871290, 0.9999982793426236416 ) ) 
 REPRESENTATION_ITEM ( '' )  );
#9700=LINE ( 'NONE', #37542, #39341 ) ;
#9701=CARTESIAN_POINT ( 'NONE',  ( 97.30629616937498838, -211.3315407142195852, 76.09614583420048461 ) ) ;
#9709=ORIENTED_EDGE ( 'NONE', *, *, #54402, .F. ) ;
#9710=DIRECTION ( 'NONE',  ( -0.000000000000000000, -0.000000000000000000, 1.000000000000000000 ) ) ;
#9711=CARTESIAN_POINT ( 'NONE',  ( 92.35000000000002274, -208.4700217866474645, 79.86645833506761960 ) ) ;
#9712=CARTESIAN_POINT ( 'NONE',  ( 93.67499999999998295, 92.29496732002878900, 81.00416666666666288 ) ) ;
#9715=VERTEX_POINT ( 'NONE', #63329 ) ;
#9719=CARTESIAN_POINT ( 'NONE',  ( -97.30629616937501680, 90.00000000000004263, 84.08656250086716000 ) ) ;
#9720=CARTESIAN_POINT ( 'NONE',  ( 94.99999999999998579, 87.33691857156068750, 82.18156250086714465 ) ) ;
#9721=ORIENTED_EDGE ( 'NONE', *, *, #43732, .T. ) ;
#9725=DIRECTION ( 'NONE',  ( 1.000000000000000000, 0.000000000000000000, 0.000000000000000000 ) ) ;
#9735=CARTESIAN_POINT ( 'NONE',  ( 94.99999999999998579, 93.05995642670504253, 88.65062500173431204 ) ) ;
#9738=CARTESIAN_POINT ( 'NONE',  ( -93.84685191531247028, -211.9973110713294489, 79.69447916753379957 ) ) ;
#9743=FACE_OUTER_BOUND ( 'NONE', #9589, .T. ) ;
#9744=EDGE_CURVE ( 'NONE', #2080, #58390, #62210, .T. ) ;
#9749=CARTESIAN_POINT ( 'NONE',  ( 92.35000000039364920, -209.9999706968037287, 82.45844277051352833 ) ) ;
#9753=CARTESIAN_POINT ( 'NONE',  ( 97.64999999999447766, 89.99999459739470353, 81.50687481489491404 ) ) ;
#9755=LINE ( 'NONE', #60530, #47209 ) ;
#9758=CARTESIAN_POINT ( 'NONE',  ( -97.65000000000001990, 90.00002803130638540, 87.53937403222812463 ) ) ;
#9760=CARTESIAN_POINT ( 'NONE',  ( 94.99999999999998579, 93.05995642670504253, 75.95062500173428077 ) ) ;
#9762=DIRECTION ( 'NONE',  ( -0.000000000000000000, -0.000000000000000000, 1.000000000000000000 ) ) ;
#9764=CARTESIAN_POINT ( 'NONE',  ( -97.64999999999994884, -211.5299782133524502, 83.06791666666664753 ) ) ;
#9765=CARTESIAN_POINT ( 'NONE',  ( -94.95306897617113862, 87.35041560265752025, 75.00000002508417651 ) ) ;
#9777=CARTESIAN_POINT ( 'NONE',  ( 95.00000000000000000, -207.3369185715606307, 88.37281250086715545 ) ) ;
#9785=CARTESIAN_POINT ( 'NONE',  ( 96.15314808468748708, -208.0026889286704943, 82.44614583420046472 ) ) ;
#9786=CARTESIAN_POINT ( 'NONE',  ( 97.30629616937498838, -209.9999999999999716, 85.67406250086715147 ) ) ;
#9788=CARTESIAN_POINT ( 'NONE',  ( 93.84685191531251292, -211.9973110713294489, 86.73239583420048859 ) ) ;
#9802=VERTEX_POINT ( 'NONE', #35112 ) ;
#9807=VERTEX_POINT ( 'NONE', #58042 ) ;
#9809=CARTESIAN_POINT ( 'NONE',  ( -97.30629616937501680, 90.00000000000004263, 89.80156250086714920 ) ) ;
#9811=VERTEX_POINT ( 'NONE', #8017 ) ;
#9814=CARTESIAN_POINT ( 'NONE',  ( -93.67499999999998295, -212.2949673200287179, 84.49666666666666970 ) ) ;
#9815=CARTESIAN_POINT ( 'NONE',  ( -93.67499999999998295, -207.7050326799711968, 88.51833333333333087 ) ) ;
#9816=CARTESIAN_POINT ( 'NONE',  ( -97.30629616937501680, 90.00000000000004263, 75.19656250086714522 ) ) ;
#9817=ORIENTED_EDGE ( 'NONE', *, *, #4967, .F. ) ;
#9818=CARTESIAN_POINT ( 'NONE',  ( 96.15314808468748708, 88.00268892867053694, 77.15447916753380753 ) ) ;
#9824=DIRECTION ( 'NONE',  ( 1.000000000000000000, 1.343011723336883198E-16, -0.000000000000000000 ) ) ;
#9826=CARTESIAN_POINT ( 'NONE',  ( -92.69370383062498320, -208.6684592857803295, 79.85322916753379729 ) ) ;
#9828=AXIS2_PLACEMENT_3D ( 'NONE', #25918, #48114, #70285 ) ;
#9829=EDGE_CURVE ( 'NONE', #26516, #22350, #69011, .T. ) ;
#9832=CARTESIAN_POINT ( 'NONE',  ( -92.34999999999999432, -209.9999999999999716, 83.96750000000000114 ) ) ;
#9835=VECTOR ( 'NONE', #12431, 1000.000000000000000 ) ;
#9842=CARTESIAN_POINT ( 'NONE',  ( -92.69370383062502583, 88.66845928578038638, 82.28739583420048120 ) ) ;
#9851=VECTOR ( 'NONE', #53555, 1000.000000000000000 ) ;
#9854=CARTESIAN_POINT ( 'NONE',  ( -94.99999999999997158, -207.3369185715606307, 78.21281250086717307 ) ) ;
#9865=EDGE_CURVE ( 'NONE', #41695, #24873, #48246, .T. ) ;
#9866=CARTESIAN_POINT ( 'NONE',  ( -2.499999999999970690, 73.00000000000001421, -251.7000000000000455 ) ) ;
#9869=ADVANCED_FACE ( 'NONE', ( #41859 ), #6908, .F. ) ;
#9877=CARTESIAN_POINT ( 'NONE',  ( -94.99999999999997158, -206.9400435732949575, 84.84062500173429555 ) ) ;
#9883=LINE ( 'NONE', #73018, #40756 ) ;
#9888=CARTESIAN_POINT ( 'NONE',  ( 93.84685191531248449, 91.99731107132950569, 76.36072916753381890 ) ) ;
#9890=DIRECTION ( 'NONE',  ( 1.000000000000000000, 0.000000000000000000, 0.000000000000000000 ) ) ;
#9892=EDGE_LOOP ( 'NONE', ( #28587, #69990, #698, #50394 ) ) ;
#9894=CARTESIAN_POINT ( 'NONE',  ( 94.99999999999998579, 87.33691857156068750, 88.53156250086713897 ) ) ;
#9896=CARTESIAN_POINT ( 'NONE',  ( 96.15314808468750130, -211.9973110713294489, 86.67947916753381321 ) ) ;
#9899=CYLINDRICAL_SURFACE ( 'NONE', #41396, 2.649999999999985700 ) ;
#9905=CARTESIAN_POINT ( 'NONE',  ( -93.84685191531247028, -211.9973110713294489, 87.94947916753380923 ) ) ;
#9906=CARTESIAN_POINT ( 'NONE',  ( -95.00000000000002842, 92.66308142843932671, 85.19781250086714408 ) ) ;
#9907=VERTEX_POINT ( 'NONE', #26771 ) ;
#9908=CARTESIAN_POINT ( 'NONE',  ( 94.99999999999998579, 87.33691857156068750, 87.26156250086714294 ) ) ;
#9909=CARTESIAN_POINT ( 'NONE',  ( -92.69370383062502583, 91.33154071421968467, 89.37822916753381719 ) ) ;
#9911=CARTESIAN_POINT ( 'NONE',  ( 96.66077099052519372, 88.39973697852393286, 74.80065534806809069 ) ) ;
#9912=CARTESIAN_POINT ( 'NONE',  ( -92.34999999999999432, -210.0000000207151629, 80.87187500099602744 ) ) ;
#9914=CARTESIAN_POINT ( 'NONE',  ( 92.35003714631601213, 91.52999965978808916, 82.40645685155122635 ) ) ;
#9922=ORIENTED_EDGE ( 'NONE', *, *, #63102, .F. ) ;
#9924=CARTESIAN_POINT ( 'NONE',  ( -92.35000000000005116, 91.52997821335253548, 82.11541666666666117 ) ) ;
#9928=CARTESIAN_POINT ( 'NONE',  ( -92.34999999999999432, -211.5299782133524218, 77.00895833506763211 ) ) ;
#9929=CARTESIAN_POINT ( 'NONE',  ( 92.35000000030105127, 90.00002455906435728, 87.53856274002153270 ) ) ;
#9932=( BOUNDED_CURVE ( )  B_SPLINE_CURVE ( 2, ( #49955, #61262, #10115, #33038, #3761, #39070, #4498 ),
 .UNSPECIFIED., .F., .F. ) 
 B_SPLINE_CURVE_WITH_KNOTS ( ( 3, 2, 2, 3 ),
 ( 0.02083333333333322115, 0.02777777777777762705, 0.03472222222222204335, 0.04166666666666644231 ),
 .UNSPECIFIED. ) 
 CURVE ( )  GEOMETRIC_REPRESENTATION_ITEM ( )  RATIONAL_B_SPLINE_CURVE ( ( 1.000000000000002220, 0.8660254037844365982, 1.000000000000000000, 0.8660254037844387076, 1.000000000000000000, 0.8660254037844430375, 0.9999999999999956701 ) ) 
 REPRESENTATION_ITEM ( '' )  );
#9935=CARTESIAN_POINT ( 'NONE',  ( -97.30629616937501680, 91.33154071421968467, 81.33489583420048064 ) ) ;
#9938=CARTESIAN_POINT ( 'NONE',  ( 92.35000000000000853, -209.9999999999999716, 86.18999999999999773 ) ) ;
#9941=DIRECTION ( 'NONE',  ( 0.000000000000000000, -1.000000000000000000, 0.000000000000000000 ) ) ;
#9946=CARTESIAN_POINT ( 'NONE',  ( 96.15314808468748708, 91.99731107132950569, 79.42989583420049371 ) ) ;
#9947=CARTESIAN_POINT ( 'NONE',  ( -93.84685191531247028, -211.9973110713294489, 81.75822916753382685 ) ) ;
#9950=CARTESIAN_POINT ( 'NONE',  ( -97.64999999953499810, 89.99996900126896548, 83.09538598081491045 ) ) ;
#9951=CARTESIAN_POINT ( 'NONE',  ( -97.64999999999994884, -208.4700217866474645, 77.24708333333332178 ) ) ;
#9955=EDGE_CURVE ( 'NONE', #5579, #37620, #60993, .T. ) ;
#9956=CARTESIAN_POINT ( 'NONE',  ( -95.00000000000002842, 87.33691857156074434, 76.62531250086715318 ) ) ;
#9957=CARTESIAN_POINT ( 'NONE',  ( 93.84685191531251292, -211.9973110713294489, 80.85864583420047325 ) ) ;
#9963=DIRECTION ( 'NONE',  ( -0.000000000000000000, -0.000000000000000000, 1.000000000000000000 ) ) ;
#9967=CARTESIAN_POINT ( 'NONE',  ( 97.64999999999999147, -209.9999999999999716, 83.33250000000001023 ) ) ;
#9973=CARTESIAN_POINT ( 'NONE',  ( 92.69370383062498320, 90.00000000000002842, 86.62656250086715204 ) ) ;
#9974=CARTESIAN_POINT ( 'NONE',  ( -97.64999999996638280, -210.0000076551254722, 78.01464417100379478 ) ) ;
#9975=CARTESIAN_POINT ( 'NONE',  ( 97.64999999999999147, -209.9999999999999716, 76.98250000000000171 ) ) ;
#9984=CARTESIAN_POINT ( 'NONE',  ( -93.09170270117147084, 88.16127723153179829, 74.99954709728268654 ) ) ;
#9985=EDGE_CURVE ( 'NONE', #59733, #51512, #63746, .T. ) ;
#9987=CARTESIAN_POINT ( 'NONE',  ( -2.499999999999970690, 73.00000000000001421, -258.2999999999999545 ) ) ;
#9991=CARTESIAN_POINT ( 'NONE',  ( -93.67499999999998295, -212.2949673200287179, 82.03604166840096923 ) ) ;
#9992=ORIENTED_EDGE ( 'NONE', *, *, #2229, .T. ) ;
#9995=ORIENTED_EDGE ( 'NONE', *, *, #34629, .F. ) ;
#9996=CARTESIAN_POINT ( 'NONE',  ( -97.65000000000001990, 90.00000000000004263, 82.45937500173430124 ) ) ;
#9999=CARTESIAN_POINT ( 'NONE',  ( 92.69370383062498320, 90.00000000000002842, 82.81656250086714977 ) ) ;
#10006=CARTESIAN_POINT ( 'NONE',  ( 93.67499999999998295, 92.29496732002878900, 87.98916666666666231 ) ) ;
#10019=CARTESIAN_POINT ( 'NONE',  ( -96.15314808468747287, -208.0026889286704943, 82.07572916753382231 ) ) ;
#10025=CARTESIAN_POINT ( 'NONE',  ( 94.99999999999998579, 86.94004357329502852, 81.98312500173430806 ) ) ;
#10026=CARTESIAN_POINT ( 'NONE',  ( -97.64999999993850111, -209.9999881782113675, 76.10900611559516449 ) ) ;
#10027=CARTESIAN_POINT ( 'NONE',  ( 97.30629616937498838, 91.33154071421968467, 79.21822916753380639 ) ) ;
#10031=CARTESIAN_POINT ( 'NONE',  ( 92.69400202757778118, 90.94645204372866942, 74.89836836546783161 ) ) ;
#10040=DIRECTION ( 'NONE',  ( 0.000000000000000000, 0.000000000000000000, -1.000000000000000000 ) ) ;
#10042=CARTESIAN_POINT ( 'NONE',  ( -95.00000000000002842, 92.66308142843932671, 83.13406250086714522 ) ) ;
#10054=CARTESIAN_POINT ( 'NONE',  ( 97.65000000000000568, -211.5299782133524218, 85.89895833506763267 ) ) ;
#10056=CARTESIAN_POINT ( 'NONE',  ( 96.15314808468748708, -208.0026889286704943, 78.79489583420048859 ) ) ;
#10057=ORIENTED_EDGE ( 'NONE', *, *, #24022, .T. ) ;
#10065=CARTESIAN_POINT ( 'NONE',  ( 93.67500000000001137, -207.7050326799711968, 87.98916666666666231 ) ) ;
#10076=CARTESIAN_POINT ( 'NONE',  ( 92.35000000000000853, -209.9999999999999716, 81.82437500173429612 ) ) ;
#10077=CARTESIAN_POINT ( 'NONE',  ( 93.67499999999999716, 87.70503267997126784, 83.12083333333332291 ) ) ;
#10079=ORIENTED_EDGE ( 'NONE', *, *, #73385, .T. ) ;
#10086=CARTESIAN_POINT ( 'NONE',  ( -93.84685191531252713, 88.00268892867056536, 83.02822916753380866 ) ) ;
#10087=CARTESIAN_POINT ( 'NONE',  ( 93.84685191531248449, 88.00268892867053694, 78.95364583420047211 ) ) ;
#10088=ORIENTED_EDGE ( 'NONE', *, *, #25903, .F. ) ;
#10091=ADVANCED_FACE ( 'NONE', ( #53746 ), #59034, .F. ) ;
#10096=CARTESIAN_POINT ( 'NONE',  ( -94.99999999999997158, -212.6630814284392557, 81.54656250086715374 ) ) ;
#10100=CARTESIAN_POINT ( 'NONE',  ( 97.64999999999997726, 91.52997821335253548, 78.94041666666664980 ) ) ;
#10104=CARTESIAN_POINT ( 'NONE',  ( 93.67499999999998295, 92.29496732002878900, 89.33854166840096411 ) ) ;
#10106=CARTESIAN_POINT ( 'NONE',  ( -94.99999999999997158, -207.3369185715606307, 79.95906250086713385 ) ) ;
#10108=CARTESIAN_POINT ( 'NONE',  ( -92.34999999999998010, 88.47002178664757821, 86.45458333333331780 ) ) ;
#10113=CARTESIAN_POINT ( 'NONE',  ( -95.00000000000002842, 86.94004357329504273, 81.26874999999999716 ) ) ;
#10115=CARTESIAN_POINT ( 'NONE',  ( -93.67500000000003979, 87.70503267997129626, 89.57666666666666799 ) ) ;
#10116=CARTESIAN_POINT ( 'NONE',  ( 97.30629616937498838, 91.33154071421968467, 89.37822916753378877 ) ) ;
#10117=DIRECTION ( 'NONE',  ( -0.000000000000000000, -0.000000000000000000, 1.000000000000000000 ) ) ;
#10121=CARTESIAN_POINT ( 'NONE',  ( 92.35002600474520307, 88.47000677280088610, 86.32229270695526679 ) ) ;
#10128=LINE ( 'NONE', #54154, #5263 ) ;
#10132=DIRECTION ( 'NONE',  ( 0.8571673007021122226, 0.000000000000000000, 0.5150380749100542666 ) ) ;
#10133=CARTESIAN_POINT ( 'NONE',  ( -94.99999999999997158, -206.9400435732949575, 84.12625000000001307 ) ) ;
#10134=DIRECTION ( 'NONE',  ( 0.000000000000000000, 0.000000000000000000, 1.000000000000000000 ) ) ;
#10136=( BOUNDED_CURVE ( )  B_SPLINE_CURVE ( 2, ( #56868, #45597, #15519, #9877, #27906, #51208, #73764 ),
 .UNSPECIFIED., .F., .F. ) 
 B_SPLINE_CURVE_WITH_KNOTS ( ( 3, 2, 2, 3 ),
 ( 0.2963422021995995026, 0.3033979182594312429, 0.3104536838003485455, 0.3175094496522546383 ),
 .UNSPECIFIED. ) 
 CURVE ( )  GEOMETRIC_REPRESENTATION_ITEM ( )  RATIONAL_B_SPLINE_CURVE ( ( 0.9999981209233991253, 0.8660263433293280411, 1.000000000000000000, 0.8660254037844387076, 1.000000000000000000, 0.8660254037844387076, 1.000000000000000000 ) ) 
 REPRESENTATION_ITEM ( '' )  );
#10142=CARTESIAN_POINT ( 'NONE',  ( 97.30629616937498838, -208.6684592857803011, 88.26697916753381890 ) ) ;
#10145=LINE ( 'NONE', #33067, #45566 ) ;
#10148=CARTESIAN_POINT ( 'NONE',  ( 96.15314808468748708, -208.0026889286704943, 79.27114583420046756 ) ) ;
#10149=CARTESIAN_POINT ( 'NONE',  ( 95.00000000000000000, -212.6630814284392557, 86.15031250086717307 ) ) ;
#10152=VECTOR ( 'NONE', #70732, 1000.000000000000000 ) ;
#10153=CARTESIAN_POINT ( 'NONE',  ( 96.15314808468748708, -208.0026889286704943, 87.04989583420048405 ) ) ;
#10155=ORIENTED_EDGE ( 'NONE', *, *, #17095, .T. ) ;
#10157=ORIENTED_EDGE ( 'NONE', *, *, #46673, .T. ) ;
#10164=CARTESIAN_POINT ( 'NONE',  ( -95.00000000000002842, 86.94004357329504273, 77.45874999999999488 ) ) ;
#10170=ORIENTED_EDGE ( 'NONE', *, *, #35051, .F. ) ;
#10179=ORIENTED_EDGE ( 'NONE', *, *, #18280, .F. ) ;
#10183=CARTESIAN_POINT ( 'NONE',  ( -97.30629616937501680, 88.66845928578038638, 75.88447916753382572 ) ) ;
#10186=CARTESIAN_POINT ( 'NONE',  ( 94.99999999999998579, 92.66308142843935514, 76.78406250086712248 ) ) ;
#10188=CARTESIAN_POINT ( 'NONE',  ( 97.65000000000000568, 91.52997821335252127, 78.38479166840096468 ) ) ;
#10189=CARTESIAN_POINT ( 'NONE',  ( -93.84685191531247028, -211.9973110713294489, 89.21947916753380525 ) ) ;
#10191=CARTESIAN_POINT ( 'NONE',  ( 92.35000000046409241, 89.99996903277681781, 77.38038495127642591 ) ) ;
#10196=CARTESIAN_POINT ( 'NONE',  ( -92.69370383062498320, -208.6684592857803295, 79.21822916753380639 ) ) ;
#10199=CARTESIAN_POINT ( 'NONE',  ( -93.67499999999998295, -212.2949673200287179, 79.41666666666665719 ) ) ;
#10205=CARTESIAN_POINT ( 'NONE',  ( 92.48632958231168288, -210.0000000000000284, 74.91808492278046572 ) ) ;
#10207=CARTESIAN_POINT ( 'NONE',  ( -97.30629616937501680, 90.00000000000004263, 83.29281250086714294 ) ) ;
#10211=ORIENTED_EDGE ( 'NONE', *, *, #49340, .F. ) ;
#10216=CYLINDRICAL_SURFACE ( 'NONE', #23761, 2.649999999999985700 ) ;
#10218=CARTESIAN_POINT ( 'NONE',  ( -96.32500000000001705, 92.29496732002878900, 89.89416666666666345 ) ) ;
#10220=CARTESIAN_POINT ( 'NONE',  ( -92.69370383062498320, -211.3315407142195852, 79.90614583420048689 ) ) ;
#10222=CARTESIAN_POINT ( 'NONE',  ( 92.34999999999999432, 88.47002178664752137, 76.16229166840095388 ) ) ;
#10233=CARTESIAN_POINT ( 'NONE',  ( -92.35000000000005116, 91.52997821335253548, 75.84479166840098685 ) ) ;
#10234=FACE_OUTER_BOUND ( 'NONE', #73021, .T. ) ;
#10235=VERTEX_POINT ( 'NONE', #15749 ) ;
#10237=CARTESIAN_POINT ( 'NONE',  ( 93.84685191531249870, -208.0026889286704943, 89.53697916753381492 ) ) ;
#10247=ADVANCED_FACE ( 'NONE', ( #49946 ), #58452, .F. ) ;
#10251=EDGE_CURVE ( 'NONE', #29023, #32074, #24106, .T. ) ;
#10256=EDGE_CURVE ( 'NONE', #23771, #48987, #48785, .T. ) ;
#10257=CARTESIAN_POINT ( 'NONE',  ( 93.84685191531248449, 88.00268892867053694, 75.93739583420048689 ) ) ;
#10266=CARTESIAN_POINT ( 'NONE',  ( 96.15314808468748708, 91.99731107132950569, 88.16114583420046813 ) ) ;
#10269=CARTESIAN_POINT ( 'NONE',  ( 95.00000000000000000, -212.6630814284392557, 85.35656250086714181 ) ) ;
#10272=CARTESIAN_POINT ( 'NONE',  ( -97.64999999999986358, -208.4700217866474361, 80.42208333333330472 ) ) ;
#10278=CARTESIAN_POINT ( 'NONE',  ( -97.30629616937495996, -209.9999999999999716, 87.73781250086713612 ) ) ;
#10279=CARTESIAN_POINT ( 'NONE',  ( -97.30629616937501680, 88.66845928578038638, 86.04447916753382231 ) ) ;
#10281=CARTESIAN_POINT ( 'NONE',  ( 93.84685191531248449, 91.99731107132950569, 86.99697916753380866 ) ) ;
#10282=CARTESIAN_POINT ( 'NONE',  ( -93.84685191531252713, 88.00268892867056536, 88.58447916753381435 ) ) ;
#10286=DIRECTION ( 'NONE',  ( -0.000000000000000000, -0.000000000000000000, 1.000000000000000000 ) ) ;
#10291=EDGE_CURVE ( 'NONE', #38100, #5092, #22595, .T. ) ;
#10292=CARTESIAN_POINT ( 'NONE',  ( -96.32500000000001705, 92.29496732002878900, 86.71916666666666629 ) ) ;
#10301=CARTESIAN_POINT ( 'NONE',  ( -96.32500000000001705, 92.29496732002878900, 80.36916666666665776 ) ) ;
#10310=CARTESIAN_POINT ( 'NONE',  ( -97.30629616937501680, 91.33154071421968467, 82.60489583420047666 ) ) ;
#10315=CARTESIAN_POINT ( 'NONE',  ( -93.67500000000003979, 92.29496732002878900, 82.16833333333332234 ) ) ;
#10316=CARTESIAN_POINT ( 'NONE',  ( -94.99999999999997158, -212.6630814284392557, 88.05531250086716000 ) ) ;
#10319=CARTESIAN_POINT ( 'NONE',  ( 92.69370383062498320, 91.33154071421968467, 79.58864583420049144 ) ) ;
#10320=CARTESIAN_POINT ( 'NONE',  ( -92.69370383062498320, -208.6684592857803295, 80.01197916753382344 ) ) ;
#10323=CARTESIAN_POINT ( 'NONE',  ( 93.67500000000001137, -207.7050326799711968, 81.08354166840096866 ) ) ;
#10324=CARTESIAN_POINT ( 'NONE',  ( -92.34999999999999432, -208.4700217866474645, 75.76541666666666686 ) ) ;
#10325=CARTESIAN_POINT ( 'NONE',  ( 92.35000000010806787, -209.9999848944895007, 78.64888723592486031 ) ) ;
#10328=CARTESIAN_POINT ( 'NONE',  ( -93.84685191531254134, 91.99731107132950569, 78.15989583420049769 ) ) ;
#10329=CARTESIAN_POINT ( 'NONE',  ( 93.84685191531249870, -208.0026889286704943, 80.01197916753380923 ) ) ;
#10340=ORIENTED_EDGE ( 'NONE', *, *, #42466, .F. ) ;
#10344=CARTESIAN_POINT ( 'NONE',  ( 96.15314808468750130, -211.9973110713294489, 76.04322916753382344 ) ) ;
#10347=CARTESIAN_POINT ( 'NONE',  ( 92.35000000000000853, -209.9999999999999716, 83.65000000000000568 ) ) ;
#10348=CARTESIAN_POINT ( 'NONE',  ( 92.69370383062498320, 91.33154071421968467, 85.93864583420048575 ) ) ;
#10350=CARTESIAN_POINT ( 'NONE',  ( 97.64999999999997726, -208.4700217866474645, 79.57541666666665492 ) ) ;
#10360=DIRECTION ( 'NONE',  ( 0.000000000000000000, 0.000000000000000000, 1.000000000000000000 ) ) ;
#10362=CARTESIAN_POINT ( 'NONE',  ( -94.99999999999997158, -209.9999999999999716, 90.00000000000000000 ) ) ;
#10364=CARTESIAN_POINT ( 'NONE',  ( -92.34999999999999432, -208.4700217866474645, 82.19479166840095274 ) ) ;
#10368=CARTESIAN_POINT ( 'NONE',  ( 92.34999999999999432, 90.00000000000002842, 83.09437500173430635 ) ) ;
#10369=CARTESIAN_POINT ( 'NONE',  ( -93.67500000000003979, 87.70503267997129626, 81.40104166840096411 ) ) ;
#10370=( BOUNDED_CURVE ( )  B_SPLINE_CURVE ( 2, ( #11578, #27771, #11956, #28135, #363, #50698, #22891 ),
 .UNSPECIFIED., .F., .F. ) 
 B_SPLINE_CURVE_WITH_KNOTS ( ( 3, 2, 2, 3 ),
 ( 0.7708333333333328152, 0.7777777777777775681, 0.7847222222222222099, 0.7916666666666669627 ),
 .UNSPECIFIED. ) 
 CURVE ( )  GEOMETRIC_REPRESENTATION_ITEM ( )  RATIONAL_B_SPLINE_CURVE ( ( 1.000000000000010658, 0.8660254037844280495, 1.000000000000000000, 0.8660254037844387076, 1.000000000000000000, 0.8660254037844322683, 1.000000000000006439 ) ) 
 REPRESENTATION_ITEM ( '' )  );
#10372=CARTESIAN_POINT ( 'NONE',  ( 93.84685191531248449, 88.00268892867053694, 84.19239583420049655 ) ) ;
#10374=CARTESIAN_POINT ( 'NONE',  ( -97.65000000000001990, 90.00000000000004263, 90.00000000000000000 ) ) ;
#10382=EDGE_CURVE ( 'NONE', #40438, #5952, #10636, .T. ) ;
#10383=EDGE_CURVE ( 'NONE', #57918, #50963, #43193, .T. ) ;
#10385=ORIENTED_EDGE ( 'NONE', *, *, #8056, .T. ) ;
#10386=AXIS2_PLACEMENT_3D ( 'NONE', #57638, #51235, #68549 ) ;
#10394=CARTESIAN_POINT ( 'NONE',  ( -94.99999999999997158, -212.6630814284392557, 81.70531250086715147 ) ) ;
#10396=CYLINDRICAL_SURFACE ( 'NONE', #45321, 2.649999999999985700 ) ;
#10399=LINE ( 'NONE', #44247, #16730 ) ;
#10403=CARTESIAN_POINT ( 'NONE',  ( 92.69370383062501162, -209.9999999999999716, 89.64281250086713726 ) ) ;
#10413=CARTESIAN_POINT ( 'NONE',  ( -93.84685191531254134, 91.99731107132950569, 79.90614583420047268 ) ) ;
#10424=CARTESIAN_POINT ( 'NONE',  ( 93.84685191531249870, -208.0026889286704943, 76.36072916753381890 ) ) ;
#10429=EDGE_CURVE ( 'NONE', #52144, #15980, #12773, .T. ) ;
#10435=EDGE_CURVE ( 'NONE', #42455, #52827, #45522, .T. ) ;
#10436=CARTESIAN_POINT ( 'NONE',  ( 96.32499999999998863, -207.7050326799711968, 86.61333333333332973 ) ) ;
#10447=CARTESIAN_POINT ( 'NONE',  ( 93.67500000000001137, -207.7050326799711968, 81.08354166840096866 ) ) ;
#10448=CARTESIAN_POINT ( 'NONE',  ( 96.32499999999997442, 92.29496732002878900, 82.80333333333332746 ) ) ;
#10449=EDGE_CURVE ( 'NONE', #19930, #72643, #48108, .T. ) ;
#10454=EDGE_CURVE ( 'NONE', #14986, #59860, #42110, .T. ) ;
#10456=VERTEX_POINT ( 'NONE', #65046 ) ;
#10458=CARTESIAN_POINT ( 'NONE',  ( -92.69370383062505425, 91.33154071421968467, 83.82197916753382572 ) ) ;
#10459=CARTESIAN_POINT ( 'NONE',  ( 97.30629616937498838, 88.66845928578037217, 78.47739583420047893 ) ) ;
#10468=CARTESIAN_POINT ( 'NONE',  ( -94.99999999999997158, -207.3369185715606307, 78.68906250086713783 ) ) ;
#10470=ORIENTED_EDGE ( 'NONE', *, *, #54756, .T. ) ;
#10475=EDGE_LOOP ( 'NONE', ( #22628, #14674, #1878, #73540 ) ) ;
#10476=CARTESIAN_POINT ( 'NONE',  ( -96.15314808468745866, -211.9973110713294489, 76.41364583420048007 ) ) ;
#10477=ORIENTED_EDGE ( 'NONE', *, *, #51104, .F. ) ;
#10486=CARTESIAN_POINT ( 'NONE',  ( 97.30629616937498838, 91.33154071421968467, 88.74322916753382628 ) ) ;
#10489=CYLINDRICAL_SURFACE ( 'NONE', #28893, 3.299999999999969624 ) ;
#10490=DIRECTION ( 'NONE',  ( -1.000000000000000000, -0.000000000000000000, -0.000000000000000000 ) ) ;
#10498=DIRECTION ( 'NONE',  ( -0.000000000000000000, -0.000000000000000000, 1.000000000000000000 ) ) ;
#10501=CARTESIAN_POINT ( 'NONE',  ( -97.64999999999994884, -211.5299782133524502, 83.70291666666668107 ) ) ;
#10509=ADVANCED_FACE ( 'NONE', ( #37208 ), #71757, .F. ) ;
#10511=CARTESIAN_POINT ( 'NONE',  ( 97.30629616937498838, -208.6684592857803011, 88.90197916753382401 ) ) ;
#10512=ORIENTED_EDGE ( 'NONE', *, *, #157, .F. ) ;
#10513=ORIENTED_EDGE ( 'NONE', *, *, #44605, .F. ) ;
#10517=CARTESIAN_POINT ( 'NONE',  ( 93.84685191531249870, -208.0026889286704943, 78.10697916753380809 ) ) ;
#10520=ORIENTED_EDGE ( 'NONE', *, *, #54756, .F. ) ;
#10521=CARTESIAN_POINT ( 'NONE',  ( 92.69370383062501162, -209.9999999999999716, 81.54656250086715374 ) ) ;
#10526=CARTESIAN_POINT ( 'NONE',  ( -92.69370383062504004, 90.00000000000004263, 74.87906250086714977 ) ) ;
#10530=ORIENTED_EDGE ( 'NONE', *, *, #948, .T. ) ;
#10535=EDGE_CURVE ( 'NONE', #66338, #37865, #2291, .T. ) ;
#10542=CARTESIAN_POINT ( 'NONE',  ( 97.30629616937498838, -208.6684592857803011, 75.40822916753381833 ) ) ;
#10551=DIRECTION ( 'NONE',  ( 0.000000000000000000, -0.000000000000000000, -1.000000000000000000 ) ) ;
#10554=CARTESIAN_POINT ( 'NONE',  ( -97.30629616937501680, 91.33154071421968467, 76.41364583420049428 ) ) ;
#10555=ORIENTED_EDGE ( 'NONE', *, *, #55706, .F. ) ;
#10556=CARTESIAN_POINT ( 'NONE',  ( 97.64999999999997726, -208.4700217866474929, 89.73541666666663730 ) ) ;
#10559=CARTESIAN_POINT ( 'NONE',  ( -94.99999999999997158, -207.3369185715606307, 85.67406250086715147 ) ) ;
#10560=ORIENTED_EDGE ( 'NONE', *, *, #24718, .T. ) ;
#10564=CARTESIAN_POINT ( 'NONE',  ( -93.84685191531248449, -208.0026889286704943, 81.17614583420048291 ) ) ;
#10567=CARTESIAN_POINT ( 'NONE',  ( -97.64999999999996305, -209.9999999999999716, 79.20499999999999829 ) ) ;
#10571=CARTESIAN_POINT ( 'NONE',  ( -96.15314808468751551, 88.00268892867056536, 82.12864583420046927 ) ) ;
#10574=( BOUNDED_CURVE ( )  B_SPLINE_CURVE ( 2, ( #13747, #26518, #36687, #32145, #71251, #65278, #60746, #3251, #15235 ),
 .UNSPECIFIED., .F., .F. ) 
 B_SPLINE_CURVE_WITH_KNOTS ( ( 3, 2, 2, 2, 3 ),
 ( 0.6561861948910822084, 0.6632419608429419577, 0.6702977263838236777, 0.6773534919247052866, 0.6773535682752291898 ),
 .UNSPECIFIED. ) 
 CURVE ( )  GEOMETRIC_REPRESENTATION_ITEM ( )  RATIONAL_B_SPLINE_CURVE ( ( 1.000000000000000000, 0.8660254037844387076, 1.000000000000000000, 0.8660254037844387076, 1.000000000000000000, 0.8660254037844387076, 1.000000000000000000, 0.9999985502592815267, 0.9999971005499384002 ) ) 
 REPRESENTATION_ITEM ( '' )  );
#10577=FACE_BOUND ( 'NONE', #74153, .T. ) ;
#10585=CARTESIAN_POINT ( 'NONE',  ( 97.64999999999999147, -209.9999999999999716, 85.87249999999998806 ) ) ;
#10586=CARTESIAN_POINT ( 'NONE',  ( -92.35000000000003695, 90.00000000000004263, 87.14249999999999829 ) ) ;
#10587=CARTESIAN_POINT ( 'NONE',  ( -96.15314808468747287, -208.0026889286704943, 78.90072916753382515 ) ) ;
#10588=ADVANCED_FACE ( 'NONE', ( #8633 ), #14995, .F. ) ;
#10599=AXIS2_PLACEMENT_3D ( 'NONE', #54198, #71458, #52707 ) ;
#10610=CARTESIAN_POINT ( 'NONE',  ( 92.69370383062501162, -209.9999999999999716, 89.64281250086713726 ) ) ;
#10611=CARTESIAN_POINT ( 'NONE',  ( -94.99999999999997158, -206.9400435732949575, 87.38062500173430180 ) ) ;
#10614=CARTESIAN_POINT ( 'NONE',  ( 96.32499999999998863, -212.2949673200287179, 89.57666666666666799 ) ) ;
#10627=CARTESIAN_POINT ( 'NONE',  ( 96.15314808468748708, 91.99731107132950569, 76.25489583420049655 ) ) ;
#10636=B_SPLINE_CURVE_WITH_KNOTS ( 'NONE', 3,
 ( #2287, #53745, #36817, #13522, #25540, #59033 ),
 .UNSPECIFIED., .F., .F.,
 ( 4, 2, 4 ),
 ( 0.000000000000000000, 0.0008269033587275365343, 0.001653806717455073069 ),
 .UNSPECIFIED. ) ;
#10638=CARTESIAN_POINT ( 'NONE',  ( 93.84685191531248449, 88.00268892867053694, 88.47864583420047779 ) ) ;
#10640=CARTESIAN_POINT ( 'NONE',  ( 92.69370383062501162, -208.6684592857803011, 83.87489583420047268 ) ) ;
#10644=CARTESIAN_POINT ( 'NONE',  ( -97.65000000000001990, 90.00000000000004263, 78.01437500173430806 ) ) ;
#10648=CARTESIAN_POINT ( 'NONE',  ( -93.84685191531248449, -208.0026889286704943, 89.43114583420047836 ) ) ;
#10649=CARTESIAN_POINT ( 'NONE',  ( -97.30629616937501680, 88.66845928578038638, 84.77447916753381207 ) ) ;
#10651=CARTESIAN_POINT ( 'NONE',  ( 94.99999999999998579, 87.33691857156068750, 86.62656250086715204 ) ) ;
#10652=CARTESIAN_POINT ( 'NONE',  ( -96.15314808468751551, 88.00268892867056536, 84.66864583420047552 ) ) ;
#10660=DIRECTION ( 'NONE',  ( -0.000000000000000000, -0.000000000000000000, 1.000000000000000000 ) ) ;
#10668=CARTESIAN_POINT ( 'NONE',  ( -93.67500000000003979, 87.70503267997129626, 82.59166666666665435 ) ) ;
#10669=DIRECTION ( 'NONE',  ( -1.000000000000000000, 0.000000000000000000, 0.000000000000000000 ) ) ;
#10678=CARTESIAN_POINT ( 'NONE',  ( -97.30629616937501680, 88.66845928578038638, 78.90072916753381094 ) ) ;
#10679=ADVANCED_FACE ( 'NONE', ( #62376 ), #40168, .F. ) ;
#10680=CARTESIAN_POINT ( 'NONE',  ( -94.99999999999997158, -209.9999999999999716, 73.40771935957695860 ) ) ;
#10688=CIRCLE ( 'NONE', #14511, 12.74999999999999822 ) ;
#10690=CARTESIAN_POINT ( 'NONE',  ( 94.99999999999998579, 87.33691857156068750, 80.43531250086715545 ) ) ;
#10691=AXIS2_PLACEMENT_3D ( 'NONE', #71918, #8036, #53531 ) ;
#10692=VECTOR ( 'NONE', #32309, 1000.000000000000000 ) ;
#10693=CARTESIAN_POINT ( 'NONE',  ( -93.84685191531247028, -211.9973110713294489, 79.85322916753381151 ) ) ;
#10697=CARTESIAN_POINT ( 'NONE',  ( -95.00000000000002842, 86.94004357329504273, 87.06312500173429214 ) ) ;
#10699=CYLINDRICAL_SURFACE ( 'NONE', #29312, 2.649999999999985700 ) ;
#10702=CARTESIAN_POINT ( 'NONE',  ( -93.84685191531254134, 91.99731107132950569, 78.79489583420048859 ) ) ;
#10703=CARTESIAN_POINT ( 'NONE',  ( 92.69370383062501162, -208.6684592857803011, 81.96989583420048575 ) ) ;
#10710=ORIENTED_EDGE ( 'NONE', *, *, #58545, .T. ) ;
#10713=FACE_OUTER_BOUND ( 'NONE', #37868, .T. ) ;
#10717=ORIENTED_EDGE ( 'NONE', *, *, #22798, .F. ) ;
#10720=ORIENTED_EDGE ( 'NONE', *, *, #64843, .F. ) ;
#10723=EDGE_CURVE ( 'NONE', #47502, #33969, #1853, .T. ) ;
#10724=VERTEX_POINT ( 'NONE', #63478 ) ;
#10727=CARTESIAN_POINT ( 'NONE',  ( 92.69370383062498320, 91.33154071421968467, 85.30364583420048064 ) ) ;
#10729=CARTESIAN_POINT ( 'NONE',  ( 95.00000000000000000, -206.9400435732949575, 77.77624999999999034 ) ) ;
#10742=CARTESIAN_POINT ( 'NONE',  ( -93.67499999999998295, -207.7050326799711968, 81.61270833506763722 ) ) ;
#10746=CARTESIAN_POINT ( 'NONE',  ( 92.34999999999999432, 88.47002178664753558, 81.87729166840097150 ) ) ;
#10747=CARTESIAN_POINT ( 'NONE',  ( -93.67500000000003979, 92.29496732002878900, 80.34270833506762699 ) ) ;
#10749=CARTESIAN_POINT ( 'NONE',  ( 94.99999999999998579, 92.66308142843935514, 84.56281250086716739 ) ) ;
#10750=CARTESIAN_POINT ( 'NONE',  ( 97.64999999999987779, 91.52997821335259232, 83.38541666666667140 ) ) ;
#10758=CARTESIAN_POINT ( 'NONE',  ( -89.99999999999998579, -204.9999999999999716, 90.00000000000000000 ) ) ;
#10759=CARTESIAN_POINT ( 'NONE',  ( -97.65000000000001990, 90.00000000000004263, 82.45937500173430124 ) ) ;
#10766=CARTESIAN_POINT ( 'NONE',  ( -0.0004442498525516064278, 0.001194404164626844313, -64.00000000000000000 ) ) ;
#10767=CARTESIAN_POINT ( 'NONE',  ( -96.15314808468747287, -208.0026889286704943, 80.80572916753382628 ) ) ;
#10769=CARTESIAN_POINT ( 'NONE',  ( -92.69370383062504004, 90.00000000000004263, 87.42031250086714067 ) ) ;
#10773=VECTOR ( 'NONE', #58443, 1000.000000000000000 ) ;
#10777=CARTESIAN_POINT ( 'NONE',  ( -0.0004442498525516064278, 0.001194404164626844313, -64.00000000000000000 ) ) ;
#10783=CARTESIAN_POINT ( 'NONE',  ( -93.67499999999998295, -207.7050326799711968, 76.53270833506762472 ) ) ;
#10784=ADVANCED_FACE ( 'NONE', ( #21756 ), #67621, .F. ) ;
#10786=LINE ( 'NONE', #74304, #5235 ) ;
#10795=CARTESIAN_POINT ( 'NONE',  ( -97.30629616937501680, 90.00000000000004263, 78.84781250086714977 ) ) ;
#10797=CARTESIAN_POINT ( 'NONE',  ( 92.69370383062501162, -208.6684592857803011, 88.95489583420048518 ) ) ;
#10799=( BOUNDED_CURVE ( )  B_SPLINE_CURVE ( 2, ( #40972, #7491, #24405, #47340, #53346, #1886, #29294 ),
 .UNSPECIFIED., .F., .F. ) 
 B_SPLINE_CURVE_WITH_KNOTS ( ( 3, 2, 2, 3 ),
 ( 0.1693384224419982043, 0.1763941385220585967, 0.1834499040629412603, 0.1905056698837211959 ),
 .UNSPECIFIED. ) 
 CURVE ( )  GEOMETRIC_REPRESENTATION_ITEM ( )  RATIONAL_B_SPLINE_CURVE ( ( 0.9999981216929038075, 0.8660263429445702599, 1.000000000000000000, 0.8660254037844387076, 1.000000000000000000, 0.8660254037844387076, 1.000000000000000000 ) ) 
 REPRESENTATION_ITEM ( '' )  );
#10801=CYLINDRICAL_SURFACE ( 'NONE', #53987, 2.649999999999985700 ) ;
#10805=CARTESIAN_POINT ( 'NONE',  ( -97.64999999999996305, -209.9999999999999716, 84.92000000000000171 ) ) ;
#10808=CARTESIAN_POINT ( 'NONE',  ( 97.30629616937498838, -211.3315407142195852, 76.73114583420048973 ) ) ;
#10815=( BOUNDED_CURVE ( )  B_SPLINE_CURVE ( 2, ( #33813, #51101, #22542, #39838, #51470, #62790, #34546 ),
 .UNSPECIFIED., .F., .F. ) 
 B_SPLINE_CURVE_WITH_KNOTS ( ( 3, 2, 2, 3 ),
 ( 0.6458333333333334814, 0.6527777777777779011, 0.6597222222222223209, 0.6666666666666667407 ),
 .UNSPECIFIED. ) 
 CURVE ( )  GEOMETRIC_REPRESENTATION_ITEM ( )  RATIONAL_B_SPLINE_CURVE ( ( 0.9999999999999978906, 0.8660254037844408170, 1.000000000000000000, 0.8660254037844387076, 1.000000000000000000, 0.8660254037844365982, 1.000000000000002220 ) ) 
 REPRESENTATION_ITEM ( '' )  );
#10818=CARTESIAN_POINT ( 'NONE',  ( 92.35000000000000853, -209.9999999999999716, 88.09499999999999886 ) ) ;
#10822=EDGE_LOOP ( 'NONE', ( #60216, #35336 ) ) ;
#10824=ORIENTED_EDGE ( 'NONE', *, *, #55503, .T. ) ;
#10825=DIRECTION ( 'NONE',  ( -0.000000000000000000, -0.000000000000000000, 1.000000000000000000 ) ) ;
#10831=CARTESIAN_POINT ( 'NONE',  ( 92.34999999999999432, 90.00000000000002842, 87.45999999999999375 ) ) ;
#10832=CARTESIAN_POINT ( 'NONE',  ( 95.00000000000000000, -206.9400435732949575, 77.22062500173429100 ) ) ;
#10833=CARTESIAN_POINT ( 'NONE',  ( 96.32499999999997442, 92.29496732002878900, 80.89833333333332632 ) ) ;
#10834=ORIENTED_EDGE ( 'NONE', *, *, #869, .T. ) ;
#10835=CARTESIAN_POINT ( 'NONE',  ( 97.64999999999999147, -210.0000000024471092, 75.15687493081163950 ) ) ;
#10840=CARTESIAN_POINT ( 'NONE',  ( -93.84685191531254134, 91.99731107132950569, 83.23989583420049598 ) ) ;
#10841=CARTESIAN_POINT ( 'NONE',  ( 96.15314808468748708, 88.00268892867053694, 77.78947916753381264 ) ) ;
#10849=CARTESIAN_POINT ( 'NONE',  ( -92.69370383062498320, -211.3315407142195852, 75.93739583420047268 ) ) ;
#10857=CARTESIAN_POINT ( 'NONE',  ( -97.30629616937497417, -211.3315407142195852, 76.36072916753381890 ) ) ;
#10859=CARTESIAN_POINT ( 'NONE',  ( -96.32500000000001705, 87.70503267997129626, 76.77083333333332860 ) ) ;
#10871=CARTESIAN_POINT ( 'NONE',  ( 96.15314808468748708, 88.00268892867053694, 84.77447916753381207 ) ) ;
#10878=CARTESIAN_POINT ( 'NONE',  ( 96.32499999999998863, -212.2949673200287179, 87.75104166840095843 ) ) ;
#10879=CARTESIAN_POINT ( 'NONE',  ( 96.32499999999998863, 87.70503267997126784, 77.51166666666665606 ) ) ;
#10885=CARTESIAN_POINT ( 'NONE',  ( -93.84685191531254134, 91.99731107132950569, 88.16114583420046813 ) ) ;
#10888=CARTESIAN_POINT ( 'NONE',  ( -94.99999999999997158, -206.9400435732949575, 84.76125000000000398 ) ) ;
#10900=CARTESIAN_POINT ( 'NONE',  ( 96.15314808468748708, -208.0026889286704943, 86.41489583420049314 ) ) ;
#10906=CARTESIAN_POINT ( 'NONE',  ( 97.30629616937498838, -211.3315407142195852, 77.84239583420047381 ) ) ;
#10908=CARTESIAN_POINT ( 'NONE',  ( 95.00000000000000000, -207.3369185715606307, 84.56281250086716739 ) ) ;
#10917=CARTESIAN_POINT ( 'NONE',  ( 97.65000000000000568, -211.5299782133524218, 77.00895833506763211 ) ) ;
#10918=CARTESIAN_POINT ( 'NONE',  ( 92.35000000000000853, -209.9999999999999716, 86.90437500173429441 ) ) ;
#10924=ORIENTED_EDGE ( 'NONE', *, *, #11540, .F. ) ;
#10926=CARTESIAN_POINT ( 'NONE',  ( 93.84685191531249870, -208.0026889286704943, 76.20197916753380696 ) ) ;
#10929=VERTEX_POINT ( 'NONE', #1099 ) ;
#10931=ORIENTED_EDGE ( 'NONE', *, *, #52692, .T. ) ;
#10932=ORIENTED_EDGE ( 'NONE', *, *, #51071, .T. ) ;
#10936=( BOUNDED_CURVE ( )  B_SPLINE_CURVE ( 2, ( #41168, #64106, #53184, #1720, #24607, #47546, #20660 ),
 .UNSPECIFIED., .F., .F. ) 
 B_SPLINE_CURVE_WITH_KNOTS ( ( 3, 2, 2, 3 ),
 ( 0.7916666666666669627, 0.7986111111111114935, 0.8055555555555558023, 0.8125000000000002220 ),
 .UNSPECIFIED. ) 
 CURVE ( )  GEOMETRIC_REPRESENTATION_ITEM ( )  RATIONAL_B_SPLINE_CURVE ( ( 0.9999999999999935607, 0.8660254037844451469, 1.000000000000000000, 0.8660254037844387076, 1.000000000000000000, 0.8660254037844343777, 1.000000000000004219 ) ) 
 REPRESENTATION_ITEM ( '' )  );
#10937=LINE ( 'NONE', #44038, #65922 ) ;
#10939=CARTESIAN_POINT ( 'NONE',  ( -92.69370383062502583, 88.66845928578038638, 76.73114583420048973 ) ) ;
#10941=CARTESIAN_POINT ( 'NONE',  ( 93.84685191531248449, 91.99731107132950569, 75.56697916753381605 ) ) ;
#10943=ORIENTED_EDGE ( 'NONE', *, *, #22515, .F. ) ;
#10945=CARTESIAN_POINT ( 'NONE',  ( -93.84685191531247028, -211.9973110713294489, 87.31447916753380412 ) ) ;
#10950=CARTESIAN_POINT ( 'NONE',  ( -94.99999999999997158, -212.6630814284392557, 80.91156250086714863 ) ) ;
#10953=FACE_OUTER_BOUND ( 'NONE', #41158, .T. ) ;
#10957=CARTESIAN_POINT ( 'NONE',  ( -97.47814808468746151, -209.9999999999999716, 89.90078125043358170 ) ) ;
#10958=CARTESIAN_POINT ( 'NONE',  ( -96.15314808468752972, 91.99731107132950569, 82.55197916753380127 ) ) ;
#10963=CARTESIAN_POINT ( 'NONE',  ( -92.34999999999999432, -208.4700217866474645, 80.28979166840095161 ) ) ;
#10967=CARTESIAN_POINT ( 'NONE',  ( 95.00000000000000000, -206.9400435732949575, 89.28562500173430294 ) ) ;
#10971=DIRECTION ( 'NONE',  ( 1.000000000000000000, 0.000000000000000000, 0.000000000000000000 ) ) ;
#10972=CARTESIAN_POINT ( 'NONE',  ( -94.99999999999997158, -212.6630814284392557, 81.07031250086716057 ) ) ;
#10979=CARTESIAN_POINT ( 'NONE',  ( -95.00000000000002842, 93.05995642670504253, 88.57124999999999204 ) ) ;
#10991=CARTESIAN_POINT ( 'NONE',  ( 92.69370383062501162, -211.3315407142195852, 87.15572916753380639 ) ) ;
#10998=CARTESIAN_POINT ( 'NONE',  ( -94.99999999999997158, -209.9999999999999716, 90.00000000000000000 ) ) ;
#10999=ORIENTED_EDGE ( 'NONE', *, *, #30469, .T. ) ;
#11007=CARTESIAN_POINT ( 'NONE',  ( 94.99999999999998579, 86.94004357329500010, 86.98374999999998636 ) ) ;
#11008=CARTESIAN_POINT ( 'NONE',  ( 94.99999999999998579, 90.00000000000002842, 90.00000000000000000 ) ) ;
#11014=CARTESIAN_POINT ( 'NONE',  ( 93.84685191531248449, 91.99731107132950569, 85.09197916753380753 ) ) ;
#11016=CARTESIAN_POINT ( 'NONE',  ( 93.84685191531249870, -208.0026889286704943, 85.72697916753379843 ) ) ;
#11025=CARTESIAN_POINT ( 'NONE',  ( 92.34999999999999432, 90.00000000000002842, 84.99937500173429328 ) ) ;
#11026=CARTESIAN_POINT ( 'NONE',  ( -92.69370383062498320, -209.9999999999999716, 86.78531250086714977 ) ) ;
#11028=CARTESIAN_POINT ( 'NONE',  ( -92.69370383062504004, 90.00000000000004263, 86.30906250086715659 ) ) ;
#11031=CARTESIAN_POINT ( 'NONE',  ( 97.30629616937498838, 90.00000000000002842, 82.97531250086714749 ) ) ;
#11032=CARTESIAN_POINT ( 'NONE',  ( -92.69370383062504004, 90.00000000000004263, 84.24531250086714351 ) ) ;
#11034=( BOUNDED_CURVE ( )  B_SPLINE_CURVE ( 2, ( #8066, #18966, #37400, #19341, #19710, #41916, #65227, #71203, #60332 ),
 .UNSPECIFIED., .F., .F. ) 
 B_SPLINE_CURVE_WITH_KNOTS ( ( 3, 2, 2, 2, 3 ),
 ( 0.8043570860654229993, 0.8043572716605899009, 0.8114130372014723980, 0.8184688027423547840, 0.8255245790564498254 ),
 .UNSPECIFIED. ) 
 CURVE ( )  GEOMETRIC_REPRESENTATION_ITEM ( )  RATIONAL_B_SPLINE_CURVE ( ( 0.9999929520380603787, 0.9999964759263327840, 1.000000000000000000, 0.8660254037844387076, 1.000000000000000000, 0.8660254037844387076, 1.000000000000000000, 0.8660254037844387076, 1.000000000000000000 ) ) 
 REPRESENTATION_ITEM ( '' )  );
#11039=CARTESIAN_POINT ( 'NONE',  ( 95.00000000000000000, -206.9400435732949575, 85.39624999999998067 ) ) ;
#11040=CARTESIAN_POINT ( 'NONE',  ( -94.99999999999997158, -207.3369185715606307, 88.21406250086712930 ) ) ;
#11047=DIRECTION ( 'NONE',  ( -0.000000000000000000, -0.000000000000000000, 1.000000000000000000 ) ) ;
#11048=ORIENTED_EDGE ( 'NONE', *, *, #24894, .T. ) ;
#11052=CARTESIAN_POINT ( 'NONE',  ( -97.65000000000001990, 90.00000000000004263, 78.57000000000000739 ) ) ;
#11054=CARTESIAN_POINT ( 'NONE',  ( 95.00000000000000000, -213.0599564267049857, 75.63312500173429953 ) ) ;
#11055=CARTESIAN_POINT ( 'NONE',  ( -97.64999999999996305, -209.9999999999999716, 76.74437500173429783 ) ) ;
#11060=CARTESIAN_POINT ( 'NONE',  ( -96.15314808468751551, 88.00268892867056536, 77.04864583420047097 ) ) ;
#11068=EDGE_CURVE ( 'NONE', #54488, #43660, #66435, .T. ) ;
#11070=CARTESIAN_POINT ( 'NONE',  ( 97.30629616937498838, 88.66845928578035796, 75.46114583420049371 ) ) ;
#11071=CARTESIAN_POINT ( 'NONE',  ( -94.99999999999997158, -207.3369185715606307, 80.75281250086716511 ) ) ;
#11079=CARTESIAN_POINT ( 'NONE',  ( -97.30629616937501680, 90.00000000000004263, 77.10156250086714635 ) ) ;
#11080=CARTESIAN_POINT ( 'NONE',  ( 93.84685191531249870, -208.0026889286704943, 78.74197916753381321 ) ) ;
#11086=VERTEX_POINT ( 'NONE', #71301 ) ;
#11092=CARTESIAN_POINT ( 'NONE',  ( 97.30629616937498838, -210.9303121318039871, 74.84209103131397001 ) ) ;
#11096=CARTESIAN_POINT ( 'NONE',  ( -95.62844927801778283, 87.44368763736515859, 74.98613922222766348 ) ) ;
#11097=CARTESIAN_POINT ( 'NONE',  ( 97.30629616937498838, 91.33154071421968467, 83.82197916753382572 ) ) ;
#11099=CARTESIAN_POINT ( 'NONE',  ( 97.64999999999997726, -211.5299782133524502, 79.46958333333333258 ) ) ;
#11100=ORIENTED_EDGE ( 'NONE', *, *, #19825, .T. ) ;
#11103=ORIENTED_EDGE ( 'NONE', *, *, #38528, .T. ) ;
#11107=CARTESIAN_POINT ( 'NONE',  ( 95.00000000000000000, -209.9999999999999716, 90.00000000000000000 ) ) ;
#11110=DIRECTION ( 'NONE',  ( 1.000000000000000000, 0.000000000000000000, 0.000000000000000000 ) ) ;
#11113=CARTESIAN_POINT ( 'NONE',  ( -93.67499999999998295, -207.7050326799711968, 80.97770833506763211 ) ) ;
#11114=ORIENTED_EDGE ( 'NONE', *, *, #46678, .T. ) ;
#11117=CARTESIAN_POINT ( 'NONE',  ( 92.34999999999999432, 88.47002178664753558, 79.33729166840096525 ) ) ;
#11118=CARTESIAN_POINT ( 'NONE',  ( -93.67500000000003979, 92.29496732002878900, 80.97770833506763211 ) ) ;
#11120=CARTESIAN_POINT ( 'NONE',  ( 94.99999999999998579, 87.33691857156068750, 84.88031250086714863 ) ) ;
#11123=DIRECTION ( 'NONE',  ( 1.000000000000000000, 0.000000000000000000, 0.000000000000000000 ) ) ;
#11127=CARTESIAN_POINT ( 'NONE',  ( 100.0010000000000190, -115.9999999999999716, 39.99999999999996447 ) ) ;
#11129=FACE_OUTER_BOUND ( 'NONE', #67867, .T. ) ;
#11131=DIRECTION ( 'NONE',  ( -0.000000000000000000, -0.000000000000000000, 1.000000000000000000 ) ) ;
#11142=CARTESIAN_POINT ( 'NONE',  ( -93.84685191531248449, -208.0026889286704943, 80.06489583420048461 ) ) ;
#11144=ADVANCED_FACE ( 'NONE', ( #33692 ), #69026, .F. ) ;
#11145=ORIENTED_EDGE ( 'NONE', *, *, #7164, .F. ) ;
#11146=CARTESIAN_POINT ( 'NONE',  ( -95.00000000000002842, 90.00000000000004263, 90.00000000000000000 ) ) ;
#11150=CARTESIAN_POINT ( 'NONE',  ( -95.62844927796862748, -212.5563123626481001, 74.98613922222868666 ) ) ;
#11160=CARTESIAN_POINT ( 'NONE',  ( 97.30629616937498838, 90.00000000000002842, 86.94406250086716170 ) ) ;
#11161=CARTESIAN_POINT ( 'NONE',  ( -92.69370383062498320, -208.6684592857803295, 88.90197916753382401 ) ) ;
#11165=CARTESIAN_POINT ( 'NONE',  ( -95.00000000000002842, 92.66308142843932671, 79.32406250086714294 ) ) ;
#11169=CARTESIAN_POINT ( 'NONE',  ( 96.32499999999998863, 87.70503267997126784, 83.22666666666665947 ) ) ;
#11173=CARTESIAN_POINT ( 'NONE',  ( 96.15314808468748708, -208.0026889286704943, 75.61989583420049144 ) ) ;
#11178=CARTESIAN_POINT ( 'NONE',  ( 100.0010000000000900, 64.99999999999997158, -290.0000000000000568 ) ) ;
#11182=CARTESIAN_POINT ( 'NONE',  ( 92.35000000000002274, -211.5299782133524502, 89.41791666666667027 ) ) ;
#11183=EDGE_CURVE ( 'NONE', #42834, #2120, #27682, .T. ) ;
#11196=CARTESIAN_POINT ( 'NONE',  ( 96.32499999999998863, -212.2949673200287179, 77.59104166840097605 ) ) ;
#11198=CARTESIAN_POINT ( 'NONE',  ( 97.64999999999997726, 88.47002178664753558, 83.27958333333333485 ) ) ;
#11200=CARTESIAN_POINT ( 'NONE',  ( 94.99999999999998579, 90.00000000000002842, 90.00000000000000000 ) ) ;
#11204=CARTESIAN_POINT ( 'NONE',  ( -96.32500000000001705, 87.70503267997129626, 88.91520833506763211 ) ) ;
#11206=CARTESIAN_POINT ( 'NONE',  ( -97.30629616937501680, 90.00000000000004263, 81.54656250086715374 ) ) ;
#11207=CARTESIAN_POINT ( 'NONE',  ( 92.69370383062498320, 91.33154071421968467, 76.88989583420047325 ) ) ;
#11208=VERTEX_POINT ( 'NONE', #39720 ) ;
#11212=CARTESIAN_POINT ( 'NONE',  ( -97.64999999999996305, -209.9999999999999716, 77.93499999999998806 ) ) ;
#11215=CARTESIAN_POINT ( 'NONE',  ( -92.69370383062498320, -209.9999999999999716, 79.16531250086714522 ) ) ;
#11223=CARTESIAN_POINT ( 'NONE',  ( -92.69370383062498320, -209.9999999999999716, 77.26031250086714408 ) ) ;
#11224=VERTEX_POINT ( 'NONE', #22419 ) ;
#11233=CARTESIAN_POINT ( 'NONE',  ( 93.84685191531248449, 91.99731107132950569, 85.72697916753379843 ) ) ;
#11235=CARTESIAN_POINT ( 'NONE',  ( -93.67500000000003979, 87.70503267997129626, 75.60666666666665492 ) ) ;
#11239=CARTESIAN_POINT ( 'NONE',  ( -92.35000000000003695, 89.99999997442942856, 84.04687500080852658 ) ) ;
#11242=VECTOR ( 'NONE', #73680, 1000.000000000000000 ) ;
#11243=( BOUNDED_CURVE ( )  B_SPLINE_CURVE ( 2, ( #7990, #59880, #4590, #67730, #9096, #39159, #15475 ),
 .UNSPECIFIED., .F., .F. ) 
 B_SPLINE_CURVE_WITH_KNOTS ( ( 3, 2, 2, 3 ),
 ( 0.3333333333333333703, 0.3402777777777777901, 0.3472222222222221544, 0.3541666666666665741 ),
 .UNSPECIFIED. ) 
 CURVE ( )  GEOMETRIC_REPRESENTATION_ITEM ( )  RATIONAL_B_SPLINE_CURVE ( ( 0.9999999999999988898, 0.8660254037844398178, 1.000000000000000000, 0.8660254037844387076, 1.000000000000000000, 0.8660254037844408170, 0.9999999999999978906 ) ) 
 REPRESENTATION_ITEM ( '' )  );
#11252=CARTESIAN_POINT ( 'NONE',  ( -93.67499999999998295, -207.7050326799711968, 83.43833333333333258 ) ) ;
#11254=( BOUNDED_CURVE ( )  B_SPLINE_CURVE ( 2, ( #17216, #22492, #73977, #46163, #23236, #57814, #6320 ),
 .UNSPECIFIED., .F., .F. ) 
 B_SPLINE_CURVE_WITH_KNOTS ( ( 3, 2, 2, 3 ),
 ( 0.06350193517735297499, 0.07055765540882327769, 0.07761342094970608008, 0.08466915177892291033 ),
 .UNSPECIFIED. ) 
 CURVE ( )  GEOMETRIC_REPRESENTATION_ITEM ( )  RATIONAL_B_SPLINE_CURVE ( ( 0.9999982793443948914, 0.8660262641177659537, 1.000000000000000000, 0.8660254037844387076, 1.000000000000000000, 0.8660260628881748524, 0.9999986817990127452 ) ) 
 REPRESENTATION_ITEM ( '' )  );
#11259=VECTOR ( 'NONE', #24515, 1000.000000000000000 ) ;
#11261=CARTESIAN_POINT ( 'NONE',  ( 95.00000000000000000, -212.6630814284392557, 86.15031250086714465 ) ) ;
#11263=ORIENTED_EDGE ( 'NONE', *, *, #45856, .T. ) ;
#11267=CARTESIAN_POINT ( 'NONE',  ( 97.30629616937498838, -209.9999999999999716, 79.16531250086714522 ) ) ;
#11269=CARTESIAN_POINT ( 'NONE',  ( 92.69370383062501162, -208.6684592857803011, 82.12864583420048348 ) ) ;
#11270=ORIENTED_EDGE ( 'NONE', *, *, #9955, .F. ) ;
#11279=CARTESIAN_POINT ( 'NONE',  ( 96.32499999999998863, -212.2949673200287179, 87.11604166840096752 ) ) ;
#11283=ORIENTED_EDGE ( 'NONE', *, *, #54318, .F. ) ;
#11284=CARTESIAN_POINT ( 'NONE',  ( -95.00000000000002842, 92.66308142843932671, 89.64281250086715147 ) ) ;
#11290=VERTEX_POINT ( 'NONE', #26013 ) ;
#11300=CARTESIAN_POINT ( 'NONE',  ( -97.30629616937501680, 91.33154071421968467, 75.14364583420049826 ) ) ;
#11303=CARTESIAN_POINT ( 'NONE',  ( 97.64999999999999147, -209.9999999999999716, 89.68250000000000455 ) ) ;
#11305=CARTESIAN_POINT ( 'NONE',  ( 94.99999999999998579, 93.05995642670504253, 75.23624999999998408 ) ) ;
#11306=CARTESIAN_POINT ( 'NONE',  ( -96.15314808468747287, -208.0026889286704943, 85.09197916753380753 ) ) ;
#11310=CARTESIAN_POINT ( 'NONE',  ( 92.35000000000006537, -208.4700217866474077, 88.04208333333330927 ) ) ;
#11311=CARTESIAN_POINT ( 'NONE',  ( -97.30629616937497417, -208.6684592857803295, 77.52489583420046415 ) ) ;
#11313=CARTESIAN_POINT ( 'NONE',  ( -97.64999999999996305, -209.9999999999999716, 88.73000000000000398 ) ) ;
#11317=CARTESIAN_POINT ( 'NONE',  ( -93.67500000000003979, 87.70503267997129626, 85.21104166840096639 ) ) ;
#11320=CARTESIAN_POINT ( 'NONE',  ( -97.30629616937501680, 90.00000000000004263, 80.11781250086713158 ) ) ;
#11324=PLANE ( 'NONE',  #49601 ) ;
#11331=CARTESIAN_POINT ( 'NONE',  ( -92.69370383062498320, -211.3315407142195852, 79.27114583420048177 ) ) ;
#11332=CARTESIAN_POINT ( 'NONE',  ( 97.64999999999999147, -209.9999999999999716, 90.00000000000000000 ) ) ;
#11342=ORIENTED_EDGE ( 'NONE', *, *, #25545, .T. ) ;
#11348=CARTESIAN_POINT ( 'NONE',  ( 96.15314808468748708, -208.0026889286704943, 88.79614583420047325 ) ) ;
#11349=CARTESIAN_POINT ( 'NONE',  ( -97.64999999999996305, -208.4700217866474645, 83.67645833506763609 ) ) ;
#11354=CARTESIAN_POINT ( 'NONE',  ( 92.35000000000006537, -211.5299782133524786, 89.41791666666667027 ) ) ;
#11358=CARTESIAN_POINT ( 'NONE',  ( -97.64999999978461176, -209.9999789922612479, 79.91868729551984529 ) ) ;
#11362=ORIENTED_EDGE ( 'NONE', *, *, #74284, .T. ) ;
#11363=( BOUNDED_CURVE ( )  B_SPLINE_CURVE ( 2, ( #721, #23612, #48385, #48754, #25086, #48023, #71676, #72052, #70935, #37493, #54401 ),
 .UNSPECIFIED., .F., .F. ) 
 B_SPLINE_CURVE_WITH_KNOTS ( ( 3, 2, 2, 2, 2, 3 ),
 ( 0.6985206468843488947, 0.6985207885473545542, 0.7055765540882368292, 0.7126323196291192152, 0.7196880851700017123, 0.7196881748034550386 ),
 .UNSPECIFIED. ) 
 CURVE ( )  GEOMETRIC_REPRESENTATION_ITEM ( )  RATIONAL_B_SPLINE_CURVE ( ( 0.9999946203249505672, 0.9999973101084687066, 1.000000000000000000, 0.8660254037844387076, 1.000000000000000000, 0.8660254037844387076, 1.000000000000000000, 0.8660254037844387076, 1.000000000000000000, 0.9999982980435435653, 0.9999965961303289852 ) ) 
 REPRESENTATION_ITEM ( '' )  );
#11370=EDGE_CURVE ( 'NONE', #68271, #62567, #52452, .T. ) ;
#11374=CARTESIAN_POINT ( 'NONE',  ( 94.99999999999998579, 87.33691857156068750, 83.45156250086714067 ) ) ;
#11376=CARTESIAN_POINT ( 'NONE',  ( 92.69370383062501162, -208.6684592857803011, 86.41489583420047893 ) ) ;
#11379=CARTESIAN_POINT ( 'NONE',  ( -97.64999999999996305, -211.5299782133524218, 81.24229166840096639 ) ) ;
#11385=CARTESIAN_POINT ( 'NONE',  ( -97.30629616937497417, -208.6684592857803011, 88.95489583420048518 ) ) ;
#11387=CARTESIAN_POINT ( 'NONE',  ( -92.69370383062502583, 88.66845928578038638, 85.62114583420047609 ) ) ;
#11390=CARTESIAN_POINT ( 'NONE',  ( 94.99999999999998579, 87.33691857156068750, 85.99156250086714692 ) ) ;
#11391=CARTESIAN_POINT ( 'NONE',  ( -92.69370383062504004, 90.00000000000004263, 83.61031250086713840 ) ) ;
#11392=B_SPLINE_CURVE_WITH_KNOTS ( 'NONE', 3,
 ( #31864, #20213, #20598, #43549 ),
 .UNSPECIFIED., .F., .F.,
 ( 4, 4 ),
 ( 2.446487931514449005E-06, 1.000000000000000000 ),
 .UNSPECIFIED. ) ;
#11394=CARTESIAN_POINT ( 'NONE',  ( -92.35000000000003695, 90.00000000000004263, 87.77749999999998920 ) ) ;
#11395=CARTESIAN_POINT ( 'NONE',  ( -97.30629616937501680, 90.00000000000004263, 89.80156250086714920 ) ) ;
#11397=CARTESIAN_POINT ( 'NONE',  ( 100.0010000000000900, 64.99999999999997158, -290.0000000000000568 ) ) ;
#11399=CARTESIAN_POINT ( 'NONE',  ( -93.84685191531247028, -211.9973110713294489, 87.94947916753380923 ) ) ;
#11407=CARTESIAN_POINT ( 'NONE',  ( -92.35000000000005116, 88.47002178664754979, 78.19958333333332234 ) ) ;
#11410=CARTESIAN_POINT ( 'NONE',  ( -92.34999999999999432, -209.9999999999999716, 88.41249999999999432 ) ) ;
#11412=CARTESIAN_POINT ( 'NONE',  ( -93.67500000000003979, 87.70503267997129626, 86.48104166840096241 ) ) ;
#11415=CARTESIAN_POINT ( 'NONE',  ( -97.30629616937501680, 90.00000000000004263, 77.57781250086713953 ) ) ;
#11421=AXIS2_PLACEMENT_3D ( 'NONE', #50532, #32118, #67456 ) ;
#11425=CARTESIAN_POINT ( 'NONE',  ( 92.69370383062498320, 91.33154071421968467, 77.04864583420048518 ) ) ;
#11427=CARTESIAN_POINT ( 'NONE',  ( -97.30629616937495996, -209.9999999999999716, 78.37156250086715659 ) ) ;
#11429=ORIENTED_EDGE ( 'NONE', *, *, #36655, .F. ) ;
#11435=CARTESIAN_POINT ( 'NONE',  ( -96.15314808468752972, 91.99731107132950569, 75.09072916753380866 ) ) ;
#11436=CARTESIAN_POINT ( 'NONE',  ( 97.30629616937498838, -209.9999999999999716, 81.70531250086713726 ) ) ;
#11442=CARTESIAN_POINT ( 'NONE',  ( -94.99999999999997158, -209.9999999999999716, 90.00000000000000000 ) ) ;
#11446=CARTESIAN_POINT ( 'NONE',  ( -94.99999999999997158, -206.9400435732949575, 83.49125000000000796 ) ) ;
#11451=ORIENTED_EDGE ( 'NONE', *, *, #65686, .F. ) ;
#11453=ORIENTED_EDGE ( 'NONE', *, *, #62752, .F. ) ;
#11455=( BOUNDED_CURVE ( )  B_SPLINE_CURVE ( 2, ( #24691, #64932, #70532, #19042, #63451, #28857, #51786 ),
 .UNSPECIFIED., .F., .F. ) 
 B_SPLINE_CURVE_WITH_KNOTS ( ( 3, 2, 2, 3 ),
 ( 0.3958333333333330373, 0.4027777777777774570, 0.4097222222222218768, 0.4166666666666662966 ),
 .UNSPECIFIED. ) 
 CURVE ( )  GEOMETRIC_REPRESENTATION_ITEM ( )  RATIONAL_B_SPLINE_CURVE ( ( 1.000000000000005329, 0.8660254037844333785, 1.000000000000000000, 0.8660254037844387076, 1.000000000000000000, 0.8660254037844462571, 0.9999999999999924505 ) ) 
 REPRESENTATION_ITEM ( '' )  );
#11456=CARTESIAN_POINT ( 'NONE',  ( 92.69370383062498320, 88.66845928578037217, 82.23447916753383424 ) ) ;
#11457=ADVANCED_FACE ( 'NONE', ( #32019 ), #73350, .F. ) ;
#11458=CARTESIAN_POINT ( 'NONE',  ( 93.67500000000001137, -212.2949673200287179, 77.40583333333331950 ) ) ;
#11466=CARTESIAN_POINT ( 'NONE',  ( -96.32499999999996021, -207.7050326799711968, 75.36854166840096525 ) ) ;
#11471=DIRECTION ( 'NONE',  ( -0.000000000000000000, -0.000000000000000000, 1.000000000000000000 ) ) ;
#11472=DIRECTION ( 'NONE',  ( -0.000000000000000000, -0.000000000000000000, 1.000000000000000000 ) ) ;
#11474=CARTESIAN_POINT ( 'NONE',  ( -92.34999999999999432, -211.5299782133524502, 82.08895833506764461 ) ) ;
#11480=CARTESIAN_POINT ( 'NONE',  ( 94.99999999999998579, 86.94004357329500010, 78.17312500173430578 ) ) ;
#11481=CARTESIAN_POINT ( 'NONE',  ( -92.35000000000005116, 91.52997821335253548, 80.92479166840098515 ) ) ;
#11484=CARTESIAN_POINT ( 'NONE',  ( 96.15314808468748708, 88.00268892867053694, 79.21822916753382060 ) ) ;
#11487=CARTESIAN_POINT ( 'NONE',  ( 97.65000000000000568, -211.5299782133524218, 79.54895833506762415 ) ) ;
#11489=ORIENTED_EDGE ( 'NONE', *, *, #20102, .T. ) ;
#11491=CARTESIAN_POINT ( 'NONE',  ( 97.65000000000000568, -208.4700217866474645, 77.03541666666666288 ) ) ;
#11498=CARTESIAN_POINT ( 'NONE',  ( -92.69370383062498320, -211.3315407142195852, 82.44614583420049314 ) ) ;
#11502=CIRCLE ( 'NONE', #48697, 23.50000000000000355 ) ;
#11503=CARTESIAN_POINT ( 'NONE',  ( -97.51367041768831712, -210.0000000000000284, 74.91808492278045151 ) ) ;
#11512=CARTESIAN_POINT ( 'NONE',  ( -92.34999999999999432, -209.9999999999999716, 90.00000000000000000 ) ) ;
#11516=CARTESIAN_POINT ( 'NONE',  ( 97.30629616937498838, 90.00000000000002842, 88.21406250086714351 ) ) ;
#11517=CARTESIAN_POINT ( 'NONE',  ( -97.30629616937497417, -211.3315407142195852, 88.58447916753382856 ) ) ;
#11521=CARTESIAN_POINT ( 'NONE',  ( -93.84685191531254134, 91.99731107132950569, 81.17614583420048291 ) ) ;
#11532=CARTESIAN_POINT ( 'NONE',  ( 97.30629616937498838, -209.9999999999999716, 74.87906250086714977 ) ) ;
#11535=CARTESIAN_POINT ( 'NONE',  ( 96.15314808468750130, -211.9973110713294489, 84.93322916753382401 ) ) ;
#11536=CARTESIAN_POINT ( 'NONE',  ( -97.65000000000004832, -208.4700217866474929, 81.05708333333332405 ) ) ;
#11540=EDGE_CURVE ( 'NONE', #64759, #61415, #39157, .T. ) ;
#11541=AXIS2_PLACEMENT_3D ( 'NONE', #27189, #61807, #33208 ) ;
#11543=CARTESIAN_POINT ( 'NONE',  ( 92.35000000000002274, -208.4700217866474645, 89.31208333333333371 ) ) ;
#11553=CARTESIAN_POINT ( 'NONE',  ( 96.32499999999998863, -212.2949673200287179, 76.95604166840095672 ) ) ;
#11554=CARTESIAN_POINT ( 'NONE',  ( 92.34999999999999432, 91.52997821335252127, 79.15208333333332291 ) ) ;
#11563=CARTESIAN_POINT ( 'NONE',  ( -93.84685191531252713, 88.00268892867056536, 81.12322916753382174 ) ) ;
#11564=CARTESIAN_POINT ( 'NONE',  ( 97.30629616937498838, 90.00000000000002842, 79.80031250086713612 ) ) ;
#11565=VERTEX_POINT ( 'NONE', #66257 ) ;
#11572=CARTESIAN_POINT ( 'NONE',  ( -93.84685191531247028, -211.9973110713294489, 77.78947916753381264 ) ) ;
#11578=CARTESIAN_POINT ( 'NONE',  ( -92.34999999999999432, -209.9999999999999716, 78.25249999999999773 ) ) ;
#11580=CARTESIAN_POINT ( 'NONE',  ( -96.15314808468747287, -208.0026889286704943, 77.47197916753380298 ) ) ;
#11584=DIRECTION ( 'NONE',  ( -1.000000000000000000, -1.343011723336883198E-16, 0.000000000000000000 ) ) ;
#11588=CARTESIAN_POINT ( 'NONE',  ( 92.69370383062498320, 90.00000000000002842, 84.56281250086713897 ) ) ;
#11590=CARTESIAN_POINT ( 'NONE',  ( -93.67500000000003979, 87.70503267997129626, 88.30666666666665776 ) ) ;
#11597=CARTESIAN_POINT ( 'NONE',  ( 94.99999999999998579, 86.94004357329502852, 78.72875000000001933 ) ) ;
#11598=EDGE_CURVE ( 'NONE', #16867, #56779, #15473, .T. ) ;
#11599=AXIS2_PLACEMENT_3D ( 'NONE', #51592, #1252, #69980 ) ;
#11601=CARTESIAN_POINT ( 'NONE',  ( -96.15314808468751551, 88.00268892867056536, 88.47864583420047779 ) ) ;
#11609=DIRECTION ( 'NONE',  ( -1.000000000000000000, -0.000000000000000000, -0.000000000000000000 ) ) ;
#11614=CARTESIAN_POINT ( 'NONE',  ( 97.30629616937498838, -209.9999999999999716, 86.94406250086716170 ) ) ;
#11619=CARTESIAN_POINT ( 'NONE',  ( 92.34999999999999432, 90.00000000000002842, 90.00000000000000000 ) ) ;
#11623=CARTESIAN_POINT ( 'NONE',  ( 93.84685191531251292, -211.9973110713294489, 79.58864583420047722 ) ) ;
#11625=EDGE_LOOP ( 'NONE', ( #69829, #68459, #13767, #64291, #68604, #10932, #28489, #60152, #25452, #61000, #7114, #63933, #21051, #41615, #33359, #30341, #53639, #64074, #62983, #16200, #135, #62453, #16758, #50826, #3871, #65365, #48809, #41419, #56696, #36976, #73571, #29929, #10710, #7019, #51069, #46147, #67338, #1741, #30296, #72460, #40167, #31792, #11048, #41782, #26718, #33387, #64919, #41004, #47835, #70325 ) ) ;
#11626=CARTESIAN_POINT ( 'NONE',  ( 95.00000000000000000, -207.3369185715606307, 82.65781250086715204 ) ) ;
#11637=CARTESIAN_POINT ( 'NONE',  ( 96.32499999999998863, -212.2949673200287179, 87.75104166840095843 ) ) ;
#11640=EDGE_CURVE ( 'NONE', #23659, #13520, #43100, .T. ) ;
#11644=ORIENTED_EDGE ( 'NONE', *, *, #53135, .F. ) ;
#11658=CARTESIAN_POINT ( 'NONE',  ( -92.35000000000005116, 91.52997821335253548, 87.19541666666667368 ) ) ;
#11660=CARTESIAN_POINT ( 'NONE',  ( 97.30629616937497417, 89.06968361095755427, 74.68334086212732359 ) ) ;
#11662=( BOUNDED_CURVE ( )  B_SPLINE_CURVE ( 2, ( #72430, #44629, #33701, #10025, #38608, #55148, #56655, #49867, #22052 ),
 .UNSPECIFIED., .F., .F. ) 
 B_SPLINE_CURVE_WITH_KNOTS ( ( 3, 2, 2, 2, 3 ),
 ( 0.4868478063929146393, 0.4939035878617654141, 0.5009593534026473005, 0.5080151189435291315, 0.5080151867253831499 ),
 .UNSPECIFIED. ) 
 CURVE ( )  GEOMETRIC_REPRESENTATION_ITEM ( )  RATIONAL_B_SPLINE_CURVE ( ( 1.000000000000000000, 0.8660254037844387076, 1.000000000000000000, 0.8660254037844387076, 1.000000000000000000, 0.8660254037844387076, 1.000000000000000000, 0.9999987129608440828, 0.9999974259464162740 ) ) 
 REPRESENTATION_ITEM ( '' )  );
#11665=CARTESIAN_POINT ( 'NONE',  ( -97.30629616937495996, -209.9999999999999716, 86.46781250086714010 ) ) ;
#11666=ORIENTED_EDGE ( 'NONE', *, *, #57368, .T. ) ;
#11667=CARTESIAN_POINT ( 'NONE',  ( 92.35000000006147047, -209.9999881782113107, 76.10900611559200968 ) ) ;
#11670=CARTESIAN_POINT ( 'NONE',  ( -96.15314808468745866, -211.9973110713294489, 75.14364583420046984 ) ) ;
#11671=DIRECTION ( 'NONE',  ( 1.000000000000000000, 0.000000000000000000, 0.000000000000000000 ) ) ;
#11678=CARTESIAN_POINT ( 'NONE',  ( -93.84685191531252713, 88.00268892867056536, 79.69447916753379957 ) ) ;
#11682=CARTESIAN_POINT ( 'NONE',  ( -96.32499999999996021, -207.7050326799711968, 80.44854166840097776 ) ) ;
#11688=CARTESIAN_POINT ( 'NONE',  ( 97.64999999999999147, -210.0000000024471092, 75.15687493081163950 ) ) ;
#11689=CARTESIAN_POINT ( 'NONE',  ( -97.65000000000001990, 91.52997821335253548, 85.58145833506763722 ) ) ;
#11690=CARTESIAN_POINT ( 'NONE',  ( -97.30629616937495996, -209.9999999999999716, 77.73656250086715147 ) ) ;
#11710=CARTESIAN_POINT ( 'NONE',  ( -92.35000000000678710, 90.00000598221780024, 82.14187520865721126 ) ) ;
#11724=DIRECTION ( 'NONE',  ( -0.000000000000000000, -0.000000000000000000, -1.000000000000000000 ) ) ;
#11729=CARTESIAN_POINT ( 'NONE',  ( 92.48104893696866213, 89.82936612246388108, 74.92125785461007581 ) ) ;
#11732=CARTESIAN_POINT ( 'NONE',  ( 96.15314808468748708, 91.99731107132950569, 84.35114583420048007 ) ) ;
#11734=CARTESIAN_POINT ( 'NONE',  ( 96.15314808468750130, -211.9973110713294489, 82.86947916753379673 ) ) ;
#11738=CARTESIAN_POINT ( 'NONE',  ( -97.64999999999996305, -209.9999999999999716, 90.00000000000000000 ) ) ;
#11739=CYLINDRICAL_SURFACE ( 'NONE', #10386, 2.649999999999999467 ) ;
#11742=CARTESIAN_POINT ( 'NONE',  ( -93.84685191531247028, -211.9973110713294489, 84.13947916753380696 ) ) ;
#11743=CARTESIAN_POINT ( 'NONE',  ( -96.15314808468751551, 88.00268892867056536, 83.55739583420049144 ) ) ;
#11745=CARTESIAN_POINT ( 'NONE',  ( 92.69370383062498320, 90.00000000000002842, 83.92781250086714806 ) ) ;
#11746=CARTESIAN_POINT ( 'NONE',  ( -92.69370383062502583, 91.33154071421968467, 83.66322916753379957 ) ) ;
#11747=EDGE_LOOP ( 'NONE', ( #23670, #47518, #39278, #55192 ) ) ;
#11748=CARTESIAN_POINT ( 'NONE',  ( -97.64999999989197477, 90.00001510551047090, 78.64888723592453346 ) ) ;
#11752=CARTESIAN_POINT ( 'NONE',  ( 97.64999999999997726, 91.52997821335254969, 87.19541666666667368 ) ) ;
#11753=CARTESIAN_POINT ( 'NONE',  ( -97.30629616937497417, -208.6684592857803295, 85.77989583420048803 ) ) ;
#11758=CARTESIAN_POINT ( 'NONE',  ( 97.64999999999999147, 90.00000000000002842, 80.15749999999999886 ) ) ;
#11762=CARTESIAN_POINT ( 'NONE',  ( -92.35000000000003695, 90.00000000000004263, 76.98250000000000171 ) ) ;
#11763=CARTESIAN_POINT ( 'NONE',  ( -96.32499999999996021, -212.2949673200287179, 78.67583333333332973 ) ) ;
#11767=CARTESIAN_POINT ( 'NONE',  ( 92.35000000000000853, -208.4700217866474645, 77.96145833506763267 ) ) ;
#11770=CARTESIAN_POINT ( 'NONE',  ( -93.84685191531252713, 88.00268892867056536, 79.69447916753379957 ) ) ;
#11781=CARTESIAN_POINT ( 'NONE',  ( -92.69370383062498320, -209.9999999999999716, 88.21406250086714351 ) ) ;
#11786=CARTESIAN_POINT ( 'NONE',  ( 97.30629616937498838, 91.33154071421968467, 76.20197916753382117 ) ) ;
#11787=CARTESIAN_POINT ( 'NONE',  ( -92.69370383062498320, -211.3315407142195852, 79.90614583420048689 ) ) ;
#11792=CARTESIAN_POINT ( 'NONE',  ( 95.00000000000000000, -213.0599564267049857, 78.80812500173429669 ) ) ;
#11794=CARTESIAN_POINT ( 'NONE',  ( 96.15314808468748708, -208.0026889286704943, 75.46114583420047950 ) ) ;
#11798=CARTESIAN_POINT ( 'NONE',  ( -97.65000000000001990, 90.00000000000004263, 75.39499999999999602 ) ) ;
#11799=EDGE_LOOP ( 'NONE', ( #19878, #64626, #27386, #6020 ) ) ;
#11801=ORIENTED_EDGE ( 'NONE', *, *, #25029, .F. ) ;
#11815=CARTESIAN_POINT ( 'NONE',  ( 97.30629616937498838, 88.66845928578037217, 83.08114583420048405 ) ) ;
#11816=DIRECTION ( 'NONE',  ( -1.000000000000000000, 0.000000000000000000, 0.000000000000000000 ) ) ;
#11817=VERTEX_POINT ( 'NONE', #65060 ) ;
#11820=ORIENTED_EDGE ( 'NONE', *, *, #4954, .F. ) ;
#11821=VERTEX_POINT ( 'NONE', #59407 ) ;
#11825=CARTESIAN_POINT ( 'NONE',  ( -0.0004442498525516064278, 0.001194404164626844313, -64.00000000000000000 ) ) ;
#11828=PLANE ( 'NONE',  #17451 ) ;
#11829=DIRECTION ( 'NONE',  ( 1.000000000000000000, 0.000000000000000000, 0.000000000000000000 ) ) ;
#11834=CARTESIAN_POINT ( 'NONE',  ( -96.32499999999996021, -207.7050326799711968, 79.17854166840096752 ) ) ;
#11838=CARTESIAN_POINT ( 'NONE',  ( 94.99999999999998579, 93.05995642670504253, 78.49062500173430124 ) ) ;
#11839=CARTESIAN_POINT ( 'NONE',  ( -97.65000000000001990, 88.47002178664754979, 80.60729166840097548 ) ) ;
#11842=CARTESIAN_POINT ( 'NONE',  ( 94.99999999999998579, 92.66308142843935514, 81.38781250086715602 ) ) ;
#11857=EDGE_CURVE ( 'NONE', #63185, #50665, #26288, .T. ) ;
#11859=CARTESIAN_POINT ( 'NONE',  ( -93.09170270117142820, -211.8387227684682159, 74.99954709728268654 ) ) ;
#11860=CARTESIAN_POINT ( 'NONE',  ( -94.99999999999997158, -207.3369185715606307, 78.21281250086717307 ) ) ;
#11867=CARTESIAN_POINT ( 'NONE',  ( -96.91066463016758803, -211.7387787020483358, 74.95660481729511559 ) ) ;
#11871=CARTESIAN_POINT ( 'NONE',  ( 96.15314808468748708, 88.00268892867053694, 75.88447916753381151 ) ) ;
#11878=CARTESIAN_POINT ( 'NONE',  ( -97.64999999999996305, -209.9999999999999716, 89.36499999999999488 ) ) ;
#11880=CARTESIAN_POINT ( 'NONE',  ( 93.84685191531248449, 91.99731107132950569, 86.52072916753382970 ) ) ;
#11887=CARTESIAN_POINT ( 'NONE',  ( -97.30629616937501680, 91.33154071421968467, 81.33489583420048064 ) ) ;
#11893=EDGE_CURVE ( 'NONE', #63185, #9070, #9932, .T. ) ;
#11897=( BOUNDED_CURVE ( )  B_SPLINE_CURVE ( 2, ( #47310, #70213, #59325, #7818, #35874, #41164, #52813 ),
 .UNSPECIFIED., .F., .F. ) 
 B_SPLINE_CURVE_WITH_KNOTS ( ( 3, 2, 2, 3 ),
 ( 0.3958333333333330373, 0.4027777777777774570, 0.4097222222222218768, 0.4166666666666662966 ),
 .UNSPECIFIED. ) 
 CURVE ( )  GEOMETRIC_REPRESENTATION_ITEM ( )  RATIONAL_B_SPLINE_CURVE ( ( 1.000000000000005329, 0.8660254037844333785, 1.000000000000000000, 0.8660254037844387076, 1.000000000000000000, 0.8660254037844462571, 0.9999999999999924505 ) ) 
 REPRESENTATION_ITEM ( '' )  );
#11898=DIRECTION ( 'NONE',  ( -0.000000000000000000, -0.000000000000000000, 1.000000000000000000 ) ) ;
#11907=CARTESIAN_POINT ( 'NONE',  ( 96.15314808468750130, -211.9973110713294489, 80.48822916753381662 ) ) ;
#11909=CARTESIAN_POINT ( 'NONE',  ( -94.99999999999997158, -206.9400435732949575, 77.22062500173429100 ) ) ;
#11910=CARTESIAN_POINT ( 'NONE',  ( 92.34999999999999432, 91.52997821335252127, 83.67645833506763609 ) ) ;
#11911=AXIS2_PLACEMENT_3D ( 'NONE', #12044, #5687, #443 ) ;
#11913=CARTESIAN_POINT ( 'NONE',  ( 97.64999999999997726, -211.5299782133524502, 85.18458333333332178 ) ) ;
#11914=VECTOR ( 'NONE', #25850, 1000.000000000000000 ) ;
#11922=CARTESIAN_POINT ( 'NONE',  ( -92.69370383062504004, 90.00000000000004263, 88.21406250086714351 ) ) ;
#11926=CARTESIAN_POINT ( 'NONE',  ( 97.64999999999997726, -208.4700217866474645, 78.38479166840096468 ) ) ;
#11927=CARTESIAN_POINT ( 'NONE',  ( 93.67499999999998295, 92.29496732002878900, 77.19416666666666060 ) ) ;
#11929=LINE ( 'NONE', #51048, #65951 ) ;
#11934=CARTESIAN_POINT ( 'NONE',  ( -93.67500000000003979, 87.70503267997129626, 88.38604166840097776 ) ) ;
#11935=CARTESIAN_POINT ( 'NONE',  ( -92.69370383062505425, 91.33154071421968467, 81.28197916753381946 ) ) ;
#11936=CARTESIAN_POINT ( 'NONE',  ( 93.84685191531248449, 88.00268892867053694, 88.63739583420048973 ) ) ;
#11938=DIRECTION ( 'NONE',  ( 0.8896955516311735312, 0.000000000000000000, -0.4565542962317865050 ) ) ;
#11941=CARTESIAN_POINT ( 'NONE',  ( -92.69370383062502583, 90.00000000000007105, 74.79348190356851944 ) ) ;
#11942=ORIENTED_EDGE ( 'NONE', *, *, #39201, .F. ) ;
#11944=AXIS2_PLACEMENT_3D ( 'NONE', #16756, #15640, #38574 ) ;
#11945=CARTESIAN_POINT ( 'NONE',  ( -97.30629616937495996, -209.9999999999999716, 76.94281250086713442 ) ) ;
#11948=ORIENTED_EDGE ( 'NONE', *, *, #51071, .F. ) ;
#11949=EDGE_CURVE ( 'NONE', #19312, #2794, #54868, .T. ) ;
#11951=VECTOR ( 'NONE', #15531, 1000.000000000000000 ) ;
#11956=CARTESIAN_POINT ( 'NONE',  ( -93.67499999999998295, -212.2949673200287179, 78.14666666666667538 ) ) ;
#11958=CARTESIAN_POINT ( 'NONE',  ( -97.30629616937495996, -209.9999999999999716, 75.67281250086713840 ) ) ;
#11962=CARTESIAN_POINT ( 'NONE',  ( -97.65000000000000568, 89.99997747911959323, 86.26937578065384571 ) ) ;
#11964=EDGE_CURVE ( 'NONE', #2629, #25433, #12345, .T. ) ;
#11965=EDGE_CURVE ( 'NONE', #18479, #44748, #27714, .T. ) ;
#11969=CARTESIAN_POINT ( 'NONE',  ( 92.69370383062498320, 91.33154071421968467, 84.50989583420049200 ) ) ;
#11979=CARTESIAN_POINT ( 'NONE',  ( 97.65000000000000568, -208.4700217866474645, 85.36979166840096411 ) ) ;
#11983=CARTESIAN_POINT ( 'NONE',  ( -96.15314808468752972, 91.99731107132950569, 89.53697916753381492 ) ) ;
#11984=LINE ( 'NONE', #34928, #19057 ) ;
#11985=VECTOR ( 'NONE', #62319, 1000.000000000000000 ) ;
#11999=CARTESIAN_POINT ( 'NONE',  ( 92.69370383062501162, -209.9999999999999716, 84.08656250086716000 ) ) ;
#12004=FACE_OUTER_BOUND ( 'NONE', #22481, .T. ) ;
#12009=CARTESIAN_POINT ( 'NONE',  ( 95.00000000000000000, -212.6630814284392557, 82.34031250086714238 ) ) ;
#12017=CARTESIAN_POINT ( 'NONE',  ( -97.65000000000006253, 91.52997821335252127, 84.23208333333334963 ) ) ;
#12018=CARTESIAN_POINT ( 'NONE',  ( 95.00000000000000000, -206.9400435732949575, 87.38062500173430180 ) ) ;
#12026=AXIS2_PLACEMENT_3D ( 'NONE', #24370, #2216, #70572 ) ;
#12034=VERTEX_POINT ( 'NONE', #9 ) ;
#12040=CARTESIAN_POINT ( 'NONE',  ( -93.67500000000003979, 92.29496732002878900, 89.15333333333333599 ) ) ;
#12042=CARTESIAN_POINT ( 'NONE',  ( 96.15314808468748708, 91.99731107132950569, 74.82614583420047438 ) ) ;
#12044=CARTESIAN_POINT ( 'NONE',  ( -0.0004442498525516064278, 0.001194404164626844313, 127.4927882439603195 ) ) ;
#12045=CARTESIAN_POINT ( 'NONE',  ( -97.30629616937497417, -211.3315407142195852, 87.15572916753380639 ) ) ;
#12051=CARTESIAN_POINT ( 'NONE',  ( -97.30629616937495996, -209.9999999999999716, 76.30781250086714351 ) ) ;
#12062=CARTESIAN_POINT ( 'NONE',  ( 92.34999999999999432, 90.00000000000002842, 88.09499999999999886 ) ) ;
#12063=CARTESIAN_POINT ( 'NONE',  ( -97.30629616937501680, 91.33154071421968467, 76.88989583420047325 ) ) ;
#12069=CARTESIAN_POINT ( 'NONE',  ( -97.64999999990722301, -209.9999861897314304, 80.55392363651652943 ) ) ;
#12072=CARTESIAN_POINT ( 'NONE',  ( 97.65000000000000568, -211.5299782133524218, 86.53395833506763779 ) ) ;
#12076=CARTESIAN_POINT ( 'NONE',  ( -93.67499999999998295, -207.7050326799711968, 89.78833333333332689 ) ) ;
#12077=DIRECTION ( 'NONE',  ( -0.000000000000000000, -0.000000000000000000, 1.000000000000000000 ) ) ;
#12078=ADVANCED_FACE ( 'NONE', ( #41289 ), #55352, .F. ) ;
#12080=EDGE_CURVE ( 'NONE', #44189, #54372, #12700, .T. ) ;
#12087=CARTESIAN_POINT ( 'NONE',  ( -94.99999999999997158, -209.9999999999999716, 90.00000000000000000 ) ) ;
#12092=CARTESIAN_POINT ( 'NONE',  ( 92.69370383062501162, -211.3315407142195852, 86.52072916753381548 ) ) ;
#12093=CARTESIAN_POINT ( 'NONE',  ( -92.35000000000005116, 91.52997821335253548, 82.19479166840095274 ) ) ;
#12100=CARTESIAN_POINT ( 'NONE',  ( -97.30629616937501680, 88.66845928578038638, 79.69447916753381378 ) ) ;
#12109=( BOUNDED_CURVE ( )  B_SPLINE_CURVE ( 2, ( #35080, #22700, #45645, #5784, #41458, #68565, #63295 ),
 .UNSPECIFIED., .F., .F. ) 
 B_SPLINE_CURVE_WITH_KNOTS ( ( 3, 2, 2, 3 ),
 ( 0.02116741234826251261, 0.02822306216352946096, 0.03527882770441181925, 0.04233441017594418571 ),
 .UNSPECIFIED. ) 
 CURVE ( )  GEOMETRIC_REPRESENTATION_ITEM ( )  RATIONAL_B_SPLINE_CURVE ( ( 0.9999956052852916333, 0.8660276011778336169, 1.000000000000000000, 0.8660254037844387076, 1.000000000000000000, 0.8660288798979943747, 0.9999930479532715966 ) ) 
 REPRESENTATION_ITEM ( '' )  );
#12114=CARTESIAN_POINT ( 'NONE',  ( 96.15314808468748708, 91.99731107132950569, 86.25614583420048120 ) ) ;
#12116=CARTESIAN_POINT ( 'NONE',  ( 95.00000000000000000, -212.6630814284392557, 83.45156250086714067 ) ) ;
#12121=CARTESIAN_POINT ( 'NONE',  ( 97.64999999999999147, -209.9999999999999716, 78.88750000000000284 ) ) ;
#12124=CARTESIAN_POINT ( 'NONE',  ( 2.499999999999979572, -90.00000000000000000, -280.0000000000000000 ) ) ;
#12125=CARTESIAN_POINT ( 'NONE',  ( -92.69370383062498320, -211.3315407142195852, 84.19239583420046813 ) ) ;
#12126=CARTESIAN_POINT ( 'NONE',  ( -95.00000000000002842, 92.66308142843932671, 81.38781250086715602 ) ) ;
#12128=CARTESIAN_POINT ( 'NONE',  ( 97.30629616937498838, 90.00000000000002842, 84.88031250086713442 ) ) ;
#12135=CARTESIAN_POINT ( 'NONE',  ( -94.99999999999997158, -207.3369185715606307, 85.67406250086715147 ) ) ;
#12141=CARTESIAN_POINT ( 'NONE',  ( 93.67499999999998295, 92.29496732002878900, 80.36916666666665776 ) ) ;
#12143=ORIENTED_EDGE ( 'NONE', *, *, #5398, .F. ) ;
#12144=CARTESIAN_POINT ( 'NONE',  ( -97.65000000000001990, 88.47002178664754979, 77.35291666666665833 ) ) ;
#12146=CARTESIAN_POINT ( 'NONE',  ( -92.69370383062502583, 91.33154071421968467, 88.74322916753379786 ) ) ;
#12147=CARTESIAN_POINT ( 'NONE',  ( 97.65000000000009095, -208.4700217866474929, 80.84541666666663673 ) ) ;
#12150=CARTESIAN_POINT ( 'NONE',  ( -93.67499999999998295, -207.7050326799711968, 78.35833333333333428 ) ) ;
#12152=CARTESIAN_POINT ( 'NONE',  ( -93.84685191531254134, 91.99731107132950569, 78.63614583420047666 ) ) ;
#12162=CARTESIAN_POINT ( 'NONE',  ( -93.84685191531248449, -208.0026889286704943, 87.68489583420048916 ) ) ;
#12169=CARTESIAN_POINT ( 'NONE',  ( 96.15314808468748708, 91.99731107132950569, 76.88989583420048746 ) ) ;
#12170=CARTESIAN_POINT ( 'NONE',  ( -97.30629616937497417, -211.3315407142195852, 75.88447916753382572 ) ) ;
#12176=CARTESIAN_POINT ( 'NONE',  ( -95.00000000000002842, 87.33691857156074434, 75.99031250086716227 ) ) ;
#12177=CARTESIAN_POINT ( 'NONE',  ( 96.15314808468748708, -208.0026889286704943, 78.00114583420048575 ) ) ;
#12189=VERTEX_POINT ( 'NONE', #25100 ) ;
#12194=CARTESIAN_POINT ( 'NONE',  ( 96.15314808468748708, 91.99731107132950569, 83.87489583420048689 ) ) ;
#12195=CARTESIAN_POINT ( 'NONE',  ( 96.90829729882592858, -211.8387227684709444, 74.99909419456535886 ) ) ;
#12207=EDGE_CURVE ( 'NONE', #71079, #63717, #15199, .T. ) ;
#12211=CARTESIAN_POINT ( 'NONE',  ( 96.32499999999998863, -212.2949673200287179, 87.11604166840096752 ) ) ;
#12212=CARTESIAN_POINT ( 'NONE',  ( 1.243286885786405054E-17, -120.0000000000000000, -80.00000000000001421 ) ) ;
#12216=CARTESIAN_POINT ( 'NONE',  ( -97.64999999999994884, -208.4700217866474645, 79.23145833506762870 ) ) ;
#12220=CARTESIAN_POINT ( 'NONE',  ( 96.32499999999997442, 92.29496732002878900, 79.07270833506763097 ) ) ;
#12221=CARTESIAN_POINT ( 'NONE',  ( -92.35000000000005116, 88.47002178664754979, 78.27895833506762813 ) ) ;
#12224=CARTESIAN_POINT ( 'NONE',  ( 94.99999999999998579, 92.66308142843935514, 78.84781250086714977 ) ) ;
#12225=CARTESIAN_POINT ( 'NONE',  ( 97.64999999999999147, 90.00000000000002842, 75.71250000000000568 ) ) ;
#12227=FACE_OUTER_BOUND ( 'NONE', #52042, .T. ) ;
#12235=EDGE_CURVE ( 'NONE', #16429, #58346, #73821, .T. ) ;
#12241=CARTESIAN_POINT ( 'NONE',  ( -96.15314808468747287, -208.0026889286704943, 76.99572916753382401 ) ) ;
#12255=CARTESIAN_POINT ( 'NONE',  ( -92.34999999999999432, -211.5299782133524218, 85.26395833506762756 ) ) ;
#12257=LINE ( 'NONE', #65257, #28550 ) ;
#12260=CARTESIAN_POINT ( 'NONE',  ( 92.69370383062498320, 91.33154071421968467, 86.57364583420047666 ) ) ;
#12262=CARTESIAN_POINT ( 'NONE',  ( -97.64998576286770060, -211.5299864331645665, 75.52729223699085992 ) ) ;
#12263=EDGE_LOOP ( 'NONE', ( #59382, #34660, #16257, #46040 ) ) ;
#12265=CARTESIAN_POINT ( 'NONE',  ( -92.69370383062505425, 88.66845928578038638, 75.30239583420048177 ) ) ;
#12266=AXIS2_PLACEMENT_3D ( 'NONE', #66027, #36697, #8121 ) ;
#12268=CARTESIAN_POINT ( 'NONE',  ( 96.15314808468748708, -208.0026889286704943, 87.52614583420047722 ) ) ;
#12277=CARTESIAN_POINT ( 'NONE',  ( 97.30629616937498838, -211.3315407142195852, 83.08114583420048405 ) ) ;
#12278=CARTESIAN_POINT ( 'NONE',  ( 92.34999999999999432, 91.52997821335252127, 89.94708333333332462 ) ) ;
#12279=FACE_OUTER_BOUND ( 'NONE', #6064, .T. ) ;
#12284=CARTESIAN_POINT ( 'NONE',  ( 97.64999999999997726, -211.5299782133524502, 83.91458333333333997 ) ) ;
#12287=MECHANICAL_DESIGN_GEOMETRIC_PRESENTATION_REPRESENTATION('',(#1501),#48311);
#12293=CARTESIAN_POINT ( 'NONE',  ( -95.00000000000002842, 87.33691857156074434, 88.05531250086716000 ) ) ;
#12294=ADVANCED_FACE ( 'NONE', ( #61918, #644 ), #69038, .T. ) ;
#12297=CARTESIAN_POINT ( 'NONE',  ( 92.35000000000002274, -208.4700217866474645, 76.69145833506763665 ) ) ;
#12298=CARTESIAN_POINT ( 'NONE',  ( 94.99999999999998579, 93.05995642670504253, 78.41125000000000966 ) ) ;
#12300=CARTESIAN_POINT ( 'NONE',  ( 92.35000000000000853, 91.52997821335253548, 79.78708333333331382 ) ) ;
#12301=VECTOR ( 'NONE', #25742, 1000.000000000000000 ) ;
#12305=CARTESIAN_POINT ( 'NONE',  ( -92.35000000000005116, 91.52997821335253548, 88.54479166840097548 ) ) ;
#12307=CARTESIAN_POINT ( 'NONE',  ( -96.15314808468752972, 91.99731107132950569, 82.07572916753382231 ) ) ;
#12309=CARTESIAN_POINT ( 'NONE',  ( 97.30629616937498838, 90.00000000000002842, 75.35531250086714294 ) ) ;
#12319=CARTESIAN_POINT ( 'NONE',  ( -97.30629616937497417, -208.6684592857803011, 74.98489583420048632 ) ) ;
#12328=ORIENTED_EDGE ( 'NONE', *, *, #44729, .T. ) ;
#12329=CARTESIAN_POINT ( 'NONE',  ( -92.69370383062498320, -209.9999999999999716, 86.94406250086716170 ) ) ;
#12330=ORIENTED_EDGE ( 'NONE', *, *, #27570, .F. ) ;
#12337=CARTESIAN_POINT ( 'NONE',  ( 96.15314808468748708, 88.00268892867053694, 84.13947916753380696 ) ) ;
#12343=CARTESIAN_POINT ( 'NONE',  ( -96.32500000000001705, 92.29496732002878900, 84.25854166840096582 ) ) ;
#12345=( BOUNDED_CURVE ( )  B_SPLINE_CURVE ( 2, ( #9749, #55611, #4133, #27024, #72876, #62387, #69132 ),
 .UNSPECIFIED., .F., .F. ) 
 B_SPLINE_CURVE_WITH_KNOTS ( ( 3, 2, 2, 3 ),
 ( 0.4656806970056959760, 0.4727362912391188665, 0.4797920567800012526, 0.4868478063929145838 ),
 .UNSPECIFIED. ) 
 CURVE ( )  GEOMETRIC_REPRESENTATION_ITEM ( )  RATIONAL_B_SPLINE_CURVE ( ( 0.9999934945994550795, 0.8660286565636856615, 1.000000000000000000, 0.8660254037844387076, 1.000000000000000000, 0.8660254037844387076, 1.000000000000000000 ) ) 
 REPRESENTATION_ITEM ( '' )  );
#12348=CARTESIAN_POINT ( 'NONE',  ( -97.30629616937501680, 90.00000000000004263, 89.00781250086714635 ) ) ;
#12349=DIRECTION ( 'NONE',  ( -0.000000000000000000, -0.000000000000000000, 1.000000000000000000 ) ) ;
#12354=AXIS2_PLACEMENT_3D ( 'NONE', #20781, #33535, #73009 ) ;
#12357=CARTESIAN_POINT ( 'NONE',  ( 97.65000000000000568, 91.52997821335252127, 77.03541666666666288 ) ) ;
#12358=CARTESIAN_POINT ( 'NONE',  ( 92.35000000000000853, -209.9999999999999716, 88.73000000000000398 ) ) ;
#12362=CARTESIAN_POINT ( 'NONE',  ( 93.84685191531251292, -211.9973110713294489, 85.46239583420047836 ) ) ;
#12366=EDGE_CURVE ( 'NONE', #63593, #18610, #40454, .T. ) ;
#12367=CARTESIAN_POINT ( 'NONE',  ( -93.67499999999998295, -207.7050326799711968, 85.97833333333332462 ) ) ;
#12370=CARTESIAN_POINT ( 'NONE',  ( 92.69370383062501162, -211.3315407142195852, 75.09072916753380866 ) ) ;
#12372=CARTESIAN_POINT ( 'NONE',  ( 95.00000000000000000, -212.6630814284392557, 80.43531250086715545 ) ) ;
#12374=ORIENTED_EDGE ( 'NONE', *, *, #43581, .T. ) ;
#12377=ORIENTED_EDGE ( 'NONE', *, *, #46328, .T. ) ;
#12379=CARTESIAN_POINT ( 'NONE',  ( 93.67500000000001137, -207.7050326799711968, 80.36916666666665776 ) ) ;
#12382=CARTESIAN_POINT ( 'NONE',  ( 95.00000000000000000, -213.0599564267049857, 85.79312500173431033 ) ) ;
#12383=CARTESIAN_POINT ( 'NONE',  ( 97.64999999999999147, 90.00000000000002842, 88.41249999999999432 ) ) ;
#12393=CARTESIAN_POINT ( 'NONE',  ( 97.64999999999999147, 90.00000000000002842, 84.68187500173429783 ) ) ;
#12395=ORIENTED_EDGE ( 'NONE', *, *, #2441, .F. ) ;
#12404=CARTESIAN_POINT ( 'NONE',  ( -96.32500000000001705, 87.70503267997129626, 86.93083333333332519 ) ) ;
#12409=VECTOR ( 'NONE', #58516, 1000.000000000000000 ) ;
#12413=CARTESIAN_POINT ( 'NONE',  ( -94.99999999999997158, -207.3369185715606307, 84.40406250086712703 ) ) ;
#12421=CARTESIAN_POINT ( 'NONE',  ( -97.30629616937497417, -208.6684592857803295, 74.98489583420048632 ) ) ;
#12422=CARTESIAN_POINT ( 'NONE',  ( 99.99999999999998579, 95.00000000000002842, 90.00000000000000000 ) ) ;
#12424=VECTOR ( 'NONE', #17892, 1000.000000000000000 ) ;
#12428=CARTESIAN_POINT ( 'NONE',  ( 96.73972734126404305, -208.4859488783623362, 74.79348190356850523 ) ) ;
#12429=CARTESIAN_POINT ( 'NONE',  ( -92.69370383062502583, 88.66845928578038638, 79.74739583420047495 ) ) ;
#12431=DIRECTION ( 'NONE',  ( -0.000000000000000000, -0.000000000000000000, -1.000000000000000000 ) ) ;
#12439=CARTESIAN_POINT ( 'NONE',  ( -92.35002849302227901, 91.52999466380659044, 87.27479280632984171 ) ) ;
#12440=CARTESIAN_POINT ( 'NONE',  ( -93.84685191531248449, -208.0026889286704943, 77.52489583420047836 ) ) ;
#12454=EDGE_CURVE ( 'NONE', #44954, #13102, #7081, .T. ) ;
#12458=CARTESIAN_POINT ( 'NONE',  ( 96.15314808468748708, -208.0026889286704943, 83.71614583420047495 ) ) ;
#12462=FACE_OUTER_BOUND ( 'NONE', #16123, .T. ) ;
#12469=CARTESIAN_POINT ( 'NONE',  ( -92.69370383062502583, 91.33154071421968467, 81.91697916753381037 ) ) ;
#12472=CARTESIAN_POINT ( 'NONE',  ( -100.0000000000000142, 95.00000000000002842, -90.00000000000000000 ) ) ;
#12477=CARTESIAN_POINT ( 'NONE',  ( 94.99999999999998579, 86.94004357329502852, 80.71312500173429783 ) ) ;
#12482=ORIENTED_EDGE ( 'NONE', *, *, #56436, .T. ) ;
#12486=CARTESIAN_POINT ( 'NONE',  ( 96.15314808468750130, -211.9973110713294489, 80.96447916753380980 ) ) ;
#12488=CARTESIAN_POINT ( 'NONE',  ( -93.67499999999998295, -207.7050326799711968, 76.45333333333333314 ) ) ;
#12489=CARTESIAN_POINT ( 'NONE',  ( -93.62329079302905654, -212.2908000246593474, 75.00000000000000000 ) ) ;
#12490=CARTESIAN_POINT ( 'NONE',  ( 97.64999999999999147, 90.00000000000002842, 85.23749999999999716 ) ) ;
#12494=CARTESIAN_POINT ( 'NONE',  ( -97.30629616937497417, -211.3315407142195852, 85.25072916753379104 ) ) ;
#12495=CARTESIAN_POINT ( 'NONE',  ( -92.69370383062502583, 88.66845928578038638, 83.08114583420048405 ) ) ;
#12500=CARTESIAN_POINT ( 'NONE',  ( 97.30629616937498838, 91.33154071421968467, 85.56822916753380071 ) ) ;
#12507=CARTESIAN_POINT ( 'NONE',  ( -97.30629616937497417, -208.6684592857803295, 87.68489583420047495 ) ) ;
#12508=CARTESIAN_POINT ( 'NONE',  ( -92.34999999999999432, -209.9999999999999716, 76.98250000000000171 ) ) ;
#12515=CARTESIAN_POINT ( 'NONE',  ( -92.35000000000005116, 88.47002178664754979, 78.83458333333334167 ) ) ;
#12516=CARTESIAN_POINT ( 'NONE',  ( -96.15314808468751551, 88.00268892867056536, 89.11364583420048291 ) ) ;
#12525=CARTESIAN_POINT ( 'NONE',  ( -92.35000000000003695, 90.00000000000004263, 90.00000000000000000 ) ) ;
#12532=CARTESIAN_POINT ( 'NONE',  ( -94.99999999999997158, -207.3369185715606307, 86.46781250086716852 ) ) ;
#12535=CARTESIAN_POINT ( 'NONE',  ( 96.15314808468748708, 88.00268892867053694, 77.31322916753381946 ) ) ;
#12538=CARTESIAN_POINT ( 'NONE',  ( -93.84685191531248449, -208.0026889286704943, 77.52489583420047836 ) ) ;
#12546=EDGE_CURVE ( 'NONE', #23968, #69024, #58481, .T. ) ;
#12547=CARTESIAN_POINT ( 'NONE',  ( -96.15314808468752972, 91.99731107132950569, 76.36072916753381890 ) ) ;
#12548=CARTESIAN_POINT ( 'NONE',  ( 97.30629616937498838, -209.9999999999999716, 76.62531250086713897 ) ) ;
#12552=ADVANCED_FACE ( 'NONE', ( #47211 ), #41559, .F. ) ;
#12553=( BOUNDED_CURVE ( )  B_SPLINE_CURVE ( 2, ( #13019, #19032, #20136, #65287, #37074, #24678, #60022 ),
 .UNSPECIFIED., .F., .F. ) 
 B_SPLINE_CURVE_WITH_KNOTS ( ( 3, 2, 2, 3 ),
 ( 0.8541666666666666297, 0.8611111111111110494, 0.8680555555555554692, 0.8749999999999997780 ),
 .UNSPECIFIED. ) 
 CURVE ( )  GEOMETRIC_REPRESENTATION_ITEM ( )  RATIONAL_B_SPLINE_CURVE ( ( 1.000000000000000000, 0.8660254037844387076, 1.000000000000000000, 0.8660254037844387076, 1.000000000000000000, 0.8660254037844430375, 0.9999999999999956701 ) ) 
 REPRESENTATION_ITEM ( '' )  );
#12561=EDGE_LOOP ( 'NONE', ( #668, #66677, #65895, #39863 ) ) ;
#12566=CARTESIAN_POINT ( 'NONE',  ( 94.99999999999998579, 87.33691857156068750, 82.34031250086714238 ) ) ;
#12571=CARTESIAN_POINT ( 'NONE',  ( 92.35000000000000853, -209.9999999999999716, 90.00000000000000000 ) ) ;
#12580=CARTESIAN_POINT ( 'NONE',  ( -94.99999999999997158, -206.9400435732949575, 85.39624999999998067 ) ) ;
#12586=CARTESIAN_POINT ( 'NONE',  ( -96.32499999999996021, -212.2949673200287179, 79.39020833506762642 ) ) ;
#12592=CARTESIAN_POINT ( 'NONE',  ( 94.99999999999998579, 86.94004357329500010, 79.44312500173428759 ) ) ;
#12593=CARTESIAN_POINT ( 'NONE',  ( -92.35000000000005116, 91.52997821335253548, 77.11479166840095445 ) ) ;
#12595=CARTESIAN_POINT ( 'NONE',  ( 97.30629616937498838, 88.66845928578037217, 81.17614583420048291 ) ) ;
#12602=CARTESIAN_POINT ( 'NONE',  ( -97.65000000000001990, 90.00000000000004263, 90.00000000000000000 ) ) ;
#12607=CARTESIAN_POINT ( 'NONE',  ( -92.34999999999999432, -209.9999999999999716, 75.71250000000000568 ) ) ;
#12608=CARTESIAN_POINT ( 'NONE',  ( -92.69370383062498320, -211.3315407142195852, 76.09614583420048461 ) ) ;
#12611=AXIS2_PLACEMENT_3D ( 'NONE', #13029, #34871, #40504 ) ;
#12614=CARTESIAN_POINT ( 'NONE',  ( -92.34999999999999432, -210.0000000334413528, 87.85687500050293863 ) ) ;
#12620=LINE ( 'NONE', #35557, #53844 ) ;
#12623=CARTESIAN_POINT ( 'NONE',  ( 92.69370383062498320, 90.00000000000002842, 86.62656250086715204 ) ) ;
#12624=CARTESIAN_POINT ( 'NONE',  ( -97.30629616937497417, -208.6684592857803295, 85.30364583420048064 ) ) ;
#12628=CARTESIAN_POINT ( 'NONE',  ( -97.64999999999994884, -211.5299782133524502, 80.52791666666665549 ) ) ;
#12630=CARTESIAN_POINT ( 'NONE',  ( -93.84685191531252713, 88.00268892867056536, 77.78947916753381264 ) ) ;
#12632=EDGE_CURVE ( 'NONE', #32195, #54291, #22912, .T. ) ;
#12636=CARTESIAN_POINT ( 'NONE',  ( 92.69370383062501162, -209.9999999999999716, 88.37281250086715545 ) ) ;
#12643=EDGE_LOOP ( 'NONE', ( #63711, #55104, #22653, #14971 ) ) ;
#12646=CARTESIAN_POINT ( 'NONE',  ( 93.84685191531251292, -211.9973110713294489, 80.38239583420048007 ) ) ;
#12649=CARTESIAN_POINT ( 'NONE',  ( -97.64999999999996305, -209.9999999999999716, 77.37937500173428873 ) ) ;
#12653=CARTESIAN_POINT ( 'NONE',  ( 95.00000000000000000, -213.0599564267049857, 85.07874999999999943 ) ) ;
#12654=ORIENTED_EDGE ( 'NONE', *, *, #35333, .T. ) ;
#12657=EDGE_LOOP ( 'NONE', ( #46159, #30625 ) ) ;
#12662=CARTESIAN_POINT ( 'NONE',  ( -92.69370383062502583, 88.66845928578038638, 88.79614583420050167 ) ) ;
#12665=CARTESIAN_POINT ( 'NONE',  ( 96.15314808468750130, -211.9973110713294489, 88.58447916753381435 ) ) ;
#12666=CARTESIAN_POINT ( 'NONE',  ( 97.64999999999997726, 91.52997821335252127, 78.94041666666666401 ) ) ;
#12668=CARTESIAN_POINT ( 'NONE',  ( -94.99999999999997158, -206.9400435732949575, 88.01562500173429271 ) ) ;
#12672=CARTESIAN_POINT ( 'NONE',  ( 92.35000000000000853, -209.9999999999999716, 90.00000000000000000 ) ) ;
#12673=CARTESIAN_POINT ( 'NONE',  ( 92.69370383062498320, 90.00000000000002842, 89.16656250086715829 ) ) ;
#12683=CARTESIAN_POINT ( 'NONE',  ( -97.30629616937495996, -209.9999999999999716, 75.03781250086713328 ) ) ;
#12693=CARTESIAN_POINT ( 'NONE',  ( -94.99999999999997158, -212.6630814284392557, 88.05531250086716000 ) ) ;
#12696=EDGE_LOOP ( 'NONE', ( #62991, #44392, #8015, #53052, #44895, #62052, #70984, #10560, #38729, #54278, #21718, #50480, #29243, #18567, #72931, #60583, #65559, #30141, #35211, #37740, #51792, #60706, #48557, #3967, #31054, #273, #17278, #54451, #36862, #37916, #64065, #53168, #16075, #32912, #59133, #702, #69815, #5382, #12757, #67321, #26084, #37060, #44263, #39512, #25598, #67976, #38200, #70563, #1666, #53916 ) ) ;
#12700=LINE ( 'NONE', #13070, #42163 ) ;
#12701=CARTESIAN_POINT ( 'NONE',  ( 97.30629616937498838, 91.33154071421968467, 79.85322916753379729 ) ) ;
#12713=CARTESIAN_POINT ( 'NONE',  ( -93.84685191531254134, 91.99731107132950569, 85.62114583420046188 ) ) ;
#12720=CARTESIAN_POINT ( 'NONE',  ( 95.00000000000000000, -206.9400435732949575, 83.49125000000000796 ) ) ;
#12725=CARTESIAN_POINT ( 'NONE',  ( 92.69370383062501162, -208.6684592857803011, 83.39864583420050792 ) ) ;
#12737=CARTESIAN_POINT ( 'NONE',  ( 93.84685191531251292, -211.9973110713294489, 75.14364583420046984 ) ) ;
#12739=CARTESIAN_POINT ( 'NONE',  ( 92.69370383062501162, -209.9999999999999716, 80.27656250086714351 ) ) ;
#12747=SURFACE_SIDE_STYLE ('',( #24054 ) ) ;
#12750=CARTESIAN_POINT ( 'NONE',  ( 92.34999999999999432, 90.00000000000002842, 90.00000000000000000 ) ) ;
#12751=CARTESIAN_POINT ( 'NONE',  ( 92.35000000000002274, -211.5299782133524502, 83.14729166840096752 ) ) ;
#12752=CARTESIAN_POINT ( 'NONE',  ( 97.30629616937498838, 90.00000000000002842, 74.87906250086714977 ) ) ;
#12754=CARTESIAN_POINT ( 'NONE',  ( 96.32499999999997442, 92.29496732002878900, 84.78770833506763438 ) ) ;
#12757=ORIENTED_EDGE ( 'NONE', *, *, #9226, .T. ) ;
#12760=CARTESIAN_POINT ( 'NONE',  ( 94.99999999999998579, 86.94004357329500010, 84.52312500173428589 ) ) ;
#12764=DIRECTION ( 'NONE',  ( -0.000000000000000000, -0.000000000000000000, 1.000000000000000000 ) ) ;
#12769=DIRECTION ( 'NONE',  ( 0.8571673007021122226, 0.000000000000000000, 0.5150380749100542666 ) ) ;
#12771=CARTESIAN_POINT ( 'NONE',  ( -93.67500000000003979, 92.29496732002878900, 88.51833333333333087 ) ) ;
#12773=LINE ( 'NONE', #31176, #68368 ) ;
#12776=( BOUNDED_CURVE ( )  B_SPLINE_CURVE ( 2, ( #6838, #29751, #25973, #59460, #42535, #18848, #71826 ),
 .UNSPECIFIED., .F., .F. ) 
 B_SPLINE_CURVE_WITH_KNOTS ( ( 3, 2, 2, 3 ),
 ( 0.6875000000000000000, 0.6944444444444443088, 0.7013888888888887285, 0.7083333333333331483 ),
 .UNSPECIFIED. ) 
 CURVE ( )  GEOMETRIC_REPRESENTATION_ITEM ( )  RATIONAL_B_SPLINE_CURVE ( ( 1.000000000000000000, 0.8660254037844387076, 1.000000000000000000, 0.8660254037844387076, 1.000000000000000000, 0.8660254037844430375, 0.9999999999999956701 ) ) 
 REPRESENTATION_ITEM ( '' )  );
#12778=CARTESIAN_POINT ( 'NONE',  ( -94.99999999999997158, -212.6630814284392557, 84.08656250086713158 ) ) ;
#12794=CARTESIAN_POINT ( 'NONE',  ( -92.69370383062502583, 88.66845928578038638, 77.84239583420045960 ) ) ;
#12806=CARTESIAN_POINT ( 'NONE',  ( -92.69370383062498320, -209.9999999999999716, 74.87906250086714977 ) ) ;
#12816=ORIENTED_EDGE ( 'NONE', *, *, #55538, .F. ) ;
#12822=CARTESIAN_POINT ( 'NONE',  ( 97.30629616937498838, -209.9999999999999716, 85.51531250086713953 ) ) ;
#12823=CARTESIAN_POINT ( 'NONE',  ( 95.00000000000000000, -212.6630814284392557, 87.42031250086715488 ) ) ;
#12827=CARTESIAN_POINT ( 'NONE',  ( 92.69370383062501162, -208.6684592857803011, 89.11364583420049712 ) ) ;
#12832=CARTESIAN_POINT ( 'NONE',  ( -97.30629616937501680, 88.66845928578038638, 82.23447916753383424 ) ) ;
#12837=DIRECTION ( 'NONE',  ( -1.000000000000000000, 0.000000000000000000, 0.000000000000000000 ) ) ;
#12844=CARTESIAN_POINT ( 'NONE',  ( 92.71977365048356035, 88.83725486022242990, 74.94226573542110259 ) ) ;
#12847=ORIENTED_EDGE ( 'NONE', *, *, #33775, .F. ) ;
#12848=CARTESIAN_POINT ( 'NONE',  ( 92.69370383062501162, -211.3315407142195852, 82.07572916753380809 ) ) ;
#12855=CARTESIAN_POINT ( 'NONE',  ( -96.32499999999996021, -207.7050326799711968, 88.70354166840097321 ) ) ;
#12856=CARTESIAN_POINT ( 'NONE',  ( 93.67500000000001137, -207.7050326799711968, 76.55916666666666970 ) ) ;
#12857=CARTESIAN_POINT ( 'NONE',  ( -94.99999999999997158, -212.6630814284392557, 83.45156250086714067 ) ) ;
#12859=CARTESIAN_POINT ( 'NONE',  ( -93.84685191531252713, 88.00268892867056536, 82.39322916753381776 ) ) ;
#12861=CARTESIAN_POINT ( 'NONE',  ( 94.99999999999998579, 87.33691857156068750, 80.27656250086714351 ) ) ;
#12865=LINE ( 'NONE', #45995, #55389 ) ;
#12867=LINE ( 'NONE', #60245, #53631 ) ;
#12868=CARTESIAN_POINT ( 'NONE',  ( -92.69370383062498320, -208.6684592857803295, 84.93322916753379559 ) ) ;
#12880=FACE_OUTER_BOUND ( 'NONE', #49994, .T. ) ;
#12887=CARTESIAN_POINT ( 'NONE',  ( -95.00000000000002842, 87.33691857156074434, 76.46656250086712703 ) ) ;
#12896=CARTESIAN_POINT ( 'NONE',  ( -92.69370383062498320, -208.6684592857803011, 86.99697916753382287 ) ) ;
#12901=CARTESIAN_POINT ( 'NONE',  ( 96.66135172262724495, 88.39919842643632819, 74.79754476654878204 ) ) ;
#12902=CARTESIAN_POINT ( 'NONE',  ( -93.84685191531248449, -208.0026889286704943, 74.98489583420048632 ) ) ;
#12909=CARTESIAN_POINT ( 'NONE',  ( 97.30629616937498838, -211.3315407142195852, 75.93739583420047268 ) ) ;
#12911=AXIS2_PLACEMENT_3D ( 'NONE', #4646, #22665, #9890 ) ;
#12915=ORIENTED_EDGE ( 'NONE', *, *, #52327, .F. ) ;
#12919=ORIENTED_EDGE ( 'NONE', *, *, #11893, .T. ) ;
#12922=CARTESIAN_POINT ( 'NONE',  ( -92.34999999999999432, -209.9999999999999716, 77.61749999999999261 ) ) ;
#12925=CARTESIAN_POINT ( 'NONE',  ( 97.30629616937498838, 88.66845928578037217, 79.27114583420048177 ) ) ;
#12926=CARTESIAN_POINT ( 'NONE',  ( 2.500000000000034639, 89.99999999999998579, -279.9999999999999432 ) ) ;
#12928=CARTESIAN_POINT ( 'NONE',  ( 97.65000000000000568, -211.0689551420226451, 75.04052853044679239 ) ) ;
#12936=CARTESIAN_POINT ( 'NONE',  ( -97.65000000000001990, 90.00000000000004263, 87.45999999999999375 ) ) ;
#12938=CARTESIAN_POINT ( 'NONE',  ( 92.34999999999999432, 90.00000000000002842, 90.00000000000000000 ) ) ;
#12944=CARTESIAN_POINT ( 'NONE',  ( -92.34999999999999432, -209.9999999999999716, 80.23687500173429044 ) ) ;
#12948=CARTESIAN_POINT ( 'NONE',  ( 94.99999999999998579, 86.94004357329500010, 76.26812500173430465 ) ) ;
#12949=CARTESIAN_POINT ( 'NONE',  ( -97.65000000000001990, 88.47002178664754979, 76.16229166840095388 ) ) ;
#12951=CARTESIAN_POINT ( 'NONE',  ( 94.99999999999998579, 87.33691857156068750, 81.70531250086715147 ) ) ;
#12952=CARTESIAN_POINT ( 'NONE',  ( 92.34999999999990905, 88.47002178664757821, 75.44791666666667140 ) ) ;
#12955=CARTESIAN_POINT ( 'NONE',  ( 92.35000000000000853, -209.9999999999999716, 79.28437500173430408 ) ) ;
#12961=EDGE_CURVE ( 'NONE', #25068, #49041, #30553, .T. ) ;
#12970=CARTESIAN_POINT ( 'NONE',  ( -94.99999999999997158, -207.3369185715606307, 78.84781250086714977 ) ) ;
#12976=DIRECTION ( 'NONE',  ( -0.000000000000000000, -0.000000000000000000, -1.000000000000000000 ) ) ;
#12977=CARTESIAN_POINT ( 'NONE',  ( -12.75000000000000000, -120.0000000000000000, 127.5000000000000000 ) ) ;
#12981=CARTESIAN_POINT ( 'NONE',  ( 92.35000000019410038, 89.99998015720535705, 86.27002759516707897 ) ) ;
#12982=DIRECTION ( 'NONE',  ( -0.8896955516311735312, 0.000000000000000000, 0.4565542962317865050 ) ) ;
#12985=( BOUNDED_CURVE ( )  B_SPLINE_CURVE ( 2, ( #45642, #34331, #69657, #22695, #39614, #11752, #28312 ),
 .UNSPECIFIED., .F., .F. ) 
 B_SPLINE_CURVE_WITH_KNOTS ( ( 3, 2, 2, 3 ),
 ( 0.1666666666666666852, 0.1736111111111111049, 0.1805555555555554970, 0.1874999999999999167 ),
 .UNSPECIFIED. ) 
 CURVE ( )  GEOMETRIC_REPRESENTATION_ITEM ( )  RATIONAL_B_SPLINE_CURVE ( ( 0.9999999999999994449, 0.8660254037844392627, 1.000000000000000000, 0.8660254037844387076, 1.000000000000000000, 0.8660254037844402619, 0.9999999999999984457 ) ) 
 REPRESENTATION_ITEM ( '' )  );
#12988=CARTESIAN_POINT ( 'NONE',  ( 94.99999999999998579, 92.66308142843932671, 82.65781250086715204 ) ) ;
#12991=CARTESIAN_POINT ( 'NONE',  ( -96.15314808468747287, -208.0026889286704943, 87.15572916753382060 ) ) ;
#12992=CARTESIAN_POINT ( 'NONE',  ( 93.67499999999998295, 92.29496732002878900, 79.17854166840096752 ) ) ;
#12995=CARTESIAN_POINT ( 'NONE',  ( -93.67499999999998295, -212.2949673200287179, 81.95666666666666345 ) ) ;
#12996=CARTESIAN_POINT ( 'NONE',  ( -97.30629616937501680, 90.00000000000004263, 75.03781250086713328 ) ) ;
#13000=CARTESIAN_POINT ( 'NONE',  ( 93.84685191531251292, -211.9973110713294489, 88.47864583420047779 ) ) ;
#13004=ORIENTED_EDGE ( 'NONE', *, *, #23092, .T. ) ;
#13014=CARTESIAN_POINT ( 'NONE',  ( 92.69370383062501162, -208.6684592857803295, 81.49364583420049257 ) ) ;
#13015=CARTESIAN_POINT ( 'NONE',  ( 93.67499999999998295, 92.29496732002878900, 89.89416666666666345 ) ) ;
#13016=CARTESIAN_POINT ( 'NONE',  ( 94.99999999999998579, 93.05995642670504253, 80.95125000000000171 ) ) ;
#13019=CARTESIAN_POINT ( 'NONE',  ( 97.64999999999999147, 90.00000000000002842, 76.98250000000000171 ) ) ;
#13021=CARTESIAN_POINT ( 'NONE',  ( 93.67500000000001137, -212.2949673200287179, 83.75583333333332803 ) ) ;
#13023=ORIENTED_EDGE ( 'NONE', *, *, #27984, .T. ) ;
#13027=CARTESIAN_POINT ( 'NONE',  ( -92.69370383062502583, 88.66845928578038638, 86.89114583420050053 ) ) ;
#13029=CARTESIAN_POINT ( 'NONE',  ( -94.99999999999997158, -209.9999999999999716, 90.00000000000000000 ) ) ;
#13030=CARTESIAN_POINT ( 'NONE',  ( 93.84685191531251292, -211.9973110713294489, 88.47864583420047779 ) ) ;
#13031=CARTESIAN_POINT ( 'NONE',  ( 97.64999999999999147, 90.00000000000002842, 79.52249999999999375 ) ) ;
#13033=CARTESIAN_POINT ( 'NONE',  ( -93.67499999999998295, -207.7050326799711968, 87.96270833506763154 ) ) ;
#13035=CARTESIAN_POINT ( 'NONE',  ( 92.34999999999999432, -211.5299782133524502, 79.89291666666666458 ) ) ;
#13037=CARTESIAN_POINT ( 'NONE',  ( -92.35000000000005116, 88.47002178664754979, 85.89895833506764689 ) ) ;
#13039=CARTESIAN_POINT ( 'NONE',  ( 92.69370383062498320, 88.66845928578037217, 75.09072916753382287 ) ) ;
#13040=ORIENTED_EDGE ( 'NONE', *, *, #16728, .T. ) ;
#13041=DIRECTION ( 'NONE',  ( 0.4565542962317865050, 0.000000000000000000, 0.8896955516311735312 ) ) ;
#13054=EDGE_LOOP ( 'NONE', ( #54407, #11362, #62530, #44600 ) ) ;
#13061=CARTESIAN_POINT ( 'NONE',  ( -97.30629616937495996, -209.9999999999999716, 87.26156250086715715 ) ) ;
#13064=ORIENTED_EDGE ( 'NONE', *, *, #20208, .F. ) ;
#13069=CARTESIAN_POINT ( 'NONE',  ( 97.64999999999992042, 91.52997821335257811, 86.56041666666668277 ) ) ;
#13070=CARTESIAN_POINT ( 'NONE',  ( 90.00000000000001421, -204.9999999999999147, 90.00000000000000000 ) ) ;
#13071=CARTESIAN_POINT ( 'NONE',  ( 97.30629616937498838, 91.33154071421968467, 81.12322916753380753 ) ) ;
#13074=CARTESIAN_POINT ( 'NONE',  ( -92.34999999999995168, 91.52997821335249284, 80.84541666666663673 ) ) ;
#13079=CARTESIAN_POINT ( 'NONE',  ( -97.64999999960629395, 90.00002930740643592, 76.74344264317980446 ) ) ;
#13084=CARTESIAN_POINT ( 'NONE',  ( -96.15314808468751551, 88.00268892867056536, 86.57364583420047666 ) ) ;
#13090=VERTEX_POINT ( 'NONE', #48598 ) ;
#13093=CARTESIAN_POINT ( 'NONE',  ( 96.32499999999998863, -207.7050326799711968, 75.89770833506763381 ) ) ;
#13099=CARTESIAN_POINT ( 'NONE',  ( 97.30629616937498838, -208.6684592857803011, 82.55197916753382970 ) ) ;
#13102=VERTEX_POINT ( 'NONE', #15113 ) ;
#13104=CARTESIAN_POINT ( 'NONE',  ( -0.0004442498525516064278, 0.001194404164626844313, 127.4927882439603195 ) ) ;
#13107=CARTESIAN_POINT ( 'NONE',  ( 92.69370383062501162, -209.9999999999999716, 76.30781250086714351 ) ) ;
#13108=ORIENTED_EDGE ( 'NONE', *, *, #30225, .T. ) ;
#13109=CARTESIAN_POINT ( 'NONE',  ( 96.15314808468750130, -211.9973110713294489, 79.85322916753381151 ) ) ;
#13110=AXIS2_PLACEMENT_3D ( 'NONE', #36086, #25179, #8250 ) ;
#13111=EDGE_LOOP ( 'NONE', ( #11451, #31224, #37533, #44924 ) ) ;
#13120=CARTESIAN_POINT ( 'NONE',  ( -97.64999999999996305, -209.9999999999999716, 90.00000000000000000 ) ) ;
#13121=CARTESIAN_POINT ( 'NONE',  ( 93.67500000000001137, -212.2949673200287179, 81.93020833506763267 ) ) ;
#13122=CARTESIAN_POINT ( 'NONE',  ( 97.64999999999997726, 88.47002178664753558, 88.99458333333333826 ) ) ;
#13126=CARTESIAN_POINT ( 'NONE',  ( 97.64999999999999147, -209.9999999999999716, 90.00000000000000000 ) ) ;
#13129=CARTESIAN_POINT ( 'NONE',  ( -93.84685191531254134, 91.99731107132950569, 87.04989583420048405 ) ) ;
#13131=CARTESIAN_POINT ( 'NONE',  ( 97.64999999999999147, 90.00000000000002842, 85.31687500173428873 ) ) ;
#13142=CARTESIAN_POINT ( 'NONE',  ( 93.67499999999998295, 92.29496732002878900, 81.63916666666666799 ) ) ;
#13144=CARTESIAN_POINT ( 'NONE',  ( -92.35000000000005116, 91.52997821335253548, 85.29041666666665833 ) ) ;
#13150=CARTESIAN_POINT ( 'NONE',  ( -94.99999999999997158, -212.6630814284392557, 81.54656250086715374 ) ) ;
#13151=EDGE_CURVE ( 'NONE', #55839, #59860, #14752, .T. ) ;
#13152=EDGE_LOOP ( 'NONE', ( #54825, #10834, #34222, #55206 ) ) ;
#13165=DIRECTION ( 'NONE',  ( -0.000000000000000000, -0.000000000000000000, 1.000000000000000000 ) ) ;
#13170=CARTESIAN_POINT ( 'NONE',  ( -93.84685191531254134, 91.99731107132950569, 75.46114583420047950 ) ) ;
#13184=CARTESIAN_POINT ( 'NONE',  ( -92.69370383062498320, -211.3315407142195852, 77.36614583420048064 ) ) ;
#13190=CARTESIAN_POINT ( 'NONE',  ( -97.64999999978466860, 90.00002100773832581, 79.91868729552945183 ) ) ;
#13197=VERTEX_POINT ( 'NONE', #6469 ) ;
#13198=( BOUNDED_CURVE ( )  B_SPLINE_CURVE ( 2, ( #6230, #38943, #16376, #5119, #56984, #33664, #39319 ),
 .UNSPECIFIED., .F., .F. ) 
 B_SPLINE_CURVE_WITH_KNOTS ( ( 3, 2, 2, 3 ),
 ( 0.3598440426530882807, 0.3668998081258831867, 0.3739555736667655728, 0.3810111478265181262 ),
 .UNSPECIFIED. ) 
 CURVE ( )  GEOMETRIC_REPRESENTATION_ITEM ( )  RATIONAL_B_SPLINE_CURVE ( ( 1.000000000000000000, 0.8660254037844387076, 1.000000000000000000, 0.8660254037844387076, 1.000000000000000000, 0.8660290377217400026, 0.9999927323225317188 ) ) 
 REPRESENTATION_ITEM ( '' )  );
#13200=CARTESIAN_POINT ( 'NONE',  ( 95.00000000000000000, -207.3369185715606307, 86.30906250086714238 ) ) ;
#13201=CARTESIAN_POINT ( 'NONE',  ( 97.30629616937498838, -211.3315407142195852, 89.43114583420049257 ) ) ;
#13207=CARTESIAN_POINT ( 'NONE',  ( -97.30629616937501680, 90.00000000000004263, 81.54656250086715374 ) ) ;
#13209=ORIENTED_EDGE ( 'NONE', *, *, #31672, .F. ) ;
#13211=FACE_OUTER_BOUND ( 'NONE', #69917, .T. ) ;
#13220=( BOUNDED_CURVE ( )  B_SPLINE_CURVE ( 2, ( #1730, #24617, #57356, #23512, #621, #46445, #69372 ),
 .UNSPECIFIED., .F., .F. ) 
 B_SPLINE_CURVE_WITH_KNOTS ( ( 3, 2, 2, 3 ),
 ( 0.5000000000000000000, 0.5069444444444444198, 0.5138888888888887285, 0.5208333333333332593 ),
 .UNSPECIFIED. ) 
 CURVE ( )  GEOMETRIC_REPRESENTATION_ITEM ( )  RATIONAL_B_SPLINE_CURVE ( ( 1.000000000000000000, 0.8660254037844387076, 1.000000000000000000, 0.8660254037844387076, 1.000000000000000000, 0.8660254037844408170, 0.9999999999999978906 ) ) 
 REPRESENTATION_ITEM ( '' )  );
#13221=CARTESIAN_POINT ( 'NONE',  ( 92.35000000000000853, -211.5299782133524218, 80.60729166840097548 ) ) ;
#13225=ORIENTED_EDGE ( 'NONE', *, *, #67849, .F. ) ;
#13226=ORIENTED_EDGE ( 'NONE', *, *, #21116, .F. ) ;
#13228=CARTESIAN_POINT ( 'NONE',  ( 97.30629616937498838, -209.9999999999999716, 79.16531250086714522 ) ) ;
#13234=CARTESIAN_POINT ( 'NONE',  ( 97.64999999999994884, 88.47002178664752137, 85.18458333333332178 ) ) ;
#13240=CARTESIAN_POINT ( 'NONE',  ( -92.69370383062498320, -211.3315407142195852, 82.92239583420045790 ) ) ;
#13241=CARTESIAN_POINT ( 'NONE',  ( -93.84685191531254134, 91.99731107132950569, 83.23989583420049598 ) ) ;
#13243=CARTESIAN_POINT ( 'NONE',  ( 93.84685191531248449, 88.00268892867053694, 80.22364583420046813 ) ) ;
#13246=DIRECTION ( 'NONE',  ( -0.000000000000000000, -0.000000000000000000, 1.000000000000000000 ) ) ;
#13251=CARTESIAN_POINT ( 'NONE',  ( -96.15314808468747287, -208.0026889286704943, 83.82197916753381151 ) ) ;
#13260=CARTESIAN_POINT ( 'NONE',  ( -97.64999999999986358, -211.5299782133524502, 78.62291666666668277 ) ) ;
#13262=CARTESIAN_POINT ( 'NONE',  ( -96.15314808468751551, 88.00268892867056536, 87.84364583420047268 ) ) ;
#13268=CARTESIAN_POINT ( 'NONE',  ( -92.69370383062504004, 90.00000000000004263, 76.62531250086713897 ) ) ;
#13273=CARTESIAN_POINT ( 'NONE',  ( 97.64999999999999147, -210.0000000983658026, 80.23687499810812085 ) ) ;
#13275=CARTESIAN_POINT ( 'NONE',  ( 92.35000000000000853, -209.9999999999999716, 82.37999999999999545 ) ) ;
#13276=CARTESIAN_POINT ( 'NONE',  ( -92.69370383062498320, -209.9999999999999716, 86.94406250086716170 ) ) ;
#13278=CARTESIAN_POINT ( 'NONE',  ( 96.66078148566039374, 88.39974787049349914, 74.80065602173002048 ) ) ;
#13279=CARTESIAN_POINT ( 'NONE',  ( -96.15314808468745866, -211.9973110713294489, 76.57239583420049200 ) ) ;
#13280=CARTESIAN_POINT ( 'NONE',  ( 92.34999999999999432, 90.00000000000002842, 88.73000000000000398 ) ) ;
#13282=CARTESIAN_POINT ( 'NONE',  ( -92.35000000000005116, 91.52997821335253548, 82.82979166840095786 ) ) ;
#13289=CARTESIAN_POINT ( 'NONE',  ( 97.30629616937498838, -209.9999999999999716, 75.99031250086714806 ) ) ;
#13291=EDGE_CURVE ( 'NONE', #21733, #32740, #30114, .T. ) ;
#13302=DIRECTION ( 'NONE',  ( -0.000000000000000000, -0.000000000000000000, -1.000000000000000000 ) ) ;
#13306=CARTESIAN_POINT ( 'NONE',  ( 92.69370383062498320, 88.66845928578037217, 80.32947916753381890 ) ) ;
#13312=EDGE_CURVE ( 'NONE', #14612, #53174, #37822, .T. ) ;
#13316=CARTESIAN_POINT ( 'NONE',  ( 94.99999999999998579, 90.00000000000002842, 90.00000000000000000 ) ) ;
#13321=CARTESIAN_POINT ( 'NONE',  ( -97.30599797242227567, 90.94645204372872627, 74.89836836546780319 ) ) ;
#13323=CARTESIAN_POINT ( 'NONE',  ( -93.67499999999998295, -207.7050326799711968, 84.15270833506762926 ) ) ;
#13326=CARTESIAN_POINT ( 'NONE',  ( -96.32499999999996021, -207.7050326799711968, 78.54354166840096241 ) ) ;
#13328=CARTESIAN_POINT ( 'NONE',  ( 97.64999999999997726, 91.52997821335252127, 74.57479166840096241 ) ) ;
#13329=CARTESIAN_POINT ( 'NONE',  ( -96.32500000000001705, 92.29496732002878900, 76.63854166840096127 ) ) ;
#13331=CARTESIAN_POINT ( 'NONE',  ( 97.30629616937498838, 91.33154071421968467, 78.10697916753383652 ) ) ;
#13338=VERTEX_POINT ( 'NONE', #9967 ) ;
#13346=( BOUNDED_CURVE ( )  B_SPLINE_CURVE ( 2, ( #5379, #68523, #73394, #28274, #44480, #73768, #73014 ),
 .UNSPECIFIED., .F., .F. ) 
 B_SPLINE_CURVE_WITH_KNOTS ( ( 3, 2, 2, 3 ),
 ( 0.5208333333333332593, 0.5277777777777776791, 0.5347222222222220989, 0.5416666666666665186 ),
 .UNSPECIFIED. ) 
 CURVE ( )  GEOMETRIC_REPRESENTATION_ITEM ( )  RATIONAL_B_SPLINE_CURVE ( ( 1.000000000000002220, 0.8660254037844365982, 1.000000000000000000, 0.8660254037844387076, 1.000000000000000000, 0.8660254037844408170, 0.9999999999999978906 ) ) 
 REPRESENTATION_ITEM ( '' )  );
#13349=CARTESIAN_POINT ( 'NONE',  ( -97.65000000000001990, 90.00000000000004263, 86.26937500173430351 ) ) ;
#13350=DIRECTION ( 'NONE',  ( -2.628368902995175337E-16, -1.000000000000000000, 0.000000000000000000 ) ) ;
#13352=CARTESIAN_POINT ( 'NONE',  ( -96.15314808468747287, -208.0026889286704943, 78.26572916753382003 ) ) ;
#13354=ORIENTED_EDGE ( 'NONE', *, *, #23420, .F. ) ;
#13355=LINE ( 'NONE', #19728, #54768 ) ;
#13357=CARTESIAN_POINT ( 'NONE',  ( 93.67499999999999716, 87.70503267997126784, 85.74020833506763495 ) ) ;
#13359=FACE_OUTER_BOUND ( 'NONE', #42431, .T. ) ;
#13361=FACE_OUTER_BOUND ( 'NONE', #21997, .T. ) ;
#13365=CARTESIAN_POINT ( 'NONE',  ( 93.84685191531248449, 88.00268892867053694, 82.28739583420048120 ) ) ;
#13366=CARTESIAN_POINT ( 'NONE',  ( -93.84685191531248449, -208.0026889286704943, 85.14489583420048291 ) ) ;
#13368=EDGE_LOOP ( 'NONE', ( #31491, #57818, #19504, #3732 ) ) ;
#13372=CARTESIAN_POINT ( 'NONE',  ( -94.99999999999997158, -213.0599564267049857, 79.99874999999998693 ) ) ;
#13373=CARTESIAN_POINT ( 'NONE',  ( -92.69370383062505425, 88.66845928578038638, 77.84239583420047381 ) ) ;
#13376=CARTESIAN_POINT ( 'NONE',  ( 96.15314808468750130, -211.9973110713294489, 86.67947916753381321 ) ) ;
#13378=AXIS2_PLACEMENT_3D ( 'NONE', #16015, #22790, #38960 ) ;
#13388=EDGE_CURVE ( 'NONE', #13338, #24878, #44572, .T. ) ;
#13389=VERTEX_POINT ( 'NONE', #56215 ) ;
#13391=CARTESIAN_POINT ( 'NONE',  ( 96.15314808468750130, -211.9973110713294489, 81.75822916753382685 ) ) ;
#13398=CARTESIAN_POINT ( 'NONE',  ( 95.00000000000000000, -213.0599564267049857, 83.80875000000000341 ) ) ;
#13399=ORIENTED_EDGE ( 'NONE', *, *, #25028, .T. ) ;
#13402=ORIENTED_EDGE ( 'NONE', *, *, #54399, .F. ) ;
#13404=CARTESIAN_POINT ( 'NONE',  ( 96.32499999999998863, -212.2949673200287179, 87.03666666666666174 ) ) ;
#13405=CARTESIAN_POINT ( 'NONE',  ( -93.84685191531252713, 88.00268892867056536, 83.02822916753380866 ) ) ;
#13408=CARTESIAN_POINT ( 'NONE',  ( 93.84685191531251292, -211.9973110713294489, 89.11364583420048291 ) ) ;
#13416=CARTESIAN_POINT ( 'NONE',  ( -96.32500000000001705, 92.29496732002878900, 85.52854166840096184 ) ) ;
#13417=CARTESIAN_POINT ( 'NONE',  ( 92.69370383062498320, 88.66845928578037217, 86.67947916753382742 ) ) ;
#13422=CARTESIAN_POINT ( 'NONE',  ( -93.67499999999998295, -207.7050326799711968, 78.43770833506764006 ) ) ;
#13426=ORIENTED_EDGE ( 'NONE', *, *, #8249, .F. ) ;
#13432=ORIENTED_EDGE ( 'NONE', *, *, #73653, .F. ) ;
#13433=CARTESIAN_POINT ( 'NONE',  ( -92.69370383062498320, -210.0000000000000568, 74.79348190356851944 ) ) ;
#13434=VECTOR ( 'NONE', #7699, 1000.000000000000000 ) ;
#13435=EDGE_CURVE ( 'NONE', #53644, #69813, #30561, .T. ) ;
#13439=( BOUNDED_CURVE ( )  B_SPLINE_CURVE ( 2, ( #55556, #44664, #49902, #40124, #5560, #5188, #28090 ),
 .UNSPECIFIED., .F., .F. ) 
 B_SPLINE_CURVE_WITH_KNOTS ( ( 3, 2, 2, 3 ),
 ( 0.5080151867278726030, 0.5150708844869413827, 0.5221266500278589628, 0.5291824299534890752 ),
 .UNSPECIFIED. ) 
 CURVE ( )  GEOMETRIC_REPRESENTATION_ITEM ( )  RATIONAL_B_SPLINE_CURVE ( ( 0.9999974259466133386, 0.8660266908234961480, 1.000000000000000000, 0.8660254037844387076, 1.000000000000000000, 0.8660254037844387076, 1.000000000000000000 ) ) 
 REPRESENTATION_ITEM ( '' )  );
#13440=CARTESIAN_POINT ( 'NONE',  ( -92.69370383062498320, -209.9999999999999716, 86.30906250086715659 ) ) ;
#13443=ORIENTED_EDGE ( 'NONE', *, *, #37797, .F. ) ;
#13444=LINE ( 'NONE', #25833, #19821 ) ;
#13446=CARTESIAN_POINT ( 'NONE',  ( 92.69370383062498320, 90.00000000000002842, 89.16656250086715829 ) ) ;
#13448=CARTESIAN_POINT ( 'NONE',  ( 96.15314808468748708, 88.00268892867053694, 82.86947916753379673 ) ) ;
#13460=CARTESIAN_POINT ( 'NONE',  ( -92.69370383062505425, 88.66845928578038638, 84.82739583420048746 ) ) ;
#13472=CARTESIAN_POINT ( 'NONE',  ( 97.30629616937498838, -211.3315407142195852, 81.81114583420048803 ) ) ;
#13477=EDGE_CURVE ( 'NONE', #7050, #74311, #56494, .T. ) ;
#13486=CARTESIAN_POINT ( 'NONE',  ( 97.30629616937498838, -208.6684592857803011, 80.64697916753382856 ) ) ;
#13492=ORIENTED_EDGE ( 'NONE', *, *, #3407, .T. ) ;
#13495=CARTESIAN_POINT ( 'NONE',  ( 97.64999999999999147, -209.9999999999999716, 80.15749999999999886 ) ) ;
#13498=CARTESIAN_POINT ( 'NONE',  ( 97.64999999999999147, -209.9999999999999716, 84.04687500173430692 ) ) ;
#13499=CARTESIAN_POINT ( 'NONE',  ( 92.34999999999999432, 91.52997821335252127, 89.31208333333333371 ) ) ;
#13505=CARTESIAN_POINT ( 'NONE',  ( -95.00000000000002842, 87.33691857156074434, 88.69031250086716511 ) ) ;
#13506=CARTESIAN_POINT ( 'NONE',  ( 93.84685191531248449, 88.00268892867053694, 84.66864583420047552 ) ) ;
#13509=CARTESIAN_POINT ( 'NONE',  ( 92.34999999999999432, 90.00000000000002842, 86.90437500173429441 ) ) ;
#13512=EDGE_CURVE ( 'NONE', #61999, #58994, #64177, .T. ) ;
#13517=DIRECTION ( 'NONE',  ( -0.000000000000000000, -0.000000000000000000, 1.000000000000000000 ) ) ;
#13519=CARTESIAN_POINT ( 'NONE',  ( -97.65000000000001990, 88.47002178664754979, 85.60791666666665378 ) ) ;
#13520=VERTEX_POINT ( 'NONE', #1701 ) ;
#13522=CARTESIAN_POINT ( 'NONE',  ( 97.25633982090072038, 90.55049048501746256, 74.79348190356850523 ) ) ;
#13525=DIRECTION ( 'NONE',  ( 1.000000000000000000, 0.000000000000000000, 0.000000000000000000 ) ) ;
#13526=CARTESIAN_POINT ( 'NONE',  ( -92.69370383062498320, -208.6684592857803011, 83.66322916753379957 ) ) ;
#13539=CARTESIAN_POINT ( 'NONE',  ( -97.30629616937501680, 88.66845928578038638, 75.09072916753382287 ) ) ;
#13544=LINE ( 'NONE', #59418, #46133 ) ;
#13550=CARTESIAN_POINT ( 'NONE',  ( -94.99999999999997158, -206.9400435732949575, 88.57124999999999204 ) ) ;
#13553=CARTESIAN_POINT ( 'NONE',  ( 92.35000000005783249, 89.99998877583867340, 75.47473230081648410 ) ) ;
#13554=CARTESIAN_POINT ( 'NONE',  ( 97.64999999999999147, -209.9999999999999716, 88.41249999999999432 ) ) ;
#13557=EDGE_CURVE ( 'NONE', #11086, #54488, #43000, .T. ) ;
#13564=CARTESIAN_POINT ( 'NONE',  ( 93.84685191531249870, -208.0026889286704943, 84.45697916753380241 ) ) ;
#13565=CARTESIAN_POINT ( 'NONE',  ( 96.15314808468750130, -211.9973110713294489, 89.37822916753381719 ) ) ;
#13569=ORIENTED_EDGE ( 'NONE', *, *, #15432, .T. ) ;
#13570=CARTESIAN_POINT ( 'NONE',  ( -96.32499999999996021, -212.2949673200287179, 80.58083333333331666 ) ) ;
#13572=CARTESIAN_POINT ( 'NONE',  ( -95.00000000000002842, 92.66308142843932671, 82.02281250086714692 ) ) ;
#13578=CARTESIAN_POINT ( 'NONE',  ( -100.0000000000000142, 85.00000000000002842, -79.99999999999998579 ) ) ;
#13586=CARTESIAN_POINT ( 'NONE',  ( 92.35000000000000853, -211.5299782133524218, 81.24229166840096639 ) ) ;
#13592=ORIENTED_EDGE ( 'NONE', *, *, #35560, .T. ) ;
#13593=CARTESIAN_POINT ( 'NONE',  ( 93.84685191531249870, -208.0026889286704943, 77.47197916753380298 ) ) ;
#13595=CARTESIAN_POINT ( 'NONE',  ( -92.35000000000003695, 90.00000000000004263, 83.33250000000001023 ) ) ;
#13596=ADVANCED_FACE ( 'NONE', ( #59549 ), #72294, .F. ) ;
#13597=ADVANCED_FACE ( 'NONE', ( #2071 ), #20434, .F. ) ;
#13601=CARTESIAN_POINT ( 'NONE',  ( 92.35000000000000853, -209.9999999999999716, 75.00000000000000000 ) ) ;
#13606=CARTESIAN_POINT ( 'NONE',  ( -97.30629616937497417, -211.3315407142195852, 81.44072916753381719 ) ) ;
#13607=CARTESIAN_POINT ( 'NONE',  ( -97.30629616937501680, 90.00000000000004263, 80.27656250086714351 ) ) ;
#13609=CARTESIAN_POINT ( 'NONE',  ( 96.15314808468748708, 88.00268892867053694, 80.32947916753380468 ) ) ;
#13613=CARTESIAN_POINT ( 'NONE',  ( 93.67499999999999716, 87.70503267997126784, 77.48520833506763950 ) ) ;
#13616=CARTESIAN_POINT ( 'NONE',  ( -93.84685191531247028, -211.9973110713294489, 82.86947916753379673 ) ) ;
#13617=CARTESIAN_POINT ( 'NONE',  ( -97.64999999999990621, -211.5299782133524786, 89.41791666666667027 ) ) ;
#13624=CARTESIAN_POINT ( 'NONE',  ( -97.30629616937501680, 90.00000000000004263, 84.56281250086713897 ) ) ;
#13630=B_SPLINE_CURVE_WITH_KNOTS ( 'NONE', 1,
 ( #59159, #47142 ),
 .UNSPECIFIED., .F., .F.,
 ( 2, 2 ),
 ( 0.000000000000000000, 1.000000000000000000 ),
 .UNSPECIFIED. ) ;
#13632=CARTESIAN_POINT ( 'NONE',  ( -97.30629616937501680, 91.33154071421968467, 76.25489583420049655 ) ) ;
#13637=CARTESIAN_POINT ( 'NONE',  ( -97.30629616937497417, -208.6684592857803011, 87.84364583420048689 ) ) ;
#13640=( BOUNDED_CURVE ( )  B_SPLINE_CURVE ( 2, ( #46570, #51467, #11983, #22163, #45853, #23, #22917, #6718, #28164, #68775, #69499, #40941, #12348, #46210, #17263, #35290, #58217, #50720, #68408, #73646, #63145, #45102, #11601, #16515, #57488, #62405, #6005, #51840, #10885, #1122, #7824, #2602, #1492, #25118, #18722, #48050, #41659, #30740, #42411, #25483, #36384, #19468, #70964, #36759, #53320, #14194, #1859, #42781, #30003, #52951, #53684, #24018, #2224, #48415, #24378, #65351, #64600, #13818, #13084, #59707, #8185, #24743, #19830, #31114, #54066, #71326, #70582, #65716, #37147, #7458, #46946, #30373, #47673, #42048, #60090, #29626, #12713, #52571, #69860, #36023, #18358, #41302, #58968, #19100, #64242, #35643, #58582, #7085, #47318, #70217, #64985, #13460, #59334, #4057, #26954, #66820, #55543, #38627, #67191, #44264, #49884, #54426, #9297, #8570, #44647, #67566, #43541, #49520, #27321, #73192, #55910, #71703, #20202, #15690, #72803, #20589, #15308, #32597, #61186, #32961, #61560, #14567, #66456, #10042, #31855, #3690, #60453, #66096, #2961, #43171, #72445, #21304, #4423, #60816, #50255, #14943, #54794, #21691, #16058, #25849, #38998, #20947, #37886, #48779, #9676, #31487, #26214, #37517, #32214, #8935, #3322, #26589, #55167, #43902, #49154, #72080, #38243, #11887, #28821, #298, #11521, #57772, #69407, #661, #56672, #62694, #51375, #5912, #17538, #33328, #68315, #33720, #27710, #23192, #40108, #16808, #39747, #63419, #34838, #6276, #29174, #73936, #56289, #17909, #10413, #22447, #4808, #61933, #52118, #34455, #5172, #28072, #74313, #46119, #50632, #11165, #73559, #23553, #46482, #45391, #28442, #69054, #22073, #57396, #10795, #34088, #45015, #40469, #67942, #16431, #39369, #22826, #62307, #51015, #57034, #5545, #45766, #68689, #17174, #63062, #51753, #64897, #6993, #13373, #12630, #36304, #42332, #35567, #59247, #48332, #24659, #53236, #69778, #6631, #30292, #1408, #35198, #41960, #7739, #58497, #47966, #31027, #29917, #52869, #58882, #19008, #29543, #2524, #53981, #46866, #19382, #25406, #1772, #30654, #64154, #63792, #18279, #70137, #71241, #41578, #47590, #70882, #70495, #65265, #53600, #18637, #2139, #40856, #24300, #25024, #13738, #12265, #47227, #36675, #64518, #59621, #12996, #58132, #8104, #35934, #52482, #41216, #1033 ),
 .UNSPECIFIED., .F., .F. ) 
 B_SPLINE_CURVE_WITH_KNOTS ( ( 3, 2, 2, 2, 2, 2, 2, 2, 2, 2, 2, 2, 2, 2, 2, 2, 2, 2, 2, 2, 2, 2, 2, 2, 2, 2, 2, 2, 2, 2, 2, 2, 2, 2, 2, 2, 2, 2, 2, 2, 2, 2, 2, 2, 2, 2, 2, 2, 2, 2, 2, 2, 2, 2, 2, 2, 2, 2, 2, 2, 2, 2, 2, 2, 2, 2, 2, 2, 2, 2, 2, 2, 2, 2, 2, 2, 2, 2, 2, 2, 2, 2, 2, 2, 2, 2, 2, 2, 2, 2, 2, 2, 2, 2, 2, 2, 2, 2, 2, 2, 2, 2, 2, 2, 2, 2, 2, 2, 2, 2, 2, 2, 2, 2, 2, 2, 2, 2, 2, 2, 2, 2, 2, 2, 2, 2, 2, 2, 2, 2, 2, 2, 2, 2, 2, 2, 2, 2, 2, 2, 2, 3 ),
 ( 0.000000000000000000, 0.007055765384978174640, 0.01411153076995634928, 0.02116729615493452218, 0.02822306153991269856, 0.03527882692489087840, 0.04233459230986904437, 0.04939035769484722421, 0.05644612307982539712, 0.06350188846480357696, 0.07055765384978175681, 0.07761341923475993665, 0.08466918461973808874, 0.09172495000471626858, 0.09878071538969444843, 0.1058364807746726144, 0.1128922461596507942, 0.1199480115446289741, 0.1270037769296071539, 0.1340595423145853338, 0.1411153076995635136, 0.1481710730845416935, 0.1552268384695198733, 0.1622826038544979976, 0.1693383692394761775, 0.1763941346244543573, 0.1834499000094325372, 0.1905056653944107170, 0.1975614307793888969, 0.2046171961643670489, 0.2116729615493452288, 0.2187287269343234364, 0.2257844923193015885, 0.2328402577042797683, 0.2398960230892579482, 0.2469517884742361002, 0.2540075538592143078, 0.2610633192441924599, 0.2681190846291706675, 0.2751748500141487641, 0.2822306153991270272, 0.2892863807841051238, 0.2963421461690833869, 0.3033979115540614835, 0.3104536769390397466, 0.3175094423240178432, 0.3245652077089959953, 0.3316209730939742029, 0.3386767384789523549, 0.3457325038639306181, 0.3527882692489087146, 0.3598440346338869222, 0.3668998000188650743, 0.3739555654038432819, 0.3810113307888214340, 0.3880670961737995861, 0.3951228615587777937, 0.4021786269437559458, 0.4092343923287340979, 0.4162901577137123055, 0.4233459230986904576, 0.4304016884836686652, 0.4374574538686468728, 0.4445132192536250249, 0.4515689846386031769, 0.4586247500235813290, 0.4656805154085595366, 0.4727362807935376887, 0.4797920461785158963, 0.4868478115634940484, 0.4939035769484722005, 0.5009593423334504081, 0.5080151077184286157, 0.5150708731034067123, 0.5221266384883849199, 0.5291824038733631275, 0.5362381692583413351, 0.5432939346433194316, 0.5503497000282975282, 0.5574054654132758468, 0.5644612307982540544, 0.5715169961832321510, 0.5785727615682102476, 0.5856285269531883442, 0.5926842923381667738, 0.5997400577231448704, 0.6067958231081229670, 0.6138515884931011746, 0.6209073538780794932, 0.6279631192630575898, 0.6350188846480356863, 0.6420746500330138939, 0.6491304154179919905, 0.6561861808029703091, 0.6632419461879484057, 0.6702977115729266133, 0.6773534769579047099, 0.6844092423428829175, 0.6914650077278612361, 0.6985207731128393327, 0.7055765384978174293, 0.7126323038827955259, 0.7196880692677738445, 0.7267438346527520521, 0.7337996000377301486, 0.7408553654227082452, 0.7479111308076865638, 0.7549668961926647714, 0.7620226615776428680, 0.7690784269626210756, 0.7761341923475991722, 0.7831899577325773798, 0.7902457231175555874, 0.7973014885025337950, 0.8043572538875118916, 0.8114130192724900992, 0.8184687846574681958, 0.8255245500424465144, 0.8325803154274246110, 0.8396360808124027075, 0.8466918461973809151, 0.8537476115823591227, 0.8608033769673373303, 0.8678591423523154269, 0.8749149077372937455, 0.8819706731222718421, 0.8890264385072500497, 0.8960822038922281463, 0.9031379692772063539, 0.9101937346621845615, 0.9172495000471626581, 0.9243052654321408657, 0.9313610308171190733, 0.9384167962020972809, 0.9454725615870753774, 0.9525283269720535850, 0.9595840923570317926, 0.9666398577420098892, 0.9736956231269880968, 0.9807513885119663044, 0.9878071538969444010, 0.9900635123082154321 ),
 .UNSPECIFIED. ) 
 CURVE ( )  GEOMETRIC_REPRESENTATION_ITEM ( )  RATIONAL_B_SPLINE_CURVE ( ( 1.000000000000000000, 0.8660254037844387076, 1.000000000000000000, 0.8660254037844387076, 1.000000000000000000, 0.8660254037844387076, 1.000000000000000000, 0.8660254037844387076, 1.000000000000000000, 0.8660254037844387076, 1.000000000000000000, 0.8660254037844387076, 1.000000000000000000, 0.8660254037844387076, 1.000000000000000000, 0.8660254037844387076, 1.000000000000000000, 0.8660254037844387076, 1.000000000000000000, 0.8660254037844387076, 1.000000000000000000, 0.8660254037844387076, 1.000000000000000000, 0.8660254037844387076, 1.000000000000000000, 0.8660254037844387076, 1.000000000000000000, 0.8660254037844387076, 1.000000000000000000, 0.8660254037844387076, 1.000000000000000000, 0.8660254037844387076, 1.000000000000000000, 0.8660254037844387076, 1.000000000000000000, 0.8660254037844387076, 1.000000000000000000, 0.8660254037844387076, 1.000000000000000000, 0.8660254037844387076, 1.000000000000000000, 0.8660254037844387076, 1.000000000000000000, 0.8660254037844387076, 1.000000000000000000, 0.8660254037844387076, 1.000000000000000000, 0.8660254037844387076, 1.000000000000000000, 0.8660254037844387076, 1.000000000000000000, 0.8660254037844387076, 1.000000000000000000, 0.8660254037844387076, 1.000000000000000000, 0.8660254037844387076, 1.000000000000000000, 0.8660254037844387076, 1.000000000000000000, 0.8660254037844387076, 1.000000000000000000, 0.8660254037844387076, 1.000000000000000000, 0.8660254037844387076, 1.000000000000000000, 0.8660254037844387076, 1.000000000000000000, 0.8660254037844387076, 1.000000000000000000, 0.8660254037844387076, 1.000000000000000000, 0.8660254037844387076, 1.000000000000000000, 0.8660254037844387076, 1.000000000000000000, 0.8660254037844387076, 1.000000000000000000, 0.8660254037844387076, 1.000000000000000000, 0.8660254037844387076, 1.000000000000000000, 0.8660254037844387076, 1.000000000000000000, 0.8660254037844387076, 1.000000000000000000, 0.8660254037844387076, 1.000000000000000000, 0.8660254037844387076, 1.000000000000000000, 0.8660254037844387076, 1.000000000000000000, 0.8660254037844387076, 1.000000000000000000, 0.8660254037844387076, 1.000000000000000000, 0.8660254037844387076, 1.000000000000000000, 0.8660254037844387076, 1.000000000000000000, 0.8660254037844387076, 1.000000000000000000, 0.8660254037844387076, 1.000000000000000000, 0.8660254037844387076, 1.000000000000000000, 0.8660254037844387076, 1.000000000000000000, 0.8660254037844387076, 1.000000000000000000, 0.8660254037844387076, 1.000000000000000000, 0.8660254037844387076, 1.000000000000000000, 0.8660254037844387076, 1.000000000000000000, 0.8660254037844387076, 1.000000000000000000, 0.8660254037844387076, 1.000000000000000000, 0.8660254037844387076, 1.000000000000000000, 0.8660254037844387076, 1.000000000000000000, 0.8660254037844387076, 1.000000000000000000, 0.8660254037844387076, 1.000000000000000000, 0.8660254037844387076, 1.000000000000000000, 0.8660254037844387076, 1.000000000000000000, 0.8660254037844387076, 1.000000000000000000, 0.8660254037844387076, 1.000000000000000000, 0.8660254037844387076, 1.000000000000000000, 0.8660254037844387076, 1.000000000000000000, 0.8660254037844387076, 1.000000000000000000, 0.8660254037844387076, 1.000000000000000000, 0.8660254037844387076, 1.000000000000000000, 0.8660254037844387076, 1.000000000000000000, 0.8660254037844387076, 1.000000000000000000, 0.8660254037844387076, 1.000000000000000000, 0.8660254037844387076, 1.000000000000000000, 0.8660254037844387076, 1.000000000000000000, 0.8660254037844387076, 1.000000000000000000, 0.8660254037844387076, 1.000000000000000000, 0.8660254037844387076, 1.000000000000000000, 0.8660254037844387076, 1.000000000000000000, 0.8660254037844387076, 1.000000000000000000, 0.8660254037844387076, 1.000000000000000000, 0.8660254037844387076, 1.000000000000000000, 0.8660254037844387076, 1.000000000000000000, 0.8660254037844387076, 1.000000000000000000, 0.8660254037844387076, 1.000000000000000000, 0.8660254037844387076, 1.000000000000000000, 0.8660254037844387076, 1.000000000000000000, 0.8660254037844387076, 1.000000000000000000, 0.8660254037844387076, 1.000000000000000000, 0.8660254037844387076, 1.000000000000000000, 0.8660254037844387076, 1.000000000000000000, 0.8660254037844387076, 1.000000000000000000, 0.8660254037844387076, 1.000000000000000000, 0.8660254037844387076, 1.000000000000000000, 0.8660254037844387076, 1.000000000000000000, 0.8660254037844387076, 1.000000000000000000, 0.8660254037844387076, 1.000000000000000000, 0.8660254037844387076, 1.000000000000000000, 0.8660254037844387076, 1.000000000000000000, 0.8660254037844387076, 1.000000000000000000, 0.8660254037844387076, 1.000000000000000000, 0.8660254037844387076, 1.000000000000000000, 0.8660254037844387076, 1.000000000000000000, 0.8660254037844387076, 1.000000000000000000, 0.8660254037844387076, 1.000000000000000000, 0.8660254037844387076, 1.000000000000000000, 0.8660254037844387076, 1.000000000000000000, 0.8660254037844387076, 1.000000000000000000, 0.8660254037844387076, 1.000000000000000000, 0.8660254037844387076, 1.000000000000000000, 0.8660254037844387076, 1.000000000000000000, 0.8660254037844387076, 1.000000000000000000, 0.8660254037844387076, 1.000000000000000000, 0.8660254037844387076, 1.000000000000000000, 0.8660254037844387076, 1.000000000000000000, 0.8660254037844387076, 1.000000000000000000, 0.8660254037844387076, 1.000000000000000000, 0.8660254037844387076, 1.000000000000000000, 0.8660254037844387076, 1.000000000000000000, 0.8660254037844387076, 1.000000000000000000, 0.8660254037844387076, 1.000000000000000000, 0.8660254037844387076, 1.000000000000000000, 0.8660254037844387076, 1.000000000000000000, 0.8660254037844387076, 1.000000000000000000, 0.8660254037844387076, 1.000000000000000000, 0.8660254037844387076, 1.000000000000000000, 0.8660254037844387076, 1.000000000000000000, 0.8660254037844387076, 1.000000000000000000, 0.8660254037844387076, 1.000000000000000000, 0.8660254037844387076, 1.000000000000000000, 0.8660254037844387076, 1.000000000000000000, 0.8660254037844387076, 1.000000000000000000, 0.8660254037844387076, 1.000000000000000000, 0.8660254037844387076, 1.000000000000000000, 0.8660254037844387076, 1.000000000000000000, 0.8660254037844387076, 1.000000000000000000, 0.8660254037844387076, 1.000000000000000000, 0.8660254037844387076, 1.000000000000000000, 0.9571563550410552290, 0.9417145902178747363 ) ) 
 REPRESENTATION_ITEM ( '' )  );
#13645=CARTESIAN_POINT ( 'NONE',  ( -92.69370383062498320, -211.3315407142195852, 76.09614583420048461 ) ) ;
#13651=EDGE_CURVE ( 'NONE', #51512, #30764, #2454, .T. ) ;
#13653=CARTESIAN_POINT ( 'NONE',  ( 97.30629616937498838, -211.3315407142195852, 75.30239583420048177 ) ) ;
#13656=CARTESIAN_POINT ( 'NONE',  ( 92.34999999999999432, 90.00000000000002842, 86.90437500173429441 ) ) ;
#13659=ORIENTED_EDGE ( 'NONE', *, *, #38596, .F. ) ;
#13668=CARTESIAN_POINT ( 'NONE',  ( 95.00000000000000000, -206.9400435732949575, 76.58562500173430010 ) ) ;
#13669=EDGE_CURVE ( 'NONE', #57350, #63128, #37731, .T. ) ;
#13674=CARTESIAN_POINT ( 'NONE',  ( 96.15314808468748708, 88.00268892867053694, 78.58322916753382970 ) ) ;
#13675=CARTESIAN_POINT ( 'NONE',  ( 92.35003969675446456, -211.5300011322842977, 88.86229325377448163 ) ) ;
#13678=ORIENTED_EDGE ( 'NONE', *, *, #61789, .F. ) ;
#13685=CARTESIAN_POINT ( 'NONE',  ( 92.34999999999999432, 91.52997821335252127, 77.96145833506763267 ) ) ;
#13689=CARTESIAN_POINT ( 'NONE',  ( -97.64999999999996305, -209.9999999999999716, 74.83937500173429669 ) ) ;
#13690=CARTESIAN_POINT ( 'NONE',  ( -95.00000000000002842, 92.66308142843932671, 88.37281250086715545 ) ) ;
#13691=CARTESIAN_POINT ( 'NONE',  ( 96.32499999999998863, 87.70503267997126784, 76.32104166840096582 ) ) ;
#13692=CARTESIAN_POINT ( 'NONE',  ( -92.35000000000003695, 90.00000000000004263, 77.06187500173429328 ) ) ;
#13695=CARTESIAN_POINT ( 'NONE',  ( 96.15314808468748708, 88.00268892867053694, 75.40822916753381833 ) ) ;
#13698=CARTESIAN_POINT ( 'NONE',  ( 0.000000000000000000, 80.00000000000000000, -90.00000000000000000 ) ) ;
#13699=CYLINDRICAL_SURFACE ( 'NONE', #43242, 2.649999999999985700 ) ;
#13702=EDGE_LOOP ( 'NONE', ( #6734, #10999, #15978, #68990 ) ) ;
#13712=AXIS2_PLACEMENT_3D ( 'NONE', #4308, #22318, #61810 ) ;
#13717=EDGE_CURVE ( 'NONE', #39802, #41314, #42624, .T. ) ;
#13723=DIRECTION ( 'NONE',  ( -0.000000000000000000, -0.000000000000000000, 1.000000000000000000 ) ) ;
#13728=EDGE_CURVE ( 'NONE', #60757, #428, #38251, .T. ) ;
#13730=VECTOR ( 'NONE', #16785, 1000.000000000000000 ) ;
#13731=CARTESIAN_POINT ( 'NONE',  ( 96.15314808468748708, 91.99731107132950569, 82.60489583420049087 ) ) ;
#13733=CARTESIAN_POINT ( 'NONE',  ( -97.30629616937497417, -208.6684592857803295, 87.20864583420048177 ) ) ;
#13736=CARTESIAN_POINT ( 'NONE',  ( -97.64999999999996305, -209.9999999999999716, 81.10999999999999943 ) ) ;
#13737=CARTESIAN_POINT ( 'NONE',  ( -97.64999999999994884, -208.4700217866474645, 80.42208333333331893 ) ) ;
#13738=CARTESIAN_POINT ( 'NONE',  ( -92.69370383062504004, 90.00000000000004263, 75.35531250086714294 ) ) ;
#13740=CARTESIAN_POINT ( 'NONE',  ( 97.30629616937498838, -208.6684592857803011, 86.20322916753382003 ) ) ;
#13747=CARTESIAN_POINT ( 'NONE',  ( -92.35000000000003695, 90.00000015433754186, 79.60187500750917877 ) ) ;
#13753=CARTESIAN_POINT ( 'NONE',  ( 97.30629616937498838, -211.3315407142195852, 79.27114583420048177 ) ) ;
#13758=CARTESIAN_POINT ( 'NONE',  ( -95.00000000000002842, 90.00000000000004263, 90.00000000000000000 ) ) ;
#13763=CARTESIAN_POINT ( 'NONE',  ( 96.32499999999998863, -212.2949673200287179, 81.95666666666666345 ) ) ;
#13764=ORIENTED_EDGE ( 'NONE', *, *, #6940, .F. ) ;
#13765=ORIENTED_EDGE ( 'NONE', *, *, #13669, .F. ) ;
#13767=ORIENTED_EDGE ( 'NONE', *, *, #38528, .F. ) ;
#13769=CARTESIAN_POINT ( 'NONE',  ( -96.15314808468751551, 88.00268892867056536, 84.19239583420049655 ) ) ;
#13772=( BOUNDED_CURVE ( )  B_SPLINE_CURVE ( 2, ( #5531, #74303, #45755, #16421, #68303, #16798, #39735 ),
 .UNSPECIFIED., .F., .F. ) 
 B_SPLINE_CURVE_WITH_KNOTS ( ( 3, 2, 2, 3 ),
 ( 0.7083333333333331483, 0.7152777777777775681, 0.7222222222222220989, 0.7291666666666665186 ),
 .UNSPECIFIED. ) 
 CURVE ( )  GEOMETRIC_REPRESENTATION_ITEM ( )  RATIONAL_B_SPLINE_CURVE ( ( 1.000000000000004219, 0.8660254037844343777, 1.000000000000000000, 0.8660254037844387076, 1.000000000000000000, 0.8660254037844408170, 0.9999999999999978906 ) ) 
 REPRESENTATION_ITEM ( '' )  );
#13773=CARTESIAN_POINT ( 'NONE',  ( 94.99999999999998579, 86.94004357329500010, 75.55375000000000796 ) ) ;
#13775=CARTESIAN_POINT ( 'NONE',  ( 94.99999999999998579, 93.05995642670504253, 79.68124999999999147 ) ) ;
#13776=EDGE_LOOP ( 'NONE', ( #14176, #35760, #5499, #20793 ) ) ;
#13779=CARTESIAN_POINT ( 'NONE',  ( -93.67500000000003979, 87.70503267997129626, 85.84604166840097150 ) ) ;
#13780=CARTESIAN_POINT ( 'NONE',  ( 92.69370383062498320, 90.00000000000002842, 85.35656250086715602 ) ) ;
#13783=CARTESIAN_POINT ( 'NONE',  ( -94.99999999999997158, -206.9400435732949575, 78.49062500173430124 ) ) ;
#13793=CARTESIAN_POINT ( 'NONE',  ( -96.32500000000001705, 92.29496732002878900, 75.36854166840096525 ) ) ;
#13794=CARTESIAN_POINT ( 'NONE',  ( -92.69370383062498320, -208.6684592857803011, 83.18697916753382060 ) ) ;
#13795=ORIENTED_EDGE ( 'NONE', *, *, #51192, .T. ) ;
#13798=ORIENTED_EDGE ( 'NONE', *, *, #62661, .F. ) ;
#13800=ORIENTED_EDGE ( 'NONE', *, *, #47609, .F. ) ;
#13802=CARTESIAN_POINT ( 'NONE',  ( 97.30629616937498838, 90.00000000000002842, 89.48406250086715374 ) ) ;
#13804=CARTESIAN_POINT ( 'NONE',  ( 96.15314808468748708, 88.00268892867053694, 80.32947916753380468 ) ) ;
#13818=CARTESIAN_POINT ( 'NONE',  ( -95.00000000000002842, 87.33691857156074434, 86.62656250086713783 ) ) ;
#13819=CARTESIAN_POINT ( 'NONE',  ( 97.64999999999999147, 90.00000000000002842, 79.52249999999999375 ) ) ;
#13821=FACE_OUTER_BOUND ( 'NONE', #21044, .T. ) ;
#13829=CARTESIAN_POINT ( 'NONE',  ( 93.84685191531251292, -211.9973110713294489, 82.92239583420048632 ) ) ;
#13830=ORIENTED_EDGE ( 'NONE', *, *, #829, .F. ) ;
#13841=CARTESIAN_POINT ( 'NONE',  ( 95.00000000000000000, -207.3369185715606307, 80.11781250086714579 ) ) ;
#13852=CARTESIAN_POINT ( 'NONE',  ( 92.35000000000000853, -209.9999999999999716, 84.99937500173429328 ) ) ;
#13853=CARTESIAN_POINT ( 'NONE',  ( 93.67499999999999716, 87.70503267997126784, 83.75583333333332803 ) ) ;
#13854=VERTEX_POINT ( 'NONE', #33175 ) ;
#13860=( BOUNDED_CURVE ( )  B_SPLINE_CURVE ( 2, ( #10610, #129, #10237, #45590, #62127, #22643, #17367, #34656, #74133, #63246, #51575, #44470, #34283, #57605, #16626, #6106, #11348, #33161, #68880, #27529, #17005, #33534, #21893, #4998, #57226, #62513, #67387, #27900, #56110, #39565, #39939, #29013, #73758, #5371, #4630, #51943, #491, #23023, #15886, #50462, #38820, #45956, #68513, #44839, #61759, #67767, #22272, #10991, #16253, #39191, #62890, #45210, #68130, #28266, #51202, #6821, #52688, #47420, #1964, #12092, #29734, #64350, #1237, #13200, #18830, #35031, #24131, #47062, #53792, #36130, #1600, #7568, #69240, #64717, #69964, #59080, #18467, #17731, #12822, #47781, #23742, #23388, #30844, #46313, #57963, #65092, #41409, #40678, #30116, #30483, #59444, #63981, #53428, #63622, #24486, #41051, #70326, #70701, #13564, #53065, #42159, #35750, #58701, #29373, #52315, #24850, #7930, #69610, #41772, #35400, #19209, #36494, #12458, #856, #58329, #6468, #7198, #46684, #18111, #65462, #48886, #8681, #2341, #19571, #44004, #9406, #37985, #20692, #14311, #9040, #32332, #25233, #55276, #26333, #71070, #2707, #9785, #3425, #60197, #66917, #21053, #72185, #3064, #25588, #26691, #31592, #49259, #42520, #15412, #25960, #59817, #36867, #54535, #15046, #42896, #3796, #31228, #48160, #20322, #8305, #61296, #48521, #60562, #38360, #32698, #43643, #31961, #54180, #66566, #49618, #19940, #43280, #13927, #71440, #60916, #71809, #65824, #37258, #72547, #66203, #14678, #37627, #54902, #40214, #45501, #57147, #68044, #38734, #56776, #44753, #11623, #45125, #39481, #56016, #68431, #44374, #10148, #16920, #11267, #67301, #21414, #27059, #16534, #5654, #4536, #72910, #67677, #16165, #28183, #51120, #27435, #4914, #15799, #28546, #61663, #62805, #33072, #62429, #10517, #62042, #55644, #51486, #22938, #10906, #47, #34200, #4162, #39858, #68800, #27814, #45879, #22554, #50372, #17281, #73293, #74044, #50743, #49992, #63167, #39104, #33829, #21806, #33444, #56407, #73666, #22182, #5285, #40963, #24043, #408, #53339, #19123, #13107, #1876, #17653, #47695, #42071, #40582, #52226, #58990, #58241, #35665, #18023, #24765, #70605, #58603, #7105, #6742, #773, #36044, #30029, #46967, #29648, #47333, #12737, #12370, #65002, #18746, #63530, #46593, #52972, #6025, #52589 ),
 .UNSPECIFIED., .F., .F. ) 
 B_SPLINE_CURVE_WITH_KNOTS ( ( 3, 2, 2, 2, 2, 2, 2, 2, 2, 2, 2, 2, 2, 2, 2, 2, 2, 2, 2, 2, 2, 2, 2, 2, 2, 2, 2, 2, 2, 2, 2, 2, 2, 2, 2, 2, 2, 2, 2, 2, 2, 2, 2, 2, 2, 2, 2, 2, 2, 2, 2, 2, 2, 2, 2, 2, 2, 2, 2, 2, 2, 2, 2, 2, 2, 2, 2, 2, 2, 2, 2, 2, 2, 2, 2, 2, 2, 2, 2, 2, 2, 2, 2, 2, 2, 2, 2, 2, 2, 2, 2, 2, 2, 2, 2, 2, 2, 2, 2, 2, 2, 2, 2, 2, 2, 2, 2, 2, 2, 2, 2, 2, 2, 2, 2, 2, 2, 2, 2, 2, 2, 2, 2, 2, 2, 2, 2, 2, 2, 2, 2, 2, 2, 2, 2, 2, 2, 2, 2, 2, 2, 3 ),
 ( 0.000000000000000000, 0.007055765384978174640, 0.01411153076995634928, 0.02116729615493452565, 0.02822306153991269856, 0.03527882692489087146, 0.04233459230986905131, 0.04939035769484722421, 0.05644612307982539712, 0.06350188846480357696, 0.07055765384978174293, 0.07761341923475992277, 0.08466918461973810262, 0.09172495000471626858, 0.09878071538969444843, 0.1058364807746726144, 0.1128922461596507942, 0.1199480115446289741, 0.1270037769296071539, 0.1340595423145853060, 0.1411153076995634859, 0.1481710730845416657, 0.1552268384695198455, 0.1622826038544980254, 0.1693383692394762052, 0.1763941346244543573, 0.1834499000094325372, 0.1905056653944107170, 0.1975614307793888969, 0.2046171961643670767, 0.2116729615493452288, 0.2187287269343234086, 0.2257844923193015885, 0.2328402577042797683, 0.2398960230892579482, 0.2469517884742361002, 0.2540075538592143078, 0.2610633192441924599, 0.2681190846291706120, 0.2751748500141488196, 0.2822306153991269717, 0.2892863807841051793, 0.2963421461690833314, 0.3033979115540614835, 0.3104536769390396911, 0.3175094423240178432, 0.3245652077089960508, 0.3316209730939742029, 0.3386767384789524105, 0.3457325038639305625, 0.3527882692489087146, 0.3598440346338869222, 0.3668998000188650743, 0.3739555654038432819, 0.3810113307888214340, 0.3880670961737995861, 0.3951228615587777937, 0.4021786269437559458, 0.4092343923287341534, 0.4162901577137123055, 0.4233459230986904576, 0.4304016884836686652, 0.4374574538686468173, 0.4445132192536250249, 0.4515689846386031769, 0.4586247500235813290, 0.4656805154085595366, 0.4727362807935376887, 0.4797920461785158963, 0.4868478115634940484, 0.4939035769484722005, 0.5009593423334504081, 0.5080151077184286157, 0.5150708731034067123, 0.5221266384883849199, 0.5291824038733631275, 0.5362381692583412240, 0.5432939346433194316, 0.5503497000282976392, 0.5574054654132758468, 0.5644612307982539434, 0.5715169961832320400, 0.5785727615682103586, 0.5856285269531884552, 0.5926842923381666628, 0.5997400577231448704, 0.6067958231081229670, 0.6138515884931011746, 0.6209073538780793822, 0.6279631192630575898, 0.6350188846480356863, 0.6420746500330137829, 0.6491304154179921015, 0.6561861808029703091, 0.6632419461879484057, 0.6702977115729265023, 0.6773534769579048209, 0.6844092423428830285, 0.6914650077278611251, 0.6985207731128393327, 0.7055765384978174293, 0.7126323038827956369, 0.7196880692677738445, 0.7267438346527520521, 0.7337996000377301486, 0.7408553654227082452, 0.7479111308076865638, 0.7549668961926647714, 0.7620226615776428680, 0.7690784269626209646, 0.7761341923475991722, 0.7831899577325774908, 0.7902457231175555874, 0.7973014885025336840, 0.8043572538875118916, 0.8114130192724900992, 0.8184687846574683068, 0.8255245500424464034, 0.8325803154274246110, 0.8396360808124027075, 0.8466918461973809151, 0.8537476115823592338, 0.8608033769673373303, 0.8678591423523154269, 0.8749149077372936345, 0.8819706731222718421, 0.8890264385072500497, 0.8960822038922281463, 0.9031379692772063539, 0.9101937346621845615, 0.9172495000471626581, 0.9243052654321408657, 0.9313610308171190733, 0.9384167962020972809, 0.9454725615870753774, 0.9525283269720535850, 0.9595840923570317926, 0.9666398577420098892, 0.9736956231269880968, 0.9807513885119663044, 0.9878071538969444010, 0.9900635123082155431 ),
 .UNSPECIFIED. ) 
 CURVE ( )  GEOMETRIC_REPRESENTATION_ITEM ( )  RATIONAL_B_SPLINE_CURVE ( ( 1.000000000000000000, 0.8660254037844387076, 1.000000000000000000, 0.8660254037844387076, 1.000000000000000000, 0.8660254037844387076, 1.000000000000000000, 0.8660254037844387076, 1.000000000000000000, 0.8660254037844387076, 1.000000000000000000, 0.8660254037844387076, 1.000000000000000000, 0.8660254037844387076, 1.000000000000000000, 0.8660254037844387076, 1.000000000000000000, 0.8660254037844387076, 1.000000000000000000, 0.8660254037844387076, 1.000000000000000000, 0.8660254037844387076, 1.000000000000000000, 0.8660254037844387076, 1.000000000000000000, 0.8660254037844387076, 1.000000000000000000, 0.8660254037844387076, 1.000000000000000000, 0.8660254037844387076, 1.000000000000000000, 0.8660254037844387076, 1.000000000000000000, 0.8660254037844387076, 1.000000000000000000, 0.8660254037844387076, 1.000000000000000000, 0.8660254037844387076, 1.000000000000000000, 0.8660254037844387076, 1.000000000000000000, 0.8660254037844387076, 1.000000000000000000, 0.8660254037844387076, 1.000000000000000000, 0.8660254037844387076, 1.000000000000000000, 0.8660254037844387076, 1.000000000000000000, 0.8660254037844387076, 1.000000000000000000, 0.8660254037844387076, 1.000000000000000000, 0.8660254037844387076, 1.000000000000000000, 0.8660254037844387076, 1.000000000000000000, 0.8660254037844387076, 1.000000000000000000, 0.8660254037844387076, 1.000000000000000000, 0.8660254037844387076, 1.000000000000000000, 0.8660254037844387076, 1.000000000000000000, 0.8660254037844387076, 1.000000000000000000, 0.8660254037844387076, 1.000000000000000000, 0.8660254037844387076, 1.000000000000000000, 0.8660254037844387076, 1.000000000000000000, 0.8660254037844387076, 1.000000000000000000, 0.8660254037844387076, 1.000000000000000000, 0.8660254037844387076, 1.000000000000000000, 0.8660254037844387076, 1.000000000000000000, 0.8660254037844387076, 1.000000000000000000, 0.8660254037844387076, 1.000000000000000000, 0.8660254037844387076, 1.000000000000000000, 0.8660254037844387076, 1.000000000000000000, 0.8660254037844387076, 1.000000000000000000, 0.8660254037844387076, 1.000000000000000000, 0.8660254037844387076, 1.000000000000000000, 0.8660254037844387076, 1.000000000000000000, 0.8660254037844387076, 1.000000000000000000, 0.8660254037844387076, 1.000000000000000000, 0.8660254037844387076, 1.000000000000000000, 0.8660254037844387076, 1.000000000000000000, 0.8660254037844387076, 1.000000000000000000, 0.8660254037844387076, 1.000000000000000000, 0.8660254037844387076, 1.000000000000000000, 0.8660254037844387076, 1.000000000000000000, 0.8660254037844387076, 1.000000000000000000, 0.8660254037844387076, 1.000000000000000000, 0.8660254037844387076, 1.000000000000000000, 0.8660254037844387076, 1.000000000000000000, 0.8660254037844387076, 1.000000000000000000, 0.8660254037844387076, 1.000000000000000000, 0.8660254037844387076, 1.000000000000000000, 0.8660254037844387076, 1.000000000000000000, 0.8660254037844387076, 1.000000000000000000, 0.8660254037844387076, 1.000000000000000000, 0.8660254037844387076, 1.000000000000000000, 0.8660254037844387076, 1.000000000000000000, 0.8660254037844387076, 1.000000000000000000, 0.8660254037844387076, 1.000000000000000000, 0.8660254037844387076, 1.000000000000000000, 0.8660254037844387076, 1.000000000000000000, 0.8660254037844387076, 1.000000000000000000, 0.8660254037844387076, 1.000000000000000000, 0.8660254037844387076, 1.000000000000000000, 0.8660254037844387076, 1.000000000000000000, 0.8660254037844387076, 1.000000000000000000, 0.8660254037844387076, 1.000000000000000000, 0.8660254037844387076, 1.000000000000000000, 0.8660254037844387076, 1.000000000000000000, 0.8660254037844387076, 1.000000000000000000, 0.8660254037844387076, 1.000000000000000000, 0.8660254037844387076, 1.000000000000000000, 0.8660254037844387076, 1.000000000000000000, 0.8660254037844387076, 1.000000000000000000, 0.8660254037844387076, 1.000000000000000000, 0.8660254037844387076, 1.000000000000000000, 0.8660254037844387076, 1.000000000000000000, 0.8660254037844387076, 1.000000000000000000, 0.8660254037844387076, 1.000000000000000000, 0.8660254037844387076, 1.000000000000000000, 0.8660254037844387076, 1.000000000000000000, 0.8660254037844387076, 1.000000000000000000, 0.8660254037844387076, 1.000000000000000000, 0.8660254037844387076, 1.000000000000000000, 0.8660254037844387076, 1.000000000000000000, 0.8660254037844387076, 1.000000000000000000, 0.8660254037844387076, 1.000000000000000000, 0.8660254037844387076, 1.000000000000000000, 0.8660254037844387076, 1.000000000000000000, 0.8660254037844387076, 1.000000000000000000, 0.8660254037844387076, 1.000000000000000000, 0.8660254037844387076, 1.000000000000000000, 0.8660254037844387076, 1.000000000000000000, 0.8660254037844387076, 1.000000000000000000, 0.8660254037844387076, 1.000000000000000000, 0.8660254037844387076, 1.000000000000000000, 0.8660254037844387076, 1.000000000000000000, 0.8660254037844387076, 1.000000000000000000, 0.8660254037844387076, 1.000000000000000000, 0.8660254037844387076, 1.000000000000000000, 0.8660254037844387076, 1.000000000000000000, 0.8660254037844387076, 1.000000000000000000, 0.8660254037844387076, 1.000000000000000000, 0.8660254037844387076, 1.000000000000000000, 0.8660254037844387076, 1.000000000000000000, 0.8660254037844387076, 1.000000000000000000, 0.8660254037844387076, 1.000000000000000000, 0.8660254037844387076, 1.000000000000000000, 0.8660254037844387076, 1.000000000000000000, 0.8660254037844387076, 1.000000000000000000, 0.8660254037844387076, 1.000000000000000000, 0.8660254037844387076, 1.000000000000000000, 0.8660254037844387076, 1.000000000000000000, 0.8660254037844387076, 1.000000000000000000, 0.8660254037844387076, 1.000000000000000000, 0.8660254037844387076, 1.000000000000000000, 0.8660254037844387076, 1.000000000000000000, 0.8660254037844387076, 1.000000000000000000, 0.8660254037844387076, 1.000000000000000000, 0.8660254037844387076, 1.000000000000000000, 0.8660254037844387076, 1.000000000000000000, 0.8660254037844387076, 1.000000000000000000, 0.8660254037844387076, 1.000000000000000000, 0.8660254037844387076, 1.000000000000000000, 0.8660254037844387076, 1.000000000000000000, 0.8660254037844387076, 1.000000000000000000, 0.8660254037844387076, 1.000000000000000000, 0.8660254037844387076, 1.000000000000000000, 0.8660254037844387076, 1.000000000000000000, 0.9571563550410531196, 0.9417145902178731820 ) ) 
 REPRESENTATION_ITEM ( '' )  );
#13861=CARTESIAN_POINT ( 'NONE',  ( -95.00000000000002842, 92.66308142843932671, 87.10281250086715943 ) ) ;
#13862=CARTESIAN_POINT ( 'NONE',  ( 97.30629616937498838, 90.00000000000002842, 80.43531250086714124 ) ) ;
#13863=ORIENTED_EDGE ( 'NONE', *, *, #64799, .F. ) ;
#13865=CARTESIAN_POINT ( 'NONE',  ( 92.34999999999999432, 88.47002178664753558, 85.05229166840096866 ) ) ;
#13868=CARTESIAN_POINT ( 'NONE',  ( 92.35003236756683975, -208.4700030992239874, 87.48645704240064447 ) ) ;
#13873=CARTESIAN_POINT ( 'NONE',  ( -97.65000000000001990, 90.00000000000004263, 76.66499999999999204 ) ) ;
#13875=CARTESIAN_POINT ( 'NONE',  ( -93.67500000000003979, 87.70503267997129626, 83.86166666666666458 ) ) ;
#13882=CARTESIAN_POINT ( 'NONE',  ( -93.84685191531248449, -208.0026889286704943, 81.81114583420047381 ) ) ;
#13890=EDGE_CURVE ( 'NONE', #68271, #14366, #9883, .T. ) ;
#13893=CARTESIAN_POINT ( 'NONE',  ( -97.64999999999996305, -209.9999999999999716, 85.55499999999999261 ) ) ;
#13896=CARTESIAN_POINT ( 'NONE',  ( 7.103376864691351012E-17, -120.0000000000000000, -80.00000000000000000 ) ) ;
#13897=CARTESIAN_POINT ( 'NONE',  ( -92.69370383062504004, 90.00000000000004263, 75.99031250086714806 ) ) ;
#13902=ADVANCED_FACE ( 'NONE', ( #47076 ), #6483, .F. ) ;
#13903=CARTESIAN_POINT ( 'NONE',  ( -92.34999999999999432, -210.0000001167898631, 84.68187499741277691 ) ) ;
#13906=CARTESIAN_POINT ( 'NONE',  ( 97.64999999999999147, -209.9999999999999716, 78.88750000000000284 ) ) ;
#13908=CARTESIAN_POINT ( 'NONE',  ( -92.34999999999999432, -209.9999999999999716, 86.50750000000000739 ) ) ;
#13919=ADVANCED_FACE ( 'NONE', ( #30133 ), #146, .T. ) ;
#13924=ADVANCED_FACE ( 'NONE', ( #18485 ), #35766, .F. ) ;
#13927=CARTESIAN_POINT ( 'NONE',  ( 96.15314808468748708, -208.0026889286704943, 80.54114583420046358 ) ) ;
#13928=CARTESIAN_POINT ( 'NONE',  ( 93.84685191531249870, -208.0026889286704943, 87.15572916753382060 ) ) ;
#13930=CARTESIAN_POINT ( 'NONE',  ( 92.69370383062501162, -208.6684592857803011, 88.47864583420047779 ) ) ;
#13935=ORIENTED_EDGE ( 'NONE', *, *, #45073, .F. ) ;
#13936=CARTESIAN_POINT ( 'NONE',  ( -97.30629616937501680, 90.00000000000004263, 75.83156250086716454 ) ) ;
#13938=ORIENTED_EDGE ( 'NONE', *, *, #71339, .T. ) ;
#13939=CARTESIAN_POINT ( 'NONE',  ( -92.34999999999999432, -210.0000000334413528, 87.85687500050293863 ) ) ;
#13951=CARTESIAN_POINT ( 'NONE',  ( 96.15314808468750130, -211.9973110713294489, 78.42447916753381776 ) ) ;
#13960=CARTESIAN_POINT ( 'NONE',  ( -97.65000000000003411, -211.5299782133524502, 75.44791666666667140 ) ) ;
#13964=CARTESIAN_POINT ( 'NONE',  ( -92.69370383062498320, -208.6684592857803011, 81.12322916753382174 ) ) ;
#13965=CARTESIAN_POINT ( 'NONE',  ( -95.00000000000002842, 92.66308142843932671, 78.84781250086714977 ) ) ;
#13967=CIRCLE ( 'NONE', #39211, 12.75000000000000000 ) ;
#13968=CARTESIAN_POINT ( 'NONE',  ( 92.69370383062498320, 91.33154071421968467, 82.60489583420047666 ) ) ;
#13970=ORIENTED_EDGE ( 'NONE', *, *, #18506, .F. ) ;
#13976=CARTESIAN_POINT ( 'NONE',  ( -94.99999999999997158, -212.6630814284392557, 81.54656250086713953 ) ) ;
#13990=CARTESIAN_POINT ( 'NONE',  ( -96.15314808468752972, 91.99731107132950569, 83.82197916753381151 ) ) ;
#13991=CARTESIAN_POINT ( 'NONE',  ( -97.30599797242217619, -209.0535479562712169, 74.89836836546777477 ) ) ;
#13995=CARTESIAN_POINT ( 'NONE',  ( -93.33921309982508774, 88.39975348990192572, 74.64190636928354650 ) ) ;
#14001=ADVANCED_FACE ( 'NONE', ( #5749 ), #45969, .F. ) ;
#14002=CYLINDRICAL_SURFACE ( 'NONE', #65243, 2.649999999999999467 ) ;
#14003=CARTESIAN_POINT ( 'NONE',  ( -94.99999999999997158, -212.6630814284392557, 84.24531250086715772 ) ) ;
#14012=PLANE ( 'NONE',  #56969 ) ;
#14016=EDGE_CURVE ( 'NONE', #51621, #4009, #12776, .T. ) ;
#14020=CARTESIAN_POINT ( 'NONE',  ( 92.69370383062501162, -208.6684592857803011, 88.47864583420047779 ) ) ;
#14033=ORIENTED_EDGE ( 'NONE', *, *, #53709, .T. ) ;
#14034=CARTESIAN_POINT ( 'NONE',  ( 92.35003715139268365, -208.4700003372809078, 76.69145685134846246 ) ) ;
#14038=CARTESIAN_POINT ( 'NONE',  ( 97.30629616937498838, 88.66845928578037217, 79.90614583420048689 ) ) ;
#14039=DIRECTION ( 'NONE',  ( -0.000000000000000000, 0.000000000000000000, 1.000000000000000000 ) ) ;
#14050=CARTESIAN_POINT ( 'NONE',  ( -97.64999999999999147, -210.0000225213925660, 84.36437578067156551 ) ) ;
#14053=CARTESIAN_POINT ( 'NONE',  ( -94.99999999999997158, -206.9400435732949575, 77.22062500173429100 ) ) ;
#14054=CARTESIAN_POINT ( 'NONE',  ( -95.00000000000002842, 87.33691857156074434, 88.05531250086716000 ) ) ;
#14055=CARTESIAN_POINT ( 'NONE',  ( 96.32499999999997442, 92.29496732002878900, 77.16770833506762983 ) ) ;
#14056=CARTESIAN_POINT ( 'NONE',  ( -92.35000000000005116, 91.52997821335253548, 75.20979166840096752 ) ) ;
#14058=CARTESIAN_POINT ( 'NONE',  ( 94.99999999999998579, 87.33691857156068750, 77.89531250086714920 ) ) ;
#14061=FACE_OUTER_BOUND ( 'NONE', #23975, .T. ) ;
#14078=CARTESIAN_POINT ( 'NONE',  ( -92.35000000000003695, 89.99999998014077107, 85.95187500101400246 ) ) ;
#14082=( BOUNDED_CURVE ( )  B_SPLINE_CURVE ( 2, ( #19410, #66405, #13404, #36332, #41992, #43487, #42359 ),
 .UNSPECIFIED., .F., .F. ) 
 B_SPLINE_CURVE_WITH_KNOTS ( ( 3, 2, 2, 3 ),
 ( 0.1874999999999999167, 0.1944444444444443365, 0.2013888888888887285, 0.2083333333333331483 ),
 .UNSPECIFIED. ) 
 CURVE ( )  GEOMETRIC_REPRESENTATION_ITEM ( )  RATIONAL_B_SPLINE_CURVE ( ( 1.000000000000001554, 0.8660254037844371533, 1.000000000000000000, 0.8660254037844387076, 1.000000000000000000, 0.8660254037844424824, 0.9999999999999962252 ) ) 
 REPRESENTATION_ITEM ( '' )  );
#14083=CARTESIAN_POINT ( 'NONE',  ( -93.33922900947476364, -211.6002630214759961, 74.80065534806806227 ) ) ;
#14088=AXIS2_PLACEMENT_3D ( 'NONE', #49454, #47984, #7759 ) ;
#14093=CARTESIAN_POINT ( 'NONE',  ( -94.99999999999997158, -213.0599564267049857, 76.18874999999999886 ) ) ;
#14098=CARTESIAN_POINT ( 'NONE',  ( 93.84685191531248449, 88.00268892867053694, 84.19239583420049655 ) ) ;
#14099=CARTESIAN_POINT ( 'NONE',  ( -93.84685191531247028, -211.9973110713294489, 86.20322916753382003 ) ) ;
#14100=CARTESIAN_POINT ( 'NONE',  ( 92.35000000049316782, -210.0000320386632495, 83.73041644179299681 ) ) ;
#14101=ORIENTED_EDGE ( 'NONE', *, *, #61002, .T. ) ;
#14103=CARTESIAN_POINT ( 'NONE',  ( -97.64999999999996305, -209.9999999999999716, 81.74500000000000455 ) ) ;
#14104=CARTESIAN_POINT ( 'NONE',  ( -97.65000000000001990, 90.00000000000004263, 84.92000000000000171 ) ) ;
#14107=CARTESIAN_POINT ( 'NONE',  ( 92.69370383062501162, -209.9999999999999716, 85.19781250086714408 ) ) ;
#14117=CARTESIAN_POINT ( 'NONE',  ( -99.99999999999998579, -124.0000000000000142, -40.00000000000002132 ) ) ;
#14118=CARTESIAN_POINT ( 'NONE',  ( 92.69370383062501162, -211.3315407142195852, 79.69447916753381378 ) ) ;
#14121=CARTESIAN_POINT ( 'NONE',  ( 95.00000000000000000, -213.0599564267049857, 80.63375000000000625 ) ) ;
#14125=CARTESIAN_POINT ( 'NONE',  ( 97.64999999999997726, -211.5299782133524502, 80.73958333333332860 ) ) ;
#14133=CARTESIAN_POINT ( 'NONE',  ( -95.00000000000002842, 92.66308142843932671, 85.19781250086714408 ) ) ;
#14134=DIRECTION ( 'NONE',  ( 1.000000000000000000, 0.000000000000000000, 0.000000000000000000 ) ) ;
#14138=CARTESIAN_POINT ( 'NONE',  ( 93.67499999999999716, 87.70503267997126784, 75.50083333333331836 ) ) ;
#14143=VERTEX_POINT ( 'NONE', #54196 ) ;
#14144=CARTESIAN_POINT ( 'NONE',  ( -93.67499999999998295, -212.2949673200287179, 84.57604166840096127 ) ) ;
#14149=CARTESIAN_POINT ( 'NONE',  ( -93.67500000000003979, 87.70503267997129626, 87.11604166840096752 ) ) ;
#14152=CARTESIAN_POINT ( 'NONE',  ( 97.30629616937498838, 91.33154071421968467, 86.99697916753382287 ) ) ;
#14156=CARTESIAN_POINT ( 'NONE',  ( -92.35000000000005116, 88.47002178664754979, 83.99395833506763154 ) ) ;
#14162=ORIENTED_EDGE ( 'NONE', *, *, #41092, .F. ) ;
#14168=CARTESIAN_POINT ( 'NONE',  ( -94.99999999999997158, -212.6630814284392557, 84.24531250086715772 ) ) ;
#14176=ORIENTED_EDGE ( 'NONE', *, *, #26965, .F. ) ;
#14178=CARTESIAN_POINT ( 'NONE',  ( 92.34999999999999432, 90.00000000000002842, 86.82500000000000284 ) ) ;
#14181=CARTESIAN_POINT ( 'NONE',  ( 92.69370383062498320, 91.33154071421968467, 76.88989583420047325 ) ) ;
#14186=CARTESIAN_POINT ( 'NONE',  ( 95.29776683160947925, 92.36156954995058754, 74.83035915144989758 ) ) ;
#14194=CARTESIAN_POINT ( 'NONE',  ( -95.00000000000002842, 87.33691857156074434, 87.26156250086714294 ) ) ;
#14206=CARTESIAN_POINT ( 'NONE',  ( 97.30629616937498838, -209.9999999999999716, 81.86406250086714920 ) ) ;
#14211=DIRECTION ( 'NONE',  ( 0.000000000000000000, 0.000000000000000000, 1.000000000000000000 ) ) ;
#14216=CARTESIAN_POINT ( 'NONE',  ( 92.35000000000000853, -209.9999999999999716, 90.00000000000000000 ) ) ;
#14229=CARTESIAN_POINT ( 'NONE',  ( 95.00000000000000000, -213.0599564267049857, 85.15812500173430521 ) ) ;
#14230=CARTESIAN_POINT ( 'NONE',  ( 97.64999999999999147, 90.00000000000002842, 85.87249999999998806 ) ) ;
#14237=CARTESIAN_POINT ( 'NONE',  ( -92.69370383062505425, 88.66845928578038638, 87.52614583420049144 ) ) ;
#14238=CARTESIAN_POINT ( 'NONE',  ( 93.84685191531248449, 91.99731107132950569, 82.55197916753380127 ) ) ;
#14240=CARTESIAN_POINT ( 'NONE',  ( 97.64999999999997726, 88.47002178664753558, 81.45395833506763950 ) ) ;
#14250=VERTEX_POINT ( 'NONE', #3444 ) ;
#14254=AXIS2_PLACEMENT_3D ( 'NONE', #45944, #50811, #28624 ) ;
#14255=CARTESIAN_POINT ( 'NONE',  ( -92.35000000000003695, 90.00000000000004263, 83.33250000000001023 ) ) ;
#14262=CARTESIAN_POINT ( 'NONE',  ( -92.69370383062498320, -209.9999999999999716, 80.43531250086714124 ) ) ;
#14274=CARTESIAN_POINT ( 'NONE',  ( 97.64999999999999147, 89.99999989488613039, 86.58687499784845443 ) ) ;
#14276=ADVANCED_FACE ( 'NONE', ( #73308 ), #17180, .F. ) ;
#14278=CARTESIAN_POINT ( 'NONE',  ( -93.84685191531252713, 88.00268892867056536, 75.88447916753381151 ) ) ;
#14290=CARTESIAN_POINT ( 'NONE',  ( -97.64999999999996305, -209.9999999999999716, 75.39499999999999602 ) ) ;
#14292=CARTESIAN_POINT ( 'NONE',  ( -94.99999999999997158, -206.9400435732949575, 87.93625000000000114 ) ) ;
#14303=VECTOR ( 'NONE', #37545, 1000.000000000000000 ) ;
#14305=VECTOR ( 'NONE', #8288, 1000.000000000000000 ) ;
#14307=DIRECTION ( 'NONE',  ( 0.000000000000000000, 0.000000000000000000, 1.000000000000000000 ) ) ;
#14310=( BOUNDED_CURVE ( )  B_SPLINE_CURVE ( 2, ( #13939, #47434, #59830, #8316, #7940, #70337, #64361, #70712, #42172 ),
 .UNSPECIFIED., .F., .F. ) 
 B_SPLINE_CURVE_WITH_KNOTS ( ( 3, 2, 2, 2, 3 ),
 ( 0.1058364832028025337, 0.1128922486546722892, 0.1199480141955893697, 0.1270037797365064502, 0.1270039290057624060 ),
 .UNSPECIFIED. ) 
 CURVE ( )  GEOMETRIC_REPRESENTATION_ITEM ( )  RATIONAL_B_SPLINE_CURVE ( ( 1.000000000000000000, 0.8660254037844387076, 1.000000000000000000, 0.8660254037844387076, 1.000000000000000000, 0.8660254037844387076, 1.000000000000000000, 0.9999971656812888243, 0.9999943314825013863 ) ) 
 REPRESENTATION_ITEM ( '' )  );
#14311=CARTESIAN_POINT ( 'NONE',  ( 96.15314808468750130, -211.9973110713294489, 82.86947916753379673 ) ) ;
#14312=CARTESIAN_POINT ( 'NONE',  ( 95.00000000000000000, -207.3369185715606307, 89.64281250086715147 ) ) ;
#14314=CARTESIAN_POINT ( 'NONE',  ( 96.15314808468748708, -208.0026889286704943, 86.41489583420049314 ) ) ;
#14315=VERTEX_POINT ( 'NONE', #9809 ) ;
#14318=CARTESIAN_POINT ( 'NONE',  ( -92.69370383062502583, 88.66845928578038638, 78.63614583420049087 ) ) ;
#14339=CARTESIAN_POINT ( 'NONE',  ( 96.15314808468748708, -208.0026889286704943, 77.36614583420046642 ) ) ;
#14341=CARTESIAN_POINT ( 'NONE',  ( -96.32500000000001705, 87.70503267997129626, 81.85083333333332689 ) ) ;
#14345=CARTESIAN_POINT ( 'NONE',  ( 92.34999999999999432, 90.00000000000002842, 76.03000000000000114 ) ) ;
#14347=CARTESIAN_POINT ( 'NONE',  ( -92.34999999999999432, -209.9999999999999716, 88.49187500173430010 ) ) ;
#14349=CARTESIAN_POINT ( 'NONE',  ( -92.69370383062498320, -209.9999999999999716, 81.70531250086713726 ) ) ;
#14350=CARTESIAN_POINT ( 'NONE',  ( -92.69370383062504004, 90.00000000000004263, 77.41906250086715602 ) ) ;
#14351=ORIENTED_EDGE ( 'NONE', *, *, #74092, .T. ) ;
#14353=CARTESIAN_POINT ( 'NONE',  ( 92.69370383062498320, 90.00000000000002842, 80.75281250086715090 ) ) ;
#14361=CARTESIAN_POINT ( 'NONE',  ( -96.15314808468745866, -211.9973110713294489, 84.03364583420047040 ) ) ;
#14363=CARTESIAN_POINT ( 'NONE',  ( -97.64999999947046661, -209.9999663481462164, 81.18829462297327382 ) ) ;
#14366=VERTEX_POINT ( 'NONE', #69907 ) ;
#14371=CARTESIAN_POINT ( 'NONE',  ( -92.35000000000003695, 90.00000000000004263, 90.00000000000000000 ) ) ;
#14372=FACE_OUTER_BOUND ( 'NONE', #54780, .T. ) ;
#14374=CARTESIAN_POINT ( 'NONE',  ( -92.69370383062502583, 88.66845928578038638, 86.73239583420047438 ) ) ;
#14375=CARTESIAN_POINT ( 'NONE',  ( -97.49696879394605276, -209.7556371990022512, 74.91343443312145212 ) ) ;
#14377=CARTESIAN_POINT ( 'NONE',  ( 97.64999999999999147, 90.00000000000002842, 77.61749999999999261 ) ) ;
#14380=FACE_OUTER_BOUND ( 'NONE', #59360, .T. ) ;
#14381=CARTESIAN_POINT ( 'NONE',  ( -96.32500000000001705, 92.29496732002878900, 82.35354166840096468 ) ) ;
#14384=DIRECTION ( 'NONE',  ( -0.000000000000000000, -0.000000000000000000, 1.000000000000000000 ) ) ;
#14385=CARTESIAN_POINT ( 'NONE',  ( -96.15314808468747287, -208.0026889286704943, 82.71072916753381321 ) ) ;
#14390=DIRECTION ( 'NONE',  ( -0.000000000000000000, -0.000000000000000000, 1.000000000000000000 ) ) ;
#14391=CARTESIAN_POINT ( 'NONE',  ( -99.99999999999997158, -214.9999999999999716, 90.00000000000000000 ) ) ;
#14394=CARTESIAN_POINT ( 'NONE',  ( -96.32500000000001705, 92.29496732002878900, 78.46416666666667084 ) ) ;
#14399=CARTESIAN_POINT ( 'NONE',  ( 93.84685191531251292, -211.9973110713294489, 75.14364583420046984 ) ) ;
#14406=EDGE_CURVE ( 'NONE', #71243, #54767, #6764, .T. ) ;
#14411=ORIENTED_EDGE ( 'NONE', *, *, #49563, .T. ) ;
#14412=EDGE_LOOP ( 'NONE', ( #46804, #43486, #8720, #43854 ) ) ;
#14413=EDGE_CURVE ( 'NONE', #2294, #39621, #51201, .T. ) ;
#14417=CARTESIAN_POINT ( 'NONE',  ( 97.65000000000000568, -208.4700217866474645, 76.47979166840096354 ) ) ;
#14421=CARTESIAN_POINT ( 'NONE',  ( 92.69370383062498320, 88.66845928578037217, 79.69447916753381378 ) ) ;
#14432=CYLINDRICAL_SURFACE ( 'NONE', #44921, 2.649999999999985700 ) ;
#14436=CARTESIAN_POINT ( 'NONE',  ( -97.64999999999994884, -208.4700217866474645, 75.42145833506764063 ) ) ;
#14439=CARTESIAN_POINT ( 'NONE',  ( 93.67499999999999716, 87.70503267997126784, 74.94520833506761903 ) ) ;
#14440=CARTESIAN_POINT ( 'NONE',  ( -95.00000000000002842, 87.33691857156074434, 87.89656250086713385 ) ) ;
#14442=CARTESIAN_POINT ( 'NONE',  ( 97.30629616937498838, 88.66845928578037217, 75.46114583420049371 ) ) ;
#14454=CARTESIAN_POINT ( 'NONE',  ( 94.99999999999998579, 90.00000000000002842, 90.00000000000000000 ) ) ;
#14457=VECTOR ( 'NONE', #67527, 1000.000000000000000 ) ;
#14461=CARTESIAN_POINT ( 'NONE',  ( 97.64999999999999147, -209.9999999999999716, 89.68250000000000455 ) ) ;
#14462=CARTESIAN_POINT ( 'NONE',  ( -96.32500000000001705, 87.70503267997129626, 76.21520833506762926 ) ) ;
#14478=CARTESIAN_POINT ( 'NONE',  ( 92.69370383062498320, 88.66845928578035796, 85.40947916753381719 ) ) ;
#14479=CARTESIAN_POINT ( 'NONE',  ( -92.69370383062498320, -211.3315407142195852, 81.81114583420048803 ) ) ;
#14482=CARTESIAN_POINT ( 'NONE',  ( 92.35000000000000853, -209.9999999999999716, 90.00000000000000000 ) ) ;
#14483=CARTESIAN_POINT ( 'NONE',  ( -92.34999999999999432, -209.9999999999999716, 79.52249999999999375 ) ) ;
#14485=CARTESIAN_POINT ( 'NONE',  ( 96.15314808468748708, -208.0026889286704943, 84.35114583420048007 ) ) ;
#14489=ORIENTED_EDGE ( 'NONE', *, *, #19612, .T. ) ;
#14496=CARTESIAN_POINT ( 'NONE',  ( 93.84685191531249870, -208.0026889286704943, 78.90072916753382515 ) ) ;
#14503=CARTESIAN_POINT ( 'NONE',  ( 97.64999999999997726, -208.4700217866474645, 80.21041666666666003 ) ) ;
#14508=ORIENTED_EDGE ( 'NONE', *, *, #70452, .T. ) ;
#14511=AXIS2_PLACEMENT_3D ( 'NONE', #22589, #10551, #28216 ) ;
#14513=CARTESIAN_POINT ( 'NONE',  ( -97.30629616937501680, 91.33154071421968467, 84.03364583420049883 ) ) ;
#14515=VECTOR ( 'NONE', #39833, 1000.000000000000000 ) ;
#14521=CARTESIAN_POINT ( 'NONE',  ( -96.32499999999996021, -207.7050326799711968, 87.43354166840096298 ) ) ;
#14526=CARTESIAN_POINT ( 'NONE',  ( -95.00000000000002842, 86.94004357329504273, 82.61812500173428475 ) ) ;
#14527=( BOUNDED_CURVE ( )  B_SPLINE_CURVE ( 2, ( #21505, #9125, #4994, #14765, #3515, #10233, #73004 ),
 .UNSPECIFIED., .F., .F. ) 
 B_SPLINE_CURVE_WITH_KNOTS ( ( 3, 2, 2, 3 ),
 ( 0.8890265259358467453, 0.8960822236920598094, 0.9031379892329426395, 0.9101937466091533091 ),
 .UNSPECIFIED. ) 
 CURVE ( )  GEOMETRIC_REPRESENTATION_ITEM ( )  RATIONAL_B_SPLINE_CURVE ( ( 0.9999974258394870308, 0.8660266908770603012, 1.000000000000000000, 0.8660254037844387076, 1.000000000000000000, 0.8660254037844387076, 1.000000000000000000 ) ) 
 REPRESENTATION_ITEM ( '' )  );
#14529=CARTESIAN_POINT ( 'NONE',  ( 94.99999999999998579, 92.66308142843935514, 87.10281250086715943 ) ) ;
#14533=CARTESIAN_POINT ( 'NONE',  ( 97.64999999999999147, 90.00000000000002842, 89.04749999999999943 ) ) ;
#14536=CARTESIAN_POINT ( 'NONE',  ( 93.67500000000001137, -207.7050326799711968, 77.82916666666665151 ) ) ;
#14537=EDGE_CURVE ( 'NONE', #6061, #44704, #17624, .T. ) ;
#14545=CARTESIAN_POINT ( 'NONE',  ( -93.67499999999998295, -212.2949673200287179, 83.22666666666665947 ) ) ;
#14546=CARTESIAN_POINT ( 'NONE',  ( -94.99999999999997158, -207.3369185715606307, 83.92781250086716227 ) ) ;
#14556=CARTESIAN_POINT ( 'NONE',  ( 96.15314808468748708, 88.00268892867053694, 77.78947916753381264 ) ) ;
#14567=CARTESIAN_POINT ( 'NONE',  ( -97.30629616937501680, 91.33154071421968467, 83.23989583420048177 ) ) ;
#14572=EDGE_CURVE ( 'NONE', #1262, #9715, #20482, .T. ) ;
#14578=CARTESIAN_POINT ( 'NONE',  ( -92.35000000000674447, -209.9999940177768565, 82.14187520865739600 ) ) ;
#14581=CARTESIAN_POINT ( 'NONE',  ( 95.00000000000000000, -207.3369185715606307, 79.48281250086715488 ) ) ;
#14582=EDGE_CURVE ( 'NONE', #23968, #9432, #71831, .T. ) ;
#14590=EDGE_LOOP ( 'NONE', ( #44751, #44787, #46509, #57175 ) ) ;
#14591=CARTESIAN_POINT ( 'NONE',  ( 93.84685191531249870, -208.0026889286704943, 75.09072916753380866 ) ) ;
#14594=VERTEX_POINT ( 'NONE', #15355 ) ;
#14604=CARTESIAN_POINT ( 'NONE',  ( 97.64999999999997726, -211.5299782133524502, 79.54895833506762415 ) ) ;
#14605=CARTESIAN_POINT ( 'NONE',  ( 97.64999999999999147, 90.00000000000002842, 84.60249999999999204 ) ) ;
#14612=VERTEX_POINT ( 'NONE', #73243 ) ;
#14614=CARTESIAN_POINT ( 'NONE',  ( -95.00000000000002842, 87.33691857156074434, 88.05531250086714579 ) ) ;
#14615=CARTESIAN_POINT ( 'NONE',  ( 92.69370383062498320, 88.66845928578037217, 83.34572916753380412 ) ) ;
#14617=CARTESIAN_POINT ( 'NONE',  ( 92.34999999999999432, 91.52997821335252127, 82.40645833506762585 ) ) ;
#14620=CARTESIAN_POINT ( 'NONE',  ( 96.32499999999998863, -207.7050326799711968, 87.32770833506762642 ) ) ;
#14629=CARTESIAN_POINT ( 'NONE',  ( -93.67500000000003979, 87.70503267997129626, 85.76666666666665151 ) ) ;
#14632=CARTESIAN_POINT ( 'NONE',  ( 92.34999999999999432, 91.52997821335252127, 88.12145833506762926 ) ) ;
#14634=DIRECTION ( 'NONE',  ( 1.000000000000000000, 0.000000000000000000, 0.000000000000000000 ) ) ;
#14635=CARTESIAN_POINT ( 'NONE',  ( -96.15314808468747287, -208.0026889286704943, 80.01197916753380923 ) ) ;
#14639=CARTESIAN_POINT ( 'NONE',  ( 95.00000000000000000, -209.9999999999999716, 90.00000000000000000 ) ) ;
#14643=CARTESIAN_POINT ( 'NONE',  ( 92.69370383062498320, 90.00000000000002842, 87.10281250086714522 ) ) ;
#14652=( GEOMETRIC_REPRESENTATION_CONTEXT ( 3 ) GLOBAL_UNCERTAINTY_ASSIGNED_CONTEXT ( ( #48865 ) ) GLOBAL_UNIT_ASSIGNED_CONTEXT ( ( #23668, #47342, #18755 ) ) REPRESENTATION_CONTEXT ( 'NONE', 'WORKASPACE' ) );
#14654=CARTESIAN_POINT ( 'NONE',  ( 2.500000000000032419, 80.00000000000000000, -279.9999999999999432 ) ) ;
#14655=CARTESIAN_POINT ( 'NONE',  ( 92.69370383062498320, 90.00000000000002842, 89.80156250086714920 ) ) ;
#14656=CARTESIAN_POINT ( 'NONE',  ( 95.39412261730194587, 87.35656277621939125, 75.00000000000001421 ) ) ;
#14659=CARTESIAN_POINT ( 'NONE',  ( -96.32499999999996021, -212.2949673200287179, 87.56583333333333030 ) ) ;
#14663=DIRECTION ( 'NONE',  ( -0.000000000000000000, -0.000000000000000000, 1.000000000000000000 ) ) ;
#14665=ORIENTED_EDGE ( 'NONE', *, *, #30383, .F. ) ;
#14668=CARTESIAN_POINT ( 'NONE',  ( 93.67500000000001137, -207.7050326799711968, 81.71854166840095957 ) ) ;
#14674=ORIENTED_EDGE ( 'NONE', *, *, #2678, .F. ) ;
#14678=CARTESIAN_POINT ( 'NONE',  ( 92.69370383062501162, -209.9999999999999716, 80.11781250086713158 ) ) ;
#14679=CARTESIAN_POINT ( 'NONE',  ( 93.84685191531251292, -211.9973110713294489, 84.82739583420048746 ) ) ;
#14682=CARTESIAN_POINT ( 'NONE',  ( 93.84685191531249870, -208.0026889286704943, 85.88572916753381037 ) ) ;
#14686=CARTESIAN_POINT ( 'NONE',  ( -93.84685191531252713, 88.00268892867056536, 76.67822916753381435 ) ) ;
#14688=VERTEX_POINT ( 'NONE', #27762 ) ;
#14690=ORIENTED_EDGE ( 'NONE', *, *, #1742, .F. ) ;
#14691=DIRECTION ( 'NONE',  ( -1.000000000000000000, -0.000000000000000000, -0.000000000000000000 ) ) ;
#14695=DIRECTION ( 'NONE',  ( 1.000000000000000000, 0.000000000000000000, 0.000000000000000000 ) ) ;
#14700=ORIENTED_EDGE ( 'NONE', *, *, #21617, .F. ) ;
#14703=CARTESIAN_POINT ( 'NONE',  ( 95.00000000000000000, -207.3369185715606307, 78.68906250086713783 ) ) ;
#14709=CARTESIAN_POINT ( 'NONE',  ( -92.35000000000003695, 90.00000000000004263, 80.79249999999998977 ) ) ;
#14711=CARTESIAN_POINT ( 'NONE',  ( -92.34999999999999432, -209.9999999999999716, 84.60249999999999204 ) ) ;
#14713=CARTESIAN_POINT ( 'NONE',  ( -96.15314808468752972, 91.99731107132950569, 78.90072916753382515 ) ) ;
#14716=CARTESIAN_POINT ( 'NONE',  ( 92.69370383062498320, 88.66845928578037217, 78.26572916753380582 ) ) ;
#14721=CARTESIAN_POINT ( 'NONE',  ( 96.90829729882861443, 88.16127723153182671, 74.99954709728268654 ) ) ;
#14724=CARTESIAN_POINT ( 'NONE',  ( -97.30629616937497417, -211.3315407142195852, 82.71072916753378479 ) ) ;
#14727=AXIS2_PLACEMENT_3D ( 'NONE', #26104, #49037, #13350 ) ;
#14735=CARTESIAN_POINT ( 'NONE',  ( -95.00000000000002842, 92.66308142843932671, 86.30906250086715659 ) ) ;
#14741=CARTESIAN_POINT ( 'NONE',  ( -94.99999999999997158, -213.0599564267049857, 85.15812500173429100 ) ) ;
#14746=CARTESIAN_POINT ( 'NONE',  ( 94.99999999999998579, 90.00000000000002842, 90.00000000000000000 ) ) ;
#14747=CARTESIAN_POINT ( 'NONE',  ( -94.99999999999997158, -212.6630814284392557, 82.34031250086714238 ) ) ;
#14751=CARTESIAN_POINT ( 'NONE',  ( 96.32499999999998863, 87.70503267997126784, 76.32104166840096582 ) ) ;
#14752=( BOUNDED_CURVE ( )  B_SPLINE_CURVE ( 2, ( #20008, #42966, #14381, #63982, #22644, #12093, #11710 ),
 .UNSPECIFIED., .F., .F. ) 
 B_SPLINE_CURVE_WITH_KNOTS ( ( 3, 2, 2, 3 ),
 ( 0.4656806970056963091, 0.4727362912391187555, 0.4797920567800010860, 0.4868478063929145838 ),
 .UNSPECIFIED. ) 
 CURVE ( )  GEOMETRIC_REPRESENTATION_ITEM ( )  RATIONAL_B_SPLINE_CURVE ( ( 0.9999934945994379820, 0.8660286565636942102, 1.000000000000000000, 0.8660254037844387076, 1.000000000000000000, 0.8660254037844387076, 1.000000000000000000 ) ) 
 REPRESENTATION_ITEM ( '' )  );
#14755=CARTESIAN_POINT ( 'NONE',  ( -97.65000000000001990, 90.00000000000004263, 88.73000000000000398 ) ) ;
#14759=CARTESIAN_POINT ( 'NONE',  ( 92.35000000030105127, 90.00002455906435728, 87.53856274002153270 ) ) ;
#14761=CARTESIAN_POINT ( 'NONE',  ( 92.35000000000003695, -208.4700217866474929, 79.78708333333331382 ) ) ;
#14765=CARTESIAN_POINT ( 'NONE',  ( -95.00000000000002842, 93.05995642670504253, 75.95062500173428077 ) ) ;
#14768=ORIENTED_EDGE ( 'NONE', *, *, #71339, .F. ) ;
#14780=ORIENTED_EDGE ( 'NONE', *, *, #56544, .F. ) ;
#14787=CARTESIAN_POINT ( 'NONE',  ( 92.69370383062498320, 88.66845928578037217, 76.51947916753381662 ) ) ;
#14794=CARTESIAN_POINT ( 'NONE',  ( 94.99999999999998579, 92.66308142843935514, 89.48406250086713953 ) ) ;
#14796=CARTESIAN_POINT ( 'NONE',  ( 92.69370383062501162, -208.6684592857803011, 89.58989583420047609 ) ) ;
#14798=CARTESIAN_POINT ( 'NONE',  ( 97.64999999999992042, 91.52997821335256390, 84.02041666666666231 ) ) ;
#14799=CARTESIAN_POINT ( 'NONE',  ( -96.73564493164514033, 91.73956328105568048, 74.87701898318914573 ) ) ;
#14800=CARTESIAN_POINT ( 'NONE',  ( 97.65000000000000568, 91.52997821335252127, 77.74979166840097378 ) ) ;
#14801=CARTESIAN_POINT ( 'NONE',  ( 0.000000000000000000, 0.000000000000000000, -80.00000000000000000 ) ) ;
#14802=CARTESIAN_POINT ( 'NONE',  ( -92.35000000000003695, 90.00000000000004263, 78.25249999999999773 ) ) ;
#14804=CARTESIAN_POINT ( 'NONE',  ( -97.64999999999994884, -211.5299782133524502, 76.16229166840095388 ) ) ;
#14805=CARTESIAN_POINT ( 'NONE',  ( -95.00000000000002842, 92.66308142843932671, 89.64281250086715147 ) ) ;
#14809=CARTESIAN_POINT ( 'NONE',  ( 94.99999999999998579, 92.66308142843935514, 89.48406250086713953 ) ) ;
#14810=CARTESIAN_POINT ( 'NONE',  ( -95.00000000000002842, 87.33691857156074434, 89.16656250086712987 ) ) ;
#14812=CARTESIAN_POINT ( 'NONE',  ( 93.84685191531248449, 91.99731107132950569, 78.26572916753382003 ) ) ;
#14815=CARTESIAN_POINT ( 'NONE',  ( 96.32499999999997442, 92.29496732002878900, 82.24770833506762813 ) ) ;
#14823=CARTESIAN_POINT ( 'NONE',  ( -92.35000000000005116, 91.52997821335253548, 81.48041666666665606 ) ) ;
#14832=CARTESIAN_POINT ( 'NONE',  ( -96.15314808468751551, 88.00268892867056536, 82.12864583420046927 ) ) ;
#14844=CARTESIAN_POINT ( 'NONE',  ( -93.67499999999998295, -207.7050326799711968, 87.24833333333333485 ) ) ;
#14849=CARTESIAN_POINT ( 'NONE',  ( 97.30629616937498838, 88.66845928578035796, 79.27114583420048177 ) ) ;
#14851=CARTESIAN_POINT ( 'NONE',  ( -97.30629616937495996, -209.9999999999999716, 83.45156250086715488 ) ) ;
#14856=CARTESIAN_POINT ( 'NONE',  ( -93.67499999999998295, -212.2949673200287179, 76.87666666666666515 ) ) ;
#14858=CARTESIAN_POINT ( 'NONE',  ( 92.69370383062501162, -209.9999999999999716, 82.65781250086713783 ) ) ;
#14861=CARTESIAN_POINT ( 'NONE',  ( 96.76339072695074606, 88.50623689698961982, 74.79348190356851944 ) ) ;
#14867=DIRECTION ( 'NONE',  ( -0.000000000000000000, -0.000000000000000000, 1.000000000000000000 ) ) ;
#14869=ADVANCED_FACE ( 'NONE', ( #51806 ), #24710, .F. ) ;
#14872=CARTESIAN_POINT ( 'NONE',  ( 96.15314808468750130, -211.9973110713294489, 78.58322916753382970 ) ) ;
#14878=CARTESIAN_POINT ( 'NONE',  ( 97.30629616937498838, 91.33154071421968467, 85.72697916753381264 ) ) ;
#14881=CARTESIAN_POINT ( 'NONE',  ( 92.35000000000002274, -211.5299782133524502, 79.89291666666666458 ) ) ;
#14890=CARTESIAN_POINT ( 'NONE',  ( -96.15314808468751551, 88.00268892867056536, 85.46239583420047836 ) ) ;
#14896=CARTESIAN_POINT ( 'NONE',  ( -96.32499999999996021, -212.2949673200287179, 87.01020833506763097 ) ) ;
#14900=CARTESIAN_POINT ( 'NONE',  ( -92.35000000000005116, 91.52997821335253548, 84.09979166840095388 ) ) ;
#14902=CARTESIAN_POINT ( 'NONE',  ( 96.15314808468748708, 91.99731107132950569, 87.04989583420048405 ) ) ;
#14914=DIRECTION ( 'NONE',  ( 1.000000000000000000, 0.000000000000000000, 0.000000000000000000 ) ) ;
#14918=CARTESIAN_POINT ( 'NONE',  ( -93.84685191531247028, -211.9973110713294489, 83.66322916753382799 ) ) ;
#14920=CYLINDRICAL_SURFACE ( 'NONE', #27315, 2.649999999999985700 ) ;
#14928=CARTESIAN_POINT ( 'NONE',  ( 96.15314808468748708, 88.00268892867053694, 78.42447916753381776 ) ) ;
#14943=CARTESIAN_POINT ( 'NONE',  ( -95.00000000000002842, 92.66308142843932671, 82.49906250086715431 ) ) ;
#14950=AXIS2_PLACEMENT_3D ( 'NONE', #37167, #31871, #43919 ) ;
#14954=FACE_BOUND ( 'NONE', #27008, .T. ) ;
#14959=CARTESIAN_POINT ( 'NONE',  ( 96.15314808468750130, -211.9973110713294489, 77.94822916753382458 ) ) ;
#14960=ORIENTED_EDGE ( 'NONE', *, *, #24447, .F. ) ;
#14964=( BOUNDED_CURVE ( )  B_SPLINE_CURVE ( 2, ( #59245, #1031, #1770, #46864, #58495, #24657, #6991 ),
 .UNSPECIFIED., .F., .F. ) 
 B_SPLINE_CURVE_WITH_KNOTS ( ( 3, 2, 2, 3 ),
 ( 0.5416666666666665186, 0.5486111111111110494, 0.5555555555555553582, 0.5624999999999997780 ),
 .UNSPECIFIED. ) 
 CURVE ( )  GEOMETRIC_REPRESENTATION_ITEM ( )  RATIONAL_B_SPLINE_CURVE ( ( 1.000000000000002220, 0.8660254037844365982, 1.000000000000000000, 0.8660254037844387076, 1.000000000000000000, 0.8660254037844430375, 0.9999999999999956701 ) ) 
 REPRESENTATION_ITEM ( '' )  );
#14965=DIRECTION ( 'NONE',  ( 1.000000000000000000, 0.000000000000000000, 0.000000000000000000 ) ) ;
#14967=CARTESIAN_POINT ( 'NONE',  ( 97.30629616937498838, -209.9999999999999716, 74.87906250086714977 ) ) ;
#14968=VERTEX_POINT ( 'NONE', #52920 ) ;
#14970=VERTEX_POINT ( 'NONE', #58548 ) ;
#14971=ORIENTED_EDGE ( 'NONE', *, *, #6722, .T. ) ;
#14973=CARTESIAN_POINT ( 'NONE',  ( -92.35000000000002274, 89.99997826787523536, 89.12687425009508502 ) ) ;
#14976=CARTESIAN_POINT ( 'NONE',  ( 97.64999999999999147, -209.9999999999999716, 78.96687500173429441 ) ) ;
#14977=CARTESIAN_POINT ( 'NONE',  ( 92.34999999999999432, 88.47002178664753558, 86.87791666666664980 ) ) ;
#14980=CARTESIAN_POINT ( 'NONE',  ( 97.64999999999999147, 89.99999997928482287, 80.87187500099604165 ) ) ;
#14983=CARTESIAN_POINT ( 'NONE',  ( -95.00000000000002842, 87.33691857156074434, 84.24531250086717193 ) ) ;
#14985=CARTESIAN_POINT ( 'NONE',  ( 92.69370383062498320, 90.00000000000002842, 82.02281250086714692 ) ) ;
#14986=VERTEX_POINT ( 'NONE', #31079 ) ;
#14995=CYLINDRICAL_SURFACE ( 'NONE', #62363, 2.649999999999999467 ) ;
#14999=CARTESIAN_POINT ( 'NONE',  ( -92.69370383062498320, -209.9999999999999716, 79.80031250086713612 ) ) ;
#15004=DIRECTION ( 'NONE',  ( -0.000000000000000000, -0.000000000000000000, 1.000000000000000000 ) ) ;
#15011=CARTESIAN_POINT ( 'NONE',  ( 94.99999999999998579, 92.66308142843932671, 89.48406250086713953 ) ) ;
#15013=CARTESIAN_POINT ( 'NONE',  ( 97.64999999999999147, 90.00000000000002842, 88.41249999999999432 ) ) ;
#15014=CARTESIAN_POINT ( 'NONE',  ( -95.00000000000002842, 93.05995642670504253, 88.65062500173428361 ) ) ;
#15026=CARTESIAN_POINT ( 'NONE',  ( -92.34999999999999432, -211.5299782133524502, 87.08958333333333712 ) ) ;
#15028=CARTESIAN_POINT ( 'NONE',  ( -93.09170270117147084, 88.16127723153179829, 74.99954709728268654 ) ) ;
#15030=ORIENTED_EDGE ( 'NONE', *, *, #43066, .F. ) ;
#15031=VECTOR ( 'NONE', #18615, 1000.000000000000000 ) ;
#15039=EDGE_CURVE ( 'NONE', #24219, #60230, #24849, .T. ) ;
#15046=CARTESIAN_POINT ( 'NONE',  ( 95.00000000000000000, -212.6630814284392557, 81.54656250086713953 ) ) ;
#15047=CARTESIAN_POINT ( 'NONE',  ( 92.69370383062501162, -211.3315407142195852, 86.67947916753382742 ) ) ;
#15050=CARTESIAN_POINT ( 'NONE',  ( 92.69370383062501162, -211.3315407142195852, 86.67947916753382742 ) ) ;
#15054=CARTESIAN_POINT ( 'NONE',  ( -93.84685191531254134, 91.99731107132950569, 78.79489583420048859 ) ) ;
#15057=ORIENTED_EDGE ( 'NONE', *, *, #40338, .F. ) ;
#15059=ORIENTED_EDGE ( 'NONE', *, *, #14413, .T. ) ;
#15066=ORIENTED_EDGE ( 'NONE', *, *, #30282, .F. ) ;
#15067=EDGE_CURVE ( 'NONE', #44704, #36890, #35832, .T. ) ;
#15079=ADVANCED_FACE ( 'NONE', ( #61158 ), #61899, .F. ) ;
#15080=CARTESIAN_POINT ( 'NONE',  ( -93.84685191531254134, 91.99731107132950569, 79.42989583420049371 ) ) ;
#15082=CARTESIAN_POINT ( 'NONE',  ( 97.30629616937498838, 91.33154071421968467, 79.21822916753380639 ) ) ;
#15085=CARTESIAN_POINT ( 'NONE',  ( -92.69370383062498320, -211.3315407142195852, 88.63739583420047552 ) ) ;
#15087=VECTOR ( 'NONE', #67899, 1000.000000000000000 ) ;
#15089=CARTESIAN_POINT ( 'NONE',  ( 94.99999999999998579, 90.00000000000002842, 90.00000000000000000 ) ) ;
#15090=CARTESIAN_POINT ( 'NONE',  ( -92.69370383062498320, -209.9999999999999716, 80.43531250086714124 ) ) ;
#15094=VECTOR ( 'NONE', #17849, 1000.000000000000000 ) ;
#15103=CARTESIAN_POINT ( 'NONE',  ( -97.30629616937501680, 88.66845928578038638, 85.25072916753379104 ) ) ;
#15106=AXIS2_PLACEMENT_3D ( 'NONE', #68572, #50518, #10669 ) ;
#15113=CARTESIAN_POINT ( 'NONE',  ( 92.35000000049295465, 89.99996796756887818, 85.63541623677173220 ) ) ;
#15117=CARTESIAN_POINT ( 'NONE',  ( -93.84685191531248449, -208.0026889286704943, 83.87489583420048689 ) ) ;
#15126=CARTESIAN_POINT ( 'NONE',  ( 93.67499999999998295, 92.29496732002878900, 77.27354166840096639 ) ) ;
#15131=CARTESIAN_POINT ( 'NONE',  ( 97.64999999999999147, 90.00000000000002842, 78.25249999999999773 ) ) ;
#15135=CARTESIAN_POINT ( 'NONE',  ( -93.67500000000003979, 92.29496732002878900, 77.72333333333332916 ) ) ;
#15151=VECTOR ( 'NONE', #4966, 1000.000000000000000 ) ;
#15154=CARTESIAN_POINT ( 'NONE',  ( 97.30629616937498838, 91.33154071421968467, 76.83697916753382628 ) ) ;
#15155=CARTESIAN_POINT ( 'NONE',  ( 95.00000000000000000, -209.9999999999999716, 90.00000000000000000 ) ) ;
#15156=DIRECTION ( 'NONE',  ( -1.000000000000000000, 0.000000000000000000, 0.000000000000000000 ) ) ;
#15162=CARTESIAN_POINT ( 'NONE',  ( 93.84685191531249870, -208.0026889286704943, 87.63197916753379957 ) ) ;
#15166=CARTESIAN_POINT ( 'NONE',  ( -92.34999999999996589, -208.4700217866474645, 80.21041666666666003 ) ) ;
#15172=CARTESIAN_POINT ( 'NONE',  ( -94.99999999999997158, -213.0599564267049857, 74.99812500173430863 ) ) ;
#15173=ADVANCED_FACE ( 'NONE', ( #11129 ), #40435, .F. ) ;
#15177=CARTESIAN_POINT ( 'NONE',  ( 97.30629616937498838, 90.00000000000002842, 86.15031250086714465 ) ) ;
#15178=CARTESIAN_POINT ( 'NONE',  ( -95.00000000000002842, 87.33691857156074434, 86.62656250086715204 ) ) ;
#15181=CARTESIAN_POINT ( 'NONE',  ( -97.64999999990722301, -209.9999861897314304, 80.55392363651652943 ) ) ;
#15184=CARTESIAN_POINT ( 'NONE',  ( -92.69370383062498320, -208.6684592857803295, 88.74322916753382628 ) ) ;
#15192=CARTESIAN_POINT ( 'NONE',  ( -97.65000000000001990, 90.00000000000004263, 79.83999999999998920 ) ) ;
#15194=DIRECTION ( 'NONE',  ( -0.000000000000000000, -0.000000000000000000, 1.000000000000000000 ) ) ;
#15196=CARTESIAN_POINT ( 'NONE',  ( 97.64997150697683992, 91.52999466380714466, 87.27479280632991276 ) ) ;
#15199=( BOUNDED_CURVE ( )  B_SPLINE_CURVE ( 2, ( #61175, #72431, #21291, #26940, #66443, #73176, #15677, #55149, #31474, #20934, #49868 ),
 .UNSPECIFIED., .F., .F. ) 
 B_SPLINE_CURVE_WITH_KNOTS ( ( 3, 2, 2, 2, 2, 3 ),
 ( 0.4233457466685775494, 0.4233459324529422196, 0.4304016979938244392, 0.4374574635347067142, 0.4445132290755889337, 0.4445132602971393343 ),
 .UNSPECIFIED. ) 
 CURVE ( )  GEOMETRIC_REPRESENTATION_ITEM ( )  RATIONAL_B_SPLINE_CURVE ( ( 0.9999929448534778942, 0.9999964723338524708, 1.000000000000000000, 0.8660254037844387076, 1.000000000000000000, 0.8660254037844387076, 1.000000000000000000, 0.8660254037844387076, 1.000000000000000000, 0.9999994071664397577, 0.9999988143381259853 ) ) 
 REPRESENTATION_ITEM ( '' )  );
#15200=EDGE_CURVE ( 'NONE', #44494, #74057, #46086, .T. ) ;
#15203=CARTESIAN_POINT ( 'NONE',  ( -97.30629616937501680, 90.00000000000004263, 82.65781250086713783 ) ) ;
#15216=EDGE_CURVE ( 'NONE', #9077, #20714, #28785, .T. ) ;
#15219=CARTESIAN_POINT ( 'NONE',  ( 93.84685191531248449, 88.00268892867053694, 80.38239583420048007 ) ) ;
#15220=CARTESIAN_POINT ( 'NONE',  ( -96.15314808468747287, -208.0026889286704943, 82.07572916753382231 ) ) ;
#15224=CARTESIAN_POINT ( 'NONE',  ( -96.32499999999996021, -212.2949673200287179, 78.04083333333333883 ) ) ;
#15227=CARTESIAN_POINT ( 'NONE',  ( -92.69370383062504004, 90.00000000000004263, 78.68906250086715204 ) ) ;
#15228=CARTESIAN_POINT ( 'NONE',  ( 92.69370383062501162, -208.6684592857803011, 83.23989583420046756 ) ) ;
#15235=CARTESIAN_POINT ( 'NONE',  ( -97.64999999992180335, 90.00001303125199570, 79.28395951162846700 ) ) ;
#15238=CARTESIAN_POINT ( 'NONE',  ( 96.15314808468750130, -211.9973110713294489, 79.21822916753382060 ) ) ;
#15241=CARTESIAN_POINT ( 'NONE',  ( -93.67500000000003979, 92.29496732002878900, 76.53270833506762472 ) ) ;
#15243=CARTESIAN_POINT ( 'NONE',  ( -96.25799313133936153, 87.71227518788532507, 74.97309184317512631 ) ) ;
#15244=CARTESIAN_POINT ( 'NONE',  ( 92.69370383062498320, 90.00000000000002842, 85.35656250086715602 ) ) ;
#15246=CARTESIAN_POINT ( 'NONE',  ( 95.04693102382854875, 87.35041560265749183, 75.00000002508419072 ) ) ;
#15247=CARTESIAN_POINT ( 'NONE',  ( 92.35000000000000853, -209.9999999999999716, 83.01499999999998636 ) ) ;
#15254=CARTESIAN_POINT ( 'NONE',  ( 92.34999999999998010, -208.4700217866475214, 89.31208333333333371 ) ) ;
#15255=EDGE_CURVE ( 'NONE', #71243, #23688, #45955, .T. ) ;
#15256=CARTESIAN_POINT ( 'NONE',  ( -97.64999999999990621, -208.4700217866474077, 85.50208333333331723 ) ) ;
#15257=VECTOR ( 'NONE', #30806, 1000.000000000000000 ) ;
#15258=CARTESIAN_POINT ( 'NONE',  ( -93.67500000000003979, 87.70503267997129626, 82.03604166840096923 ) ) ;
#15261=EDGE_CURVE ( 'NONE', #5579, #49448, #25309, .T. ) ;
#15265=CARTESIAN_POINT ( 'NONE',  ( -96.32499999999996021, -207.7050326799711968, 86.79854166840097207 ) ) ;
#15269=CARTESIAN_POINT ( 'NONE',  ( -97.65000000000001990, 90.00000000000004263, 81.82437500173429612 ) ) ;
#15271=CARTESIAN_POINT ( 'NONE',  ( 96.15314808468748708, 91.99731107132950569, 83.87489583420048689 ) ) ;
#15273=CARTESIAN_POINT ( 'NONE',  ( -92.75110981005069277, 89.40965860031441537, 74.79348190356854786 ) ) ;
#15279=CARTESIAN_POINT ( 'NONE',  ( -95.00000000000002842, 90.00000000000004263, 90.00000000000000000 ) ) ;
#15281=VERTEX_POINT ( 'NONE', #55738 ) ;
#15286=CARTESIAN_POINT ( 'NONE',  ( -97.30629616937497417, -211.3315407142195852, 83.50447916753383026 ) ) ;
#15289=EDGE_CURVE ( 'NONE', #42474, #69810, #70502, .T. ) ;
#15291=DIRECTION ( 'NONE',  ( 1.000000000000000000, 0.000000000000000000, 0.000000000000000000 ) ) ;
#15295=CARTESIAN_POINT ( 'NONE',  ( 97.30629616937498838, 90.00000000000002842, 79.80031250086713612 ) ) ;
#15301=CARTESIAN_POINT ( 'NONE',  ( -96.32499999999996021, -212.2949673200287179, 86.93083333333332519 ) ) ;
#15302=EDGE_CURVE ( 'NONE', #5092, #52184, #58023, .T. ) ;
#15305=ADVANCED_FACE ( 'NONE', ( #38075 ), #38451, .T. ) ;
#15306=CARTESIAN_POINT ( 'NONE',  ( 92.34999999999999432, 88.47002178664752137, 76.79729166840095900 ) ) ;
#15308=CARTESIAN_POINT ( 'NONE',  ( -93.84685191531252713, 88.00268892867056536, 83.50447916753381605 ) ) ;
#15310=VECTOR ( 'NONE', #21373, 1000.000000000000000 ) ;
#15314=DIRECTION ( 'NONE',  ( -0.000000000000000000, -0.000000000000000000, 1.000000000000000000 ) ) ;
#15318=CARTESIAN_POINT ( 'NONE',  ( 92.69370383062501162, -209.9999999999999716, 78.37156250086715659 ) ) ;
#15321=VECTOR ( 'NONE', #26758, 1000.000000000000000 ) ;
#15327=CARTESIAN_POINT ( 'NONE',  ( 92.69370383062501162, -211.3315407142195852, 75.24947916753383481 ) ) ;
#15338=CARTESIAN_POINT ( 'NONE',  ( 97.64999999999997726, -208.4700217866474645, 81.55979166840097605 ) ) ;
#15340=CARTESIAN_POINT ( 'NONE',  ( 97.64999999999997726, 88.47002178664753558, 82.64458333333331552 ) ) ;
#15345=ORIENTED_EDGE ( 'NONE', *, *, #37718, .T. ) ;
#15347=CARTESIAN_POINT ( 'NONE',  ( -97.30629616937501680, 88.66845928578038638, 86.04447916753382231 ) ) ;
#15349=CARTESIAN_POINT ( 'NONE',  ( 96.15314808468748708, 91.99731107132950569, 81.17614583420048291 ) ) ;
#15355=CARTESIAN_POINT ( 'NONE',  ( 23.49955575014745435, 0.001194404164629722436, -80.00000000000000000 ) ) ;
#15364=CARTESIAN_POINT ( 'NONE',  ( 97.64999999999999147, 90.00000000000002842, 87.85687500173429498 ) ) ;
#15367=CARTESIAN_POINT ( 'NONE',  ( -97.30629616937495996, -209.9999999999999716, 80.75281250086715090 ) ) ;
#15376=B_SPLINE_CURVE_WITH_KNOTS ( 'NONE', 3,
 ( #70445, #65210, #59566, #53548, #41899, #25352, #30240, #60679, #53180, #64840, #71936, #8051, #24603, #36996, #65955, #14799, #70826, #60319, #13321, #25713, #47906, #43404, #30972, #20450 ),
 .UNSPECIFIED., .F., .F.,
 ( 4, 2, 2, 2, 2, 2, 2, 2, 2, 2, 2, 4 ),
 ( -0.009991285186810493213, -0.009254074022779614286, -0.008516862858748735360, -0.007779651694717856433, -0.007411046112702417837, -0.007042440530686980109, -0.006673834948671541513, -0.006305229366656103784, -0.005568018202625168479, -0.004830807038594233174, -0.004462201456578745139, -0.004093595874563257103 ),
 .UNSPECIFIED. ) ;
#15379=CARTESIAN_POINT ( 'NONE',  ( 97.30629616937498838, 90.00000000000002842, 88.05531250086713158 ) ) ;
#15384=DIRECTION ( 'NONE',  ( -4.476705744456276711E-17, 1.000000000000000000, -0.000000000000000000 ) ) ;
#15387=CARTESIAN_POINT ( 'NONE',  ( -92.35000000000003695, 89.99999990163421160, 80.23687499810812085 ) ) ;
#15388=CARTESIAN_POINT ( 'NONE',  ( -97.65000000000001990, 90.00000000000004263, 87.53937500173429953 ) ) ;
#15395=CARTESIAN_POINT ( 'NONE',  ( -96.32499999999996021, -207.7050326799711968, 85.44916666666665606 ) ) ;
#15397=( BOUNDED_CURVE ( )  B_SPLINE_CURVE ( 2, ( #69528, #42808, #2253, #65738, #19128, #59359, #60117 ),
 .UNSPECIFIED., .F., .F. ) 
 B_SPLINE_CURVE_WITH_KNOTS ( ( 3, 2, 2, 3 ),
 ( 0.6875000000000000000, 0.6944444444444443088, 0.7013888888888887285, 0.7083333333333331483 ),
 .UNSPECIFIED. ) 
 CURVE ( )  GEOMETRIC_REPRESENTATION_ITEM ( )  RATIONAL_B_SPLINE_CURVE ( ( 1.000000000000000000, 0.8660254037844387076, 1.000000000000000000, 0.8660254037844387076, 1.000000000000000000, 0.8660254037844430375, 0.9999999999999956701 ) ) 
 REPRESENTATION_ITEM ( '' )  );
#15412=CARTESIAN_POINT ( 'NONE',  ( 96.15314808468748708, -208.0026889286704943, 81.81114583420047381 ) ) ;
#15413=CARTESIAN_POINT ( 'NONE',  ( 92.69370383062501162, -209.9999999999999716, 86.62656250086715204 ) ) ;
#15415=CARTESIAN_POINT ( 'NONE',  ( 92.69370383062501162, -209.9999999999999716, 86.62656250086715204 ) ) ;
#15421=CARTESIAN_POINT ( 'NONE',  ( -92.69370383062502583, 91.33154071421968467, 78.10697916753383652 ) ) ;
#15432=EDGE_CURVE ( 'NONE', #40405, #48739, #17193, .T. ) ;
#15433=VERTEX_POINT ( 'NONE', #61576 ) ;
#15439=ORIENTED_EDGE ( 'NONE', *, *, #47267, .F. ) ;
#15442=CARTESIAN_POINT ( 'NONE',  ( 97.30629616937498838, -208.6684592857803011, 74.77322916753379900 ) ) ;
#15443=DIRECTION ( 'NONE',  ( -0.000000000000000000, -0.000000000000000000, 1.000000000000000000 ) ) ;
#15445=ORIENTED_EDGE ( 'NONE', *, *, #15719, .F. ) ;
#15448=DIRECTION ( 'NONE',  ( -0.000000000000000000, -0.000000000000000000, 1.000000000000000000 ) ) ;
#15451=CARTESIAN_POINT ( 'NONE',  ( -92.35000000000005116, 91.52997821335253548, 89.73541666666666572 ) ) ;
#15454=CARTESIAN_POINT ( 'NONE',  ( 97.30629616937498838, 90.00000000000002842, 77.89531250086714920 ) ) ;
#15457=CARTESIAN_POINT ( 'NONE',  ( -92.69370383062498320, -209.9999999999999716, 88.69031250086715090 ) ) ;
#15458=CIRCLE ( 'NONE', #3467, 2.649999999999985700 ) ;
#15459=CARTESIAN_POINT ( 'NONE',  ( 96.90829729882862864, -211.8387227684681591, 74.99954709728268654 ) ) ;
#15462=CARTESIAN_POINT ( 'NONE',  ( -97.30629616937497417, -211.3315407142195852, 78.90072916753381094 ) ) ;
#15465=CARTESIAN_POINT ( 'NONE',  ( 92.34999999999999432, 90.00000000000002842, 86.82500000000000284 ) ) ;
#15473=LINE ( 'NONE', #38415, #57684 ) ;
#15475=CARTESIAN_POINT ( 'NONE',  ( 97.64999999999999147, 90.00000000000002842, 84.60249999999999204 ) ) ;
#15476=CARTESIAN_POINT ( 'NONE',  ( 95.05423112903736182, -207.6112450486803880, 74.83591575723767164 ) ) ;
#15477=CARTESIAN_POINT ( 'NONE',  ( -96.15314808468752972, 91.99731107132950569, 80.64697916753381435 ) ) ;
#15488=CARTESIAN_POINT ( 'NONE',  ( -95.00000000000002842, 93.05995642670504253, 89.84125000000000227 ) ) ;
#15490=CARTESIAN_POINT ( 'NONE',  ( -94.99999999999997158, -207.3369185715606307, 78.84781250086714977 ) ) ;
#15512=CARTESIAN_POINT ( 'NONE',  ( -97.64996763243318867, -208.4700030992240727, 87.48645704240065868 ) ) ;
#15519=CARTESIAN_POINT ( 'NONE',  ( -96.32499999999996021, -207.7050326799711968, 84.89354166840095672 ) ) ;
#15525=AXIS2_PLACEMENT_3D ( 'NONE', #28537, #68035, #45111 ) ;
#15530=CARTESIAN_POINT ( 'NONE',  ( 93.84685191531248449, 88.00268892867053694, 77.20739583420048291 ) ) ;
#15531=DIRECTION ( 'NONE',  ( -0.000000000000000000, -0.000000000000000000, 1.000000000000000000 ) ) ;
#15538=CARTESIAN_POINT ( 'NONE',  ( 94.99999999999998579, 92.66308142843935514, 87.57906250086713840 ) ) ;
#15540=CARTESIAN_POINT ( 'NONE',  ( 97.30629616937498838, -208.6684592857803011, 84.29822916753380468 ) ) ;
#15552=CARTESIAN_POINT ( 'NONE',  ( -97.30629616937497417, -211.3315407142195852, 87.15572916753380639 ) ) ;
#15554=CARTESIAN_POINT ( 'NONE',  ( -97.30629616937501680, 90.00000000000004263, 87.26156250086715715 ) ) ;
#15555=ADVANCED_FACE ( 'NONE', ( #12279 ), #1053, .F. ) ;
#15557=CARTESIAN_POINT ( 'NONE',  ( 97.30629616937498838, 90.00000000000002842, 87.42031250086714067 ) ) ;
#15558=CARTESIAN_POINT ( 'NONE',  ( -97.30629616937501680, 91.33154071421968467, 87.04989583420048405 ) ) ;
#15562=CYLINDRICAL_SURFACE ( 'NONE', #11541, 2.649999999999985700 ) ;
#15570=CARTESIAN_POINT ( 'NONE',  ( -95.00000000000002842, 86.94004357329504273, 81.26874999999999716 ) ) ;
#15572=CARTESIAN_POINT ( 'NONE',  ( -97.64999999999994884, 88.47002178664749295, 78.62291666666668277 ) ) ;
#15576=CARTESIAN_POINT ( 'NONE',  ( -97.65000000000001990, 90.00000000000004263, 90.00000000000000000 ) ) ;
#15580=CARTESIAN_POINT ( 'NONE',  ( -92.69370383062502583, 88.66845928578038638, 80.38239583420049428 ) ) ;
#15593=CARTESIAN_POINT ( 'NONE',  ( 93.84685191531248449, 88.00268892867053694, 79.74739583420048916 ) ) ;
#15594=CARTESIAN_POINT ( 'NONE',  ( -97.30629616937497417, -208.6684592857803295, 82.12864583420048348 ) ) ;
#15599=CARTESIAN_POINT ( 'NONE',  ( -93.67499999999998295, -212.2949673200287179, 79.41666666666665719 ) ) ;
#15607=CARTESIAN_POINT ( 'NONE',  ( -96.15314808468751551, 88.00268892867056536, 77.20739583420048291 ) ) ;
#15608=CARTESIAN_POINT ( 'NONE',  ( 93.84685191531249870, -208.0026889286704943, 81.91697916753381037 ) ) ;
#15616=ADVANCED_FACE ( 'NONE', ( #29934 ), #58901, .F. ) ;
#15620=CARTESIAN_POINT ( 'NONE',  ( 92.69370383062501162, -211.3315407142195852, 75.24947916753383481 ) ) ;
#15623=( BOUNDED_CURVE ( )  B_SPLINE_CURVE ( 2, ( #29690, #24087, #68085, #11305, #57921, #39520, #62463 ),
 .UNSPECIFIED., .F., .F. ) 
 B_SPLINE_CURVE_WITH_KNOTS ( ( 3, 2, 2, 3 ),
 ( 0.9583333333333337034, 0.9652777777777781232, 0.9722222222222225430, 0.9791666666666669627 ),
 .UNSPECIFIED. ) 
 CURVE ( )  GEOMETRIC_REPRESENTATION_ITEM ( )  RATIONAL_B_SPLINE_CURVE ( ( 0.9999999999999935607, 0.8660254037844451469, 1.000000000000000000, 0.8660254037844387076, 1.000000000000000000, 0.8660254037844322683, 1.000000000000006439 ) ) 
 REPRESENTATION_ITEM ( '' )  );
#15624=CARTESIAN_POINT ( 'NONE',  ( -96.91066463018650268, 88.26122129797420257, 74.95660481729453295 ) ) ;
#15625=CARTESIAN_POINT ( 'NONE',  ( 96.15314808468748708, 88.00268892867053694, 86.83822916753382515 ) ) ;
#15627=EDGE_CURVE ( 'NONE', #423, #30489, #67676, .T. ) ;
#15629=CARTESIAN_POINT ( 'NONE',  ( 96.32499999999998863, -207.7050326799711968, 77.08833333333332405 ) ) ;
#15638=CARTESIAN_POINT ( 'NONE',  ( -97.65000000000001990, 88.47002178664754979, 81.87729166840097150 ) ) ;
#15640=DIRECTION ( 'NONE',  ( -0.000000000000000000, -0.000000000000000000, 1.000000000000000000 ) ) ;
#15642=VERTEX_POINT ( 'NONE', #30309 ) ;
#15643=CARTESIAN_POINT ( 'NONE',  ( -97.64999999999994884, -211.5299782133524502, 85.05229166840096866 ) ) ;
#15648=CARTESIAN_POINT ( 'NONE',  ( -95.00000000000002842, 93.05995642670501411, 84.20562500173429044 ) ) ;
#15649=( BOUNDED_CURVE ( )  B_SPLINE_CURVE ( 2, ( #39897, #41371, #24090 ),
 .UNSPECIFIED., .F., .F. ) 
 B_SPLINE_CURVE_WITH_KNOTS ( ( 3, 3 ),
 ( 0.000000000000000000, 2.334341054548227728E-05 ),
 .UNSPECIFIED. ) 
 CURVE ( )  GEOMETRIC_REPRESENTATION_ITEM ( )  RATIONAL_B_SPLINE_CURVE ( ( 0.9459494467533928752, 0.9464399322878992438, 0.9469490141588211563 ) ) 
 REPRESENTATION_ITEM ( '' )  );
#15652=CARTESIAN_POINT ( 'NONE',  ( 97.30629616937498838, 90.00000000000002842, 81.86406250086714920 ) ) ;
#15653=CARTESIAN_POINT ( 'NONE',  ( -94.99999999999997158, -209.9999999999999716, 90.00000000000000000 ) ) ;
#15654=CARTESIAN_POINT ( 'NONE',  ( -92.35000000002592913, -210.0000117261698165, 82.77687459617060028 ) ) ;
#15671=CARTESIAN_POINT ( 'NONE',  ( -93.84685191531247028, -211.9973110713294489, 79.85322916753381151 ) ) ;
#15677=CARTESIAN_POINT ( 'NONE',  ( 96.32499999999998863, -207.7050326799711968, 82.88270833506763324 ) ) ;
#15678=CARTESIAN_POINT ( 'NONE',  ( 94.99999999999998579, 87.33691857156068750, 77.73656250086713726 ) ) ;
#15680=DIRECTION ( 'NONE',  ( -0.000000000000000000, 0.000000000000000000, 1.000000000000000000 ) ) ;
#15681=LINE ( 'NONE', #8560, #66095 ) ;
#15682=CARTESIAN_POINT ( 'NONE',  ( 92.50303120605391882, 90.24436280099763508, 74.91343443312143791 ) ) ;
#15686=CARTESIAN_POINT ( 'NONE',  ( -97.64999999996642543, 89.99999234487438571, 78.01464417100932280 ) ) ;
#15687=ORIENTED_EDGE ( 'NONE', *, *, #59417, .F. ) ;
#15688=EDGE_CURVE ( 'NONE', #40498, #64184, #40873, .T. ) ;
#15689=CIRCLE ( 'NONE', #45703, 3.299999999999983391 ) ;
#15690=CARTESIAN_POINT ( 'NONE',  ( -92.69370383062505425, 91.33154071421968467, 83.66322916753381378 ) ) ;
#15693=CARTESIAN_POINT ( 'NONE',  ( 7.103376864691351012E-17, -120.0000000000000000, -85.59999999999999432 ) ) ;
#15697=DIRECTION ( 'NONE',  ( 1.000000000000000000, 0.000000000000000000, 0.000000000000000000 ) ) ;
#15703=CARTESIAN_POINT ( 'NONE',  ( 95.00000000000000000, -212.6630814284392557, 78.53031250086715431 ) ) ;
#15706=ORIENTED_EDGE ( 'NONE', *, *, #44819, .T. ) ;
#15707=DIRECTION ( 'NONE',  ( 1.000000000000000000, 0.000000000000000000, 0.000000000000000000 ) ) ;
#15712=EDGE_CURVE ( 'NONE', #23400, #23659, #32150, .T. ) ;
#15715=CARTESIAN_POINT ( 'NONE',  ( 95.00000000000000000, -212.6630814284392557, 75.99031250086716227 ) ) ;
#15719=EDGE_CURVE ( 'NONE', #39507, #67503, #26826, .T. ) ;
#15725=CARTESIAN_POINT ( 'NONE',  ( 92.35000000000000853, -209.9999999999999716, 79.91937500173429498 ) ) ;
#15726=CARTESIAN_POINT ( 'NONE',  ( 94.99999999999998579, 86.94004357329500010, 83.17374999999999829 ) ) ;
#15734=CARTESIAN_POINT ( 'NONE',  ( -92.69370383062504004, 90.00000000000004263, 83.76906250086716454 ) ) ;
#15735=CARTESIAN_POINT ( 'NONE',  ( 96.15314808468748708, 91.99731107132950569, 78.00114583420048575 ) ) ;
#15742=CIRCLE ( 'NONE', #3739, 26.50000000000000355 ) ;
#15743=CARTESIAN_POINT ( 'NONE',  ( -97.30629616937497417, -208.6684592857803011, 82.60489583420047666 ) ) ;
#15749=CARTESIAN_POINT ( 'NONE',  ( -97.51367041768831712, -210.0000000000000284, 74.91808492278045151 ) ) ;
#15751=CARTESIAN_POINT ( 'NONE',  ( -92.69370383062498320, -209.9999999999999716, 81.07031250086714635 ) ) ;
#15759=AXIS2_PLACEMENT_3D ( 'NONE', #24177, #62943, #57654 ) ;
#15762=CARTESIAN_POINT ( 'NONE',  ( 92.69370383062498320, 88.66845928578035796, 87.15572916753380639 ) ) ;
#15766=CARTESIAN_POINT ( 'NONE',  ( -2.499999999999970690, 73.00000000000001421, -201.6999999999999886 ) ) ;
#15777=CARTESIAN_POINT ( 'NONE',  ( -96.32499999999996021, -212.2949673200287179, 85.02583333333332405 ) ) ;
#15791=CARTESIAN_POINT ( 'NONE',  ( 95.00000000000000000, -207.3369185715606307, 87.73781250086715033 ) ) ;
#15797=EDGE_LOOP ( 'NONE', ( #31605, #58435 ) ) ;
#15799=CARTESIAN_POINT ( 'NONE',  ( 96.15314808468750130, -211.9973110713294489, 78.42447916753381776 ) ) ;
#15800=CARTESIAN_POINT ( 'NONE',  ( 96.15314808468750130, -211.9973110713294489, 85.56822916753381492 ) ) ;
#15801=ADVANCED_FACE ( 'NONE', ( #65284 ), #8868, .F. ) ;
#15803=CARTESIAN_POINT ( 'NONE',  ( 93.84685191531249870, -208.0026889286704943, 86.52072916753382970 ) ) ;
#15824=B_SPLINE_CURVE_WITH_KNOTS ( 'NONE', 3,
 ( #57636, #29042, #64014, #12489, #520, #23414 ),
 .UNSPECIFIED., .F., .F.,
 ( 4, 2, 4 ),
 ( 0.7528176110417461597, 0.8153862273023197993, 0.8779548435628933278 ),
 .UNSPECIFIED. ) ;
#15826=ORIENTED_EDGE ( 'NONE', *, *, #68832, .F. ) ;
#15829=FACE_BOUND ( 'NONE', #17372, .T. ) ;
#15833=DIRECTION ( 'NONE',  ( -0.000000000000000000, -0.000000000000000000, 1.000000000000000000 ) ) ;
#15835=CARTESIAN_POINT ( 'NONE',  ( -95.73425683495055694, 85.91408486779589282, 74.64692065633565221 ) ) ;
#15837=CARTESIAN_POINT ( 'NONE',  ( 94.99999999999998579, 87.33691857156068750, 77.10156250086711793 ) ) ;
#15842=CARTESIAN_POINT ( 'NONE',  ( 96.66135172262730180, -211.6008015735635865, 74.79754476654878204 ) ) ;
#15845=CARTESIAN_POINT ( 'NONE',  ( -93.84685191531248449, -208.0026889286704943, 79.27114583420046756 ) ) ;
#15855=CARTESIAN_POINT ( 'NONE',  ( 92.49008991410272529, -209.8784921249854563, 74.91582548749271098 ) ) ;
#15857=CARTESIAN_POINT ( 'NONE',  ( -95.00000000000002842, 87.33691857156074434, 81.54656250086715374 ) ) ;
#15861=( BOUNDED_CURVE ( )  B_SPLINE_CURVE ( 2, ( #19377, #64514, #12992, #47960, #69773, #52478, #53232 ),
 .UNSPECIFIED., .F., .F. ) 
 B_SPLINE_CURVE_WITH_KNOTS ( ( 3, 2, 2, 3 ),
 ( 0.6773535682752295228, 0.6844092574655884498, 0.6914650230064715020, 0.6985206468843488947 ),
 .UNSPECIFIED. ) 
 CURVE ( )  GEOMETRIC_REPRESENTATION_ITEM ( )  RATIONAL_B_SPLINE_CURVE ( ( 0.9999971005499255217, 0.8660268535251636202, 1.000000000000000000, 0.8660254037844387076, 1.000000000000000000, 0.8660280936759700010, 0.9999946203249505672 ) ) 
 REPRESENTATION_ITEM ( '' )  );
#15870=CARTESIAN_POINT ( 'NONE',  ( -96.15314808468747287, -208.0026889286704943, 79.53572916753381605 ) ) ;
#15877=CARTESIAN_POINT ( 'NONE',  ( -97.64999999999996305, -209.9999999999999716, 90.00000000000000000 ) ) ;
#15885=ORIENTED_EDGE ( 'NONE', *, *, #51192, .F. ) ;
#15886=CARTESIAN_POINT ( 'NONE',  ( 93.84685191531249870, -208.0026889286704943, 87.63197916753379957 ) ) ;
#15903=CARTESIAN_POINT ( 'NONE',  ( 97.30629616937498838, 88.66845928578037217, 76.09614583420048461 ) ) ;
#15908=VERTEX_POINT ( 'NONE', #61861 ) ;
#15912=CARTESIAN_POINT ( 'NONE',  ( 92.69370383062501162, -208.6684592857803011, 84.50989583420046358 ) ) ;
#15921=CARTESIAN_POINT ( 'NONE',  ( -92.69370383062498320, -209.9999999999999716, 88.69031250086715090 ) ) ;
#15922=CARTESIAN_POINT ( 'NONE',  ( -92.69370383062502583, 88.66845928578038638, 86.89114583420050053 ) ) ;
#15924=CARTESIAN_POINT ( 'NONE',  ( 97.30629616937498838, 88.66845928578037217, 89.27239583420048064 ) ) ;
#15925=CARTESIAN_POINT ( 'NONE',  ( -97.30629616937501680, 91.33154071421968467, 86.41489583420047893 ) ) ;
#15929=FACE_OUTER_BOUND ( 'NONE', #6235, .T. ) ;
#15930=CARTESIAN_POINT ( 'NONE',  ( -97.30629616937497417, -211.3315407142195852, 89.06072916753382174 ) ) ;
#15935=ORIENTED_EDGE ( 'NONE', *, *, #13651, .T. ) ;
#15936=CARTESIAN_POINT ( 'NONE',  ( -96.32500000000001705, 87.70503267997129626, 82.48583333333333201 ) ) ;
#15942=DIRECTION ( 'NONE',  ( 1.000000000000000000, 0.000000000000000000, 0.000000000000000000 ) ) ;
#15946=CARTESIAN_POINT ( 'NONE',  ( -92.69370383062504004, 90.00000000000004263, 81.07031250086714635 ) ) ;
#15949=CARTESIAN_POINT ( 'NONE',  ( 92.35000000039362078, 90.00002930319625705, 82.45844277051448046 ) ) ;
#15955=CARTESIAN_POINT ( 'NONE',  ( -96.15314808468747287, -208.0026889286704943, 89.69572916753382685 ) ) ;
#15959=CARTESIAN_POINT ( 'NONE',  ( 94.99999999999998579, 92.66308142843932671, 81.38781250086715602 ) ) ;
#15960=CARTESIAN_POINT ( 'NONE',  ( -92.69370383062498320, -211.3315407142195852, 83.71614583420048916 ) ) ;
#15964=CARTESIAN_POINT ( 'NONE',  ( -96.32499999999996021, -207.7050326799711968, 76.55916666666666970 ) ) ;
#15967=CARTESIAN_POINT ( 'NONE',  ( -92.69370383062505425, 88.66845928578038638, 78.63614583420046245 ) ) ;
#15968=CARTESIAN_POINT ( 'NONE',  ( 92.69370383062501162, -211.3315407142195852, 80.17072916753379275 ) ) ;
#15974=CARTESIAN_POINT ( 'NONE',  ( -92.35000000000177067, -209.9999969335172807, 75.79187510780353421 ) ) ;
#15976=DIRECTION ( 'NONE',  ( 1.000000000000000000, 0.000000000000000000, 0.000000000000000000 ) ) ;
#15978=ORIENTED_EDGE ( 'NONE', *, *, #68668, .T. ) ;
#15980=VERTEX_POINT ( 'NONE', #16359 ) ;
#15981=CARTESIAN_POINT ( 'NONE',  ( 97.30629616937498838, -208.6684592857803295, 74.93197916753381094 ) ) ;
#15986=CARTESIAN_POINT ( 'NONE',  ( 93.84685191531248449, 88.00268892867053694, 88.00239583420048461 ) ) ;
#15988=CARTESIAN_POINT ( 'NONE',  ( 95.00000000000000000, -206.9400435732949575, 79.04625000000000057 ) ) ;
#15989=ORIENTED_EDGE ( 'NONE', *, *, #5463, .F. ) ;
#15992=VERTEX_POINT ( 'NONE', #12472 ) ;
#15993=ORIENTED_EDGE ( 'NONE', *, *, #56987, .F. ) ;
#15996=CARTESIAN_POINT ( 'NONE',  ( 97.64999999999999147, -210.0000001051138270, 86.58687499784845443 ) ) ;
#16000=LINE ( 'NONE', #61881, #17631 ) ;
#16002=CARTESIAN_POINT ( 'NONE',  ( -92.34999999999999432, -209.9999999999999716, 82.14187500173429157 ) ) ;
#16006=CARTESIAN_POINT ( 'NONE',  ( 93.67499999999998295, 92.29496732002878900, 83.62354166840097491 ) ) ;
#16007=CARTESIAN_POINT ( 'NONE',  ( -92.35000000000005116, 88.47002178664754979, 82.72395833506762131 ) ) ;
#16010=CARTESIAN_POINT ( 'NONE',  ( 97.30629616937498838, 90.00000000000002842, 83.13406250086715943 ) ) ;
#16012=CARTESIAN_POINT ( 'NONE',  ( -97.30629616937501680, 90.00000000000004263, 89.80156250086714920 ) ) ;
#16015=CARTESIAN_POINT ( 'NONE',  ( 2.500000000000034639, 90.00000000000000000, -310.0000000000000000 ) ) ;
#16020=VECTOR ( 'NONE', #10117, 1000.000000000000000 ) ;
#16026=ORIENTED_EDGE ( 'NONE', *, *, #13151, .T. ) ;
#16032=CARTESIAN_POINT ( 'NONE',  ( -93.84685191531248449, -208.0026889286704943, 79.42989583420049371 ) ) ;
#16035=ORIENTED_EDGE ( 'NONE', *, *, #47771, .F. ) ;
#16041=CARTESIAN_POINT ( 'NONE',  ( 97.30629616937498838, 90.00000000000002842, 75.35531250086714294 ) ) ;
#16057=B_SPLINE_CURVE_WITH_KNOTS ( 'NONE', 1,
 ( #8521, #9624 ),
 .UNSPECIFIED., .F., .F.,
 ( 2, 2 ),
 ( 0.000000000000000000, 1.000000000000000000 ),
 .UNSPECIFIED. ) ;
#16058=CARTESIAN_POINT ( 'NONE',  ( -92.69370383062504004, 90.00000000000004263, 82.34031250086714238 ) ) ;
#16064=( BOUNDED_CURVE ( )  B_SPLINE_CURVE ( 2, ( #48187, #7232, #42923, #71097, #14341, #42550, #37290 ),
 .UNSPECIFIED., .F., .F. ) 
 B_SPLINE_CURVE_WITH_KNOTS ( ( 3, 2, 2, 3 ),
 ( 0.5208333333333332593, 0.5277777777777776791, 0.5347222222222220989, 0.5416666666666665186 ),
 .UNSPECIFIED. ) 
 CURVE ( )  GEOMETRIC_REPRESENTATION_ITEM ( )  RATIONAL_B_SPLINE_CURVE ( ( 1.000000000000002220, 0.8660254037844365982, 1.000000000000000000, 0.8660254037844387076, 1.000000000000000000, 0.8660254037844408170, 0.9999999999999978906 ) ) 
 REPRESENTATION_ITEM ( '' )  );
#16065=DIRECTION ( 'NONE',  ( 1.000000000000000000, 0.000000000000000000, 0.000000000000000000 ) ) ;
#16073=CARTESIAN_POINT ( 'NONE',  ( 97.30629616937498838, -211.3315407142195852, 78.63614583420049087 ) ) ;
#16075=ORIENTED_EDGE ( 'NONE', *, *, #5722, .T. ) ;
#16076=DIRECTION ( 'NONE',  ( -0.000000000000000000, -0.000000000000000000, 1.000000000000000000 ) ) ;
#16079=( BOUNDED_CURVE ( )  B_SPLINE_CURVE ( 2, ( #36917, #30525, #54223, #65874, #2754, #54947, #31639 ),
 .UNSPECIFIED., .F., .F. ) 
 B_SPLINE_CURVE_WITH_KNOTS ( ( 3, 2, 2, 3 ),
 ( 0.8541666666666666297, 0.8611111111111110494, 0.8680555555555554692, 0.8749999999999997780 ),
 .UNSPECIFIED. ) 
 CURVE ( )  GEOMETRIC_REPRESENTATION_ITEM ( )  RATIONAL_B_SPLINE_CURVE ( ( 1.000000000000000000, 0.8660254037844387076, 1.000000000000000000, 0.8660254037844387076, 1.000000000000000000, 0.8660254037844430375, 0.9999999999999956701 ) ) 
 REPRESENTATION_ITEM ( '' )  );
#16082=CARTESIAN_POINT ( 'NONE',  ( 93.67500000000001137, -212.2949673200287179, 88.20083333333332121 ) ) ;
#16091=CARTESIAN_POINT ( 'NONE',  ( -2.500000000000015543, -73.00000000000001421, -258.2999999999999545 ) ) ;
#16092=CARTESIAN_POINT ( 'NONE',  ( 97.64999999999997726, -211.5299782133524502, 81.45395833506763950 ) ) ;
#16093=CARTESIAN_POINT ( 'NONE',  ( 94.99999999999998579, 93.05995642670504253, 81.58624999999999261 ) ) ;
#16099=CARTESIAN_POINT ( 'NONE',  ( 92.35000000019411459, 89.99998015682159291, 84.36502760998348549 ) ) ;
#16100=CARTESIAN_POINT ( 'NONE',  ( -97.30629616937501680, 91.33154071421968467, 84.66864583420047552 ) ) ;
#16101=CARTESIAN_POINT ( 'NONE',  ( 97.30629616937498838, 88.66845928578037217, 79.11239583420046984 ) ) ;
#16107=CARTESIAN_POINT ( 'NONE',  ( -95.00000000000002842, 90.00000000000004263, 90.00000000000000000 ) ) ;
#16110=CARTESIAN_POINT ( 'NONE',  ( -93.84685191531247028, -211.9973110713294489, 81.59947916753381492 ) ) ;
#16114=EDGE_CURVE ( 'NONE', #68978, #5092, #14310, .T. ) ;
#16115=CARTESIAN_POINT ( 'NONE',  ( 97.64999999999999147, 90.00000000000002842, 80.15749999999999886 ) ) ;
#16119=VECTOR ( 'NONE', #54455, 1000.000000000000000 ) ;
#16122=CARTESIAN_POINT ( 'NONE',  ( -93.84685191531247028, -211.9973110713294489, 75.24947916753380639 ) ) ;
#16123=EDGE_LOOP ( 'NONE', ( #34387, #22957, #23440, #30060, #3296, #43008, #53448, #2490, #37420, #10720, #46193, #8782, #72461, #69266, #19853, #1586, #41678, #2073, #6127, #41369, #10520, #73110, #40730, #29467, #62422, #54174, #8529, #16456, #65575, #27446, #44397, #36365, #61092, #3716, #59925, #10170, #25917, #61343, #28790, #73016, #49625, #36136, #13798, #87, #24040, #70116, #700, #26355, #3164, #56324, #18943, #64218 ) ) ;
#16125=LINE ( 'NONE', #60878, #47084 ) ;
#16130=AXIS2_PLACEMENT_3D ( 'NONE', #63401, #13723, #71230 ) ;
#16134=CARTESIAN_POINT ( 'NONE',  ( 94.99999999999998579, 92.66308142843932671, 88.21406250086712930 ) ) ;
#16150=CARTESIAN_POINT ( 'NONE',  ( -96.32499999999996021, -212.2949673200287179, 84.39083333333333314 ) ) ;
#16153=ADVANCED_FACE ( 'NONE', ( #13211 ), #1613, .F. ) ;
#16159=CARTESIAN_POINT ( 'NONE',  ( 95.00000000000000000, -207.3369185715606307, 89.64281250086715147 ) ) ;
#16165=CARTESIAN_POINT ( 'NONE',  ( 95.00000000000000000, -207.3369185715606307, 78.68906250086713783 ) ) ;
#16168=CARTESIAN_POINT ( 'NONE',  ( 96.15314808468750130, -211.9973110713294489, 81.75822916753382685 ) ) ;
#16190=CARTESIAN_POINT ( 'NONE',  ( 96.15314808468748708, -208.0026889286704943, 76.09614583420047040 ) ) ;
#16199=CARTESIAN_POINT ( 'NONE',  ( -95.00000000000002842, 92.66308142843932671, 75.03781250086714749 ) ) ;
#16200=ORIENTED_EDGE ( 'NONE', *, *, #69412, .T. ) ;
#16201=CARTESIAN_POINT ( 'NONE',  ( 94.99999999999998579, 87.33691857156068750, 78.37156250086714238 ) ) ;
#16204=CARTESIAN_POINT ( 'NONE',  ( -92.69370383062498320, -208.6684592857803011, 86.20322916753382003 ) ) ;
#16209=CARTESIAN_POINT ( 'NONE',  ( -93.84685191531248449, -208.0026889286704943, 80.54114583420046358 ) ) ;
#16213=ORIENTED_EDGE ( 'NONE', *, *, #25460, .F. ) ;
#16219=CARTESIAN_POINT ( 'NONE',  ( -93.84685191531252713, 88.00268892867056536, 83.50447916753381605 ) ) ;
#16231=CARTESIAN_POINT ( 'NONE',  ( 95.00000000000000000, -213.0599564267049857, 86.42812500173430124 ) ) ;
#16234=CARTESIAN_POINT ( 'NONE',  ( -96.15314808468745866, -211.9973110713294489, 77.84239583420048803 ) ) ;
#16247=LINE ( 'NONE', #63884, #41401 ) ;
#16250=VERTEX_POINT ( 'NONE', #55657 ) ;
#16253=CARTESIAN_POINT ( 'NONE',  ( 92.69370383062501162, -209.9999999999999716, 87.10281250086714522 ) ) ;
#16257=ORIENTED_EDGE ( 'NONE', *, *, #8294, .T. ) ;
#16265=DIRECTION ( 'NONE',  ( -1.000000000000000000, 0.000000000000000000, 0.000000000000000000 ) ) ;
#16268=CARTESIAN_POINT ( 'NONE',  ( 93.84685191531248449, 88.00268892867053694, 76.57239583420049200 ) ) ;
#16277=ORIENTED_EDGE ( 'NONE', *, *, #13512, .F. ) ;
#16279=CARTESIAN_POINT ( 'NONE',  ( 97.30629616937498838, -209.9999999999999716, 85.51531250086713953 ) ) ;
#16282=ADVANCED_FACE ( 'NONE', ( #38744 ), #66578, .F. ) ;
#16283=CYLINDRICAL_SURFACE ( 'NONE', #3020, 2.649999999999985700 ) ;
#16291=CARTESIAN_POINT ( 'NONE',  ( -96.15314808468745866, -211.9973110713294489, 87.84364583420047268 ) ) ;
#16292=CARTESIAN_POINT ( 'NONE',  ( -92.69370383062502583, 91.33154071421968467, 86.99697916753382287 ) ) ;
#16295=CARTESIAN_POINT ( 'NONE',  ( 93.84685191531248449, 88.00268892867053694, 88.47864583420047779 ) ) ;
#16296=CARTESIAN_POINT ( 'NONE',  ( -97.30629616937501680, 91.33154071421968467, 85.14489583420048291 ) ) ;
#16298=( BOUNDED_CURVE ( )  B_SPLINE_CURVE ( 2, ( #67436, #33964, #45644, #22698, #57274, #56912, #68927 ),
 .UNSPECIFIED., .F., .F. ) 
 B_SPLINE_CURVE_WITH_KNOTS ( ( 3, 2, 2, 3 ),
 ( 0.5208333333333332593, 0.5277777777777776791, 0.5347222222222220989, 0.5416666666666665186 ),
 .UNSPECIFIED. ) 
 CURVE ( )  GEOMETRIC_REPRESENTATION_ITEM ( )  RATIONAL_B_SPLINE_CURVE ( ( 1.000000000000002220, 0.8660254037844365982, 1.000000000000000000, 0.8660254037844387076, 1.000000000000000000, 0.8660254037844408170, 0.9999999999999978906 ) ) 
 REPRESENTATION_ITEM ( '' )  );
#16304=LINE ( 'NONE', #16678, #38664 ) ;
#16307=CYLINDRICAL_SURFACE ( 'NONE', #27058, 2.649999999999985700 ) ;
#16314=CARTESIAN_POINT ( 'NONE',  ( -93.67500000000003979, 87.70503267997129626, 81.32166666666667254 ) ) ;
#16316=DIRECTION ( 'NONE',  ( 1.000000000000000000, 0.000000000000000000, 0.000000000000000000 ) ) ;
#16319=CARTESIAN_POINT ( 'NONE',  ( 97.64999999999994884, 88.94459177146599416, 75.04099707143591047 ) ) ;
#16320=CARTESIAN_POINT ( 'NONE',  ( -93.67499999999998295, -207.7050326799711968, 79.62833333333333030 ) ) ;
#16322=CARTESIAN_POINT ( 'NONE',  ( -93.84685191531254134, 91.99731107132950569, 83.08114583420048405 ) ) ;
#16324=ADVANCED_FACE ( 'NONE', ( #27824 ), #57896, .F. ) ;
#16325=EDGE_CURVE ( 'NONE', #52479, #35704, #50752, .T. ) ;
#16328=CARTESIAN_POINT ( 'NONE',  ( 95.00000000000000000, -209.9999999999999716, 90.00000000000000000 ) ) ;
#16330=CARTESIAN_POINT ( 'NONE',  ( -96.15314808468747287, -208.0026889286704943, 89.06072916753382174 ) ) ;
#16333=CARTESIAN_POINT ( 'NONE',  ( 97.30629616937498838, 90.00000000000002842, 81.22906250086715829 ) ) ;
#16334=CARTESIAN_POINT ( 'NONE',  ( -92.69370383062498320, -208.6684592857803295, 81.28197916753381946 ) ) ;
#16337=CARTESIAN_POINT ( 'NONE',  ( 97.65000000000000568, -208.4700217866474645, 80.92479166840097093 ) ) ;
#16343=CARTESIAN_POINT ( 'NONE',  ( -95.00000000000002842, 92.66308142843932671, 79.48281250086715488 ) ) ;
#16344=CARTESIAN_POINT ( 'NONE',  ( 96.15314808468750130, -211.9973110713294489, 79.69447916753379957 ) ) ;
#16352=CARTESIAN_POINT ( 'NONE',  ( 94.99999999999998579, 90.00000000000002842, 90.00000000000000000 ) ) ;
#16357=CARTESIAN_POINT ( 'NONE',  ( 96.66135172262728759, -211.6008015735635865, 74.79754476654878204 ) ) ;
#16358=ORIENTED_EDGE ( 'NONE', *, *, #22748, .T. ) ;
#16359=CARTESIAN_POINT ( 'NONE',  ( 92.35000000030105127, 90.00002455906435728, 87.53856274002153270 ) ) ;
#16361=CARTESIAN_POINT ( 'NONE',  ( 93.84685191531248449, 91.99731107132950569, 86.52072916753382970 ) ) ;
#16363=CARTESIAN_POINT ( 'NONE',  ( 93.67500000000001137, -207.7050326799711968, 76.55916666666666970 ) ) ;
#16375=CARTESIAN_POINT ( 'NONE',  ( -97.64999247309853558, -211.5299825590109890, 88.22729196900363036 ) ) ;
#16376=CARTESIAN_POINT ( 'NONE',  ( 96.32499999999998863, 87.70503267997126784, 83.94104166840097037 ) ) ;
#16379=CARTESIAN_POINT ( 'NONE',  ( -94.99999999999997158, -206.9400435732949575, 82.30062500173428930 ) ) ;
#16383=CARTESIAN_POINT ( 'NONE',  ( 97.64999999999997726, 88.47002178664753558, 83.99395833506763154 ) ) ;
#16384=CARTESIAN_POINT ( 'NONE',  ( -96.32500000000001705, 87.70503267997129626, 78.12020833506763040 ) ) ;
#16386=VERTEX_POINT ( 'NONE', #40598 ) ;
#16387=CARTESIAN_POINT ( 'NONE',  ( 97.30629616937498838, 90.00000000000002842, 84.40406250086715545 ) ) ;
#16389=CARTESIAN_POINT ( 'NONE',  ( -92.35000000000005116, -208.4700217866473793, 86.56041666666668277 ) ) ;
#16390=CARTESIAN_POINT ( 'NONE',  ( -96.32499999999996021, -212.2949673200287179, 82.56520833506762358 ) ) ;
#16408=CARTESIAN_POINT ( 'NONE',  ( -92.69370383062498320, -208.6684592857803011, 81.28197916753381946 ) ) ;
#16410=CARTESIAN_POINT ( 'NONE',  ( -97.30629616937501680, 88.66845928578038638, 87.79072916753381151 ) ) ;
#16412=CARTESIAN_POINT ( 'NONE',  ( -94.99999999999997158, -213.0599564267049857, 77.53812500173428646 ) ) ;
#16421=CARTESIAN_POINT ( 'NONE',  ( -94.99999999999997158, -206.9400435732949575, 79.04624999999997215 ) ) ;
#16425=CARTESIAN_POINT ( 'NONE',  ( 97.64996928176857693, -208.4700040514683224, 79.01979289519827887 ) ) ;
#16427=CARTESIAN_POINT ( 'NONE',  ( -93.84685191531247028, -211.9973110713294489, 89.37822916753381719 ) ) ;
#16429=VERTEX_POINT ( 'NONE', #33453 ) ;
#16431=CARTESIAN_POINT ( 'NONE',  ( -92.69370383062505425, 91.33154071421968467, 78.58322916753381548 ) ) ;
#16432=FACE_OUTER_BOUND ( 'NONE', #64938, .T. ) ;
#16439=CARTESIAN_POINT ( 'NONE',  ( 92.69370383062501162, -209.9999999999999716, 75.19656250086714522 ) ) ;
#16443=VECTOR ( 'NONE', #40842, 1000.000000000000000 ) ;
#16444=VERTEX_POINT ( 'NONE', #68053 ) ;
#16453=CARTESIAN_POINT ( 'NONE',  ( 92.35000000006145626, -209.9999881787626919, 81.82400613091914465 ) ) ;
#16454=CARTESIAN_POINT ( 'NONE',  ( 93.67500000000001137, -212.2949673200287179, 88.83583333333334053 ) ) ;
#16456=ORIENTED_EDGE ( 'NONE', *, *, #19113, .F. ) ;
#16463=DIRECTION ( 'NONE',  ( -0.000000000000000000, -0.000000000000000000, 1.000000000000000000 ) ) ;
#16464=ORIENTED_EDGE ( 'NONE', *, *, #53786, .T. ) ;
#16466=CARTESIAN_POINT ( 'NONE',  ( 97.64999999999997726, -208.4700217866474645, 75.20979166840096752 ) ) ;
#16467=CARTESIAN_POINT ( 'NONE',  ( 92.34999999999999432, 91.52997821335252127, 81.05708333333333826 ) ) ;
#16472=CARTESIAN_POINT ( 'NONE',  ( -96.32499999999996021, -207.7050326799711968, 82.98854166840096980 ) ) ;
#16475=CARTESIAN_POINT ( 'NONE',  ( -96.15314808468752972, 91.99731107132950569, 84.61572916753381435 ) ) ;
#16476=EDGE_CURVE ( 'NONE', #6402, #47170, #45078, .T. ) ;
#16477=CARTESIAN_POINT ( 'NONE',  ( 96.15314808468748708, 88.00268892867053694, 79.05947916753380866 ) ) ;
#16485=CARTESIAN_POINT ( 'NONE',  ( -96.15314808468745866, -211.9973110713294489, 76.41364583420048007 ) ) ;
#16487=VERTEX_POINT ( 'NONE', #35674 ) ;
#16495=CARTESIAN_POINT ( 'NONE',  ( -92.69370383062498320, -208.6684592857803011, 76.67822916753378593 ) ) ;
#16497=CARTESIAN_POINT ( 'NONE',  ( -93.67500000000003979, 87.70503267997129626, 76.87666666666666515 ) ) ;
#16502=CARTESIAN_POINT ( 'NONE',  ( 94.99999999999998579, 92.66308142843932671, 83.76906250086715033 ) ) ;
#16511=( BOUNDED_SURFACE ( )  B_SPLINE_SURFACE ( 1, 2, ( 
 ( #3909, #4279, #55391, #14794, #50856, #66318, #26810, #60673, #73781, #39221, #38843, #50100, #61783, #43758, #27170, #37741, #44111, #43398, #5023, #27927, #49734, #9894, #10638, #33560, #56519, #32077, #55015, #4652, #10266, #72659, #73030, #67411, #44497, #67787, #50489, #61413, #27554, #21164, #67035, #15538, #32812, #3545, #33188, #56134, #32450, #21919, #61032, #49375, #55764, #72306, #20805, #44865, #38475, #66676, #39591, #23047, #28661, #51601, #30415, #23408, #63642, #39961, #53361, #34305, #12114, #68157, #17391, #69268, #45976, #57252, #7865, #5758, #47717, #35055, #16653, #30781, #45236, #156, #62537, #53728, #70631, #17754, #29035, #40701, #22672, #57627, #11014, #68903, #22293, #59378, #33941, #40322, #63270, #42091, #13506, #19146, #56888, #5394, #59012, #7505, #11732, #51967, #46337, #515, #65030, #1901, #34677, #24787, #6132, #36432, #28289, #51228, #74157, #45617, #68542, #62918, #17026, #11374, #20993, #14615, #61239, #72492, #3731, #31528, #37928, #19510, #3002, #8617, #54467, #9339, #3366, #43586, #19877, #32264, #14238, #66503, #48093, #71742, #49195, #25895, #37193, #9720, #60135, #26633, #14985, #60859, #32639, #48824, #20244, #8977, #72122, #55212, #25167, #43946, #66862, #2271, #31163, #43215, #54840, #42825, #15349, #36801, #25524, #49564, #38292, #71007, #20633, #42457, #66138, #54113, #71371, #65397, #37564, #60497, #13862, #59749, #8232, #2645, #31903, #26257, #48458, #65754, #26999, #56335, #4853, #67982, #11564, #55584, #38671, #45810, #4104, #67608, #44307, #61601, #50301, #22494, #45056, #21736, #73236, #16101, #16477, #39040, #10087, #68735, #49933, #61979, #67239, #33010, #44693, #45436, #39413, #10459, #33375, #27754, #62358, #50679, #72849, #63106, #21349, #73606, #15735, #55956, #28483, #28119, #10841, #51054, #4472, #33762, #27367, #22116, #56719, #17218, #40153, #5218, #73979, #41286, #68363, #51419, #16858, #39788, #62739, #11207, #34134, #57081, #5588, #22875, #58929, #41622, #52526, #18680, #69455, #35246, #17954, #23974, #57443, #41262, #58540, #705, #7036, #6322, #53278, #46908, #19054, #30336, #35977, #63834, #70178, #51798, #58177, #40899, #12309, #64560, #35607, #1452, #52161, #13039, #46528, #24339, #5959, #29581, #29962, #6675, #1080, #42005, #69817 ),
 ( #28868, #7421, #1815, #347, #24702, #18319, #52913, #64201, #47635, #63462, #46166, #23238, #12673, #70542, #29222, #69099, #17585, #47274, #23599, #64942, #34499, #40517, #11936, #34883, #57817, #54755, #59664, #66055, #42738, #32180, #3285, #49110, #55122, #3648, #8148, #31810, #26174, #36349, #8893, #72036, #25444, #42373, #31071, #26549, #65674, #37102, #49482, #20549, #43503, #66422, #54388, #14529, #14902, #14152, #59290, #60051, #8534, #25810, #43861, #13417, #70923, #72406, #7783, #48373, #2186, #19423, #54026, #37845, #2919, #2564, #71286, #19793, #48741, #31446, #30699, #20911, #53647, #71664, #25072, #48010, #60776, #60413, #20163, #9259, #13780, #43124, #65312, #37481, #36717, #28396, #51332, #27280, #33291, #11120, #56996, #39705, #55500, #4017, #28030, #10749, #4382, #73519, #16387, #44970, #16768, #73891, #10372, #50970, #50211, #67521, #73145, #56246, #15271, #22026, #39328, #32919, #62265, #38584, #34045, #4761, #74270, #62647, #68272, #21650, #22400, #9635, #16010, #44606, #38955, #45348, #67897, #33673, #9999, #5500, #61892, #56629, #38203, #27666, #5128, #50592, #22786, #66776, #61148, #32554, #26916, #49846, #72762, #21263, #44224, #67147, #15652, #61515, #55870, #12951, #64476, #45727, #263, #6239, #23888, #11842, #58837, #5867, #69013, #12595, #35526, #17131, #40812, #18237, #46442, #29139, #30252, #57734, #70097, #58454, #6951, #53192, #69371, #17867, #52438, #41179, #1369, #68649, #35889, #7337, #40064, #23154, #52077, #46824, #34793, #1728, #28777, #17498, #29876, #52829, #63024, #64115, #24260, #620, #46078, #40428, #11484, #23511, #63748, #34411, #47184, #18599, #41540, #12224, #69737, #57355, #35160, #51715, #58097, #6598, #29502, #63375, #992, #7694, #14812, #55035, #36631, #13331, #30611, #19338, #65971, #14058, #65224, #42294, #59576, #59962, #8062, #70456, #32096, #47552, #30984, #41913, #24616, #71949, #71577, #31357, #20074, #24983, #8446, #18963, #25364, #64852, #60693, #9172, #53940, #65591, #43417, #37759, #20463, #36267, #59203, #60330, #43029, #2478, #54309, #48662, #2834, #49018, #31726, #42654, #8808, #48291, #71199, #19706, #37008, #53559, #25724, #14442, #13695, #37397, #70838, #66339, #54670, #2096, #47920, #26088, #3199, #39238, #20823, #4300, #9911 ) ),
 .UNSPECIFIED., .F., .F., .F. ) 
 B_SPLINE_SURFACE_WITH_KNOTS ( ( 2, 2 ),
 ( 3, 2, 2, 2, 2, 2, 2, 2, 2, 2, 2, 2, 2, 2, 2, 2, 2, 2, 2, 2, 2, 2, 2, 2, 2, 2, 2, 2, 2, 2, 2, 2, 2, 2, 2, 2, 2, 2, 2, 2, 2, 2, 2, 2, 2, 2, 2, 2, 2, 2, 2, 2, 2, 2, 2, 2, 2, 2, 2, 2, 2, 2, 2, 2, 2, 2, 2, 2, 2, 2, 2, 2, 2, 2, 2, 2, 2, 2, 2, 2, 2, 2, 2, 2, 2, 2, 2, 2, 2, 2, 2, 2, 2, 2, 2, 2, 2, 2, 2, 2, 2, 2, 2, 2, 2, 2, 2, 2, 2, 2, 2, 2, 2, 2, 2, 2, 2, 2, 2, 2, 2, 2, 2, 2, 2, 2, 2, 2, 2, 2, 2, 2, 2, 2, 2, 2, 2, 2, 2, 2, 2, 2, 3 ),
 ( 0.000000000000000000, 1.000000000000000000 ),
 ( 0.000000000000000000, 0.006944444444444444059, 0.01388888888888888812, 0.02083333333333333218, 0.02777777777777777624, 0.03472222222222222376, 0.04166666666666666435, 0.04861111111111111188, 0.05555555555555555247, 0.06250000000000000000, 0.06944444444444444753, 0.07638888888888889506, 0.08333333333333332871, 0.09027777777777777624, 0.09722222222222222376, 0.1041666666666666713, 0.1111111111111111049, 0.1180555555555555525, 0.1250000000000000000, 0.1319444444444444475, 0.1388888888888888951, 0.1458333333333333426, 0.1527777777777777901, 0.1597222222222222099, 0.1666666666666666574, 0.1736111111111111049, 0.1805555555555555525, 0.1875000000000000000, 0.1944444444444444475, 0.2013888888888888951, 0.2083333333333333426, 0.2152777777777777901, 0.2222222222222222099, 0.2291666666666666574, 0.2361111111111111049, 0.2430555555555555525, 0.2500000000000000000, 0.2569444444444444198, 0.2638888888888888951, 0.2708333333333333148, 0.2777777777777777901, 0.2847222222222222099, 0.2916666666666666852, 0.2986111111111111049, 0.3055555555555555802, 0.3125000000000000000, 0.3194444444444444198, 0.3263888888888888951, 0.3333333333333333148, 0.3402777777777777901, 0.3472222222222222099, 0.3541666666666666852, 0.3611111111111111049, 0.3680555555555555802, 0.3750000000000000000, 0.3819444444444444198, 0.3888888888888888951, 0.3958333333333333148, 0.4027777777777777901, 0.4097222222222222099, 0.4166666666666666852, 0.4236111111111111049, 0.4305555555555555802, 0.4375000000000000000, 0.4444444444444444198, 0.4513888888888888951, 0.4583333333333333148, 0.4652777777777777901, 0.4722222222222222099, 0.4791666666666666852, 0.4861111111111111049, 0.4930555555555555802, 0.5000000000000000000, 0.5069444444444444198, 0.5138888888888888395, 0.5208333333333333703, 0.5277777777777777901, 0.5347222222222222099, 0.5416666666666666297, 0.5486111111111111605, 0.5555555555555555802, 0.5625000000000000000, 0.5694444444444444198, 0.5763888888888888395, 0.5833333333333333703, 0.5902777777777777901, 0.5972222222222222099, 0.6041666666666666297, 0.6111111111111111605, 0.6180555555555555802, 0.6250000000000000000, 0.6319444444444444198, 0.6388888888888888395, 0.6458333333333333703, 0.6527777777777777901, 0.6597222222222222099, 0.6666666666666666297, 0.6736111111111111605, 0.6805555555555555802, 0.6875000000000000000, 0.6944444444444444198, 0.7013888888888888395, 0.7083333333333333703, 0.7152777777777777901, 0.7222222222222222099, 0.7291666666666666297, 0.7361111111111111605, 0.7430555555555555802, 0.7500000000000000000, 0.7569444444444444198, 0.7638888888888888395, 0.7708333333333333703, 0.7777777777777777901, 0.7847222222222222099, 0.7916666666666666297, 0.7986111111111111605, 0.8055555555555555802, 0.8125000000000000000, 0.8194444444444444198, 0.8263888888888888395, 0.8333333333333333703, 0.8402777777777777901, 0.8472222222222222099, 0.8541666666666666297, 0.8611111111111111605, 0.8680555555555555802, 0.8750000000000000000, 0.8819444444444444198, 0.8888888888888888395, 0.8958333333333333703, 0.9027777777777777901, 0.9097222222222222099, 0.9166666666666666297, 0.9236111111111111605, 0.9305555555555555802, 0.9375000000000000000, 0.9444444444444444198, 0.9513888888888888395, 0.9583333333333333703, 0.9652777777777777901, 0.9722222222222222099, 0.9791666666666666297, 0.9842227634901433708 ),
 .UNSPECIFIED. ) 
 GEOMETRIC_REPRESENTATION_ITEM ( )  RATIONAL_B_SPLINE_SURFACE ( (
 ( 1.000000000000000000, 0.8660254037844387076, 1.000000000000000000, 0.8660254037844387076, 1.000000000000000000, 0.8660254037844387076, 1.000000000000000000, 0.8660254037844387076, 1.000000000000000000, 0.8660254037844387076, 1.000000000000000000, 0.8660254037844387076, 1.000000000000000000, 0.8660254037844387076, 1.000000000000000000, 0.8660254037844387076, 1.000000000000000000, 0.8660254037844387076, 1.000000000000000000, 0.8660254037844387076, 1.000000000000000000, 0.8660254037844387076, 1.000000000000000000, 0.8660254037844387076, 1.000000000000000000, 0.8660254037844387076, 1.000000000000000000, 0.8660254037844387076, 1.000000000000000000, 0.8660254037844387076, 1.000000000000000000, 0.8660254037844387076, 1.000000000000000000, 0.8660254037844387076, 1.000000000000000000, 0.8660254037844387076, 1.000000000000000000, 0.8660254037844387076, 1.000000000000000000, 0.8660254037844387076, 1.000000000000000000, 0.8660254037844387076, 1.000000000000000000, 0.8660254037844387076, 1.000000000000000000, 0.8660254037844387076, 1.000000000000000000, 0.8660254037844387076, 1.000000000000000000, 0.8660254037844387076, 1.000000000000000000, 0.8660254037844387076, 1.000000000000000000, 0.8660254037844387076, 1.000000000000000000, 0.8660254037844387076, 1.000000000000000000, 0.8660254037844387076, 1.000000000000000000, 0.8660254037844387076, 1.000000000000000000, 0.8660254037844387076, 1.000000000000000000, 0.8660254037844387076, 1.000000000000000000, 0.8660254037844387076, 1.000000000000000000, 0.8660254037844387076, 1.000000000000000000, 0.8660254037844387076, 1.000000000000000000, 0.8660254037844387076, 1.000000000000000000, 0.8660254037844387076, 1.000000000000000000, 0.8660254037844387076, 1.000000000000000000, 0.8660254037844387076, 1.000000000000000000, 0.8660254037844387076, 1.000000000000000000, 0.8660254037844387076, 1.000000000000000000, 0.8660254037844387076, 1.000000000000000000, 0.8660254037844387076, 1.000000000000000000, 0.8660254037844387076, 1.000000000000000000, 0.8660254037844387076, 1.000000000000000000, 0.8660254037844387076, 1.000000000000000000, 0.8660254037844387076, 1.000000000000000000, 0.8660254037844387076, 1.000000000000000000, 0.8660254037844387076, 1.000000000000000000, 0.8660254037844387076, 1.000000000000000000, 0.8660254037844387076, 1.000000000000000000, 0.8660254037844387076, 1.000000000000000000, 0.8660254037844387076, 1.000000000000000000, 0.8660254037844387076, 1.000000000000000000, 0.8660254037844387076, 1.000000000000000000, 0.8660254037844387076, 1.000000000000000000, 0.8660254037844387076, 1.000000000000000000, 0.8660254037844387076, 1.000000000000000000, 0.8660254037844387076, 1.000000000000000000, 0.8660254037844387076, 1.000000000000000000, 0.8660254037844387076, 1.000000000000000000, 0.8660254037844387076, 1.000000000000000000, 0.8660254037844387076, 1.000000000000000000, 0.8660254037844387076, 1.000000000000000000, 0.8660254037844387076, 1.000000000000000000, 0.8660254037844387076, 1.000000000000000000, 0.8660254037844387076, 1.000000000000000000, 0.8660254037844387076, 1.000000000000000000, 0.8660254037844387076, 1.000000000000000000, 0.8660254037844387076, 1.000000000000000000, 0.8660254037844387076, 1.000000000000000000, 0.8660254037844387076, 1.000000000000000000, 0.8660254037844387076, 1.000000000000000000, 0.8660254037844387076, 1.000000000000000000, 0.8660254037844387076, 1.000000000000000000, 0.8660254037844387076, 1.000000000000000000, 0.8660254037844387076, 1.000000000000000000, 0.8660254037844387076, 1.000000000000000000, 0.8660254037844387076, 1.000000000000000000, 0.8660254037844387076, 1.000000000000000000, 0.8660254037844387076, 1.000000000000000000, 0.8660254037844387076, 1.000000000000000000, 0.8660254037844387076, 1.000000000000000000, 0.8660254037844387076, 1.000000000000000000, 0.8660254037844387076, 1.000000000000000000, 0.8660254037844387076, 1.000000000000000000, 0.8660254037844387076, 1.000000000000000000, 0.8660254037844387076, 1.000000000000000000, 0.8660254037844387076, 1.000000000000000000, 0.8660254037844387076, 1.000000000000000000, 0.8660254037844387076, 1.000000000000000000, 0.8660254037844387076, 1.000000000000000000, 0.8660254037844387076, 1.000000000000000000, 0.8660254037844387076, 1.000000000000000000, 0.8660254037844387076, 1.000000000000000000, 0.8660254037844387076, 1.000000000000000000, 0.8660254037844387076, 1.000000000000000000, 0.8660254037844387076, 1.000000000000000000, 0.8660254037844387076, 1.000000000000000000, 0.8660254037844387076, 1.000000000000000000, 0.8660254037844387076, 1.000000000000000000, 0.8660254037844387076, 1.000000000000000000, 0.8660254037844387076, 1.000000000000000000, 0.8660254037844387076, 1.000000000000000000, 0.8660254037844387076, 1.000000000000000000, 0.8660254037844387076, 1.000000000000000000, 0.8660254037844387076, 1.000000000000000000, 0.8660254037844387076, 1.000000000000000000, 0.8660254037844387076, 1.000000000000000000, 0.8660254037844387076, 1.000000000000000000, 0.8660254037844387076, 1.000000000000000000, 0.8660254037844387076, 1.000000000000000000, 0.8660254037844387076, 1.000000000000000000, 0.8660254037844387076, 1.000000000000000000, 0.8660254037844387076, 1.000000000000000000, 0.8660254037844387076, 1.000000000000000000, 0.8660254037844387076, 1.000000000000000000, 0.8660254037844387076, 1.000000000000000000, 0.8660254037844387076, 1.000000000000000000, 0.8660254037844387076, 1.000000000000000000, 0.8660254037844387076, 1.000000000000000000, 0.8660254037844387076, 1.000000000000000000, 0.8660254037844387076, 1.000000000000000000, 0.8660254037844387076, 1.000000000000000000, 0.8660254037844387076, 1.000000000000000000, 0.8660254037844387076, 1.000000000000000000, 0.8660254037844387076, 1.000000000000000000, 0.8660254037844387076, 1.000000000000000000, 0.8660254037844387076, 1.000000000000000000, 0.8660254037844387076, 1.000000000000000000, 0.8660254037844387076, 1.000000000000000000, 0.8660254037844387076, 1.000000000000000000, 0.8660254037844387076, 1.000000000000000000, 0.8660254037844387076, 1.000000000000000000, 0.8660254037844387076, 1.000000000000000000, 0.8660254037844387076, 1.000000000000000000, 0.8660254037844387076, 1.000000000000000000, 0.8660254037844387076, 1.000000000000000000, 0.8660254037844387076, 1.000000000000000000, 0.8660254037844387076, 1.000000000000000000, 0.8660254037844387076, 1.000000000000000000, 0.9024560516293018697, 0.9469512977404641596),
 ( 1.000000000000000000, 0.8660254037844387076, 1.000000000000000000, 0.8660254037844387076, 1.000000000000000000, 0.8660254037844387076, 1.000000000000000000, 0.8660254037844387076, 1.000000000000000000, 0.8660254037844387076, 1.000000000000000000, 0.8660254037844387076, 1.000000000000000000, 0.8660254037844387076, 1.000000000000000000, 0.8660254037844387076, 1.000000000000000000, 0.8660254037844387076, 1.000000000000000000, 0.8660254037844387076, 1.000000000000000000, 0.8660254037844387076, 1.000000000000000000, 0.8660254037844387076, 1.000000000000000000, 0.8660254037844387076, 1.000000000000000000, 0.8660254037844387076, 1.000000000000000000, 0.8660254037844387076, 1.000000000000000000, 0.8660254037844387076, 1.000000000000000000, 0.8660254037844387076, 1.000000000000000000, 0.8660254037844387076, 1.000000000000000000, 0.8660254037844387076, 1.000000000000000000, 0.8660254037844387076, 1.000000000000000000, 0.8660254037844387076, 1.000000000000000000, 0.8660254037844387076, 1.000000000000000000, 0.8660254037844387076, 1.000000000000000000, 0.8660254037844387076, 1.000000000000000000, 0.8660254037844387076, 1.000000000000000000, 0.8660254037844387076, 1.000000000000000000, 0.8660254037844387076, 1.000000000000000000, 0.8660254037844387076, 1.000000000000000000, 0.8660254037844387076, 1.000000000000000000, 0.8660254037844387076, 1.000000000000000000, 0.8660254037844387076, 1.000000000000000000, 0.8660254037844387076, 1.000000000000000000, 0.8660254037844387076, 1.000000000000000000, 0.8660254037844387076, 1.000000000000000000, 0.8660254037844387076, 1.000000000000000000, 0.8660254037844387076, 1.000000000000000000, 0.8660254037844387076, 1.000000000000000000, 0.8660254037844387076, 1.000000000000000000, 0.8660254037844387076, 1.000000000000000000, 0.8660254037844387076, 1.000000000000000000, 0.8660254037844387076, 1.000000000000000000, 0.8660254037844387076, 1.000000000000000000, 0.8660254037844387076, 1.000000000000000000, 0.8660254037844387076, 1.000000000000000000, 0.8660254037844387076, 1.000000000000000000, 0.8660254037844387076, 1.000000000000000000, 0.8660254037844387076, 1.000000000000000000, 0.8660254037844387076, 1.000000000000000000, 0.8660254037844387076, 1.000000000000000000, 0.8660254037844387076, 1.000000000000000000, 0.8660254037844387076, 1.000000000000000000, 0.8660254037844387076, 1.000000000000000000, 0.8660254037844387076, 1.000000000000000000, 0.8660254037844387076, 1.000000000000000000, 0.8660254037844387076, 1.000000000000000000, 0.8660254037844387076, 1.000000000000000000, 0.8660254037844387076, 1.000000000000000000, 0.8660254037844387076, 1.000000000000000000, 0.8660254037844387076, 1.000000000000000000, 0.8660254037844387076, 1.000000000000000000, 0.8660254037844387076, 1.000000000000000000, 0.8660254037844387076, 1.000000000000000000, 0.8660254037844387076, 1.000000000000000000, 0.8660254037844387076, 1.000000000000000000, 0.8660254037844387076, 1.000000000000000000, 0.8660254037844387076, 1.000000000000000000, 0.8660254037844387076, 1.000000000000000000, 0.8660254037844387076, 1.000000000000000000, 0.8660254037844387076, 1.000000000000000000, 0.8660254037844387076, 1.000000000000000000, 0.8660254037844387076, 1.000000000000000000, 0.8660254037844387076, 1.000000000000000000, 0.8660254037844387076, 1.000000000000000000, 0.8660254037844387076, 1.000000000000000000, 0.8660254037844387076, 1.000000000000000000, 0.8660254037844387076, 1.000000000000000000, 0.8660254037844387076, 1.000000000000000000, 0.8660254037844387076, 1.000000000000000000, 0.8660254037844387076, 1.000000000000000000, 0.8660254037844387076, 1.000000000000000000, 0.8660254037844387076, 1.000000000000000000, 0.8660254037844387076, 1.000000000000000000, 0.8660254037844387076, 1.000000000000000000, 0.8660254037844387076, 1.000000000000000000, 0.8660254037844387076, 1.000000000000000000, 0.8660254037844387076, 1.000000000000000000, 0.8660254037844387076, 1.000000000000000000, 0.8660254037844387076, 1.000000000000000000, 0.8660254037844387076, 1.000000000000000000, 0.8660254037844387076, 1.000000000000000000, 0.8660254037844387076, 1.000000000000000000, 0.8660254037844387076, 1.000000000000000000, 0.8660254037844387076, 1.000000000000000000, 0.8660254037844387076, 1.000000000000000000, 0.8660254037844387076, 1.000000000000000000, 0.8660254037844387076, 1.000000000000000000, 0.8660254037844387076, 1.000000000000000000, 0.8660254037844387076, 1.000000000000000000, 0.8660254037844387076, 1.000000000000000000, 0.8660254037844387076, 1.000000000000000000, 0.8660254037844387076, 1.000000000000000000, 0.8660254037844387076, 1.000000000000000000, 0.8660254037844387076, 1.000000000000000000, 0.8660254037844387076, 1.000000000000000000, 0.8660254037844387076, 1.000000000000000000, 0.8660254037844387076, 1.000000000000000000, 0.8660254037844387076, 1.000000000000000000, 0.8660254037844387076, 1.000000000000000000, 0.8660254037844387076, 1.000000000000000000, 0.8660254037844387076, 1.000000000000000000, 0.8660254037844387076, 1.000000000000000000, 0.8660254037844387076, 1.000000000000000000, 0.8660254037844387076, 1.000000000000000000, 0.8660254037844387076, 1.000000000000000000, 0.8660254037844387076, 1.000000000000000000, 0.8660254037844387076, 1.000000000000000000, 0.8660254037844387076, 1.000000000000000000, 0.8660254037844387076, 1.000000000000000000, 0.8660254037844387076, 1.000000000000000000, 0.8660254037844387076, 1.000000000000000000, 0.8660254037844387076, 1.000000000000000000, 0.8660254037844387076, 1.000000000000000000, 0.8660254037844387076, 1.000000000000000000, 0.8660254037844387076, 1.000000000000000000, 0.8660254037844387076, 1.000000000000000000, 0.8660254037844387076, 1.000000000000000000, 0.8660254037844387076, 1.000000000000000000, 0.8660254037844387076, 1.000000000000000000, 0.8660254037844387076, 1.000000000000000000, 0.8660254037844387076, 1.000000000000000000, 0.8660254037844387076, 1.000000000000000000, 0.8660254037844387076, 1.000000000000000000, 0.8660254037844387076, 1.000000000000000000, 0.8660254037844387076, 1.000000000000000000, 0.8660254037844387076, 1.000000000000000000, 0.8660254037844387076, 1.000000000000000000, 0.8660254037844387076, 1.000000000000000000, 0.8660254037844387076, 1.000000000000000000, 0.8660254037844387076, 1.000000000000000000, 0.8660254037844387076, 1.000000000000000000, 0.8660254037844387076, 1.000000000000000000, 0.9024560516293018697, 0.9469512977404641596) ) ) 
 REPRESENTATION_ITEM ( '' )  SURFACE ( )  );
#16513=CARTESIAN_POINT ( 'NONE',  ( 96.32499999999998863, 87.70503267997126784, 78.78166666666666629 ) ) ;
#16515=CARTESIAN_POINT ( 'NONE',  ( -97.30629616937501680, 88.66845928578038638, 88.42572916753381662 ) ) ;
#16517=CARTESIAN_POINT ( 'NONE',  ( -97.64999999999994884, -211.5299782133524502, 86.24291666666665890 ) ) ;
#16526=CARTESIAN_POINT ( 'NONE',  ( 92.69370383062501162, -211.3315407142195852, 86.67947916753382742 ) ) ;
#16530=EDGE_CURVE ( 'NONE', #32728, #4573, #962, .T. ) ;
#16534=CARTESIAN_POINT ( 'NONE',  ( 93.84685191531251292, -211.9973110713294489, 78.95364583420047211 ) ) ;
#16537=CARTESIAN_POINT ( 'NONE',  ( 93.84685191531251292, -211.9973110713294489, 84.19239583420049655 ) ) ;
#16549=CARTESIAN_POINT ( 'NONE',  ( 96.32499999999997442, 92.29496732002878900, 85.97833333333332462 ) ) ;
#16553=ORIENTED_EDGE ( 'NONE', *, *, #41317, .F. ) ;
#16558=VERTEX_POINT ( 'NONE', #7853 ) ;
#16559=CARTESIAN_POINT ( 'NONE',  ( 96.15314808468750130, -211.9973110713294489, 76.51947916753380241 ) ) ;
#16562=ORIENTED_EDGE ( 'NONE', *, *, #28166, .F. ) ;
#16567=CARTESIAN_POINT ( 'NONE',  ( -96.32499999999996021, -207.7050326799711968, 88.62416666666665321 ) ) ;
#16570=CARTESIAN_POINT ( 'NONE',  ( -95.00000000000002842, 87.33691857156074434, 76.62531250086715318 ) ) ;
#16573=CARTESIAN_POINT ( 'NONE',  ( 97.30629616937498838, 88.66845928578037217, 75.93739583420047268 ) ) ;
#16577=CARTESIAN_POINT ( 'NONE',  ( -96.15314808468745866, -211.9973110713294489, 87.20864583420046756 ) ) ;
#16583=CARTESIAN_POINT ( 'NONE',  ( -94.99999999999997158, -212.6630814284392557, 79.64156250086713840 ) ) ;
#16586=CARTESIAN_POINT ( 'NONE',  ( -94.99999999999997158, -213.0599564267049857, 79.36374999999996760 ) ) ;
#16589=CARTESIAN_POINT ( 'NONE',  ( 1.243286885786405054E-17, -120.0000000000000000, -85.60000000000000853 ) ) ;
#16590=CARTESIAN_POINT ( 'NONE',  ( -97.30629616937501680, 90.00000000000004263, 81.38781250086714181 ) ) ;
#16604=CARTESIAN_POINT ( 'NONE',  ( -97.30629616937497417, -211.3315407142195852, 77.78947916753381264 ) ) ;
#16608=ORIENTED_EDGE ( 'NONE', *, *, #5627, .F. ) ;
#16613=AXIS2_PLACEMENT_3D ( 'NONE', #34354, #67460, #5442 ) ;
#16626=CARTESIAN_POINT ( 'NONE',  ( 93.84685191531249870, -208.0026889286704943, 88.90197916753380980 ) ) ;
#16627=CARTESIAN_POINT ( 'NONE',  ( -97.64999999999994884, 91.52997821335257811, 77.88208333333332689 ) ) ;
#16629=CYLINDRICAL_SURFACE ( 'NONE', #45307, 3.299999999999969624 ) ;
#16636=ORIENTED_EDGE ( 'NONE', *, *, #2343, .T. ) ;
#16640=EDGE_CURVE ( 'NONE', #50612, #16250, #23995, .T. ) ;
#16642=CARTESIAN_POINT ( 'NONE',  ( 97.64999999999997726, 88.47002178664753558, 87.08958333333333712 ) ) ;
#16643=FACE_OUTER_BOUND ( 'NONE', #11799, .T. ) ;
#16653=CARTESIAN_POINT ( 'NONE',  ( 93.84685191531248449, 91.99731107132950569, 85.72697916753379843 ) ) ;
#16656=CARTESIAN_POINT ( 'NONE',  ( 95.00000000000000000, -207.3369185715606307, 85.03906250086714635 ) ) ;
#16666=CARTESIAN_POINT ( 'NONE',  ( -92.69370383062498320, -211.3315407142195852, 88.63739583420047552 ) ) ;
#16667=CARTESIAN_POINT ( 'NONE',  ( -97.30629616937501680, 88.66845928578038638, 86.67947916753382742 ) ) ;
#16670=CARTESIAN_POINT ( 'NONE',  ( 97.30629616937498838, 91.33154071421968467, 83.02822916753379445 ) ) ;
#16671=CARTESIAN_POINT ( 'NONE',  ( -95.00000000000002842, 92.66308142843932671, 84.40406250086712703 ) ) ;
#16672=ORIENTED_EDGE ( 'NONE', *, *, #72647, .F. ) ;
#16675=DIRECTION ( 'NONE',  ( 1.000000000000000000, 0.000000000000000000, 0.000000000000000000 ) ) ;
#16678=CARTESIAN_POINT ( 'NONE',  ( -26.50044424985255276, 0.001194404164626844313, -64.00000000000000000 ) ) ;
#16679=CARTESIAN_POINT ( 'NONE',  ( -95.00000000000002842, 90.00000000000004263, 90.00000000000000000 ) ) ;
#16686=ORIENTED_EDGE ( 'NONE', *, *, #31911, .T. ) ;
#16689=CARTESIAN_POINT ( 'NONE',  ( -96.32500000000001705, 87.70503267997129626, 79.31083333333333485 ) ) ;
#16698=CARTESIAN_POINT ( 'NONE',  ( -92.69370383062504004, 90.00000000000004263, 77.26031250086714408 ) ) ;
#16704=CARTESIAN_POINT ( 'NONE',  ( -97.30629616937495996, -209.9999999999999716, 88.53156250086716739 ) ) ;
#16707=CARTESIAN_POINT ( 'NONE',  ( 97.30629616937498838, 88.66845928578035796, 76.09614583420048461 ) ) ;
#16711=CARTESIAN_POINT ( 'NONE',  ( -94.99999999999997158, -212.6630814284392557, 79.16531250086715943 ) ) ;
#16712=CARTESIAN_POINT ( 'NONE',  ( -97.64999999996712177, 90.00000839536629371, 84.99910573348492449 ) ) ;
#16713=ORIENTED_EDGE ( 'NONE', *, *, #64751, .F. ) ;
#16714=CARTESIAN_POINT ( 'NONE',  ( -92.35000000000003695, 90.00002467581377630, 87.22187585518554442 ) ) ;
#16715=CARTESIAN_POINT ( 'NONE',  ( -96.32499999999996021, -207.7050326799711968, 75.92416666666666458 ) ) ;
#16723=CARTESIAN_POINT ( 'NONE',  ( -93.84685191531252713, 88.00268892867056536, 77.31322916753381946 ) ) ;
#16724=CARTESIAN_POINT ( 'NONE',  ( 92.69370383062501162, -211.3315407142195852, 81.44072916753381719 ) ) ;
#16728=EDGE_CURVE ( 'NONE', #65017, #73292, #72836, .T. ) ;
#16730=VECTOR ( 'NONE', #9659, 1000.000000000000000 ) ;
#16738=CARTESIAN_POINT ( 'NONE',  ( 92.69370383062501162, -208.6684592857803295, 75.14364583420049826 ) ) ;
#16741=CARTESIAN_POINT ( 'NONE',  ( 93.67500000000001137, -212.2949673200287179, 83.75583333333332803 ) ) ;
#16742=( BOUNDED_CURVE ( )  B_SPLINE_CURVE ( 2, ( #33585, #50510, #62942, #44519, #73437, #38866, #40349 ),
 .UNSPECIFIED., .F., .F. ) 
 B_SPLINE_CURVE_WITH_KNOTS ( ( 3, 2, 2, 3 ),
 ( 0.5000000000000000000, 0.5069444444444444198, 0.5138888888888887285, 0.5208333333333332593 ),
 .UNSPECIFIED. ) 
 CURVE ( )  GEOMETRIC_REPRESENTATION_ITEM ( )  RATIONAL_B_SPLINE_CURVE ( ( 1.000000000000000000, 0.8660254037844387076, 1.000000000000000000, 0.8660254037844387076, 1.000000000000000000, 0.8660254037844408170, 0.9999999999999978906 ) ) 
 REPRESENTATION_ITEM ( '' )  );
#16743=CARTESIAN_POINT ( 'NONE',  ( 96.15314808468748708, 88.00268892867053694, 84.93322916753382401 ) ) ;
#16745=CARTESIAN_POINT ( 'NONE',  ( 96.32499999999998863, -207.7050326799711968, 79.62833333333333030 ) ) ;
#16748=ORIENTED_EDGE ( 'NONE', *, *, #36567, .T. ) ;
#16756=CARTESIAN_POINT ( 'NONE',  ( 95.00000000000000000, -209.9999999999999716, 90.00000000000000000 ) ) ;
#16758=ORIENTED_EDGE ( 'NONE', *, *, #51683, .T. ) ;
#16759=CARTESIAN_POINT ( 'NONE',  ( -93.67499999999998295, -207.7050326799711968, 82.88270833506763324 ) ) ;
#16763=ORIENTED_EDGE ( 'NONE', *, *, #70526, .T. ) ;
#16764=CARTESIAN_POINT ( 'NONE',  ( 97.64999999999997726, 91.52997821335252127, 81.55979166840097605 ) ) ;
#16765=CARTESIAN_POINT ( 'NONE',  ( -92.35000000000003695, 90.00000000000004263, 79.60187500173429953 ) ) ;
#16768=CARTESIAN_POINT ( 'NONE',  ( 96.15314808468748708, 88.00268892867053694, 84.29822916753381890 ) ) ;
#16769=CARTESIAN_POINT ( 'NONE',  ( -93.67499999999998295, -207.7050326799711968, 86.61333333333332973 ) ) ;
#16782=PLANE ( 'NONE',  #33602 ) ;
#16785=DIRECTION ( 'NONE',  ( 0.000000000000000000, 0.000000000000000000, 1.000000000000000000 ) ) ;
#16786=CARTESIAN_POINT ( 'NONE',  ( -94.99999999999997158, -207.3369185715606307, 82.65781250086715204 ) ) ;
#16788=CARTESIAN_POINT ( 'NONE',  ( -95.00000000000002842, 87.33691857156074434, 87.26156250086714294 ) ) ;
#16791=CARTESIAN_POINT ( 'NONE',  ( -93.67499999999998295, -212.2949673200287179, 77.59104166840097605 ) ) ;
#16795=CARTESIAN_POINT ( 'NONE',  ( 97.30629616937498838, 91.33154071421968467, 75.40822916753381833 ) ) ;
#16798=CARTESIAN_POINT ( 'NONE',  ( -92.35000000000000853, -208.4700217866474929, 78.94041666666664980 ) ) ;
#16801=DIRECTION ( 'NONE',  ( -0.000000000000000000, -0.000000000000000000, 1.000000000000000000 ) ) ;
#16802=CARTESIAN_POINT ( 'NONE',  ( -23.50044424985255276, 0.001194404164626844313, -64.00000000000000000 ) ) ;
#16804=CARTESIAN_POINT ( 'NONE',  ( -94.99999999999997158, -207.3369185715606307, 89.00781250086716057 ) ) ;
#16808=CARTESIAN_POINT ( 'NONE',  ( -92.69370383062505425, 88.66845928578038638, 80.38239583420049428 ) ) ;
#16816=CARTESIAN_POINT ( 'NONE',  ( 97.64999999999449187, -210.0000054026048701, 81.50687481489494246 ) ) ;
#16820=CARTESIAN_POINT ( 'NONE',  ( 96.66077099052525057, -211.6002630214759961, 74.80065534806806227 ) ) ;
#16831=CARTESIAN_POINT ( 'NONE',  ( 95.00000000000000000, -206.9400435732949575, 86.66624999999999091 ) ) ;
#16834=ORIENTED_EDGE ( 'NONE', *, *, #36313, .F. ) ;
#16848=CARTESIAN_POINT ( 'NONE',  ( 95.00000000000000000, -206.9400435732949575, 77.85562500173429612 ) ) ;
#16849=CARTESIAN_POINT ( 'NONE',  ( 96.32499999999998863, 87.70503267997126784, 81.32166666666667254 ) ) ;
#16851=VERTEX_POINT ( 'NONE', #58072 ) ;
#16856=CARTESIAN_POINT ( 'NONE',  ( -93.67500000000003979, 92.29496732002878900, 89.23270833506762756 ) ) ;
#16857=CARTESIAN_POINT ( 'NONE',  ( -95.00000000000002842, 87.33691857156074434, 81.70531250086715147 ) ) ;
#16858=CARTESIAN_POINT ( 'NONE',  ( 93.84685191531248449, 88.00268892867053694, 77.04864583420047097 ) ) ;
#16860=DIRECTION ( 'NONE',  ( 1.000000000000000000, 0.000000000000000000, 0.000000000000000000 ) ) ;
#16866=CARTESIAN_POINT ( 'NONE',  ( -94.99999999999997158, -207.3369185715606307, 76.78406250086712248 ) ) ;
#16867=VERTEX_POINT ( 'NONE', #73592 ) ;
#16870=VERTEX_POINT ( 'NONE', #67596 ) ;
#16871=CARTESIAN_POINT ( 'NONE',  ( -95.00000000000002842, 90.00000000000004263, 90.00000000000000000 ) ) ;
#16874=CARTESIAN_POINT ( 'NONE',  ( -96.15314808468745866, -211.9973110713294489, 77.04864583420047097 ) ) ;
#16885=CARTESIAN_POINT ( 'NONE',  ( 94.99999999999998579, 92.66308142843932671, 85.03906250086714635 ) ) ;
#16886=LINE ( 'NONE', #27785, #16020 ) ;
#16887=CARTESIAN_POINT ( 'NONE',  ( -92.34999999999999432, -209.9999999999999716, 90.00000000000000000 ) ) ;
#16888=DIRECTION ( 'NONE',  ( -1.000000000000000000, -0.000000000000000000, -0.000000000000000000 ) ) ;
#16897=CARTESIAN_POINT ( 'NONE',  ( -92.35000000000003695, 90.00000000000004263, 90.00000000000000000 ) ) ;
#16903=CARTESIAN_POINT ( 'NONE',  ( -92.34999999999999432, -209.9999999999999716, 83.33250000000001023 ) ) ;
#16906=CARTESIAN_POINT ( 'NONE',  ( -92.35000000018064270, -210.0000309433161476, 78.33187387208045038 ) ) ;
#16907=EDGE_LOOP ( 'NONE', ( #34482, #63340, #24438, #50549 ) ) ;
#16908=ADVANCED_FACE ( 'NONE', ( #44679 ), #46153, .F. ) ;
#16912=CARTESIAN_POINT ( 'NONE',  ( 97.30629616937498838, -209.9999999999999716, 84.40406250086715545 ) ) ;
#16920=CARTESIAN_POINT ( 'NONE',  ( 97.30629616937498838, -208.6684592857803295, 79.21822916753380639 ) ) ;
#16921=EDGE_LOOP ( 'NONE', ( #24076, #1798, #63244, #30429 ) ) ;
#16922=CARTESIAN_POINT ( 'NONE',  ( 92.69370383062501162, -209.9999999999999716, 82.18156250086715886 ) ) ;
#16925=ORIENTED_EDGE ( 'NONE', *, *, #4199, .T. ) ;
#16926=CARTESIAN_POINT ( 'NONE',  ( 97.65000000000000568, 91.52997821335252127, 80.28979166840095161 ) ) ;
#16930=CARTESIAN_POINT ( 'NONE',  ( -96.15314808468752972, 91.99731107132950569, 75.09072916753380866 ) ) ;
#16931=CARTESIAN_POINT ( 'NONE',  ( 92.34999999999999432, 90.00000000000002842, 90.00000000000000000 ) ) ;
#16933=CARTESIAN_POINT ( 'NONE',  ( 97.64999999999690772, -210.0000040461968638, 77.06187486178042434 ) ) ;
#16934=CARTESIAN_POINT ( 'NONE',  ( 93.67500000000001137, -212.2949673200287179, 88.28020833506764120 ) ) ;
#16935=ORIENTED_EDGE ( 'NONE', *, *, #31388, .F. ) ;
#16937=EDGE_LOOP ( 'NONE', ( #53996, #66981, #72927, #64723 ) ) ;
#16946=VECTOR ( 'NONE', #360, 1000.000000000000000 ) ;
#16948=ORIENTED_EDGE ( 'NONE', *, *, #38685, .T. ) ;
#16952=CARTESIAN_POINT ( 'NONE',  ( -96.15314808468751551, 88.00268892867056536, 75.30239583420048177 ) ) ;
#16953=ORIENTED_EDGE ( 'NONE', *, *, #55622, .F. ) ;
#16954=CARTESIAN_POINT ( 'NONE',  ( 92.69370383062498320, 90.00000000000002842, 89.64281250086713726 ) ) ;
#16955=( BOUNDED_CURVE ( )  B_SPLINE_CURVE ( 2, ( #9929, #32851, #21575, #39627, #9190, #15196, #73818 ),
 .UNSPECIFIED., .F., .F. ) 
 B_SPLINE_CURVE_WITH_KNOTS ( ( 3, 2, 2, 3 ),
 ( 0.1270039290051391268, 0.1340595452767650020, 0.1411153108176473603, 0.1481709449575277227 ),
 .UNSPECIFIED. ) 
 CURVE ( )  GEOMETRIC_REPRESENTATION_ITEM ( )  RATIONAL_B_SPLINE_CURVE ( ( 0.9999943314824810692, 0.8660282381031599863, 1.000000000000000000, 0.8660254037844387076, 1.000000000000000000, 0.8660278988214527018, 0.9999950100189032298 ) ) 
 REPRESENTATION_ITEM ( '' )  );
#16958=CARTESIAN_POINT ( 'NONE',  ( -97.30629616937497417, -211.3315407142195852, 85.25072916753379104 ) ) ;
#16961=CARTESIAN_POINT ( 'NONE',  ( 94.37155072198216033, -212.5563123626347419, 74.98613922222766348 ) ) ;
#16963=CARTESIAN_POINT ( 'NONE',  ( -93.51319757292672818, -208.1953243530631994, 74.81083481226637844 ) ) ;
#16969=CARTESIAN_POINT ( 'NONE',  ( 92.34999999999999432, 90.00000000000002842, 90.00000000000000000 ) ) ;
#16972=CARTESIAN_POINT ( 'NONE',  ( -92.69370383062504004, 90.00000000000004263, 81.07031250086714635 ) ) ;
#16973=CARTESIAN_POINT ( 'NONE',  ( -12.75044424985254921, 0.001194404164626844313, -85.60000000000000853 ) ) ;
#16982=CARTESIAN_POINT ( 'NONE',  ( 96.32499999999998863, -212.2949673200287179, 86.48104166840096241 ) ) ;
#16985=CARTESIAN_POINT ( 'NONE',  ( -93.67500000000003979, 92.29496732002878900, 87.32770833506762642 ) ) ;
#16986=CARTESIAN_POINT ( 'NONE',  ( -92.69370383062498320, -209.9999999999999716, 79.32406250086715715 ) ) ;
#17005=CARTESIAN_POINT ( 'NONE',  ( 96.15314808468750130, -211.9973110713294489, 88.58447916753381435 ) ) ;
#17018=CARTESIAN_POINT ( 'NONE',  ( -0.0004442498525516064278, 0.001194404164626844313, -64.00000000000000000 ) ) ;
#17026=CARTESIAN_POINT ( 'NONE',  ( 96.15314808468748708, 88.00268892867053694, 83.50447916753381605 ) ) ;
#17028=CARTESIAN_POINT ( 'NONE',  ( 93.84685191531249870, -208.0026889286704943, 84.45697916753380241 ) ) ;
#17032=CARTESIAN_POINT ( 'NONE',  ( -93.67500000000003979, 87.70503267997129626, 84.49666666666666970 ) ) ;
#17037=CARTESIAN_POINT ( 'NONE',  ( -94.99999999999997158, -207.3369185715606307, 88.84906250086713442 ) ) ;
#17038=CARTESIAN_POINT ( 'NONE',  ( -96.15314808468752972, 91.99731107132950569, 87.15572916753382060 ) ) ;
#17041=CARTESIAN_POINT ( 'NONE',  ( 93.84685191531248449, 88.00268892867053694, 85.93864583420048575 ) ) ;
#17042=CARTESIAN_POINT ( 'NONE',  ( -92.69370383062504004, 90.00000000000004263, 86.15031250086714465 ) ) ;
#17044=ORIENTED_EDGE ( 'NONE', *, *, #27848, .T. ) ;
#17045=CARTESIAN_POINT ( 'NONE',  ( -96.32500000000001705, 92.29496732002878900, 87.98916666666666231 ) ) ;
#17046=CARTESIAN_POINT ( 'NONE',  ( 92.35000000000000853, -211.5299782133524218, 76.16229166840095388 ) ) ;
#17049=CARTESIAN_POINT ( 'NONE',  ( -96.15314808468747287, -208.0026889286704943, 85.09197916753380753 ) ) ;
#17050=LINE ( 'NONE', #4674, #49879 ) ;
#17052=CARTESIAN_POINT ( 'NONE',  ( -99.99999999999998579, -116.0000000000000000, 39.99999999999996447 ) ) ;
#17061=CARTESIAN_POINT ( 'NONE',  ( -95.00000000000002842, 86.94004357329504273, 77.45874999999999488 ) ) ;
#17065=CARTESIAN_POINT ( 'NONE',  ( -97.64999999960622290, -209.9999706925929672, 76.74344264316562203 ) ) ;
#17068=CARTESIAN_POINT ( 'NONE',  ( -97.64999999999992042, -208.4700217866474929, 79.78708333333331382 ) ) ;
#17070=CARTESIAN_POINT ( 'NONE',  ( -96.15314808468752972, 91.99731107132950569, 80.01197916753380923 ) ) ;
#17075=FACE_OUTER_BOUND ( 'NONE', #66317, .T. ) ;
#17076=CARTESIAN_POINT ( 'NONE',  ( -95.00000000000002842, 86.94004357329504273, 75.63312500173429953 ) ) ;
#17077=CARTESIAN_POINT ( 'NONE',  ( -92.69370383062498320, -208.6684592857803011, 89.53697916753382913 ) ) ;
#17081=CARTESIAN_POINT ( 'NONE',  ( 96.15314808468748708, 88.00268892867053694, 76.67822916753381435 ) ) ;
#17082=CARTESIAN_POINT ( 'NONE',  ( -92.69370383062498320, -209.9999999999999716, 79.95906250086714806 ) ) ;
#17087=CARTESIAN_POINT ( 'NONE',  ( -92.34999999999999432, -209.9999999999999716, 75.71250000000000568 ) ) ;
#17088=CARTESIAN_POINT ( 'NONE',  ( 97.64999999999999147, -209.9999999999999716, 78.96687500173429441 ) ) ;
#17090=CARTESIAN_POINT ( 'NONE',  ( -97.30629616937501680, 90.00000000000004263, 75.19656250086714522 ) ) ;
#17091=CARTESIAN_POINT ( 'NONE',  ( 97.30629616937498838, -208.6684592857803011, 79.21822916753380639 ) ) ;
#17095=EDGE_CURVE ( 'NONE', #42482, #14594, #72546, .T. ) ;
#17096=CARTESIAN_POINT ( 'NONE',  ( -95.00000000000002842, 93.05995642670504253, 75.23624999999998408 ) ) ;
#17098=AXIS2_PLACEMENT_3D ( 'NONE', #2570, #53653, #35613 ) ;
#17106=CARTESIAN_POINT ( 'NONE',  ( 92.69370383062501162, -208.6684592857803295, 75.77864583420048916 ) ) ;
#17108=VERTEX_POINT ( 'NONE', #59650 ) ;
#17109=CARTESIAN_POINT ( 'NONE',  ( 96.15314808468748708, 88.00268892867053694, 81.75822916753382685 ) ) ;
#17110=CARTESIAN_POINT ( 'NONE',  ( 97.64999999999997726, -211.5299782133524502, 78.83458333333334167 ) ) ;
#17119=DIRECTION ( 'NONE',  ( 1.000000000000000000, 0.000000000000000000, 0.000000000000000000 ) ) ;
#17120=CARTESIAN_POINT ( 'NONE',  ( 92.35000000000000853, -209.9999999999999716, 86.90437500173429441 ) ) ;
#17124=CARTESIAN_POINT ( 'NONE',  ( -97.64999999999994884, -208.4700217866474645, 83.67645833506762187 ) ) ;
#17126=FACE_OUTER_BOUND ( 'NONE', #60760, .T. ) ;
#17128=CARTESIAN_POINT ( 'NONE',  ( 97.64999999999997726, 91.52997821335252127, 77.74979166840097378 ) ) ;
#17129=CARTESIAN_POINT ( 'NONE',  ( -95.00000000000002842, 93.05995642670501411, 79.76062500173429726 ) ) ;
#17131=CARTESIAN_POINT ( 'NONE',  ( 94.99999999999998579, 87.33691857156068750, 81.07031250086716057 ) ) ;
#17132=CARTESIAN_POINT ( 'NONE',  ( 97.64999999999999147, 90.00000000000002842, 83.33250000000001023 ) ) ;
#17136=DIRECTION ( 'NONE',  ( -0.000000000000000000, -0.000000000000000000, 1.000000000000000000 ) ) ;
#17142=ORIENTED_EDGE ( 'NONE', *, *, #49373, .T. ) ;
#17143=EDGE_CURVE ( 'NONE', #33107, #72660, #37395, .T. ) ;
#17150=DIRECTION ( 'NONE',  ( -0.000000000000000000, -0.000000000000000000, 1.000000000000000000 ) ) ;
#17152=CARTESIAN_POINT ( 'NONE',  ( -93.84685191531247028, -211.9973110713294489, 80.48822916753381662 ) ) ;
#17155=ADVANCED_FACE ( 'NONE', ( #3636 ), #37834, .F. ) ;
#17158=DIRECTION ( 'NONE',  ( 0.000000000000000000, 0.000000000000000000, 1.000000000000000000 ) ) ;
#17160=CYLINDRICAL_SURFACE ( 'NONE', #28456, 2.649999999999985700 ) ;
#17164=CARTESIAN_POINT ( 'NONE',  ( -97.64996284860670528, -208.4700003372805384, 76.69145685134844825 ) ) ;
#17165=LINE ( 'NONE', #51003, #59250 ) ;
#17167=EDGE_CURVE ( 'NONE', #48244, #29385, #9244, .T. ) ;
#17169=CARTESIAN_POINT ( 'NONE',  ( 94.99999999999998579, 92.66308142843932671, 85.83281250086717762 ) ) ;
#17170=CARTESIAN_POINT ( 'NONE',  ( -97.30629616937497417, -208.6684592857803295, 88.47864583420047779 ) ) ;
#17171=CARTESIAN_POINT ( 'NONE',  ( -97.64999999994212487, -210.0000112241608292, 75.47473230080855444 ) ) ;
#17174=CARTESIAN_POINT ( 'NONE',  ( -96.15314808468752972, 91.99731107132950569, 78.10697916753380809 ) ) ;
#17175=EDGE_CURVE ( 'NONE', #59589, #29023, #16057, .T. ) ;
#17180=( BOUNDED_SURFACE ( )  B_SPLINE_SURFACE ( 1, 2, ( 
 ( #33088, #73683, #37999, #55293, #4180, #49634, #50004, #72926, #21430, #44388, #67314, #38747, #61678, #56029, #4551, #50382, #51879, #74056, #46242, #34960, #45516, #33843, #16934, #69176, #40229, #17293, #46982, #63179, #785, #69539, #57161, #68811, #11637, #34580, #39872, #62816, #46608, #69894, #5664, #12018, #22952, #57899, #29659, #60, #11279, #45890, #52242, #28943, #10918, #51504, #22570, #57527, #6396, #58257, #6038, #419, #51132, #52608, #18389, #63913, #1161, #68441, #41336, #23314, #23672, #17664, #40602, #6753, #63544, #12382, #18036, #28559, #40977, #29298, #35328, #56788, #24058, #5298, #28200, #34213, #7496, #14229, #36793, #36421, #13852, #42817, #52990, #70623, #19868, #65746, #71733, #59739, #25159, #7124, #53351, #19137, #20236, #54105, #42448, #48447, #35677, #31152, #13498, #2636, #59368, #58619, #53718, #37184, #64637, #30041, #1891, #24778, #25885, #7857, #30772, #1529, #48085, #8223, #24409, #12751, #70252, #70997, #42083, #65019, #48815, #2261, #25516, #71362, #36058, #47707, #19500, #65385, #18759, #41697, #60125, #64277, #59003, #8607, #31520, #54458, #2991, #47347, #13121, #30406, #10076, #61228, #43206, #9329, #31891, #15338, #38660, #16092, #49555, #32629, #8969, #61967, #27743, #21726, #10447, #26249, #50667, #72480, #55943, #3724, #32255, #39029, #26622, #44682, #4463, #37918, #38283, #4843, #20984, #67599, #55203, #73595, #43936, #60488, #43576, #20622, #15725, #9711, #66853, #21339, #55574, #33365, #72113, #14604, #4093, #3356, #66129, #72839, #26987, #37556, #56326, #54831, #61592, #66494, #14976, #32999, #67227, #49188, #60848, #49922, #44297, #27357, #50293, #73225, #51408, #11926, #6310, #68352, #5577, #28472, #55648, #28108, #51045, #57807, #6666, #16848, #23229, #34123, #46155, #40888, #11196, #73968, #57070, #63452, #40141, #22106, #62728, #10832, #68724, #17573, #69443, #22863, #11553, #62349, #63824, #29572, #696, #12297, #5208, #52514, #45801, #34872, #17209, #63096, #17946, #34489, #23586, #29213, #39779, #57432, #58168, #5949, #46517, #28858, #45046, #51787, #39402, #22483, #45425, #69087, #336, #40505, #52151, #35235, #67972, #16466, #33753, #56705, #35597, #61034, #30689, #53269, #69808, #66679, #1069, #71931, #24329, #29953, #66322, #9156, #18670 ),
 ( #37743, #14796, #49378, #49001, #9531, #32079, #64552, #55017, #60676, #3547, #13408, #20446, #43401, #59282, #1444, #26448, #64191, #52903, #72309, #20808, #12665, #41252, #13030, #58920, #47265, #58531, #70533, #23964, #32452, #43760, #41613, #7027, #46900, #3182, #1806, #18309, #70168, #35968, #15162, #19043, #24692, #53636, #7410, #38101, #30325, #47624, #41997, #64933, #36337, #26073, #7774, #49737, #45620, #55393, #50858, #4283, #9896, #45238, #62539, #73032, #73414, #11376, #27172, #5025, #56136, #50102, #21538, #5396, #27930, #27556, #73783, #33944, #44113, #61785, #11016, #56890, #62920, #22296, #16279, #72661, #44499, #10269, #3912, #68159, #33562, #39593, #26812, #16656, #4654, #28292, #50491, #21166, #44867, #51230, #55766, #67037, #67414, #15912, #17028, #21922, #67789, #15540, #39223, #74159, #38477, #61416, #32814, #62153, #33191, #10640, #39964, #56521, #22674, #68544, #38845, #17756, #40703, #12116, #40325, #63272, #69991, #18860, #6134, #35423, #46340, #58352, #53088, #23410, #11734, #69270, #1263, #52337, #34308, #517, #23049, #6495, #29764, #7227, #63645, #23774, #159, #1628, #41799, #12848, #24511, #17393, #64745, #35057, #47087, #57989, #29394, #30143, #886, #35777, #18494, #29038, #46711, #70350, #69637, #58730, #18135, #57254, #41076, #64010, #12486, #6851, #52716, #64375, #45979, #24157, #34679, #68905, #47447, #5760, #41434, #28663, #51604, #57630, #51970, #26357, #59845, #9065, #54564, #1989, #37652, #70729, #60226, #8332, #7594, #66228, #48184, #71464, #24879, #71095, #31255, #25983, #19600, #42546, #13228, #30508, #54929, #20347, #48911, #31619, #25260, #19966, #65119, #14703, #60588, #31988, #47810, #65488, #13951, #3091, #54204, #71836, #2731, #3454, #65851, #43307, #25616, #30875, #19233, #53819, #42187, #43672, #49285, #36159, #20716, #48552, #13593, #36894, #14339, #72212, #59104, #42921, #8702, #53452, #36523, #37287, #59469, #7954, #2368, #73320, #22206, #27839, #72935, #28210, #16559, #56043, #32360, #50395, #50766, #21440, #10926, #49647, #16190, #73695, #56427, #39509, #39130, #51140, #45146, #55674, #68068, #62451, #4936, #4559, #62065, #10542, #21829, #66944, #33853, #55302, #21075, #56799, #5310, #3821, #26715, #4191, #50013, #15442, #72576, #61691, #66592 ) ),
 .UNSPECIFIED., .F., .F., .F. ) 
 B_SPLINE_SURFACE_WITH_KNOTS ( ( 2, 2 ),
 ( 3, 2, 2, 2, 2, 2, 2, 2, 2, 2, 2, 2, 2, 2, 2, 2, 2, 2, 2, 2, 2, 2, 2, 2, 2, 2, 2, 2, 2, 2, 2, 2, 2, 2, 2, 2, 2, 2, 2, 2, 2, 2, 2, 2, 2, 2, 2, 2, 2, 2, 2, 2, 2, 2, 2, 2, 2, 2, 2, 2, 2, 2, 2, 2, 2, 2, 2, 2, 2, 2, 2, 2, 2, 2, 2, 2, 2, 2, 2, 2, 2, 2, 2, 2, 2, 2, 2, 2, 2, 2, 2, 2, 2, 2, 2, 2, 2, 2, 2, 2, 2, 2, 2, 2, 2, 2, 2, 2, 2, 2, 2, 2, 2, 2, 2, 2, 2, 2, 2, 2, 2, 2, 2, 2, 2, 2, 2, 2, 2, 2, 2, 2, 2, 2, 2, 2, 2, 2, 2, 2, 2, 2, 3 ),
 ( 0.000000000000000000, 1.000000000000000000 ),
 ( 0.000000000000000000, 0.006944444444444444059, 0.01388888888888888812, 0.02083333333333333218, 0.02777777777777777624, 0.03472222222222222376, 0.04166666666666666435, 0.04861111111111111188, 0.05555555555555555247, 0.06250000000000000000, 0.06944444444444444753, 0.07638888888888889506, 0.08333333333333332871, 0.09027777777777777624, 0.09722222222222222376, 0.1041666666666666713, 0.1111111111111111049, 0.1180555555555555525, 0.1250000000000000000, 0.1319444444444444475, 0.1388888888888888951, 0.1458333333333333426, 0.1527777777777777901, 0.1597222222222222099, 0.1666666666666666574, 0.1736111111111111049, 0.1805555555555555525, 0.1875000000000000000, 0.1944444444444444475, 0.2013888888888888951, 0.2083333333333333426, 0.2152777777777777901, 0.2222222222222222099, 0.2291666666666666574, 0.2361111111111111049, 0.2430555555555555525, 0.2500000000000000000, 0.2569444444444444198, 0.2638888888888888951, 0.2708333333333333148, 0.2777777777777777901, 0.2847222222222222099, 0.2916666666666666852, 0.2986111111111111049, 0.3055555555555555802, 0.3125000000000000000, 0.3194444444444444198, 0.3263888888888888951, 0.3333333333333333148, 0.3402777777777777901, 0.3472222222222222099, 0.3541666666666666852, 0.3611111111111111049, 0.3680555555555555802, 0.3750000000000000000, 0.3819444444444444198, 0.3888888888888888951, 0.3958333333333333148, 0.4027777777777777901, 0.4097222222222222099, 0.4166666666666666852, 0.4236111111111111049, 0.4305555555555555802, 0.4375000000000000000, 0.4444444444444444198, 0.4513888888888888951, 0.4583333333333333148, 0.4652777777777777901, 0.4722222222222222099, 0.4791666666666666852, 0.4861111111111111049, 0.4930555555555555802, 0.5000000000000000000, 0.5069444444444444198, 0.5138888888888888395, 0.5208333333333333703, 0.5277777777777777901, 0.5347222222222222099, 0.5416666666666666297, 0.5486111111111111605, 0.5555555555555555802, 0.5625000000000000000, 0.5694444444444444198, 0.5763888888888888395, 0.5833333333333333703, 0.5902777777777777901, 0.5972222222222222099, 0.6041666666666666297, 0.6111111111111111605, 0.6180555555555555802, 0.6250000000000000000, 0.6319444444444444198, 0.6388888888888888395, 0.6458333333333333703, 0.6527777777777777901, 0.6597222222222222099, 0.6666666666666666297, 0.6736111111111111605, 0.6805555555555555802, 0.6875000000000000000, 0.6944444444444444198, 0.7013888888888888395, 0.7083333333333333703, 0.7152777777777777901, 0.7222222222222222099, 0.7291666666666666297, 0.7361111111111111605, 0.7430555555555555802, 0.7500000000000000000, 0.7569444444444444198, 0.7638888888888888395, 0.7708333333333333703, 0.7777777777777777901, 0.7847222222222222099, 0.7916666666666666297, 0.7986111111111111605, 0.8055555555555555802, 0.8125000000000000000, 0.8194444444444444198, 0.8263888888888888395, 0.8333333333333333703, 0.8402777777777777901, 0.8472222222222222099, 0.8541666666666666297, 0.8611111111111111605, 0.8680555555555555802, 0.8750000000000000000, 0.8819444444444444198, 0.8888888888888888395, 0.8958333333333333703, 0.9027777777777777901, 0.9097222222222222099, 0.9166666666666666297, 0.9236111111111111605, 0.9305555555555555802, 0.9375000000000000000, 0.9444444444444444198, 0.9513888888888888395, 0.9583333333333333703, 0.9652777777777777901, 0.9722222222222222099, 0.9791666666666666297, 0.9842226981114289286 ),
 .UNSPECIFIED. ) 
 GEOMETRIC_REPRESENTATION_ITEM ( )  RATIONAL_B_SPLINE_SURFACE ( (
 ( 1.000000000000000000, 0.8660254037844387076, 1.000000000000000000, 0.8660254037844387076, 1.000000000000000000, 0.8660254037844387076, 1.000000000000000000, 0.8660254037844387076, 1.000000000000000000, 0.8660254037844387076, 1.000000000000000000, 0.8660254037844387076, 1.000000000000000000, 0.8660254037844387076, 1.000000000000000000, 0.8660254037844387076, 1.000000000000000000, 0.8660254037844387076, 1.000000000000000000, 0.8660254037844387076, 1.000000000000000000, 0.8660254037844387076, 1.000000000000000000, 0.8660254037844387076, 1.000000000000000000, 0.8660254037844387076, 1.000000000000000000, 0.8660254037844387076, 1.000000000000000000, 0.8660254037844387076, 1.000000000000000000, 0.8660254037844387076, 1.000000000000000000, 0.8660254037844387076, 1.000000000000000000, 0.8660254037844387076, 1.000000000000000000, 0.8660254037844387076, 1.000000000000000000, 0.8660254037844387076, 1.000000000000000000, 0.8660254037844387076, 1.000000000000000000, 0.8660254037844387076, 1.000000000000000000, 0.8660254037844387076, 1.000000000000000000, 0.8660254037844387076, 1.000000000000000000, 0.8660254037844387076, 1.000000000000000000, 0.8660254037844387076, 1.000000000000000000, 0.8660254037844387076, 1.000000000000000000, 0.8660254037844387076, 1.000000000000000000, 0.8660254037844387076, 1.000000000000000000, 0.8660254037844387076, 1.000000000000000000, 0.8660254037844387076, 1.000000000000000000, 0.8660254037844387076, 1.000000000000000000, 0.8660254037844387076, 1.000000000000000000, 0.8660254037844387076, 1.000000000000000000, 0.8660254037844387076, 1.000000000000000000, 0.8660254037844387076, 1.000000000000000000, 0.8660254037844387076, 1.000000000000000000, 0.8660254037844387076, 1.000000000000000000, 0.8660254037844387076, 1.000000000000000000, 0.8660254037844387076, 1.000000000000000000, 0.8660254037844387076, 1.000000000000000000, 0.8660254037844387076, 1.000000000000000000, 0.8660254037844387076, 1.000000000000000000, 0.8660254037844387076, 1.000000000000000000, 0.8660254037844387076, 1.000000000000000000, 0.8660254037844387076, 1.000000000000000000, 0.8660254037844387076, 1.000000000000000000, 0.8660254037844387076, 1.000000000000000000, 0.8660254037844387076, 1.000000000000000000, 0.8660254037844387076, 1.000000000000000000, 0.8660254037844387076, 1.000000000000000000, 0.8660254037844387076, 1.000000000000000000, 0.8660254037844387076, 1.000000000000000000, 0.8660254037844387076, 1.000000000000000000, 0.8660254037844387076, 1.000000000000000000, 0.8660254037844387076, 1.000000000000000000, 0.8660254037844387076, 1.000000000000000000, 0.8660254037844387076, 1.000000000000000000, 0.8660254037844387076, 1.000000000000000000, 0.8660254037844387076, 1.000000000000000000, 0.8660254037844387076, 1.000000000000000000, 0.8660254037844387076, 1.000000000000000000, 0.8660254037844387076, 1.000000000000000000, 0.8660254037844387076, 1.000000000000000000, 0.8660254037844387076, 1.000000000000000000, 0.8660254037844387076, 1.000000000000000000, 0.8660254037844387076, 1.000000000000000000, 0.8660254037844387076, 1.000000000000000000, 0.8660254037844387076, 1.000000000000000000, 0.8660254037844387076, 1.000000000000000000, 0.8660254037844387076, 1.000000000000000000, 0.8660254037844387076, 1.000000000000000000, 0.8660254037844387076, 1.000000000000000000, 0.8660254037844387076, 1.000000000000000000, 0.8660254037844387076, 1.000000000000000000, 0.8660254037844387076, 1.000000000000000000, 0.8660254037844387076, 1.000000000000000000, 0.8660254037844387076, 1.000000000000000000, 0.8660254037844387076, 1.000000000000000000, 0.8660254037844387076, 1.000000000000000000, 0.8660254037844387076, 1.000000000000000000, 0.8660254037844387076, 1.000000000000000000, 0.8660254037844387076, 1.000000000000000000, 0.8660254037844387076, 1.000000000000000000, 0.8660254037844387076, 1.000000000000000000, 0.8660254037844387076, 1.000000000000000000, 0.8660254037844387076, 1.000000000000000000, 0.8660254037844387076, 1.000000000000000000, 0.8660254037844387076, 1.000000000000000000, 0.8660254037844387076, 1.000000000000000000, 0.8660254037844387076, 1.000000000000000000, 0.8660254037844387076, 1.000000000000000000, 0.8660254037844387076, 1.000000000000000000, 0.8660254037844387076, 1.000000000000000000, 0.8660254037844387076, 1.000000000000000000, 0.8660254037844387076, 1.000000000000000000, 0.8660254037844387076, 1.000000000000000000, 0.8660254037844387076, 1.000000000000000000, 0.8660254037844387076, 1.000000000000000000, 0.8660254037844387076, 1.000000000000000000, 0.8660254037844387076, 1.000000000000000000, 0.8660254037844387076, 1.000000000000000000, 0.8660254037844387076, 1.000000000000000000, 0.8660254037844387076, 1.000000000000000000, 0.8660254037844387076, 1.000000000000000000, 0.8660254037844387076, 1.000000000000000000, 0.8660254037844387076, 1.000000000000000000, 0.8660254037844387076, 1.000000000000000000, 0.8660254037844387076, 1.000000000000000000, 0.8660254037844387076, 1.000000000000000000, 0.8660254037844387076, 1.000000000000000000, 0.8660254037844387076, 1.000000000000000000, 0.8660254037844387076, 1.000000000000000000, 0.8660254037844387076, 1.000000000000000000, 0.8660254037844387076, 1.000000000000000000, 0.8660254037844387076, 1.000000000000000000, 0.8660254037844387076, 1.000000000000000000, 0.8660254037844387076, 1.000000000000000000, 0.8660254037844387076, 1.000000000000000000, 0.8660254037844387076, 1.000000000000000000, 0.8660254037844387076, 1.000000000000000000, 0.8660254037844387076, 1.000000000000000000, 0.8660254037844387076, 1.000000000000000000, 0.8660254037844387076, 1.000000000000000000, 0.8660254037844387076, 1.000000000000000000, 0.8660254037844387076, 1.000000000000000000, 0.8660254037844387076, 1.000000000000000000, 0.8660254037844387076, 1.000000000000000000, 0.8660254037844387076, 1.000000000000000000, 0.8660254037844387076, 1.000000000000000000, 0.8660254037844387076, 1.000000000000000000, 0.8660254037844387076, 1.000000000000000000, 0.8660254037844387076, 1.000000000000000000, 0.8660254037844387076, 1.000000000000000000, 0.8660254037844387076, 1.000000000000000000, 0.8660254037844387076, 1.000000000000000000, 0.8660254037844387076, 1.000000000000000000, 0.8660254037844387076, 1.000000000000000000, 0.8660254037844387076, 1.000000000000000000, 0.8660254037844387076, 1.000000000000000000, 0.8660254037844387076, 1.000000000000000000, 0.9024573129378109515, 0.9469501470576147106),
 ( 1.000000000000000000, 0.8660254037844387076, 1.000000000000000000, 0.8660254037844387076, 1.000000000000000000, 0.8660254037844387076, 1.000000000000000000, 0.8660254037844387076, 1.000000000000000000, 0.8660254037844387076, 1.000000000000000000, 0.8660254037844387076, 1.000000000000000000, 0.8660254037844387076, 1.000000000000000000, 0.8660254037844387076, 1.000000000000000000, 0.8660254037844387076, 1.000000000000000000, 0.8660254037844387076, 1.000000000000000000, 0.8660254037844387076, 1.000000000000000000, 0.8660254037844387076, 1.000000000000000000, 0.8660254037844387076, 1.000000000000000000, 0.8660254037844387076, 1.000000000000000000, 0.8660254037844387076, 1.000000000000000000, 0.8660254037844387076, 1.000000000000000000, 0.8660254037844387076, 1.000000000000000000, 0.8660254037844387076, 1.000000000000000000, 0.8660254037844387076, 1.000000000000000000, 0.8660254037844387076, 1.000000000000000000, 0.8660254037844387076, 1.000000000000000000, 0.8660254037844387076, 1.000000000000000000, 0.8660254037844387076, 1.000000000000000000, 0.8660254037844387076, 1.000000000000000000, 0.8660254037844387076, 1.000000000000000000, 0.8660254037844387076, 1.000000000000000000, 0.8660254037844387076, 1.000000000000000000, 0.8660254037844387076, 1.000000000000000000, 0.8660254037844387076, 1.000000000000000000, 0.8660254037844387076, 1.000000000000000000, 0.8660254037844387076, 1.000000000000000000, 0.8660254037844387076, 1.000000000000000000, 0.8660254037844387076, 1.000000000000000000, 0.8660254037844387076, 1.000000000000000000, 0.8660254037844387076, 1.000000000000000000, 0.8660254037844387076, 1.000000000000000000, 0.8660254037844387076, 1.000000000000000000, 0.8660254037844387076, 1.000000000000000000, 0.8660254037844387076, 1.000000000000000000, 0.8660254037844387076, 1.000000000000000000, 0.8660254037844387076, 1.000000000000000000, 0.8660254037844387076, 1.000000000000000000, 0.8660254037844387076, 1.000000000000000000, 0.8660254037844387076, 1.000000000000000000, 0.8660254037844387076, 1.000000000000000000, 0.8660254037844387076, 1.000000000000000000, 0.8660254037844387076, 1.000000000000000000, 0.8660254037844387076, 1.000000000000000000, 0.8660254037844387076, 1.000000000000000000, 0.8660254037844387076, 1.000000000000000000, 0.8660254037844387076, 1.000000000000000000, 0.8660254037844387076, 1.000000000000000000, 0.8660254037844387076, 1.000000000000000000, 0.8660254037844387076, 1.000000000000000000, 0.8660254037844387076, 1.000000000000000000, 0.8660254037844387076, 1.000000000000000000, 0.8660254037844387076, 1.000000000000000000, 0.8660254037844387076, 1.000000000000000000, 0.8660254037844387076, 1.000000000000000000, 0.8660254037844387076, 1.000000000000000000, 0.8660254037844387076, 1.000000000000000000, 0.8660254037844387076, 1.000000000000000000, 0.8660254037844387076, 1.000000000000000000, 0.8660254037844387076, 1.000000000000000000, 0.8660254037844387076, 1.000000000000000000, 0.8660254037844387076, 1.000000000000000000, 0.8660254037844387076, 1.000000000000000000, 0.8660254037844387076, 1.000000000000000000, 0.8660254037844387076, 1.000000000000000000, 0.8660254037844387076, 1.000000000000000000, 0.8660254037844387076, 1.000000000000000000, 0.8660254037844387076, 1.000000000000000000, 0.8660254037844387076, 1.000000000000000000, 0.8660254037844387076, 1.000000000000000000, 0.8660254037844387076, 1.000000000000000000, 0.8660254037844387076, 1.000000000000000000, 0.8660254037844387076, 1.000000000000000000, 0.8660254037844387076, 1.000000000000000000, 0.8660254037844387076, 1.000000000000000000, 0.8660254037844387076, 1.000000000000000000, 0.8660254037844387076, 1.000000000000000000, 0.8660254037844387076, 1.000000000000000000, 0.8660254037844387076, 1.000000000000000000, 0.8660254037844387076, 1.000000000000000000, 0.8660254037844387076, 1.000000000000000000, 0.8660254037844387076, 1.000000000000000000, 0.8660254037844387076, 1.000000000000000000, 0.8660254037844387076, 1.000000000000000000, 0.8660254037844387076, 1.000000000000000000, 0.8660254037844387076, 1.000000000000000000, 0.8660254037844387076, 1.000000000000000000, 0.8660254037844387076, 1.000000000000000000, 0.8660254037844387076, 1.000000000000000000, 0.8660254037844387076, 1.000000000000000000, 0.8660254037844387076, 1.000000000000000000, 0.8660254037844387076, 1.000000000000000000, 0.8660254037844387076, 1.000000000000000000, 0.8660254037844387076, 1.000000000000000000, 0.8660254037844387076, 1.000000000000000000, 0.8660254037844387076, 1.000000000000000000, 0.8660254037844387076, 1.000000000000000000, 0.8660254037844387076, 1.000000000000000000, 0.8660254037844387076, 1.000000000000000000, 0.8660254037844387076, 1.000000000000000000, 0.8660254037844387076, 1.000000000000000000, 0.8660254037844387076, 1.000000000000000000, 0.8660254037844387076, 1.000000000000000000, 0.8660254037844387076, 1.000000000000000000, 0.8660254037844387076, 1.000000000000000000, 0.8660254037844387076, 1.000000000000000000, 0.8660254037844387076, 1.000000000000000000, 0.8660254037844387076, 1.000000000000000000, 0.8660254037844387076, 1.000000000000000000, 0.8660254037844387076, 1.000000000000000000, 0.8660254037844387076, 1.000000000000000000, 0.8660254037844387076, 1.000000000000000000, 0.8660254037844387076, 1.000000000000000000, 0.8660254037844387076, 1.000000000000000000, 0.8660254037844387076, 1.000000000000000000, 0.8660254037844387076, 1.000000000000000000, 0.8660254037844387076, 1.000000000000000000, 0.8660254037844387076, 1.000000000000000000, 0.8660254037844387076, 1.000000000000000000, 0.8660254037844387076, 1.000000000000000000, 0.8660254037844387076, 1.000000000000000000, 0.8660254037844387076, 1.000000000000000000, 0.8660254037844387076, 1.000000000000000000, 0.8660254037844387076, 1.000000000000000000, 0.8660254037844387076, 1.000000000000000000, 0.8660254037844387076, 1.000000000000000000, 0.8660254037844387076, 1.000000000000000000, 0.8660254037844387076, 1.000000000000000000, 0.8660254037844387076, 1.000000000000000000, 0.8660254037844387076, 1.000000000000000000, 0.8660254037844387076, 1.000000000000000000, 0.8660254037844387076, 1.000000000000000000, 0.8660254037844387076, 1.000000000000000000, 0.8660254037844387076, 1.000000000000000000, 0.8660254037844387076, 1.000000000000000000, 0.8660254037844387076, 1.000000000000000000, 0.8660254037844387076, 1.000000000000000000, 0.9024573129378109515, 0.9469501470576147106) ) ) 
 REPRESENTATION_ITEM ( '' )  SURFACE ( )  );
#17187=CARTESIAN_POINT ( 'NONE',  ( 97.30629616937498838, -208.6684592857803011, 76.83697916753382628 ) ) ;
#17191=CARTESIAN_POINT ( 'NONE',  ( 97.30629616937498838, -208.6684592857803295, 86.36197916753383197 ) ) ;
#17193=LINE ( 'NONE', #67583, #47151 ) ;
#17199=CARTESIAN_POINT ( 'NONE',  ( 97.64999999999997726, -208.4700217866474645, 87.83041666666666458 ) ) ;
#17203=ORIENTED_EDGE ( 'NONE', *, *, #6945, .T. ) ;
#17209=CARTESIAN_POINT ( 'NONE',  ( 97.64999999999999147, -209.9999999999999716, 76.42687500173430237 ) ) ;
#17210=CARTESIAN_POINT ( 'NONE',  ( 92.34999999999999432, 88.47002178664753558, 79.25791666666665947 ) ) ;
#17212=FACE_OUTER_BOUND ( 'NONE', #44016, .T. ) ;
#17216=CARTESIAN_POINT ( 'NONE',  ( 97.64999999994533653, -210.0000170172949367, 88.49187441316098557 ) ) ;
#17217=CARTESIAN_POINT ( 'NONE',  ( -95.00000000000002842, 92.66308142843932671, 82.65781250086715204 ) ) ;
#17218=CARTESIAN_POINT ( 'NONE',  ( 94.99999999999998579, 92.66308142843935514, 77.41906250086714181 ) ) ;
#17223=EDGE_CURVE ( 'NONE', #59860, #7101, #19144, .T. ) ;
#17227=CARTESIAN_POINT ( 'NONE',  ( -97.30629616937497417, -211.3315407142195852, 77.63072916753380071 ) ) ;
#17232=EDGE_CURVE ( 'NONE', #58994, #19312, #34515, .T. ) ;
#17235=DIRECTION ( 'NONE',  ( -0.000000000000000000, -0.000000000000000000, 1.000000000000000000 ) ) ;
#17240=CARTESIAN_POINT ( 'NONE',  ( -97.30629616937497417, -208.6684592857803011, 75.61989583420047722 ) ) ;
#17246=CARTESIAN_POINT ( 'NONE',  ( -96.15314808468747287, -208.0026889286704943, 76.20197916753380696 ) ) ;
#17247=CARTESIAN_POINT ( 'NONE',  ( -92.35000000010070664, 90.00002309722640348, 83.41187580057902551 ) ) ;
#17250=CARTESIAN_POINT ( 'NONE',  ( 93.84685191531248449, 88.00268892867053694, 85.93864583420048575 ) ) ;
#17263=CARTESIAN_POINT ( 'NONE',  ( -96.15314808468752972, 91.99731107132950569, 88.90197916753380980 ) ) ;
#17273=LINE ( 'NONE', #52216, #74024 ) ;
#17274=CARTESIAN_POINT ( 'NONE',  ( 93.84685191531251292, -211.9973110713294489, 84.19239583420049655 ) ) ;
#17277=CARTESIAN_POINT ( 'NONE',  ( -97.65000000000001990, 90.00000000000004263, 90.00000000000000000 ) ) ;
#17278=ORIENTED_EDGE ( 'NONE', *, *, #42102, .T. ) ;
#17281=CARTESIAN_POINT ( 'NONE',  ( 97.30629616937498838, -208.6684592857803295, 77.31322916753380525 ) ) ;
#17283=CARTESIAN_POINT ( 'NONE',  ( 95.00000000000000000, -207.3369185715606307, 83.29281250086717137 ) ) ;
#17285=CARTESIAN_POINT ( 'NONE',  ( -93.67499999999998295, -212.2949673200287179, 88.30666666666665776 ) ) ;
#17286=ORIENTED_EDGE ( 'NONE', *, *, #23694, .T. ) ;
#17291=ORIENTED_EDGE ( 'NONE', *, *, #12366, .T. ) ;
#17292=CYLINDRICAL_SURFACE ( 'NONE', #46122, 2.649999999999985700 ) ;
#17293=CARTESIAN_POINT ( 'NONE',  ( 92.35000000000002274, -208.4700217866474645, 88.12145833506762926 ) ) ;
#17301=ADVANCED_FACE ( 'NONE', ( #74253 ), #50578, .F. ) ;
#17302=EDGE_CURVE ( 'NONE', #51617, #17407, #29481, .T. ) ;
#17312=ORIENTED_EDGE ( 'NONE', *, *, #9518, .F. ) ;
#17313=CARTESIAN_POINT ( 'NONE',  ( 92.35000000000000853, -209.9999999999999716, 76.03000000000000114 ) ) ;
#17314=DIRECTION ( 'NONE',  ( -0.000000000000000000, -0.000000000000000000, 1.000000000000000000 ) ) ;
#17316=CARTESIAN_POINT ( 'NONE',  ( -97.65000000000001990, 91.52997821335253548, 86.77208333333334167 ) ) ;
#17322=CARTESIAN_POINT ( 'NONE',  ( -94.99999999999997158, -212.6630814284392557, 87.26156250086714294 ) ) ;
#17324=ORIENTED_EDGE ( 'NONE', *, *, #11964, .F. ) ;
#17327=CARTESIAN_POINT ( 'NONE',  ( 93.67500000000001137, -207.7050326799711968, 87.98916666666666231 ) ) ;
#17328=CARTESIAN_POINT ( 'NONE',  ( -93.84685191531247028, -211.9973110713294489, 75.24947916753380639 ) ) ;
#17337=CARTESIAN_POINT ( 'NONE',  ( -97.30629616937501680, 90.00000000000004263, 78.84781250086714977 ) ) ;
#17342=CYLINDRICAL_SURFACE ( 'NONE', #53321, 2.649999999999985700 ) ;
#17343=CARTESIAN_POINT ( 'NONE',  ( 92.35002600474523149, -211.5299932271990428, 86.32229270695526679 ) ) ;
#17346=VECTOR ( 'NONE', #7026, 1000.000000000000000 ) ;
#17349=CARTESIAN_POINT ( 'NONE',  ( -94.99999999999997158, -207.3369185715606307, 75.03781250086714749 ) ) ;
#17362=ORIENTED_EDGE ( 'NONE', *, *, #41607, .F. ) ;
#17367=CARTESIAN_POINT ( 'NONE',  ( 97.30629616937498838, -209.9999999999999716, 89.32531250086714181 ) ) ;
#17372=EDGE_LOOP ( 'NONE', ( #73593, #42343 ) ) ;
#17374=ORIENTED_EDGE ( 'NONE', *, *, #10449, .T. ) ;
#17377=FACE_OUTER_BOUND ( 'NONE', #70090, .T. ) ;
#17379=ADVANCED_FACE ( 'NONE', ( #73131 ), #73879, .F. ) ;
#17381=CARTESIAN_POINT ( 'NONE',  ( 1.243286885786405054E-17, -120.0000000000000000, 127.5000000000000000 ) ) ;
#17386=( BOUNDED_CURVE ( )  B_SPLINE_CURVE ( 2, ( #30991, #25733, #43038, #71584, #43423, #26095, #37015 ),
 .UNSPECIFIED., .F., .F. ) 
 B_SPLINE_CURVE_WITH_KNOTS ( ( 3, 2, 2, 3 ),
 ( 0.6458333333333334814, 0.6527777777777779011, 0.6597222222222223209, 0.6666666666666667407 ),
 .UNSPECIFIED. ) 
 CURVE ( )  GEOMETRIC_REPRESENTATION_ITEM ( )  RATIONAL_B_SPLINE_CURVE ( ( 0.9999999999999978906, 0.8660254037844408170, 1.000000000000000000, 0.8660254037844387076, 1.000000000000000000, 0.8660254037844365982, 1.000000000000002220 ) ) 
 REPRESENTATION_ITEM ( '' )  );
#17391=CARTESIAN_POINT ( 'NONE',  ( 97.30629616937498838, 90.00000000000002842, 86.15031250086714465 ) ) ;
#17393=CARTESIAN_POINT ( 'NONE',  ( 92.69370383062501162, -208.6684592857803011, 81.96989583420048575 ) ) ;
#17397=CARTESIAN_POINT ( 'NONE',  ( 97.64999999999999147, 90.00000000000002842, 85.87249999999998806 ) ) ;
#17402=CARTESIAN_POINT ( 'NONE',  ( -93.84685191531248449, -208.0026889286704943, 84.35114583420048007 ) ) ;
#17403=CARTESIAN_POINT ( 'NONE',  ( -93.84685191531254134, 91.99731107132950569, 81.96989583420048575 ) ) ;
#17405=CARTESIAN_POINT ( 'NONE',  ( 94.99999999999998579, 87.33691857156068750, 84.72156250086713669 ) ) ;
#17406=CARTESIAN_POINT ( 'NONE',  ( -92.69370383062502583, 91.33154071421968467, 84.93322916753379559 ) ) ;
#17407=VERTEX_POINT ( 'NONE', #46430 ) ;
#17413=FACE_OUTER_BOUND ( 'NONE', #56316, .T. ) ;
#17414=CARTESIAN_POINT ( 'NONE',  ( 97.65000000000003411, -208.4700217866474929, 85.29041666666665833 ) ) ;
#17415=CARTESIAN_POINT ( 'NONE',  ( -94.99999999999997158, -207.3369185715606307, 86.30906250086714238 ) ) ;
#17417=LINE ( 'NONE', #28689, #53007 ) ;
#17424=CARTESIAN_POINT ( 'NONE',  ( -93.67500000000003979, 92.29496732002878900, 79.62833333333333030 ) ) ;
#17428=CARTESIAN_POINT ( 'NONE',  ( -94.22990255303811580, -207.7668333712727531, 74.81945665767622700 ) ) ;
#17429=CARTESIAN_POINT ( 'NONE',  ( -95.00000000000002842, 93.05995642670504253, 79.76062500173429726 ) ) ;
#17435=CARTESIAN_POINT ( 'NONE',  ( -95.00000000000002842, 92.66308142843932671, 79.95906250086713385 ) ) ;
#17442=CARTESIAN_POINT ( 'NONE',  ( -92.35000000000179909, 90.00000306648279036, 75.79187510780352000 ) ) ;
#17443=CARTESIAN_POINT ( 'NONE',  ( -97.30629616937497417, -211.3315407142195852, 88.58447916753382856 ) ) ;
#17444=CARTESIAN_POINT ( 'NONE',  ( 92.69370383062498320, 88.66845928578035796, 75.88447916753382572 ) ) ;
#17445=CARTESIAN_POINT ( 'NONE',  ( -94.99999999999997158, -207.3369185715606307, 78.21281250086717307 ) ) ;
#17448=CARTESIAN_POINT ( 'NONE',  ( 92.34999999999999432, 88.47002178664752137, 87.59229166840096070 ) ) ;
#17450=CARTESIAN_POINT ( 'NONE',  ( 97.64999999946594755, -209.9999467985095976, 78.96687695417307395 ) ) ;
#17451=AXIS2_PLACEMENT_3D ( 'NONE', #14801, #3187, #70447 ) ;
#17452=CARTESIAN_POINT ( 'NONE',  ( -93.84685191531254134, 91.99731107132950569, 75.61989583420049144 ) ) ;
#17453=CARTESIAN_POINT ( 'NONE',  ( 93.84685191531251292, -211.9973110713294489, 75.77864583420047495 ) ) ;
#17457=ORIENTED_EDGE ( 'NONE', *, *, #67815, .F. ) ;
#17459=DIRECTION ( 'NONE',  ( -0.000000000000000000, -0.000000000000000000, 1.000000000000000000 ) ) ;
#17464=EDGE_LOOP ( 'NONE', ( #42096, #62076, #49672, #3098, #50951 ) ) ;
#17473=CARTESIAN_POINT ( 'NONE',  ( 97.30629616937498838, 91.33154071421968467, 84.45697916753383083 ) ) ;
#17474=DIRECTION ( 'NONE',  ( -0.000000000000000000, -0.000000000000000000, -1.000000000000000000 ) ) ;
#17477=ADVANCED_FACE ( 'NONE', ( #41900 ), #605, .F. ) ;
#17484=CARTESIAN_POINT ( 'NONE',  ( -93.67499999999998295, -207.7050326799711968, 85.34333333333333371 ) ) ;
#17487=CARTESIAN_POINT ( 'NONE',  ( 92.35000000000000853, -209.9999678301211361, 82.45937388908919274 ) ) ;
#17489=DIRECTION ( 'NONE',  ( -0.000000000000000000, -0.000000000000000000, 1.000000000000000000 ) ) ;
#17491=CARTESIAN_POINT ( 'NONE',  ( -92.34999999999999432, -209.9999999999999716, 82.77687500173431090 ) ) ;
#17495=CARTESIAN_POINT ( 'NONE',  ( 96.32499999999998863, 87.70503267997126784, 79.49604166840096298 ) ) ;
#17496=CARTESIAN_POINT ( 'NONE',  ( -96.32500000000001705, 92.29496732002878900, 81.08354166840096866 ) ) ;
#17497=ORIENTED_EDGE ( 'NONE', *, *, #5640, .T. ) ;
#17498=CARTESIAN_POINT ( 'NONE',  ( 92.69370383062498320, 88.66845928578037217, 79.69447916753381378 ) ) ;
#17502=CARTESIAN_POINT ( 'NONE',  ( -97.64998927488493052, 91.52998440550061332, 86.85145790673756494 ) ) ;
#17503=CARTESIAN_POINT ( 'NONE',  ( 96.32499999999997442, 92.29496732002878900, 81.61270833506763722 ) ) ;
#17505=DIRECTION ( 'NONE',  ( 1.000000000000000000, 0.000000000000000000, 0.000000000000000000 ) ) ;
#17506=CARTESIAN_POINT ( 'NONE',  ( 95.00000000000000000, -206.9400435732949575, 77.14124999999999943 ) ) ;
#17515=CARTESIAN_POINT ( 'NONE',  ( -93.84685191531248449, -208.0026889286704943, 78.15989583420049769 ) ) ;
#17523=CARTESIAN_POINT ( 'NONE',  ( 92.69370383062498320, 91.33154071421968467, 76.25489583420049655 ) ) ;
#17525=CARTESIAN_POINT ( 'NONE',  ( 97.64998213368511415, 88.47001147152583655, 78.27895762153869441 ) ) ;
#17533=CARTESIAN_POINT ( 'NONE',  ( 96.15314808468748708, 88.00268892867053694, 86.20322916753382003 ) ) ;
#17538=CARTESIAN_POINT ( 'NONE',  ( -97.30629616937501680, 90.00000000000004263, 80.75281250086715090 ) ) ;
#17540=CARTESIAN_POINT ( 'NONE',  ( 97.30629616937498838, -209.9999999999999716, 89.32531250086714181 ) ) ;
#17548=CARTESIAN_POINT ( 'NONE',  ( 96.15314808468750130, -211.9973110713294489, 76.04322916753382344 ) ) ;
#17552=EDGE_CURVE ( 'NONE', #60251, #42384, #52303, .T. ) ;
#17554=CARTESIAN_POINT ( 'NONE',  ( 97.30629616937498838, -209.9999999999999716, 82.49906250086715431 ) ) ;
#17561=CARTESIAN_POINT ( 'NONE',  ( 95.00000000000000000, -213.0599564267049857, 88.88875000000000171 ) ) ;
#17568=CARTESIAN_POINT ( 'NONE',  ( -97.30629616937501680, 91.33154071421968467, 87.20864583420049598 ) ) ;
#17572=CARTESIAN_POINT ( 'NONE',  ( 97.64999999981932888, -210.0000309431867436, 78.33187387208516839 ) ) ;
#17573=CARTESIAN_POINT ( 'NONE',  ( 97.64999999999997726, -208.4700217866474645, 77.11479166840095445 ) ) ;
#17574=CARTESIAN_POINT ( 'NONE',  ( 92.34999999999999432, 88.47002178664753558, 77.35291666666665833 ) ) ;
#17578=CARTESIAN_POINT ( 'NONE',  ( 95.00000000000000000, -209.9999999999999716, 90.00000000000000000 ) ) ;
#17583=CARTESIAN_POINT ( 'NONE',  ( -95.00000000000002842, 93.05995642670501411, 88.65062500173431204 ) ) ;
#17584=CARTESIAN_POINT ( 'NONE',  ( -92.69370383062504004, 90.00000000000004263, 80.59406250086715318 ) ) ;
#17585=CARTESIAN_POINT ( 'NONE',  ( 96.15314808468748708, 91.99731107132950569, 88.95489583420049939 ) ) ;
#17586=ADVANCED_FACE ( 'NONE', ( #36621 ), #14432, .F. ) ;
#17591=CARTESIAN_POINT ( 'NONE',  ( -97.64999999999997726, -210.0000225208801794, 86.26937578065384571 ) ) ;
#17595=CARTESIAN_POINT ( 'NONE',  ( -93.84685191531247028, -211.9973110713294489, 77.15447916753380753 ) ) ;
#17600=ORIENTED_EDGE ( 'NONE', *, *, #32172, .T. ) ;
#17605=CARTESIAN_POINT ( 'NONE',  ( -94.99999999999997158, -207.3369185715606307, 74.87906250086713555 ) ) ;
#17610=CARTESIAN_POINT ( 'NONE',  ( -97.64999999980591383, 89.99998015720542810, 86.27002759516649633 ) ) ;
#17616=CARTESIAN_POINT ( 'NONE',  ( 94.99999999999998579, 92.66308142843932671, 85.67406250086715147 ) ) ;
#17617=CARTESIAN_POINT ( 'NONE',  ( -97.64999999999986358, -211.5299782133525071, 83.70291666666668107 ) ) ;
#17624=( BOUNDED_CURVE ( )  B_SPLINE_CURVE ( 2, ( #48465, #60141, #37198, #43222, #71379, #47363, #31533 ),
 .UNSPECIFIED., .F., .F. ) 
 B_SPLINE_CURVE_WITH_KNOTS ( ( 3, 2, 2, 3 ),
 ( 0.7708333333333328152, 0.7777777777777775681, 0.7847222222222222099, 0.7916666666666669627 ),
 .UNSPECIFIED. ) 
 CURVE ( )  GEOMETRIC_REPRESENTATION_ITEM ( )  RATIONAL_B_SPLINE_CURVE ( ( 1.000000000000010658, 0.8660254037844280495, 1.000000000000000000, 0.8660254037844387076, 1.000000000000000000, 0.8660254037844322683, 1.000000000000006439 ) ) 
 REPRESENTATION_ITEM ( '' )  );
#17631=VECTOR ( 'NONE', #68262, 1000.000000000000000 ) ;
#17643=CARTESIAN_POINT ( 'NONE',  ( 92.69370383062501162, -211.3315407142195852, 84.77447916753381207 ) ) ;
#17650=FACE_OUTER_BOUND ( 'NONE', #42170, .T. ) ;
#17653=CARTESIAN_POINT ( 'NONE',  ( 93.84685191531249870, -208.0026889286704943, 76.20197916753380696 ) ) ;
#17655=CARTESIAN_POINT ( 'NONE',  ( 96.15314808468748708, -208.0026889286704943, 81.96989583420048575 ) ) ;
#17664=CARTESIAN_POINT ( 'NONE',  ( 97.64999999999997726, -208.4700217866474645, 86.00479166840096923 ) ) ;
#17679=ORIENTED_EDGE ( 'NONE', *, *, #23092, .F. ) ;
#17684=CARTESIAN_POINT ( 'NONE',  ( 26.49955575014745079, 0.001194404164630089764, -64.00000000000000000 ) ) ;
#17685=CARTESIAN_POINT ( 'NONE',  ( -96.32500000000001705, 92.29496732002878900, 88.62416666666665321 ) ) ;
#17688=CARTESIAN_POINT ( 'NONE',  ( 94.99999999999998579, 87.33691857156068750, 75.83156250086715033 ) ) ;
#17692=CARTESIAN_POINT ( 'NONE',  ( -92.69370383062498320, -211.3315407142195852, 85.46239583420047836 ) ) ;
#17694=CARTESIAN_POINT ( 'NONE',  ( -96.32499999999996021, -212.2949673200287179, 79.39020833506762642 ) ) ;
#17696=CARTESIAN_POINT ( 'NONE',  ( -94.99999999999997158, -212.6630814284392557, 75.83156250086715033 ) ) ;
#17703=CARTESIAN_POINT ( 'NONE',  ( 92.34999999999993747, 88.47002178664756400, 88.14791666666667425 ) ) ;
#17704=CARTESIAN_POINT ( 'NONE',  ( -92.69370383062504004, 90.00000000000004263, 78.53031250086714010 ) ) ;
#17708=CARTESIAN_POINT ( 'NONE',  ( -93.67499999999998295, -207.7050326799711968, 80.34270833506762699 ) ) ;
#17714=CARTESIAN_POINT ( 'NONE',  ( -94.99999999999997158, -206.9400435732949575, 89.84125000000000227 ) ) ;
#17728=CARTESIAN_POINT ( 'NONE',  ( -97.64999999999996305, -209.9999999999999716, 90.00000000000000000 ) ) ;
#17731=CARTESIAN_POINT ( 'NONE',  ( 97.30629616937498838, -208.6684592857803295, 85.56822916753380071 ) ) ;
#17732=CARTESIAN_POINT ( 'NONE',  ( -92.35001333515619137, -208.4700140875914371, 83.46479220096853169 ) ) ;
#17734=CARTESIAN_POINT ( 'NONE',  ( 93.67500000000001137, -212.2949673200287179, 89.47083333333333144 ) ) ;
#17736=CARTESIAN_POINT ( 'NONE',  ( 92.35000000000000853, -211.5299782133524218, 85.05229166840096866 ) ) ;
#17738=CARTESIAN_POINT ( 'NONE',  ( -95.00000000000002842, 87.33691857156074434, 79.80031250086715033 ) ) ;
#17742=VECTOR ( 'NONE', #9963, 1000.000000000000000 ) ;
#17748=ORIENTED_EDGE ( 'NONE', *, *, #19748, .F. ) ;
#17749=ORIENTED_EDGE ( 'NONE', *, *, #20208, .T. ) ;
#17754=CARTESIAN_POINT ( 'NONE',  ( 94.99999999999998579, 87.33691857156068750, 85.35656250086714181 ) ) ;
#17756=CARTESIAN_POINT ( 'NONE',  ( 97.30629616937498838, -211.3315407142195852, 83.55739583420047722 ) ) ;
#17763=CARTESIAN_POINT ( 'NONE',  ( 12.75000000000000000, -120.0000000000000000, -85.60000000000000853 ) ) ;
#17766=CARTESIAN_POINT ( 'NONE',  ( -96.15314808468745866, -211.9973110713294489, 82.76364583420047438 ) ) ;
#17767=CARTESIAN_POINT ( 'NONE',  ( -97.30629616937501680, 91.33154071421968467, 82.12864583420048348 ) ) ;
#17768=ORIENTED_EDGE ( 'NONE', *, *, #4967, .T. ) ;
#17769=CARTESIAN_POINT ( 'NONE',  ( 93.84685191531248449, 88.00268892867053694, 83.39864583420047950 ) ) ;
#17775=DIRECTION ( 'NONE',  ( -0.000000000000000000, -0.000000000000000000, 1.000000000000000000 ) ) ;
#17776=CARTESIAN_POINT ( 'NONE',  ( -92.69370383062498320, -209.9999999999999716, 86.78531250086714977 ) ) ;
#17785=CARTESIAN_POINT ( 'NONE',  ( -96.32500000000001705, 92.29496732002878900, 77.19416666666666060 ) ) ;
#17792=CARTESIAN_POINT ( 'NONE',  ( -97.30629616937501680, 88.66845928578038638, 78.26572916753380582 ) ) ;
#17799=CARTESIAN_POINT ( 'NONE',  ( -93.84685191531248449, -208.0026889286704943, 85.14489583420048291 ) ) ;
#17804=CARTESIAN_POINT ( 'NONE',  ( 96.32499999999998863, -207.7050326799711968, 79.07270833506763097 ) ) ;
#17806=AXIS2_PLACEMENT_3D ( 'NONE', #40204, #6371, #28916 ) ;
#17807=CARTESIAN_POINT ( 'NONE',  ( 92.69370383062498320, 90.00000000000002842, 75.83156250086716454 ) ) ;
#17808=EDGE_CURVE ( 'NONE', #37620, #69189, #8615, .T. ) ;
#17809=CARTESIAN_POINT ( 'NONE',  ( -92.69370383062498320, -211.3315407142195852, 78.00114583420049996 ) ) ;
#17810=LINE ( 'NONE', #30200, #68692 ) ;
#17814=FACE_OUTER_BOUND ( 'NONE', #37679, .T. ) ;
#17817=CARTESIAN_POINT ( 'NONE',  ( 95.00000000000000000, -212.6630814284392557, 78.37156250086714238 ) ) ;
#17821=( BOUNDED_CURVE ( )  B_SPLINE_CURVE ( 2, ( #46499, #12278, #13015, #24314, #41978, #17926, #46139 ),
 .UNSPECIFIED., .F., .F. ) 
 B_SPLINE_CURVE_WITH_KNOTS ( ( 3, 2, 2, 3 ),
 ( 0.000000000000000000, 0.006944444444444406762, 0.01388888888888881352, 0.02083333333333322115 ),
 .UNSPECIFIED. ) 
 CURVE ( )  GEOMETRIC_REPRESENTATION_ITEM ( )  RATIONAL_B_SPLINE_CURVE ( ( 1.000000000000000000, 0.8660254037844387076, 1.000000000000000000, 0.8660254037844387076, 1.000000000000000000, 0.8660254037844408170, 0.9999999999999978906 ) ) 
 REPRESENTATION_ITEM ( '' )  );
#17829=VECTOR ( 'NONE', #55708, 1000.000000000000000 ) ;
#17838=ORIENTED_EDGE ( 'NONE', *, *, #11068, .T. ) ;
#17839=CARTESIAN_POINT ( 'NONE',  ( 94.99999999999998579, 92.66308142843935514, 84.56281250086716739 ) ) ;
#17849=DIRECTION ( 'NONE',  ( -0.000000000000000000, -0.000000000000000000, 1.000000000000000000 ) ) ;
#17852=CARTESIAN_POINT ( 'NONE',  ( 97.65000000000000568, -211.5299782133524218, 87.16895833506762870 ) ) ;
#17855=B_SPLINE_CURVE_WITH_KNOTS ( 'NONE', 3,
 ( #48126, #65062, #30814, #68575, #2301, #1566, #59409, #47747 ),
 .UNSPECIFIED., .F., .F.,
 ( 4, 2, 2, 4 ),
 ( 0.001653806717454348388, 0.002539064216006851459, 0.002981692965283072420, 0.003424321714559292948 ),
 .UNSPECIFIED. ) ;
#17859=CARTESIAN_POINT ( 'NONE',  ( -94.99999999999997158, -213.0599564267049857, 80.07812500173432113 ) ) ;
#17863=CARTESIAN_POINT ( 'NONE',  ( 97.64999999999997726, 88.47002178664753558, 78.91395833506763324 ) ) ;
#17864=CARTESIAN_POINT ( 'NONE',  ( -97.65000000000001990, 90.00000000000004263, 78.64937500173429896 ) ) ;
#17867=CARTESIAN_POINT ( 'NONE',  ( 94.99999999999998579, 87.33691857156068750, 80.43531250086715545 ) ) ;
#17872=ORIENTED_EDGE ( 'NONE', *, *, #52908, .T. ) ;
#17883=CARTESIAN_POINT ( 'NONE',  ( -93.84685191531248449, -208.0026889286704943, 76.88989583420048746 ) ) ;
#17892=DIRECTION ( 'NONE',  ( -0.000000000000000000, -0.000000000000000000, 1.000000000000000000 ) ) ;
#17898=EDGE_CURVE ( 'NONE', #4009, #65017, #42228, .T. ) ;
#17900=CARTESIAN_POINT ( 'NONE',  ( 93.84685191531248449, 91.99731107132950569, 87.15572916753382060 ) ) ;
#17909=CARTESIAN_POINT ( 'NONE',  ( -95.00000000000002842, 92.66308142843932671, 79.95906250086713385 ) ) ;
#17914=CARTESIAN_POINT ( 'NONE',  ( 95.00000000000000000, -212.6630814284392557, 88.53156250086713897 ) ) ;
#17920=DIRECTION ( 'NONE',  ( 1.000000000000000000, 0.000000000000000000, 0.000000000000000000 ) ) ;
#17922=VERTEX_POINT ( 'NONE', #891 ) ;
#17924=CARTESIAN_POINT ( 'NONE',  ( 92.69370383062501162, -211.3315407142195852, 82.86947916753379673 ) ) ;
#17926=CARTESIAN_POINT ( 'NONE',  ( 97.64999999999997726, 91.52997821335253548, 89.73541666666663730 ) ) ;
#17928=CARTESIAN_POINT ( 'NONE',  ( -92.34999999999999432, -208.4700217866474645, 77.11479166840095445 ) ) ;
#17931=EDGE_CURVE ( 'NONE', #41327, #15281, #52759, .T. ) ;
#17933=CARTESIAN_POINT ( 'NONE',  ( 97.64999999999997726, -208.4700217866474645, 85.29041666666665833 ) ) ;
#17937=VERTEX_POINT ( 'NONE', #11738 ) ;
#17943=CARTESIAN_POINT ( 'NONE',  ( -92.69370383062502583, 91.33154071421968467, 86.36197916753383197 ) ) ;
#17946=CARTESIAN_POINT ( 'NONE',  ( 96.32499999999998863, -212.2949673200287179, 76.32104166840096582 ) ) ;
#17947=CARTESIAN_POINT ( 'NONE',  ( 92.34999999999999432, 90.00000000000002842, 77.29999999999999716 ) ) ;
#17949=CARTESIAN_POINT ( 'NONE',  ( -94.99999999999997158, -213.0599564267049857, 88.96812500173430749 ) ) ;
#17952=ORIENTED_EDGE ( 'NONE', *, *, #43202, .F. ) ;
#17953=CARTESIAN_POINT ( 'NONE',  ( -95.00000000000002842, 92.66308142843932671, 80.11781250086714579 ) ) ;
#17954=CARTESIAN_POINT ( 'NONE',  ( 92.69370383062498320, 90.00000000000002842, 76.30781250086714351 ) ) ;
#17965=CARTESIAN_POINT ( 'NONE',  ( -96.15314808468747287, -208.0026889286704943, 78.74197916753381321 ) ) ;
#17975=CARTESIAN_POINT ( 'NONE',  ( -96.15314808468745866, -211.9973110713294489, 87.36739583420049371 ) ) ;
#17976=VERTEX_POINT ( 'NONE', #28669 ) ;
#17977=CARTESIAN_POINT ( 'NONE',  ( -97.64999999999997726, -208.4700217866474645, 81.69208333333332916 ) ) ;
#17983=CARTESIAN_POINT ( 'NONE',  ( 93.84685191531248449, 88.00268892867053694, 86.57364583420047666 ) ) ;
#17985=CARTESIAN_POINT ( 'NONE',  ( -95.00000000000002842, 86.94004357329504273, 75.55375000000000796 ) ) ;
#17990=ADVANCED_FACE ( 'NONE', ( #51610 ), #47092, .F. ) ;
#17998=CARTESIAN_POINT ( 'NONE',  ( 97.64999999999999147, -209.9999999999999716, 90.00000000000000000 ) ) ;
#18001=EDGE_CURVE ( 'NONE', #19615, #29989, #48190, .T. ) ;
#18003=CARTESIAN_POINT ( 'NONE',  ( 92.34999999999999432, 90.00000000000002842, 85.55499999999999261 ) ) ;
#18006=CARTESIAN_POINT ( 'NONE',  ( 93.67499999999998295, 92.29496732002878900, 77.19416666666666060 ) ) ;
#18009=VECTOR ( 'NONE', #26186, 1000.000000000000000 ) ;
#18012=AXIS2_PLACEMENT_3D ( 'NONE', #67422, #56142, #38106 ) ;
#18014=CARTESIAN_POINT ( 'NONE',  ( 95.00000000000000000, -212.6630814284392557, 84.88031250086714863 ) ) ;
#18023=CARTESIAN_POINT ( 'NONE',  ( 93.84685191531251292, -211.9973110713294489, 75.77864583420047495 ) ) ;
#18025=CARTESIAN_POINT ( 'NONE',  ( 97.30629616937498838, -211.3315407142195852, 79.27114583420048177 ) ) ;
#18029=AXIS2_PLACEMENT_3D ( 'NONE', #46950, #8190, #64990 ) ;
#18030=EDGE_LOOP ( 'NONE', ( #72684, #59082 ) ) ;
#18036=CARTESIAN_POINT ( 'NONE',  ( 93.67500000000001137, -212.2949673200287179, 85.74020833506763495 ) ) ;
#18037=CARTESIAN_POINT ( 'NONE',  ( 93.67499999999999716, 87.70503267997126784, 89.47083333333333144 ) ) ;
#18040=EDGE_LOOP ( 'NONE', ( #25914, #42891, #17600, #68885 ) ) ;
#18044=CARTESIAN_POINT ( 'NONE',  ( 92.34999999999999432, 91.52997821335252127, 84.94645833506763211 ) ) ;
#18058=CARTESIAN_POINT ( 'NONE',  ( -93.67500000000003979, 92.29496732002878900, 87.88333333333332575 ) ) ;
#18060=CARTESIAN_POINT ( 'NONE',  ( 92.35000000000000853, -208.4700217866474645, 89.94708333333332462 ) ) ;
#18062=( BOUNDED_CURVE ( )  B_SPLINE_CURVE ( 2, ( #9753, #54871, #4503, #50337, #73267, #65158, #37954, #9374, #21381 ),
 .UNSPECIFIED., .F., .F. ) 
 B_SPLINE_CURVE_WITH_KNOTS ( ( 3, 2, 2, 2, 3 ),
 ( 0.5291824299508944840, 0.5362381811070600079, 0.5432939466479423940, 0.5503497121888247801, 0.5503499107226623721 ),
 .UNSPECIFIED. ) 
 CURVE ( )  GEOMETRIC_REPRESENTATION_ITEM ( )  RATIONAL_B_SPLINE_CURVE ( ( 1.000000000000000000, 0.8660254037844387076, 1.000000000000000000, 0.8660254037844387076, 1.000000000000000000, 0.8660254037844387076, 1.000000000000000000, 0.9999962302473670572, 0.9999924607068793048 ) ) 
 REPRESENTATION_ITEM ( '' )  );
#18063=FACE_OUTER_BOUND ( 'NONE', #26262, .T. ) ;
#18064=CARTESIAN_POINT ( 'NONE',  ( -96.15314808468745866, -211.9973110713294489, 82.12864583420046927 ) ) ;
#18065=ORIENTED_EDGE ( 'NONE', *, *, #72647, .T. ) ;
#18068=CARTESIAN_POINT ( 'NONE',  ( -94.99999999999997158, -207.3369185715606307, 75.51406250086714067 ) ) ;
#18077=LINE ( 'NONE', #68195, #20357 ) ;
#18080=CARTESIAN_POINT ( 'NONE',  ( -92.35000000000009379, 91.52997821335256390, 76.40041666666667197 ) ) ;
#18082=CARTESIAN_POINT ( 'NONE',  ( -96.15314808468752972, 91.99731107132950569, 76.83697916753381207 ) ) ;
#18094=CARTESIAN_POINT ( 'NONE',  ( -96.15314808468745866, -211.9973110713294489, 76.57239583420049200 ) ) ;
#18095=DIRECTION ( 'NONE',  ( -0.000000000000000000, -0.000000000000000000, 1.000000000000000000 ) ) ;
#18099=EDGE_CURVE ( 'NONE', #35608, #71243, #60010, .T. ) ;
#18109=EDGE_CURVE ( 'NONE', #67219, #30790, #21555, .T. ) ;
#18111=CARTESIAN_POINT ( 'NONE',  ( 93.84685191531251292, -211.9973110713294489, 83.39864583420047950 ) ) ;
#18114=CARTESIAN_POINT ( 'NONE',  ( -93.67500000000003979, 92.29496732002878900, 79.62833333333333030 ) ) ;
#18116=ORIENTED_EDGE ( 'NONE', *, *, #47115, .F. ) ;
#18117=CARTESIAN_POINT ( 'NONE',  ( 92.35000000000000853, -209.9999999999999716, 84.99937500173429328 ) ) ;
#18119=VECTOR ( 'NONE', #12769, 1000.000000000000000 ) ;
#18120=CARTESIAN_POINT ( 'NONE',  ( -92.69370383062502583, 91.33154071421968467, 80.64697916753382856 ) ) ;
#18127=DIRECTION ( 'NONE',  ( -0.000000000000000000, -0.000000000000000000, -1.000000000000000000 ) ) ;
#18128=VERTEX_POINT ( 'NONE', #63468 ) ;
#18129=CARTESIAN_POINT ( 'NONE',  ( 96.32499999999998863, 87.70503267997126784, 80.76604166840097321 ) ) ;
#18134=VERTEX_POINT ( 'NONE', #5592 ) ;
#18135=CARTESIAN_POINT ( 'NONE',  ( 96.15314808468748708, -208.0026889286704943, 81.17614583420048291 ) ) ;
#18141=CARTESIAN_POINT ( 'NONE',  ( -96.15314808468745866, -211.9973110713294489, 84.66864583420047552 ) ) ;
#18142=CARTESIAN_POINT ( 'NONE',  ( -95.00000000000002842, 92.66308142843932671, 80.75281250086715090 ) ) ;
#18144=CARTESIAN_POINT ( 'NONE',  ( 93.84685191531248449, 91.99731107132950569, 83.18697916753382060 ) ) ;
#18150=DIRECTION ( 'NONE',  ( -0.000000000000000000, -0.000000000000000000, 1.000000000000000000 ) ) ;
#18151=CARTESIAN_POINT ( 'NONE',  ( -96.15314808468747287, -208.0026889286704943, 87.63197916753379957 ) ) ;
#18155=CYLINDRICAL_SURFACE ( 'NONE', #15759, 2.649999999999985700 ) ;
#18164=CARTESIAN_POINT ( 'NONE',  ( -93.67500000000003979, 92.29496732002878900, 77.08833333333332405 ) ) ;
#18166=CARTESIAN_POINT ( 'NONE',  ( -96.15314808468752972, 91.99731107132950569, 86.99697916753380866 ) ) ;
#18167=CARTESIAN_POINT ( 'NONE',  ( 96.32499999999998863, -207.7050326799711968, 80.89833333333332632 ) ) ;
#18171=ORIENTED_EDGE ( 'NONE', *, *, #70966, .F. ) ;
#18172=CARTESIAN_POINT ( 'NONE',  ( -97.30629616937501680, 88.66845928578038638, 79.53572916753380184 ) ) ;
#18179=CARTESIAN_POINT ( 'NONE',  ( -93.84685191531247028, -211.9973110713294489, 87.47322916753381605 ) ) ;
#18182=EDGE_CURVE ( 'NONE', #69810, #31889, #49877, .T. ) ;
#18184=CARTESIAN_POINT ( 'NONE',  ( 97.30629616937498838, 90.00000000000002842, 77.41906250086715602 ) ) ;
#18185=CARTESIAN_POINT ( 'NONE',  ( -92.69370383062498320, -209.9999999999999716, 76.14906250086716000 ) ) ;
#18193=CARTESIAN_POINT ( 'NONE',  ( -97.30629616937501680, 88.66845928578038638, 76.51947916753381662 ) ) ;
#18194=CARTESIAN_POINT ( 'NONE',  ( 92.69370383062501162, -211.3315407142195852, 78.26572916753380582 ) ) ;
#18209=ORIENTED_EDGE ( 'NONE', *, *, #51777, .T. ) ;
#18210=ORIENTED_EDGE ( 'NONE', *, *, #17931, .F. ) ;
#18211=CARTESIAN_POINT ( 'NONE',  ( 93.84685191531248449, 91.99731107132950569, 84.61572916753381435 ) ) ;
#18212=CARTESIAN_POINT ( 'NONE',  ( 90.00000000000000000, 95.00000000000002842, 90.00000000000000000 ) ) ;
#18213=CARTESIAN_POINT ( 'NONE',  ( 95.00000000000000000, -206.9400435732949575, 75.23624999999999829 ) ) ;
#18215=ORIENTED_EDGE ( 'NONE', *, *, #22515, .T. ) ;
#18223=DIRECTION ( 'NONE',  ( 0.000000000000000000, 0.000000000000000000, 1.000000000000000000 ) ) ;
#18227=CARTESIAN_POINT ( 'NONE',  ( 97.65000000000000568, -209.9999753241869200, 87.22187585518551600 ) ) ;
#18228=LINE ( 'NONE', #41167, #10773 ) ;
#18230=CARTESIAN_POINT ( 'NONE',  ( -93.67499999999998295, -212.2949673200287179, 77.59104166840097605 ) ) ;
#18234=CARTESIAN_POINT ( 'NONE',  ( 92.34999999999999432, 90.00000000000002842, 78.64937500173429896 ) ) ;
#18235=CARTESIAN_POINT ( 'NONE',  ( -95.00000000000002842, 93.05995642670501411, 77.22062500173429100 ) ) ;
#18237=CARTESIAN_POINT ( 'NONE',  ( 92.69370383062498320, 88.66845928578037217, 80.96447916753382401 ) ) ;
#18249=ORIENTED_EDGE ( 'NONE', *, *, #11965, .F. ) ;
#18253=CARTESIAN_POINT ( 'NONE',  ( -97.30629616937497417, -208.6684592857803011, 76.41364583420049428 ) ) ;
#18262=CARTESIAN_POINT ( 'NONE',  ( 92.34999999999999432, 90.00000000000002842, 85.55499999999999261 ) ) ;
#18264=DIRECTION ( 'NONE',  ( -0.000000000000000000, -0.000000000000000000, 1.000000000000000000 ) ) ;
#18267=ADVANCED_FACE ( 'NONE', ( #22879 ), #48376, .F. ) ;
#18272=( BOUNDED_CURVE ( )  B_SPLINE_CURVE ( 2, ( #1970, #42165, #48890, #65100, #13570, #25240, #71446 ),
 .UNSPECIFIED., .F., .F. ) 
 B_SPLINE_CURVE_WITH_KNOTS ( ( 3, 2, 2, 3 ),
 ( 0.6041666666666670737, 0.6111111111111116045, 0.6180555555555559133, 0.6250000000000003331 ),
 .UNSPECIFIED. ) 
 CURVE ( )  GEOMETRIC_REPRESENTATION_ITEM ( )  RATIONAL_B_SPLINE_CURVE ( ( 0.9999999999999914513, 0.8660254037844472563, 1.000000000000000000, 0.8660254037844387076, 1.000000000000000000, 0.8660254037844322683, 1.000000000000006439 ) ) 
 REPRESENTATION_ITEM ( '' )  );
#18273=CARTESIAN_POINT ( 'NONE',  ( 96.15314808468748708, 91.99731107132950569, 87.68489583420048916 ) ) ;
#18274=CARTESIAN_POINT ( 'NONE',  ( -93.84685191531247028, -211.9973110713294489, 85.56822916753381492 ) ) ;
#18277=CARTESIAN_POINT ( 'NONE',  ( 92.35000000046504454, -210.0000309987310061, 83.09538598081256566 ) ) ;
#18278=CARTESIAN_POINT ( 'NONE',  ( -96.32499999999996021, -212.2949673200287179, 80.58083333333331666 ) ) ;
#18279=CARTESIAN_POINT ( 'NONE',  ( -93.84685191531254134, 91.99731107132950569, 76.09614583420047040 ) ) ;
#18280=EDGE_CURVE ( 'NONE', #21000, #2294, #55161, .T. ) ;
#18282=CARTESIAN_POINT ( 'NONE',  ( 93.84685191531249870, -208.0026889286704943, 85.72697916753379843 ) ) ;
#18285=CARTESIAN_POINT ( 'NONE',  ( 97.65000000000000568, 88.47002178664752137, 87.16895833506762870 ) ) ;
#18290=VERTEX_POINT ( 'NONE', #18324 ) ;
#18291=CARTESIAN_POINT ( 'NONE',  ( 92.69370383062501162, -209.9999999999999716, 80.27656250086714351 ) ) ;
#18293=CARTESIAN_POINT ( 'NONE',  ( 97.64999999999999147, 90.00000000000002842, 80.79249999999998977 ) ) ;
#18295=CYLINDRICAL_SURFACE ( 'NONE', #56178, 2.649999999999985700 ) ;
#18296=CARTESIAN_POINT ( 'NONE',  ( 97.64999999999997726, -211.5299782133524502, 85.81958333333331268 ) ) ;
#18298=EDGE_LOOP ( 'NONE', ( #3573, #21163, #64998, #42622 ) ) ;
#18305=CARTESIAN_POINT ( 'NONE',  ( -96.15314808468751551, 88.00268892867056536, 86.09739583420049769 ) ) ;
#18308=LINE ( 'NONE', #41251, #24583 ) ;
#18309=CARTESIAN_POINT ( 'NONE',  ( 92.69370383062501162, -211.3315407142195852, 87.79072916753381151 ) ) ;
#18310=CARTESIAN_POINT ( 'NONE',  ( 92.34999999999999432, 88.47002178664753558, 77.98791666666664923 ) ) ;
#18313=CARTESIAN_POINT ( 'NONE',  ( 97.64999999999999147, 90.00000000000002842, 79.52249999999999375 ) ) ;
#18318=CARTESIAN_POINT ( 'NONE',  ( -93.67500000000003979, 87.70503267997129626, 89.02104166840096866 ) ) ;
#18319=CARTESIAN_POINT ( 'NONE',  ( 97.30629616937498838, 91.33154071421968467, 89.53697916753382913 ) ) ;
#18322=ADVANCED_FACE ( 'NONE', ( #19426 ), #23979, .F. ) ;
#18324=CARTESIAN_POINT ( 'NONE',  ( -92.35000000000006537, -209.9999992849074317, 85.31687502647974952 ) ) ;
#18330=CARTESIAN_POINT ( 'NONE',  ( -96.15314808468747287, -208.0026889286704943, 74.93197916753379673 ) ) ;
#18332=EDGE_LOOP ( 'NONE', ( #69923, #69346 ) ) ;
#18337=CARTESIAN_POINT ( 'NONE',  ( -93.84685191531248449, -208.0026889286704943, 88.95489583420049939 ) ) ;
#18340=VERTEX_POINT ( 'NONE', #46912 ) ;
#18344=CARTESIAN_POINT ( 'NONE',  ( 94.99999999999998579, 87.33691857156068750, 81.54656250086713953 ) ) ;
#18346=CARTESIAN_POINT ( 'NONE',  ( -95.00000000000002842, 93.05995642670504253, 80.39562500173430237 ) ) ;
#18357=CARTESIAN_POINT ( 'NONE',  ( 99.99999999999998579, 95.00000000000002842, 90.00000000000000000 ) ) ;
#18358=CARTESIAN_POINT ( 'NONE',  ( -93.84685191531252713, 88.00268892867056536, 85.40947916753380298 ) ) ;
#18363=VECTOR ( 'NONE', #39335, 1000.000000000000000 ) ;
#18370=CARTESIAN_POINT ( 'NONE',  ( 92.69370383062501162, -211.3315407142195852, 82.86947916753382515 ) ) ;
#18377=ORIENTED_EDGE ( 'NONE', *, *, #25545, .F. ) ;
#18378=CARTESIAN_POINT ( 'NONE',  ( 95.00000000000000000, -207.3369185715606307, 78.21281250086717307 ) ) ;
#18381=CARTESIAN_POINT ( 'NONE',  ( -94.99999999999997158, -213.0599564267049857, 88.25374999999999659 ) ) ;
#18389=CARTESIAN_POINT ( 'NONE',  ( 93.67500000000001137, -212.2949673200287179, 86.37520833506764006 ) ) ;
#18390=CARTESIAN_POINT ( 'NONE',  ( 94.99999999999998579, 93.05995642670504253, 87.30124999999999602 ) ) ;
#18396=ORIENTED_EDGE ( 'NONE', *, *, #47143, .F. ) ;
#18400=CARTESIAN_POINT ( 'NONE',  ( 94.99999999999998579, 93.05995642670504253, 84.84062500173429555 ) ) ;
#18401=EDGE_CURVE ( 'NONE', #57350, #41695, #44974, .T. ) ;
#18415=CARTESIAN_POINT ( 'NONE',  ( -93.67500000000003979, 87.70503267997129626, 86.40166666666667084 ) ) ;
#18422=CARTESIAN_POINT ( 'NONE',  ( -96.15314808468747287, -208.0026889286704943, 83.18697916753382060 ) ) ;
#18424=AXIS2_PLACEMENT_3D ( 'NONE', #9386, #32312, #22072 ) ;
#18429=CARTESIAN_POINT ( 'NONE',  ( -92.69370383062498320, -211.3315407142195852, 75.93739583420050110 ) ) ;
#18433=AXIS2_PLACEMENT_3D ( 'NONE', #52470, #7365, #52107 ) ;
#18439=CARTESIAN_POINT ( 'NONE',  ( -93.84685191531252713, 88.00268892867056536, 79.05947916753380866 ) ) ;
#18447=LINE ( 'NONE', #64327, #29896 ) ;
#18449=CARTESIAN_POINT ( 'NONE',  ( -97.65000000000003411, 89.99996406754254963, 85.63437624451402996 ) ) ;
#18450=CARTESIAN_POINT ( 'NONE',  ( -93.84685191531248449, -208.0026889286704943, 74.98489583420048632 ) ) ;
#18462=DIRECTION ( 'NONE',  ( -0.000000000000000000, -0.000000000000000000, 1.000000000000000000 ) ) ;
#18466=( BOUNDED_CURVE ( )  B_SPLINE_CURVE ( 2, ( #59362, #37177, #60120, #31514, #37912, #43198, #8963 ),
 .UNSPECIFIED., .F., .F. ) 
 B_SPLINE_CURVE_WITH_KNOTS ( ( 3, 2, 2, 3 ),
 ( 0.4374999999999994449, 0.4444444444444441422, 0.4513888888888888951, 0.4583333333333335924 ),
 .UNSPECIFIED. ) 
 CURVE ( )  GEOMETRIC_REPRESENTATION_ITEM ( )  RATIONAL_B_SPLINE_CURVE ( ( 1.000000000000010658, 0.8660254037844280495, 1.000000000000000000, 0.8660254037844387076, 1.000000000000000000, 0.8660254037844333785, 1.000000000000005329 ) ) 
 REPRESENTATION_ITEM ( '' )  );
#18467=CARTESIAN_POINT ( 'NONE',  ( 96.15314808468748708, -208.0026889286704943, 85.62114583420046188 ) ) ;
#18468=CARTESIAN_POINT ( 'NONE',  ( 92.69370383062501162, -208.6684592857803295, 87.84364583420048689 ) ) ;
#18471=EDGE_CURVE ( 'NONE', #22009, #63717, #31814, .T. ) ;
#18475=CARTESIAN_POINT ( 'NONE',  ( 93.67500000000001137, -212.2949673200287179, 85.10520833506762983 ) ) ;
#18477=CARTESIAN_POINT ( 'NONE',  ( -92.69370383062504004, 90.00000000000004263, 81.86406250086714920 ) ) ;
#18479=VERTEX_POINT ( 'NONE', #19796 ) ;
#18485=FACE_OUTER_BOUND ( 'NONE', #18298, .T. ) ;
#18487=CARTESIAN_POINT ( 'NONE',  ( -92.35000000000003695, 90.00000000000004263, 75.71250000000000568 ) ) ;
#18489=( BOUNDED_CURVE ( )  B_SPLINE_CURVE ( 2, ( #56445, #4956, #27855 ),
 .UNSPECIFIED., .F., .F. ) 
 B_SPLINE_CURVE_WITH_KNOTS ( ( 3, 3 ),
 ( 0.000000000000000000, 2.334341054613931057E-05 ),
 .UNSPECIFIED. ) 
 CURVE ( )  GEOMETRIC_REPRESENTATION_ITEM ( )  RATIONAL_B_SPLINE_CURVE ( ( 0.9459494467533609008, 0.9464399322878827014, 0.9469490141588213783 ) ) 
 REPRESENTATION_ITEM ( '' )  );
#18494=CARTESIAN_POINT ( 'NONE',  ( 93.84685191531251292, -211.9973110713294489, 81.49364583420047836 ) ) ;
#18502=CARTESIAN_POINT ( 'NONE',  ( -97.30629616937497417, -211.3315407142195852, 83.34572916753380412 ) ) ;
#18503=CARTESIAN_POINT ( 'NONE',  ( -97.30629616937501680, 91.33154071421968467, 80.85864583420048746 ) ) ;
#18506=EDGE_CURVE ( 'NONE', #71848, #36383, #54719, .T. ) ;
#18507=CARTESIAN_POINT ( 'NONE',  ( 93.84685191531248449, 91.99731107132950569, 81.28197916753380525 ) ) ;
#18508=ORIENTED_EDGE ( 'NONE', *, *, #9435, .F. ) ;
#18514=CARTESIAN_POINT ( 'NONE',  ( -97.30629616937495996, -209.9999999999999716, 85.83281250086714920 ) ) ;
#18522=ORIENTED_EDGE ( 'NONE', *, *, #51104, .T. ) ;
#18523=CARTESIAN_POINT ( 'NONE',  ( 2.499999999999984457, -73.00000000000001421, -258.2999999999999545 ) ) ;
#18526=CARTESIAN_POINT ( 'NONE',  ( -96.15314808468752972, 91.99731107132950569, 87.63197916753379957 ) ) ;
#18542=CARTESIAN_POINT ( 'NONE',  ( -94.99999999999997158, -207.3369185715606307, 87.73781250086715033 ) ) ;
#18549=CARTESIAN_POINT ( 'NONE',  ( -92.69370383062498320, -208.6684592857803295, 75.56697916753383026 ) ) ;
#18555=CARTESIAN_POINT ( 'NONE',  ( -96.15314808468751551, 88.00268892867056536, 75.93739583420048689 ) ) ;
#18556=CARTESIAN_POINT ( 'NONE',  ( 92.69370383062501162, -209.9999999999999716, 76.30781250086714351 ) ) ;
#18560=DIRECTION ( 'NONE',  ( -0.000000000000000000, -0.000000000000000000, 1.000000000000000000 ) ) ;
#18562=EDGE_CURVE ( 'NONE', #44941, #15992, #4022, .T. ) ;
#18567=ORIENTED_EDGE ( 'NONE', *, *, #56601, .T. ) ;
#18569=ORIENTED_EDGE ( 'NONE', *, *, #32978, .F. ) ;
#18573=CARTESIAN_POINT ( 'NONE',  ( 96.15314808468748708, 91.99731107132950569, 78.79489583420048859 ) ) ;
#18576=AXIS2_PLACEMENT_3D ( 'NONE', #45982, #68907, #35059 ) ;
#18577=FACE_OUTER_BOUND ( 'NONE', #66580, .T. ) ;
#18589=DIRECTION ( 'NONE',  ( 0.000000000000000000, 0.000000000000000000, -1.000000000000000000 ) ) ;
#18591=EDGE_CURVE ( 'NONE', #57700, #66667, #70070, .T. ) ;
#18593=CARTESIAN_POINT ( 'NONE',  ( -96.32499999999996021, -212.2949673200287179, 80.66020833506763665 ) ) ;
#18596=CARTESIAN_POINT ( 'NONE',  ( 97.64999999999996305, 88.93103996628909158, 74.48490336299444436 ) ) ;
#18597=CARTESIAN_POINT ( 'NONE',  ( -97.65000000000001990, 90.00000000000004263, 77.37937500173428873 ) ) ;
#18599=CARTESIAN_POINT ( 'NONE',  ( 92.69370383062498320, 91.33154071421968467, 78.95364583420048632 ) ) ;
#18600=CARTESIAN_POINT ( 'NONE',  ( 92.34999999999999432, 90.00000000000002842, 90.00000000000000000 ) ) ;
#18603=CARTESIAN_POINT ( 'NONE',  ( -97.64999999996715019, 90.00000839192523472, 86.90410584365564262 ) ) ;
#18606=CARTESIAN_POINT ( 'NONE',  ( -92.35000000000003695, 90.00000015433754186, 79.60187500750917877 ) ) ;
#18608=EDGE_CURVE ( 'NONE', #35348, #22766, #5873, .T. ) ;
#18610=VERTEX_POINT ( 'NONE', #27671 ) ;
#18613=( BOUNDED_CURVE ( )  B_SPLINE_CURVE ( 2, ( #21497, #68119, #34269, #51188, #44454, #22630, #61745 ),
 .UNSPECIFIED., .F., .F. ) 
 B_SPLINE_CURVE_WITH_KNOTS ( ( 3, 2, 2, 3 ),
 ( 0.8466920362367555963, 0.8537476304467667143, 0.8608033959876489893, 0.8678591737214816915 ),
 .UNSPECIFIED. ) 
 CURVE ( )  GEOMETRIC_REPRESENTATION_ITEM ( )  RATIONAL_B_SPLINE_CURVE ( ( 0.9999934937104166810, 0.8660286570082263990, 1.000000000000000000, 0.8660254037844387076, 1.000000000000000000, 0.8660254037844387076, 1.000000000000000000 ) ) 
 REPRESENTATION_ITEM ( '' )  );
#18615=DIRECTION ( 'NONE',  ( -0.000000000000000000, -0.000000000000000000, 1.000000000000000000 ) ) ;
#18617=CARTESIAN_POINT ( 'NONE',  ( -96.15314808468747287, -208.0026889286704943, 77.63072916753381492 ) ) ;
#18623=DIRECTION ( 'NONE',  ( 1.000000000000000000, 0.000000000000000000, 0.000000000000000000 ) ) ;
#18627=CARTESIAN_POINT ( 'NONE',  ( -96.32499999999996021, -212.2949673200287179, 85.10520833506762983 ) ) ;
#18628=DIRECTION ( 'NONE',  ( -1.343011723336883198E-16, 1.000000000000000000, 0.000000000000000000 ) ) ;
#18632=CARTESIAN_POINT ( 'NONE',  ( 94.99999999999998579, 87.33691857156068750, 83.61031250086715261 ) ) ;
#18633=CARTESIAN_POINT ( 'NONE',  ( -92.69370383062498320, -209.9999999999999716, 88.21406250086714351 ) ) ;
#18636=CARTESIAN_POINT ( 'NONE',  ( -97.64999999999994884, -211.5299782133524502, 82.43291666666665662 ) ) ;
#18637=CARTESIAN_POINT ( 'NONE',  ( -97.30629616937501680, 91.33154071421968467, 75.61989583420047722 ) ) ;
#18640=CARTESIAN_POINT ( 'NONE',  ( 97.30629616937498838, -209.9999999999999716, 85.51531250086713953 ) ) ;
#18654=CARTESIAN_POINT ( 'NONE',  ( 92.69370383062501162, -209.9999999999999716, 83.45156250086715488 ) ) ;
#18661=CARTESIAN_POINT ( 'NONE',  ( 96.32499999999998863, -207.7050326799711968, 83.43833333333333258 ) ) ;
#18667=CARTESIAN_POINT ( 'NONE',  ( -93.84685191531254134, 91.99731107132950569, 88.31989583420048007 ) ) ;
#18670=CARTESIAN_POINT ( 'NONE',  ( 96.90829146052659837, -211.8387288276635729, 74.44346887015069569 ) ) ;
#18671=CARTESIAN_POINT ( 'NONE',  ( 92.34999999999999432, 91.52997821335252127, 78.51708333333334622 ) ) ;
#18674=CARTESIAN_POINT ( 'NONE',  ( 96.32499999999997442, 92.29496732002878900, 79.62833333333333030 ) ) ;
#18677=CARTESIAN_POINT ( 'NONE',  ( -97.64999999999996305, -209.9999999999999716, 84.92000000000000171 ) ) ;
#18679=CARTESIAN_POINT ( 'NONE',  ( -92.35000000000005116, 91.52997821335253548, 86.63979166840097434 ) ) ;
#18680=CARTESIAN_POINT ( 'NONE',  ( 94.99999999999998579, 87.33691857156068750, 76.46656250086712703 ) ) ;
#18702=( BOUNDED_CURVE ( )  B_SPLINE_CURVE ( 2, ( #46800, #28100, #24238, #24592, #53537, #47894, #69715, #45417, #62721 ),
 .UNSPECIFIED., .F., .F. ) 
 B_SPLINE_CURVE_WITH_KNOTS ( ( 3, 2, 2, 2, 3 ),
 ( 0.5291824299508929297, 0.5362381811070600079, 0.5432939466479423940, 0.5503497121888247801, 0.5503499107226623721 ),
 .UNSPECIFIED. ) 
 CURVE ( )  GEOMETRIC_REPRESENTATION_ITEM ( )  RATIONAL_B_SPLINE_CURVE ( ( 1.000000000000000000, 0.8660254037844387076, 1.000000000000000000, 0.8660254037844387076, 1.000000000000000000, 0.8660254037844387076, 1.000000000000000000, 0.9999962302473670572, 0.9999924607068793048 ) ) 
 REPRESENTATION_ITEM ( '' )  );
#18703=CARTESIAN_POINT ( 'NONE',  ( -93.84685191531248449, -208.0026889286704943, 88.31989583420048007 ) ) ;
#18708=CARTESIAN_POINT ( 'NONE',  ( -93.67500000000003979, 92.29496732002878900, 83.51770833506763836 ) ) ;
#18712=CARTESIAN_POINT ( 'NONE',  ( 97.30629616937498838, 88.66845928578035796, 81.65239583420047609 ) ) ;
#18720=CARTESIAN_POINT ( 'NONE',  ( 92.35000000049298308, -210.0000320324309939, 85.63541623677062375 ) ) ;
#18722=CARTESIAN_POINT ( 'NONE',  ( -96.15314808468751551, 88.00268892867056536, 87.84364583420047268 ) ) ;
#18735=CARTESIAN_POINT ( 'NONE',  ( 92.69370383062501162, -208.6684592857803011, 81.49364583420047836 ) ) ;
#18740=ORIENTED_EDGE ( 'NONE', *, *, #60062, .T. ) ;
#18744=DIRECTION ( 'NONE',  ( -0.000000000000000000, -0.000000000000000000, 1.000000000000000000 ) ) ;
#18746=CARTESIAN_POINT ( 'NONE',  ( 92.69370383062501162, -208.6684592857803295, 74.98489583420048632 ) ) ;
#18748=ORIENTED_EDGE ( 'NONE', *, *, #19948, .T. ) ;
#18749=CARTESIAN_POINT ( 'NONE',  ( 96.15314808468750130, -211.9973110713294489, 78.58322916753382970 ) ) ;
#18752=ORIENTED_EDGE ( 'NONE', *, *, #31388, .T. ) ;
#18753=VERTEX_POINT ( 'NONE', #64120 ) ;
#18754=CARTESIAN_POINT ( 'NONE',  ( -97.64999999950698850, -210.0000320324311076, 85.63541623677365067 ) ) ;
#18755=( NAMED_UNIT ( * ) SI_UNIT ( $, .STERADIAN. ) SOLID_ANGLE_UNIT ( ) );
#18759=CARTESIAN_POINT ( 'NONE',  ( 92.35000000000000853, -209.9999999999999716, 82.45937500173430124 ) ) ;
#18760=CARTESIAN_POINT ( 'NONE',  ( 93.67499999999998295, 92.29496732002878900, 89.25916666666667254 ) ) ;
#18768=CARTESIAN_POINT ( 'NONE',  ( -96.15314808468751551, 88.00268892867056536, 88.00239583420048461 ) ) ;
#18770=CARTESIAN_POINT ( 'NONE',  ( 94.99999999999998579, 93.05995642670504253, 85.47562500173431488 ) ) ;
#18778=CARTESIAN_POINT ( 'NONE',  ( 92.34999999999996589, 91.52997821335250705, 81.69208333333332916 ) ) ;
#18779=CARTESIAN_POINT ( 'NONE',  ( -97.65000000000001990, 91.52997821335253548, 86.13708333333332234 ) ) ;
#18785=CARTESIAN_POINT ( 'NONE',  ( -92.69370383062498320, -211.3315407142195852, 82.92239583420045790 ) ) ;
#18790=CARTESIAN_POINT ( 'NONE',  ( 97.65000000000000568, 91.52997821335252127, 89.17979166840096639 ) ) ;
#18798=CARTESIAN_POINT ( 'NONE',  ( 97.65000000000000568, 91.52997821335252127, 82.82979166840095786 ) ) ;
#18799=CARTESIAN_POINT ( 'NONE',  ( -93.67499999999998295, -207.7050326799711968, 86.69270833506763552 ) ) ;
#18801=CARTESIAN_POINT ( 'NONE',  ( -96.15314808468751551, 88.00268892867056536, 77.68364583420047609 ) ) ;
#18812=CARTESIAN_POINT ( 'NONE',  ( -96.32499999999996021, -207.7050326799711968, 89.89416666666666345 ) ) ;
#18817=VERTEX_POINT ( 'NONE', #626 ) ;
#18830=CARTESIAN_POINT ( 'NONE',  ( 96.15314808468748708, -208.0026889286704943, 86.25614583420048120 ) ) ;
#18831=CARTESIAN_POINT ( 'NONE',  ( 96.15314808468748708, -208.0026889286704943, 88.95489583420049939 ) ) ;
#18835=CARTESIAN_POINT ( 'NONE',  ( -97.65000000000001990, 90.00000000000004263, 79.83999999999998920 ) ) ;
#18840=CARTESIAN_POINT ( 'NONE',  ( -92.69370383062504004, 90.00000000000004263, 80.59406250086715318 ) ) ;
#18848=CARTESIAN_POINT ( 'NONE',  ( 92.35000000000006537, -211.5299782133524786, 79.25791666666667368 ) ) ;
#18855=CARTESIAN_POINT ( 'NONE',  ( 93.74200686866046794, 87.71227518788542454, 74.97309184317514053 ) ) ;
#18860=CARTESIAN_POINT ( 'NONE',  ( 92.69370383062501162, -208.6684592857803011, 83.23989583420046756 ) ) ;
#18864=DIRECTION ( 'NONE',  ( -0.000000000000000000, -0.000000000000000000, 1.000000000000000000 ) ) ;
#18865=CARTESIAN_POINT ( 'NONE',  ( 93.67499999999999716, 87.70503267997126784, 85.02583333333332405 ) ) ;
#18869=CARTESIAN_POINT ( 'NONE',  ( -92.69370383062498320, -208.6684592857803011, 83.02822916753379445 ) ) ;
#18871=CARTESIAN_POINT ( 'NONE',  ( -93.84685191531252713, 88.00268892867056536, 83.02822916753380866 ) ) ;
#18873=CARTESIAN_POINT ( 'NONE',  ( 92.69370383062498320, 90.00000000000002842, 82.02281250086714692 ) ) ;
#18880=CARTESIAN_POINT ( 'NONE',  ( -97.30629616937497417, -208.6684592857803295, 84.50989583420049200 ) ) ;
#18887=CARTESIAN_POINT ( 'NONE',  ( -93.67500000000003979, 87.70503267997129626, 76.24166666666666003 ) ) ;
#18888=CARTESIAN_POINT ( 'NONE',  ( -93.67499999999998295, -212.2949673200287179, 78.78166666666666629 ) ) ;
#18889=CARTESIAN_POINT ( 'NONE',  ( -92.69370383062502583, 91.33154071421968467, 89.37822916753381719 ) ) ;
#18892=CARTESIAN_POINT ( 'NONE',  ( 92.35000000000000853, -209.9999999999999716, 78.01437500173430806 ) ) ;
#18904=CARTESIAN_POINT ( 'NONE',  ( -92.69370383062498320, -211.3315407142195852, 86.89114583420050053 ) ) ;
#18908=( BOUNDED_CURVE ( )  B_SPLINE_CURVE ( 2, ( #60168, #72156, #21022, #43614, #26663, #15014, #31560, #61634, #60892, #27403, #27028 ),
 .UNSPECIFIED., .F., .F. ) 
 B_SPLINE_CURVE_WITH_KNOTS ( ( 3, 2, 2, 2, 2, 3 ),
 ( 0.04233441017594418571, 0.04233459324529416368, 0.04939035878617631381, 0.05644612432705845700, 0.06350188986794061408, 0.06350193517735455706 ),
 .UNSPECIFIED. ) 
 CURVE ( )  GEOMETRIC_REPRESENTATION_ITEM ( )  RATIONAL_B_SPLINE_CURVE ( ( 0.9999930479532715966, 0.9999965238864443329, 1.000000000000000000, 0.8660254037844387076, 1.000000000000000000, 0.8660254037844387076, 1.000000000000000000, 0.8660254037844387076, 1.000000000000000000, 0.9999991396666452204, 0.9999982793443398243 ) ) 
 REPRESENTATION_ITEM ( '' )  );
#18910=CARTESIAN_POINT ( 'NONE',  ( -96.15314808468745866, -211.9973110713294489, 77.20739583420048291 ) ) ;
#18917=AXIS2_PLACEMENT_3D ( 'NONE', #3984, #6120, #23398 ) ;
#18919=CARTESIAN_POINT ( 'NONE',  ( 95.00000000000000000, -207.3369185715606307, 78.68906250086713783 ) ) ;
#18938=CARTESIAN_POINT ( 'NONE',  ( 93.84685191531248449, 88.00268892867053694, 81.01739583420049939 ) ) ;
#18940=AXIS2_PLACEMENT_3D ( 'NONE', #59734, #60484, #72107 ) ;
#18941=CARTESIAN_POINT ( 'NONE',  ( 92.35000000000000853, -209.9999999999999716, 76.03000000000000114 ) ) ;
#18943=ORIENTED_EDGE ( 'NONE', *, *, #53709, .F. ) ;
#18946=EDGE_LOOP ( 'NONE', ( #47148, #2663, #21004, #28967 ) ) ;
#18955=CARTESIAN_POINT ( 'NONE',  ( -92.34999999999999432, -210.0000000255707278, 84.04687500080852658 ) ) ;
#18958=CARTESIAN_POINT ( 'NONE',  ( -93.67499999999998295, -207.7050326799711968, 79.07270833506763097 ) ) ;
#18960=CARTESIAN_POINT ( 'NONE',  ( 92.34999999999999432, 90.00000000000002842, 76.10937500173430692 ) ) ;
#18961=CARTESIAN_POINT ( 'NONE',  ( -96.32500000000001705, 87.70503267997129626, 74.94520833506761903 ) ) ;
#18962=EDGE_LOOP ( 'NONE', ( #51214, #60345, #1987, #71360 ) ) ;
#18963=CARTESIAN_POINT ( 'NONE',  ( 94.99999999999998579, 92.66308142843935514, 76.94281250086714863 ) ) ;
#18964=CARTESIAN_POINT ( 'NONE',  ( 97.65000000000009095, 88.47002178664756400, 75.65958333333333030 ) ) ;
#18966=CARTESIAN_POINT ( 'NONE',  ( 92.35000000000000853, -210.0000348529810310, 77.37937620717862330 ) ) ;
#18981=CARTESIAN_POINT ( 'NONE',  ( -93.84685191531248449, -208.0026889286704943, 78.79489583420048859 ) ) ;
#18983=EDGE_LOOP ( 'NONE', ( #29563, #33343, #50949, #38076 ) ) ;
#18988=CARTESIAN_POINT ( 'NONE',  ( 94.99999999999998579, 86.94004357329502852, 85.79312500173431033 ) ) ;
#18992=DIRECTION ( 'NONE',  ( -0.000000000000000000, -0.000000000000000000, 1.000000000000000000 ) ) ;
#18995=CARTESIAN_POINT ( 'NONE',  ( -96.32499999999996021, -207.7050326799711968, 77.90854166840097150 ) ) ;
#18999=CARTESIAN_POINT ( 'NONE',  ( 94.99999999999998579, 87.33691857156068750, 82.34031250086714238 ) ) ;
#19002=CARTESIAN_POINT ( 'NONE',  ( -96.15314808468745866, -211.9973110713294489, 85.46239583420047836 ) ) ;
#19003=CARTESIAN_POINT ( 'NONE',  ( 97.64999999999999147, -210.0000000255706709, 84.04687500080852658 ) ) ;
#19005=EDGE_CURVE ( 'NONE', #9070, #14968, #36934, .T. ) ;
#19007=CARTESIAN_POINT ( 'NONE',  ( -92.34999999999999432, -211.5299782133524502, 82.64458333333331552 ) ) ;
#19008=CARTESIAN_POINT ( 'NONE',  ( -92.69370383062505425, 91.33154071421968467, 76.67822916753378593 ) ) ;
#19011=CARTESIAN_POINT ( 'NONE',  ( 96.15314808468748708, -208.0026889286704943, 88.79614583420047325 ) ) ;
#19020=DIRECTION ( 'NONE',  ( -0.000000000000000000, -0.000000000000000000, 1.000000000000000000 ) ) ;
#19023=ORIENTED_EDGE ( 'NONE', *, *, #57956, .T. ) ;
#19026=CARTESIAN_POINT ( 'NONE',  ( 97.30629616937498838, -211.3315407142195852, 82.44614583420049314 ) ) ;
#19032=CARTESIAN_POINT ( 'NONE',  ( 97.65000000000000568, 88.47002178664752137, 76.92958333333332632 ) ) ;
#19034=CARTESIAN_POINT ( 'NONE',  ( 97.64999999999999147, -209.9999999999999716, 86.50750000000000739 ) ) ;
#19039=FACE_OUTER_BOUND ( 'NONE', #20541, .T. ) ;
#19040=CARTESIAN_POINT ( 'NONE',  ( -95.00000000000002842, 92.66308142843932671, 87.10281250086715943 ) ) ;
#19042=CARTESIAN_POINT ( 'NONE',  ( -95.00000000000002842, 86.94004357329504273, 83.80875000000000341 ) ) ;
#19043=CARTESIAN_POINT ( 'NONE',  ( 95.00000000000000000, -207.3369185715606307, 87.57906250086713840 ) ) ;
#19044=( BOUNDED_CURVE ( )  B_SPLINE_CURVE ( 2, ( #13554, #24838, #30470, #58319, #64703, #46304, #29724 ),
 .UNSPECIFIED., .F., .T. ) 
 B_SPLINE_CURVE_WITH_KNOTS ( ( 3, 2, 2, 3 ),
 ( 0.1041666666666670182, 0.1111111111111114103, 0.1180555555555558161, 0.1250000000000002220 ),
 .UNSPECIFIED. ) 
 CURVE ( )  GEOMETRIC_REPRESENTATION_ITEM ( )  RATIONAL_B_SPLINE_CURVE ( ( 0.9999999999999933387, 0.8660254037844453689, 1.000000000000000000, 0.8660254037844387076, 1.000000000000000000, 0.8660254037844343777, 1.000000000000004219 ) ) 
 REPRESENTATION_ITEM ( '' )  );
#19050=CARTESIAN_POINT ( 'NONE',  ( -96.32499999999996021, -212.2949673200287179, 85.02583333333332405 ) ) ;
#19052=CARTESIAN_POINT ( 'NONE',  ( -92.35000000000005116, 88.47002178664754979, 87.16895833506762870 ) ) ;
#19054=CARTESIAN_POINT ( 'NONE',  ( 93.84685191531248449, 88.00268892867053694, 75.77864583420047495 ) ) ;
#19057=VECTOR ( 'NONE', #63146, 1000.000000000000000 ) ;
#19059=DIRECTION ( 'NONE',  ( 1.000000000000000000, 0.000000000000000000, 0.000000000000000000 ) ) ;
#19063=CARTESIAN_POINT ( 'NONE',  ( -93.67500000000003979, 92.29496732002878900, 81.61270833506763722 ) ) ;
#19071=CARTESIAN_POINT ( 'NONE',  ( -97.30629616937495996, -209.9999999999999716, 86.62656250086715204 ) ) ;
#19081=CARTESIAN_POINT ( 'NONE',  ( 96.32499999999997442, 92.29496732002878900, 86.61333333333332973 ) ) ;
#19082=EDGE_CURVE ( 'NONE', #69246, #26229, #16298, .T. ) ;
#19084=CARTESIAN_POINT ( 'NONE',  ( 96.15314808468748708, 91.99731107132950569, 83.08114583420048405 ) ) ;
#19091=CARTESIAN_POINT ( 'NONE',  ( -92.35000000000312070, 89.99999595380251094, 77.06187486178039592 ) ) ;
#19094=CARTESIAN_POINT ( 'NONE',  ( -92.35000000000003695, 89.99999988321006583, 84.68187499741277691 ) ) ;
#19096=EDGE_CURVE ( 'NONE', #40132, #53667, #17050, .T. ) ;
#19097=DIRECTION ( 'NONE',  ( -0.000000000000000000, -0.000000000000000000, 1.000000000000000000 ) ) ;
#19100=CARTESIAN_POINT ( 'NONE',  ( -97.30629616937501680, 88.66845928578038638, 85.25072916753379104 ) ) ;
#19113=EDGE_CURVE ( 'NONE', #17976, #57167, #16742, .T. ) ;
#19115=CARTESIAN_POINT ( 'NONE',  ( 95.00000000000000000, -212.6630814284392557, 82.97531250086716170 ) ) ;
#19123=CARTESIAN_POINT ( 'NONE',  ( 92.69370383062501162, -211.3315407142195852, 76.36072916753381890 ) ) ;
#19125=CARTESIAN_POINT ( 'NONE',  ( 92.69370383062501162, -208.6684592857803011, 79.58864583420047722 ) ) ;
#19128=CARTESIAN_POINT ( 'NONE',  ( 93.67499999999999716, 87.70503267997126784, 79.31083333333333485 ) ) ;
#19137=CARTESIAN_POINT ( 'NONE',  ( 92.35000000000002274, -211.5299782133524502, 84.41729166840097776 ) ) ;
#19138=CARTESIAN_POINT ( 'NONE',  ( 97.64999999999997726, 91.52997821335252127, 87.83041666666666458 ) ) ;
#19144=( BOUNDED_CURVE ( )  B_SPLINE_CURVE ( 2, ( #49097, #49469, #15258, #72021, #20535, #15638, #26902, #42726, #67133 ),
 .UNSPECIFIED., .F., .F. ) 
 B_SPLINE_CURVE_WITH_KNOTS ( ( 3, 2, 2, 2, 3 ),
 ( 0.4868478063929145838, 0.4939035878617653585, 0.5009593534026471895, 0.5080151189435290204, 0.5080151867253830389 ),
 .UNSPECIFIED. ) 
 CURVE ( )  GEOMETRIC_REPRESENTATION_ITEM ( )  RATIONAL_B_SPLINE_CURVE ( ( 1.000000000000000000, 0.8660254037844387076, 1.000000000000000000, 0.8660254037844387076, 1.000000000000000000, 0.8660254037844387076, 1.000000000000000000, 0.9999987129608440828, 0.9999974259464162740 ) ) 
 REPRESENTATION_ITEM ( '' )  );
#19145=CARTESIAN_POINT ( 'NONE',  ( -93.84685191531252713, 88.00268892867056536, 88.74322916753382628 ) ) ;
#19146=CARTESIAN_POINT ( 'NONE',  ( 92.69370383062498320, 88.66845928578037217, 84.61572916753380014 ) ) ;
#19148=CARTESIAN_POINT ( 'NONE',  ( 96.32499999999998863, 87.70503267997126784, 87.75104166840095843 ) ) ;
#19150=CARTESIAN_POINT ( 'NONE',  ( -92.35000000000005116, 88.47002178664754979, 85.89895833506763267 ) ) ;
#19155=CARTESIAN_POINT ( 'NONE',  ( 93.67499999999998295, 92.29496732002878900, 75.36854166840096525 ) ) ;
#19156=CARTESIAN_POINT ( 'NONE',  ( -92.35000000000005116, 91.52997821335253548, 84.02041666666667652 ) ) ;
#19158=CARTESIAN_POINT ( 'NONE',  ( -97.64999999999996305, -209.9999999999999716, 90.00000000000000000 ) ) ;
#19161=CARTESIAN_POINT ( 'NONE',  ( 93.67500000000001137, -212.2949673200287179, 85.02583333333332405 ) ) ;
#19162=CARTESIAN_POINT ( 'NONE',  ( -97.30629616937497417, -208.6684592857803011, 81.33489583420048064 ) ) ;
#19164=AXIS2_PLACEMENT_3D ( 'NONE', #68286, #43959, #66158 ) ;
#19173=ADVANCED_FACE ( 'NONE', ( #39244 ), #55788, .F. ) ;
#19181=CARTESIAN_POINT ( 'NONE',  ( -95.00000000000002842, 92.66308142843932671, 75.51406250086714067 ) ) ;
#19193=CARTESIAN_POINT ( 'NONE',  ( -93.67499999999998295, -207.7050326799711968, 87.88333333333332575 ) ) ;
#19198=ADVANCED_FACE ( 'NONE', ( #73055 ), #21563, .F. ) ;
#19201=DIRECTION ( 'NONE',  ( -1.000000000000000000, -0.000000000000000000, -0.000000000000000000 ) ) ;
#19204=CARTESIAN_POINT ( 'NONE',  ( 97.65000000000000568, 88.47002178664752137, 83.35895833506764063 ) ) ;
#19209=CARTESIAN_POINT ( 'NONE',  ( 93.84685191531249870, -208.0026889286704943, 83.82197916753381151 ) ) ;
#19210=CARTESIAN_POINT ( 'NONE',  ( 93.84685191531249870, -208.0026889286704943, 89.06072916753382174 ) ) ;
#19211=EDGE_LOOP ( 'NONE', ( #51948, #74242 ) ) ;
#19212=CARTESIAN_POINT ( 'NONE',  ( 93.84685191531249870, -208.0026889286704943, 89.06072916753382174 ) ) ;
#19216=ORIENTED_EDGE ( 'NONE', *, *, #61962, .T. ) ;
#19217=CARTESIAN_POINT ( 'NONE',  ( -93.84685191531252713, 88.00268892867056536, 80.48822916753381662 ) ) ;
#19223=DIRECTION ( 'NONE',  ( 0.000000000000000000, 0.000000000000000000, -1.000000000000000000 ) ) ;
#19230=VECTOR ( 'NONE', #66972, 1000.000000000000000 ) ;
#19233=CARTESIAN_POINT ( 'NONE',  ( 97.30629616937498838, -209.9999999999999716, 77.89531250086714920 ) ) ;
#19244=CARTESIAN_POINT ( 'NONE',  ( 92.34999999999998010, -208.4700217866475214, 76.61208333333333087 ) ) ;
#19246=CARTESIAN_POINT ( 'NONE',  ( -96.15314808468747287, -208.0026889286704943, 80.64697916753381435 ) ) ;
#19248=CARTESIAN_POINT ( 'NONE',  ( -93.84685191531252713, 88.00268892867056536, 79.21822916753382060 ) ) ;
#19250=CARTESIAN_POINT ( 'NONE',  ( 96.15314808468748708, 88.00268892867053694, 82.23447916753380582 ) ) ;
#19254=CARTESIAN_POINT ( 'NONE',  ( 97.64999999999996305, 90.00000034979572661, 77.69687501385438111 ) ) ;
#19257=CARTESIAN_POINT ( 'NONE',  ( -97.30629616937497417, -208.6684592857803295, 81.96989583420047154 ) ) ;
#19263=EDGE_LOOP ( 'NONE', ( #32727, #33696, #5708, #29117 ) ) ;
#19267=CARTESIAN_POINT ( 'NONE',  ( -97.30629616937501680, 91.33154071421968467, 84.50989583420046358 ) ) ;
#19268=CARTESIAN_POINT ( 'NONE',  ( -95.78927932462332251, -207.7213858236420947, 74.85481846778735360 ) ) ;
#19274=CARTESIAN_POINT ( 'NONE',  ( -95.00000000000002842, 92.66308142843932671, 76.14906250086716000 ) ) ;
#19281=CARTESIAN_POINT ( 'NONE',  ( -97.64998344411672804, -208.4700122281038261, 79.23145767387356386 ) ) ;
#19282=CARTESIAN_POINT ( 'NONE',  ( -96.15314808468747287, -208.0026889286704943, 87.15572916753382060 ) ) ;
#19289=CARTESIAN_POINT ( 'NONE',  ( -97.30629616937497417, -208.6684592857803295, 76.41364583420049428 ) ) ;
#19292=CARTESIAN_POINT ( 'NONE',  ( -97.64999999999997726, -209.9999872712514275, 81.82437456149081356 ) ) ;
#19293=CARTESIAN_POINT ( 'NONE',  ( 97.64999999999999147, 90.00000000000002842, 75.71250000000000568 ) ) ;
#19294=CARTESIAN_POINT ( 'NONE',  ( -95.00000000000002842, 86.94004357329504273, 88.33312500173431658 ) ) ;
#19296=CIRCLE ( 'NONE', #68524, 12.75000000000000000 ) ;
#19299=CARTESIAN_POINT ( 'NONE',  ( 95.00000000000000000, -207.3369185715606307, 74.87906250086713555 ) ) ;
#19309=ORIENTED_EDGE ( 'NONE', *, *, #9312, .T. ) ;
#19312=VERTEX_POINT ( 'NONE', #12508 ) ;
#19313=CARTESIAN_POINT ( 'NONE',  ( 96.15314808468748708, 88.00268892867053694, 79.21822916753382060 ) ) ;
#19314=CARTESIAN_POINT ( 'NONE',  ( 95.00000000000000000, -213.0599564267049857, 88.96812500173430749 ) ) ;
#19320=ORIENTED_EDGE ( 'NONE', *, *, #55622, .T. ) ;
#19332=CARTESIAN_POINT ( 'NONE',  ( -96.32499999999996021, -212.2949673200287179, 75.58020833506763836 ) ) ;
#19335=CARTESIAN_POINT ( 'NONE',  ( 93.67499999999998295, 92.29496732002878900, 75.36854166840096525 ) ) ;
#19336=CARTESIAN_POINT ( 'NONE',  ( -95.00000000000002842, 86.94004357329504273, 76.26812500173430465 ) ) ;
#19338=CARTESIAN_POINT ( 'NONE',  ( 97.30629616937498838, 88.66845928578037217, 78.00114583420049996 ) ) ;
#19341=CARTESIAN_POINT ( 'NONE',  ( 92.35000000000000853, -208.4700217866474645, 77.32645833506762756 ) ) ;
#19354=CARTESIAN_POINT ( 'NONE',  ( -97.64999999999996305, -209.9999999999999716, 90.00000000000000000 ) ) ;
#19356=CARTESIAN_POINT ( 'NONE',  ( 97.65000000000000568, -208.4700217866474645, 87.90979166840097037 ) ) ;
#19359=( BOUNDED_CURVE ( )  B_SPLINE_CURVE ( 2, ( #56195, #27618, #50546, #73470, #39281, #58790, #1684, #30204, #2050 ),
 .UNSPECIFIED., .F., .F. ) 
 B_SPLINE_CURVE_WITH_KNOTS ( ( 3, 2, 2, 2, 3 ),
 ( 0.2540073681283125939, 0.2540075594717653429, 0.2610633250126476734, 0.2681190905535300595, 0.2751748541904413536 ),
 .UNSPECIFIED. ) 
 CURVE ( )  GEOMETRIC_REPRESENTATION_ITEM ( )  RATIONAL_B_SPLINE_CURVE ( ( 0.9999927337532750204, 0.9999963667781091026, 1.000000000000000000, 0.8660254037844387076, 1.000000000000000000, 0.8660254037844387076, 1.000000000000000000, 0.8660254037844387076, 1.000000000000000000 ) ) 
 REPRESENTATION_ITEM ( '' )  );
#19360=CARTESIAN_POINT ( 'NONE',  ( -96.15314808468745866, -211.9973110713294489, 75.30239583420048177 ) ) ;
#19371=CARTESIAN_POINT ( 'NONE',  ( -97.64999999999996305, -209.9999999999999716, 76.03000000000000114 ) ) ;
#19375=CARTESIAN_POINT ( 'NONE',  ( 97.30629616937498838, 90.00000000000002842, 84.40406250086715545 ) ) ;
#19376=CARTESIAN_POINT ( 'NONE',  ( -93.84685191531248449, -208.0026889286704943, 87.04989583420048405 ) ) ;
#19377=CARTESIAN_POINT ( 'NONE',  ( 92.35000000007821086, 90.00001303125209517, 79.28395951162845279 ) ) ;
#19381=CARTESIAN_POINT ( 'NONE',  ( -92.34999999999999432, -209.9999999999999716, 81.42749999999999488 ) ) ;
#19382=CARTESIAN_POINT ( 'NONE',  ( -96.15314808468751551, 88.00268892867056536, 76.41364583420048007 ) ) ;
#19385=CARTESIAN_POINT ( 'NONE',  ( 92.69370383062501162, -208.6684592857803011, 88.31989583420046586 ) ) ;
#19386=ORIENTED_EDGE ( 'NONE', *, *, #8056, .F. ) ;
#19393=VECTOR ( 'NONE', #26911, 1000.000000000000000 ) ;
#19398=CARTESIAN_POINT ( 'NONE',  ( 96.15314808468748708, -208.0026889286704943, 80.06489583420048461 ) ) ;
#19400=CARTESIAN_POINT ( 'NONE',  ( -95.00000000000002842, 93.05995642670504253, 76.58562500173430010 ) ) ;
#19402=FACE_OUTER_BOUND ( 'NONE', #11747, .T. ) ;
#19404=CARTESIAN_POINT ( 'NONE',  ( 92.35000000000000853, -209.9999999999999716, 80.47499999999999432 ) ) ;
#19410=CARTESIAN_POINT ( 'NONE',  ( 97.64999999999999147, -209.9999999999999716, 87.14249999999999829 ) ) ;
#19411=EDGE_CURVE ( 'NONE', #23675, #8687, #4237, .T. ) ;
#19412=CARTESIAN_POINT ( 'NONE',  ( -96.15314808468751551, 88.00268892867056536, 82.92239583420048632 ) ) ;
#19416=FACE_OUTER_BOUND ( 'NONE', #8458, .T. ) ;
#19418=CARTESIAN_POINT ( 'NONE',  ( -92.34999999999999432, -209.9999999999999716, 89.12687500173430521 ) ) ;
#19422=CARTESIAN_POINT ( 'NONE',  ( -93.67500000000003979, 92.29496732002878900, 85.42270833506762528 ) ) ;
#19423=CARTESIAN_POINT ( 'NONE',  ( 97.30629616937498838, 91.33154071421968467, 86.36197916753383197 ) ) ;
#19425=CARTESIAN_POINT ( 'NONE',  ( -93.14543241548912533, 88.62117599715713823, 74.79348190356850523 ) ) ;
#19426=FACE_OUTER_BOUND ( 'NONE', #13152, .T. ) ;
#19431=ORIENTED_EDGE ( 'NONE', *, *, #4077, .F. ) ;
#19433=CARTESIAN_POINT ( 'NONE',  ( -97.30629616937497417, -211.3315407142195852, 75.72572916753381378 ) ) ;
#19442=CARTESIAN_POINT ( 'NONE',  ( -97.30629616937497417, -211.3315407142195852, 89.21947916753381946 ) ) ;
#19453=CARTESIAN_POINT ( 'NONE',  ( 97.30629616937498838, 91.33154071421968467, 88.90197916753382401 ) ) ;
#19455=CARTESIAN_POINT ( 'NONE',  ( 93.84685191531248449, 91.99731107132950569, 80.64697916753381435 ) ) ;
#19457=PLANE ( 'NONE',  #44628 ) ;
#19466=DIRECTION ( 'NONE',  ( -0.000000000000000000, -0.000000000000000000, 1.000000000000000000 ) ) ;
#19468=CARTESIAN_POINT ( 'NONE',  ( -92.69370383062505425, 91.33154071421968467, 87.47322916753380184 ) ) ;
#19476=CARTESIAN_POINT ( 'NONE',  ( 95.00000000000000000, -207.3369185715606307, 80.75281250086715090 ) ) ;
#19478=ORIENTED_EDGE ( 'NONE', *, *, #47609, .T. ) ;
#19487=CARTESIAN_POINT ( 'NONE',  ( 93.84685191531249870, -208.0026889286704943, 79.53572916753381605 ) ) ;
#19498=EDGE_LOOP ( 'NONE', ( #27082, #15706, #21413, #12143 ) ) ;
#19500=CARTESIAN_POINT ( 'NONE',  ( 93.67500000000001137, -212.2949673200287179, 82.56520833506762358 ) ) ;
#19502=CARTESIAN_POINT ( 'NONE',  ( 92.34999999999999432, 91.52997821335252127, 86.77208333333334167 ) ) ;
#19503=EDGE_CURVE ( 'NONE', #36972, #56117, #57592, .T. ) ;
#19504=ORIENTED_EDGE ( 'NONE', *, *, #17175, .T. ) ;
#19509=CARTESIAN_POINT ( 'NONE',  ( -97.30629616937501680, 90.00000000000004263, 87.26156250086715715 ) ) ;
#19510=CARTESIAN_POINT ( 'NONE',  ( 97.30629616937498838, 91.33154071421968467, 83.02822916753379445 ) ) ;
#19512=CARTESIAN_POINT ( 'NONE',  ( 97.64999999999999147, 90.00000000000002842, 87.22187500173430408 ) ) ;
#19515=CARTESIAN_POINT ( 'NONE',  ( 95.00000000000000000, -206.9400435732949575, 87.38062500173430180 ) ) ;
#19523=CARTESIAN_POINT ( 'NONE',  ( -93.67500000000003979, 87.70503267997129626, 85.13166666666666060 ) ) ;
#19529=CARTESIAN_POINT ( 'NONE',  ( -97.30629616937497417, -211.3315407142195852, 82.71072916753379900 ) ) ;
#19542=CARTESIAN_POINT ( 'NONE',  ( 92.34999999999999432, 91.52997821335252127, 83.04145833506764518 ) ) ;
#19544=CARTESIAN_POINT ( 'NONE',  ( -97.30629616937501680, 91.33154071421968467, 75.61989583420047722 ) ) ;
#19549=UNCERTAINTY_MEASURE_WITH_UNIT (LENGTH_MEASURE( 1.000000000000000082E-05 ), #25581, 'distance_accuracy_value', 'NONE');
#19557=CARTESIAN_POINT ( 'NONE',  ( 92.35001423713268309, 88.47001356683512086, 75.52729223699087413 ) ) ;
#19558=CARTESIAN_POINT ( 'NONE',  ( -93.67499999999998295, -212.2949673200287179, 87.03666666666666174 ) ) ;
#19561=LINE ( 'NONE', #59429, #14305 ) ;
#19563=CARTESIAN_POINT ( 'NONE',  ( -97.64999999994218172, 89.99998877583867340, 75.47473230081648410 ) ) ;
#19568=VERTEX_POINT ( 'NONE', #41683 ) ;
#19570=( BOUNDED_CURVE ( )  B_SPLINE_CURVE ( 2, ( #6497, #34313, #17032, #46717, #69640, #5763, #6137 ),
 .UNSPECIFIED., .F., .F. ) 
 B_SPLINE_CURVE_WITH_KNOTS ( ( 3, 2, 2, 3 ),
 ( 0.3541666666666665741, 0.3611111111111109939, 0.3680555555555554137, 0.3749999999999998335 ),
 .UNSPECIFIED. ) 
 CURVE ( )  GEOMETRIC_REPRESENTATION_ITEM ( )  RATIONAL_B_SPLINE_CURVE ( ( 1.000000000000002220, 0.8660254037844365982, 1.000000000000000000, 0.8660254037844387076, 1.000000000000000000, 0.8660254037844419273, 0.9999999999999967804 ) ) 
 REPRESENTATION_ITEM ( '' )  );
#19571=CARTESIAN_POINT ( 'NONE',  ( 95.00000000000000000, -207.3369185715606307, 83.13406250086714522 ) ) ;
#19572=CARTESIAN_POINT ( 'NONE',  ( 97.30629616937498838, -208.6684592857803295, 87.63197916753381378 ) ) ;
#19575=CARTESIAN_POINT ( 'NONE',  ( 95.00000000000000000, -207.3369185715606307, 88.37281250086715545 ) ) ;
#19576=ORIENTED_EDGE ( 'NONE', *, *, #73317, .T. ) ;
#19580=CARTESIAN_POINT ( 'NONE',  ( -92.69370383062502583, 88.66845928578038638, 76.09614583420048461 ) ) ;
#19587=CARTESIAN_POINT ( 'NONE',  ( 92.34999999999999432, 89.99999348150291212, 88.17437522718662990 ) ) ;
#19591=CARTESIAN_POINT ( 'NONE',  ( 94.99999999999998579, 90.00000000000002842, 90.00000000000000000 ) ) ;
#19593=CARTESIAN_POINT ( 'NONE',  ( 97.65000000000006253, -211.5299782133523934, 86.45458333333331780 ) ) ;
#19596=ORIENTED_EDGE ( 'NONE', *, *, #55280, .T. ) ;
#19597=ORIENTED_EDGE ( 'NONE', *, *, #55538, .T. ) ;
#19600=CARTESIAN_POINT ( 'NONE',  ( 96.15314808468748708, -208.0026889286704943, 79.27114583420046756 ) ) ;
#19607=CARTESIAN_POINT ( 'NONE',  ( -92.35000000000016485, 88.47002178664749295, 80.73958333333335702 ) ) ;
#19608=DIRECTION ( 'NONE',  ( -0.000000000000000000, -0.000000000000000000, 1.000000000000000000 ) ) ;
#19609=CYLINDRICAL_SURFACE ( 'NONE', #4898, 2.649999999999985700 ) ;
#19611=CARTESIAN_POINT ( 'NONE',  ( -97.30629616937497417, -208.6684592857803011, 80.69989583420048973 ) ) ;
#19612=EDGE_CURVE ( 'NONE', #59733, #21161, #24397, .T. ) ;
#19613=CARTESIAN_POINT ( 'NONE',  ( -95.00000000000002842, 87.33691857156074434, 78.53031250086715431 ) ) ;
#19615=VERTEX_POINT ( 'NONE', #58988 ) ;
#19616=CARTESIAN_POINT ( 'NONE',  ( 92.69370383062498320, 88.66845928578037217, 82.71072916753379900 ) ) ;
#19623=CARTESIAN_POINT ( 'NONE',  ( -97.30629616937495996, -209.9999999999999716, 82.65781250086713783 ) ) ;
#19624=CARTESIAN_POINT ( 'NONE',  ( 97.64999999999999147, 90.00000000000002842, 87.14249999999999829 ) ) ;
#19634=CARTESIAN_POINT ( 'NONE',  ( -95.00000000000002842, 92.66308142843932671, 84.40406250086712703 ) ) ;
#19639=CARTESIAN_POINT ( 'NONE',  ( -95.00000000000002842, 87.33691857156074434, 75.19656250086714522 ) ) ;
#19644=PLANE ( 'NONE',  #30926 ) ;
#19646=CARTESIAN_POINT ( 'NONE',  ( 97.64999999999994884, -211.5299782133524786, 82.64458333333332973 ) ) ;
#19647=CARTESIAN_POINT ( 'NONE',  ( -97.30629616937497417, -211.3315407142195852, 81.59947916753381492 ) ) ;
#19651=CARTESIAN_POINT ( 'NONE',  ( -92.35000000000003695, 90.00000000000004263, 90.00000000000000000 ) ) ;
#19655=DIRECTION ( 'NONE',  ( -1.000000000000000000, -4.476705744456277943E-17, 0.000000000000000000 ) ) ;
#19662=CARTESIAN_POINT ( 'NONE',  ( 92.69370383062501162, -208.6684592857803011, 89.11364583420049712 ) ) ;
#19663=ORIENTED_EDGE ( 'NONE', *, *, #6722, .F. ) ;
#19675=VERTEX_POINT ( 'NONE', #60833 ) ;
#19681=CARTESIAN_POINT ( 'NONE',  ( 97.30629616937498838, 90.00000000000002842, 79.95906250086714806 ) ) ;
#19689=CARTESIAN_POINT ( 'NONE',  ( -92.34999999999999432, -209.9999999999999716, 90.00000000000000000 ) ) ;
#19697=CARTESIAN_POINT ( 'NONE',  ( -94.99999999999997158, -209.9999999999999716, 90.00000000000000000 ) ) ;
#19698=CARTESIAN_POINT ( 'NONE',  ( -93.09170853947338742, -211.8387288276635729, 74.44346887015069569 ) ) ;
#19700=FACE_OUTER_BOUND ( 'NONE', #30121, .T. ) ;
#19702=CARTESIAN_POINT ( 'NONE',  ( 97.64999999999999147, 90.00000000000002842, 77.06187500173429328 ) ) ;
#19703=CARTESIAN_POINT ( 'NONE',  ( -97.65000000000001990, 90.00000000000004263, 74.83937500173429669 ) ) ;
#19706=CARTESIAN_POINT ( 'NONE',  ( 94.99999999999998579, 92.66308142843935514, 75.67281250086716682 ) ) ;
#19709=DIRECTION ( 'NONE',  ( -0.000000000000000000, -0.000000000000000000, 1.000000000000000000 ) ) ;
#19710=CARTESIAN_POINT ( 'NONE',  ( 93.67500000000001137, -207.7050326799711968, 77.27354166840096639 ) ) ;
#19711=LINE ( 'NONE', #47924, #13434 ) ;
#19717=CARTESIAN_POINT ( 'NONE',  ( 7.103376864691351012E-17, -120.0000000000000000, -85.59999999999999432 ) ) ;
#19728=CARTESIAN_POINT ( 'NONE',  ( -92.35000000000003695, 90.00000000000004263, 90.00000000000000000 ) ) ;
#19733=DIRECTION ( 'NONE',  ( 0.000000000000000000, -0.000000000000000000, -1.000000000000000000 ) ) ;
#19735=DIRECTION ( 'NONE',  ( 1.000000000000000000, 0.000000000000000000, 0.000000000000000000 ) ) ;
#19740=CARTESIAN_POINT ( 'NONE',  ( 94.99999999999998579, 87.33691857156068750, 82.97531250086714749 ) ) ;
#19741=CARTESIAN_POINT ( 'NONE',  ( -92.69370383062498320, -209.9999999999999716, 87.57906250086715261 ) ) ;
#19744=DIRECTION ( 'NONE',  ( -0.000000000000000000, -0.000000000000000000, 1.000000000000000000 ) ) ;
#19745=CARTESIAN_POINT ( 'NONE',  ( -94.99999999999997158, -206.9400435732949575, 80.31624999999998238 ) ) ;
#19748=EDGE_CURVE ( 'NONE', #5237, #27457, #53381, .T. ) ;
#19749=CARTESIAN_POINT ( 'NONE',  ( 93.84685191531251292, -211.9973110713294489, 84.03364583420047040 ) ) ;
#19757=ADVANCED_FACE ( 'NONE', ( #32234, #43561 ), #55187, .T. ) ;
#19763=CARTESIAN_POINT ( 'NONE',  ( 97.30629616937498838, -211.3315407142195852, 78.00114583420049996 ) ) ;
#19768=ADVANCED_FACE ( 'NONE', ( #8589 ), #25500, .F. ) ;
#19769=CARTESIAN_POINT ( 'NONE',  ( -92.35000000010070664, 90.00002309722640348, 83.41187580057902551 ) ) ;
#19770=CARTESIAN_POINT ( 'NONE',  ( 96.32499999999998863, -207.7050326799711968, 81.53333333333333144 ) ) ;
#19773=ORIENTED_EDGE ( 'NONE', *, *, #68582, .F. ) ;
#19778=CARTESIAN_POINT ( 'NONE',  ( -97.30629616937501680, 90.00000000000004263, 83.45156250086715488 ) ) ;
#19781=CARTESIAN_POINT ( 'NONE',  ( 97.64999999999997726, 91.52997821335252127, 75.13041666666666174 ) ) ;
#19783=CARTESIAN_POINT ( 'NONE',  ( -92.34999999999999432, -211.5299782133524502, 84.62895833506763665 ) ) ;
#19785=ORIENTED_EDGE ( 'NONE', *, *, #27570, .T. ) ;
#19789=CARTESIAN_POINT ( 'NONE',  ( -92.35000000000005116, 91.52997821335253548, 85.36979166840096411 ) ) ;
#19790=( BOUNDED_CURVE ( )  B_SPLINE_CURVE ( 2, ( #59520, #19646, #60270, #41848, #37700, #60632, #13275 ),
 .UNSPECIFIED., .F., .F. ) 
 B_SPLINE_CURVE_WITH_KNOTS ( ( 3, 2, 2, 3 ),
 ( 0.4791666666666668517, 0.4861111111111112160, 0.4930555555555556357, 0.5000000000000000000 ),
 .UNSPECIFIED. ) 
 CURVE ( )  GEOMETRIC_REPRESENTATION_ITEM ( )  RATIONAL_B_SPLINE_CURVE ( ( 0.9999999999999967804, 0.8660254037844419273, 1.000000000000000000, 0.8660254037844387076, 1.000000000000000000, 0.8660254037844387076, 1.000000000000000000 ) ) 
 REPRESENTATION_ITEM ( '' )  );
#19793=CARTESIAN_POINT ( 'NONE',  ( 92.69370383062498320, 88.66845928578037217, 86.04447916753382231 ) ) ;
#19795=CARTESIAN_POINT ( 'NONE',  ( -92.91683521822002945, 88.99941091287938377, 74.79348190356857629 ) ) ;
#19796=CARTESIAN_POINT ( 'NONE',  ( 92.35000000019411459, -210.0000198427945861, 86.27002759516706476 ) ) ;
#19797=CYLINDRICAL_SURFACE ( 'NONE', #72083, 2.649999999999985700 ) ;
#19807=CARTESIAN_POINT ( 'NONE',  ( -96.15314808468747287, -208.0026889286704943, 85.25072916753381946 ) ) ;
#19811=AXIS2_PLACEMENT_3D ( 'NONE', #49649, #72577, #21076 ) ;
#19815=AXIS2_PLACEMENT_3D ( 'NONE', #67570, #26960, #16065 ) ;
#19816=CARTESIAN_POINT ( 'NONE',  ( 92.69370383062498320, 90.00000000000002842, 88.53156250086716739 ) ) ;
#19817=DIRECTION ( 'NONE',  ( 0.000000000000000000, 0.000000000000000000, -1.000000000000000000 ) ) ;
#19818=CARTESIAN_POINT ( 'NONE',  ( 92.69370383062498320, 91.33154071421968467, 81.96989583420047154 ) ) ;
#19821=VECTOR ( 'NONE', #54049, 1000.000000000000000 ) ;
#19825=EDGE_CURVE ( 'NONE', #35387, #20380, #42652, .T. ) ;
#19828=LINE ( 'NONE', #65714, #26536 ) ;
#19830=CARTESIAN_POINT ( 'NONE',  ( -96.15314808468752972, 91.99731107132950569, 86.36197916753381776 ) ) ;
#19839=DIRECTION ( 'NONE',  ( -0.000000000000000000, -0.000000000000000000, 1.000000000000000000 ) ) ;
#19843=CARTESIAN_POINT ( 'NONE',  ( 92.69370383062501162, -209.9999999999999716, 83.45156250086715488 ) ) ;
#19848=ADVANCED_FACE ( 'NONE', ( #67041 ), #16283, .F. ) ;
#19853=ORIENTED_EDGE ( 'NONE', *, *, #14537, .F. ) ;
#19856=CARTESIAN_POINT ( 'NONE',  ( 92.69370383062501162, -211.3315407142195852, 76.51947916753381662 ) ) ;
#19860=EDGE_CURVE ( 'NONE', #72633, #3278, #55600, .T. ) ;
#19868=CARTESIAN_POINT ( 'NONE',  ( 96.32499999999998863, -207.7050326799711968, 84.78770833506763438 ) ) ;
#19869=CARTESIAN_POINT ( 'NONE',  ( 97.64999999999997726, 88.47002178664753558, 86.45458333333333201 ) ) ;
#19876=CARTESIAN_POINT ( 'NONE',  ( -92.69370383062505425, 91.33154071421968467, 86.36197916753383197 ) ) ;
#19877=CARTESIAN_POINT ( 'NONE',  ( 92.69370383062498320, 90.00000000000002842, 82.65781250086713783 ) ) ;
#19878=ORIENTED_EDGE ( 'NONE', *, *, #35542, .F. ) ;
#19880=CARTESIAN_POINT ( 'NONE',  ( 94.99999999999998579, 93.05995642670504253, 84.20562500173429044 ) ) ;
#19883=CARTESIAN_POINT ( 'NONE',  ( 97.64997150697853101, -208.4700053361938217, 87.27479280632981329 ) ) ;
#19890=CARTESIAN_POINT ( 'NONE',  ( -93.67500000000003979, 87.70503267997129626, 83.22666666666665947 ) ) ;
#19896=CARTESIAN_POINT ( 'NONE',  ( -94.99999999999997158, -207.3369185715606307, 78.05406250086714692 ) ) ;
#19908=CARTESIAN_POINT ( 'NONE',  ( -97.30629616937501680, 90.00000000000004263, 89.16656250086715829 ) ) ;
#19914=AXIS2_PLACEMENT_3D ( 'NONE', #50103, #21542, #38847 ) ;
#19918=ADVANCED_FACE ( 'NONE', ( #55396 ), #3917, .F. ) ;
#19919=CARTESIAN_POINT ( 'NONE',  ( 95.00000000000000000, -213.0599564267049857, 78.72875000000001933 ) ) ;
#19922=CARTESIAN_POINT ( 'NONE',  ( -94.99999999999997158, -206.9400435732949575, 86.66624999999999091 ) ) ;
#19930=VERTEX_POINT ( 'NONE', #62923 ) ;
#19933=CARTESIAN_POINT ( 'NONE',  ( 92.35001469785311201, -208.4700133008379908, 81.77145774807790701 ) ) ;
#19936=VERTEX_POINT ( 'NONE', #17397 ) ;
#19940=CARTESIAN_POINT ( 'NONE',  ( 93.84685191531249870, -208.0026889286704943, 80.64697916753381435 ) ) ;
#19941=CARTESIAN_POINT ( 'NONE',  ( 95.00000000000000000, -207.3369185715606307, 88.37281250086715545 ) ) ;
#19943=CARTESIAN_POINT ( 'NONE',  ( 97.30629616937498838, -208.6684592857803011, 86.99697916753382287 ) ) ;
#19947=EDGE_CURVE ( 'NONE', #1126, #18290, #23053, .T. ) ;
#19948=EDGE_CURVE ( 'NONE', #32439, #40132, #19570, .T. ) ;
#19949=CARTESIAN_POINT ( 'NONE',  ( -93.84685191531252713, 88.00268892867056536, 76.04322916753382344 ) ) ;
#19961=CARTESIAN_POINT ( 'NONE',  ( 92.35000000000000853, -209.9999999999999716, 86.18999999999999773 ) ) ;
#19965=ORIENTED_EDGE ( 'NONE', *, *, #69130, .F. ) ;
#19966=CARTESIAN_POINT ( 'NONE',  ( 92.69370383062501162, -208.6684592857803011, 78.79489583420047438 ) ) ;
#19976=CARTESIAN_POINT ( 'NONE',  ( -94.99999999999997158, -206.9400435732949575, 88.65062500173428361 ) ) ;
#19978=CARTESIAN_POINT ( 'NONE',  ( -97.30629616937497417, -208.6684592857803011, 81.33489583420048064 ) ) ;
#19979=CARTESIAN_POINT ( 'NONE',  ( -95.00000000000002842, 92.66308142843932671, 79.48281250086715488 ) ) ;
#19982=CARTESIAN_POINT ( 'NONE',  ( 97.30629616937498838, 91.33154071421968467, 79.85322916753379729 ) ) ;
#19989=CARTESIAN_POINT ( 'NONE',  ( -97.30629616937495996, -209.9999999999999716, 81.38781250086714181 ) ) ;
#19990=CARTESIAN_POINT ( 'NONE',  ( -94.99999999999997158, -213.0599564267049857, 89.52374999999999261 ) ) ;
#19995=EDGE_LOOP ( 'NONE', ( #34649, #30436, #14690, #10513 ) ) ;
#19997=CARTESIAN_POINT ( 'NONE',  ( -96.32500000000001705, 87.70503267997129626, 75.50083333333331836 ) ) ;
#19998=CARTESIAN_POINT ( 'NONE',  ( -97.64997399466426486, 88.47000677245993927, 84.41729270697882725 ) ) ;
#19999=CARTESIAN_POINT ( 'NONE',  ( -92.69370383062502583, 88.66845928578038638, 83.55739583420047722 ) ) ;
#20008=CARTESIAN_POINT ( 'NONE',  ( -97.64999999960637922, 90.00002930319634231, 82.45844277051273252 ) ) ;
#20010=CYLINDRICAL_SURFACE ( 'NONE', #57398, 2.649999999999999467 ) ;
#20012=CARTESIAN_POINT ( 'NONE',  ( 92.34999999999999432, 90.00000000000002842, 86.18999999999999773 ) ) ;
#20013=CARTESIAN_POINT ( 'NONE',  ( -93.84685191531247028, -211.9973110713294489, 83.66322916753382799 ) ) ;
#20016=( BOUNDED_CURVE ( )  B_SPLINE_CURVE ( 2, ( #14274, #25558, #37227, #39452, #62012, #10121, #44724 ),
 .UNSPECIFIED., .F., .F. ) 
 B_SPLINE_CURVE_WITH_KNOTS ( ( 3, 2, 2, 3 ),
 ( 0.1905056698837213069, 0.1975614351447063655, 0.2046172006855887515, 0.2116728463006668226 ),
 .UNSPECIFIED. ) 
 CURVE ( )  GEOMETRIC_REPRESENTATION_ITEM ( )  RATIONAL_B_SPLINE_CURVE ( ( 1.000000000000000000, 0.8660254037844387076, 1.000000000000000000, 0.8660254037844387076, 1.000000000000000000, 0.8660276809308541379, 0.9999954457845777744 ) ) 
 REPRESENTATION_ITEM ( '' )  );
#20019=CARTESIAN_POINT ( 'NONE',  ( 93.84685191531248449, 88.00268892867053694, 75.30239583420048177 ) ) ;
#20025=CARTESIAN_POINT ( 'NONE',  ( -97.65000000000001990, 90.00000000000004263, 78.57000000000000739 ) ) ;
#20029=CARTESIAN_POINT ( 'NONE',  ( 96.15314808468750130, -211.9973110713294489, 88.74322916753382628 ) ) ;
#20030=EDGE_CURVE ( 'NONE', #27941, #39489, #15824, .T. ) ;
#20031=ORIENTED_EDGE ( 'NONE', *, *, #53988, .T. ) ;
#20033=CARTESIAN_POINT ( 'NONE',  ( 92.35000000000002274, -208.4700217866474645, 87.40708333333333258 ) ) ;
#20040=CARTESIAN_POINT ( 'NONE',  ( -92.35000000000003695, 90.00000000000004263, 84.60249999999999204 ) ) ;
#20047=ORIENTED_EDGE ( 'NONE', *, *, #19860, .F. ) ;
#20048=CARTESIAN_POINT ( 'NONE',  ( -23.50000000000000355, -120.0000000000000000, -64.00000000000000000 ) ) ;
#20052=CARTESIAN_POINT ( 'NONE',  ( 92.69370383062498320, 91.33154071421968467, 78.95364583420048632 ) ) ;
#20056=VERTEX_POINT ( 'NONE', #56893 ) ;
#20058=CARTESIAN_POINT ( 'NONE',  ( -23.50000000000000355, -120.0000000000000000, -80.00000000000000000 ) ) ;
#20067=CARTESIAN_POINT ( 'NONE',  ( -92.34999999999999432, -208.4700217866474645, 74.57479166840096241 ) ) ;
#20068=CARTESIAN_POINT ( 'NONE',  ( -92.69370383062502583, 88.66845928578038638, 87.52614583420049144 ) ) ;
#20071=CARTESIAN_POINT ( 'NONE',  ( 94.99999999999998579, 86.94004357329500010, 74.99812500173430863 ) ) ;
#20072=CARTESIAN_POINT ( 'NONE',  ( -92.69370383062504004, 90.00000000000004263, 88.69031250086715090 ) ) ;
#20074=CARTESIAN_POINT ( 'NONE',  ( 92.69370383062498320, 90.00000000000002842, 77.10156250086714635 ) ) ;
#20081=CARTESIAN_POINT ( 'NONE',  ( -93.67500000000003979, 92.29496732002878900, 89.15333333333333599 ) ) ;
#20083=CARTESIAN_POINT ( 'NONE',  ( -92.35000000000000853, -211.5299782133524218, 87.72458333333332803 ) ) ;
#20091=CARTESIAN_POINT ( 'NONE',  ( -95.00000000000002842, 93.05995642670504253, 86.11062500173430578 ) ) ;
#20092=EDGE_CURVE ( 'NONE', #65477, #21000, #60449, .T. ) ;
#20095=CARTESIAN_POINT ( 'NONE',  ( -97.30629616937495996, -209.9999999999999716, 75.83156250086716454 ) ) ;
#20102=EDGE_CURVE ( 'NONE', #33622, #42810, #54209, .T. ) ;
#20105=CARTESIAN_POINT ( 'NONE',  ( -0.0004442498525516064278, 0.001194404164626844313, -80.00000000000001421 ) ) ;
#20111=CARTESIAN_POINT ( 'NONE',  ( 93.84685191531248449, 91.99731107132950569, 83.98072916753382344 ) ) ;
#20112=CARTESIAN_POINT ( 'NONE',  ( -93.84685191531248449, -208.0026889286704943, 81.96989583420048575 ) ) ;
#20115=CARTESIAN_POINT ( 'NONE',  ( -92.34999999999999432, -209.9999999999999716, 81.42749999999999488 ) ) ;
#20116=CARTESIAN_POINT ( 'NONE',  ( -96.32499999999996021, -207.7050326799711968, 79.09916666666666174 ) ) ;
#20118=CARTESIAN_POINT ( 'NONE',  ( 93.84685191531249870, -208.0026889286704943, 83.82197916753381151 ) ) ;
#20122=CARTESIAN_POINT ( 'NONE',  ( 97.08316478178004161, 88.99941091287935535, 74.79348190356853365 ) ) ;
#20126=AXIS2_PLACEMENT_3D ( 'NONE', #10777, #29161, #51738 ) ;
#20132=CARTESIAN_POINT ( 'NONE',  ( 95.00000000000000000, -207.3369185715606307, 77.57781250086715374 ) ) ;
#20136=CARTESIAN_POINT ( 'NONE',  ( 96.32499999999998863, 87.70503267997126784, 76.87666666666666515 ) ) ;
#20138=CARTESIAN_POINT ( 'NONE',  ( 96.32499999999998863, -207.7050326799711968, 80.89833333333332632 ) ) ;
#20146=CARTESIAN_POINT ( 'NONE',  ( -93.84685191531252713, 88.00268892867056536, 85.56822916753381492 ) ) ;
#20150=CARTESIAN_POINT ( 'NONE',  ( 97.64999999999997726, 88.47002178664753558, 76.29458333333333542 ) ) ;
#20155=CARTESIAN_POINT ( 'NONE',  ( -94.99999999999997158, -213.0599564267049857, 87.06312500173430635 ) ) ;
#20160=CARTESIAN_POINT ( 'NONE',  ( -97.65000000000001990, 88.47002178664754979, 87.59229166840096070 ) ) ;
#20163=CARTESIAN_POINT ( 'NONE',  ( 93.84685191531248449, 88.00268892867053694, 85.46239583420047836 ) ) ;
#20177=CARTESIAN_POINT ( 'NONE',  ( -97.64999999999996305, -209.9999999999999716, 83.01499999999998636 ) ) ;
#20178=CARTESIAN_POINT ( 'NONE',  ( -96.15314808468745866, -211.9973110713294489, 84.82739583420048746 ) ) ;
#20181=LINE ( 'NONE', #43145, #52486 ) ;
#20184=EDGE_CURVE ( 'NONE', #55652, #29642, #1993, .T. ) ;
#20186=CARTESIAN_POINT ( 'NONE',  ( 93.84685191531248449, 91.99731107132950569, 89.69572916753382685 ) ) ;
#20189=CARTESIAN_POINT ( 'NONE',  ( 97.30629616937498838, 90.00000000000002842, 76.62531250086713897 ) ) ;
#20194=CARTESIAN_POINT ( 'NONE',  ( 93.98225765065670601, 92.19538700400579501, 74.85985921673514554 ) ) ;
#20200=VECTOR ( 'NONE', #572, 1000.000000000000000 ) ;
#20202=CARTESIAN_POINT ( 'NONE',  ( -93.84685191531254134, 91.99731107132950569, 83.71614583420047495 ) ) ;
#20203=CARTESIAN_POINT ( 'NONE',  ( -90.00000000000002842, 95.00000000000002842, 90.00000000000000000 ) ) ;
#20206=CARTESIAN_POINT ( 'NONE',  ( 92.35000000039364920, -209.9999706968037287, 82.45844277051352833 ) ) ;
#20208=EDGE_CURVE ( 'NONE', #68971, #6723, #41803, .T. ) ;
#20212=CARTESIAN_POINT ( 'NONE',  ( 94.99999999999998579, 93.05995642670504253, 85.39624999999998067 ) ) ;
#20213=CARTESIAN_POINT ( 'NONE',  ( 96.82636346428385821, 88.24022384386941553, 74.93163452119478052 ) ) ;
#20214=CARTESIAN_POINT ( 'NONE',  ( 93.84685191531251292, -211.9973110713294489, 80.38239583420048007 ) ) ;
#20219=( BOUNDED_CURVE ( )  B_SPLINE_CURVE ( 2, ( #14711, #4196, #9814, #3459, #60596, #72581, #44784 ),
 .UNSPECIFIED., .F., .F. ) 
 B_SPLINE_CURVE_WITH_KNOTS ( ( 3, 2, 2, 3 ),
 ( 0.3541666666666665741, 0.3611111111111109939, 0.3680555555555554137, 0.3749999999999998335 ),
 .UNSPECIFIED. ) 
 CURVE ( )  GEOMETRIC_REPRESENTATION_ITEM ( )  RATIONAL_B_SPLINE_CURVE ( ( 1.000000000000002220, 0.8660254037844365982, 1.000000000000000000, 0.8660254037844387076, 1.000000000000000000, 0.8660254037844419273, 0.9999999999999967804 ) ) 
 REPRESENTATION_ITEM ( '' )  );
#20224=CARTESIAN_POINT ( 'NONE',  ( 97.30629616937498838, -208.6684592857803011, 76.83697916753382628 ) ) ;
#20230=ORIENTED_EDGE ( 'NONE', *, *, #21925, .T. ) ;
#20236=CARTESIAN_POINT ( 'NONE',  ( 92.35000000000000853, -209.9999999999999716, 84.36437500173430237 ) ) ;
#20237=CARTESIAN_POINT ( 'NONE',  ( 96.32499999999997442, 92.29496732002878900, 84.07333333333333769 ) ) ;
#20239=CARTESIAN_POINT ( 'NONE',  ( -89.99999999999998579, -124.0000000000000142, -40.00000000000002132 ) ) ;
#20242=ORIENTED_EDGE ( 'NONE', *, *, #15627, .F. ) ;
#20243=CARTESIAN_POINT ( 'NONE',  ( -93.84685191531254134, 91.99731107132950569, 87.68489583420048916 ) ) ;
#20244=CARTESIAN_POINT ( 'NONE',  ( 96.15314808468748708, 91.99731107132950569, 81.81114583420047381 ) ) ;
#20245=EDGE_LOOP ( 'NONE', ( #68135, #5492, #21895, #3823 ) ) ;
#20247=CARTESIAN_POINT ( 'NONE',  ( 97.64999999999999147, 90.00000000000002842, 82.77687500173431090 ) ) ;
#20249=ADVANCED_FACE ( 'NONE', ( #67986 ), #5222, .F. ) ;
#20262=CARTESIAN_POINT ( 'NONE',  ( -97.65000000000001990, 90.00000000000004263, 84.28499999999999659 ) ) ;
#20265=CARTESIAN_POINT ( 'NONE',  ( -92.34999999999999432, -208.4700217866474645, 80.92479166840097093 ) ) ;
#20267=CARTESIAN_POINT ( 'NONE',  ( 96.32499999999998863, 87.70503267997126784, 89.02104166840096866 ) ) ;
#20269=CARTESIAN_POINT ( 'NONE',  ( -0.0004442498525516064278, 0.001194404164626844313, -80.00000000000000000 ) ) ;
#20270=CARTESIAN_POINT ( 'NONE',  ( -93.84685191531247028, -211.9973110713294489, 77.78947916753381264 ) ) ;
#20274=FACE_OUTER_BOUND ( 'NONE', #52240, .T. ) ;
#20278=DIRECTION ( 'NONE',  ( -0.000000000000000000, -0.000000000000000000, 1.000000000000000000 ) ) ;
#20279=CARTESIAN_POINT ( 'NONE',  ( 97.30629616937498838, 90.00000000000002842, 87.42031250086714067 ) ) ;
#20284=CARTESIAN_POINT ( 'NONE',  ( -92.69370383062502583, 91.33154071421968467, 76.04322916753380923 ) ) ;
#20296=LINE ( 'NONE', #33422, #4069 ) ;
#20300=CARTESIAN_POINT ( 'NONE',  ( 93.67499999999999716, 87.70503267997126784, 75.58020833506763836 ) ) ;
#20301=CARTESIAN_POINT ( 'NONE',  ( -97.64999999999994884, -208.4700217866474645, 88.04208333333332348 ) ) ;
#20302=CARTESIAN_POINT ( 'NONE',  ( -93.62329079302944024, 87.70919997534043944, 75.00000000000000000 ) ) ;
#20309=PRESENTATION_STYLE_ASSIGNMENT (( #7922 ) ) ;
#20310=CARTESIAN_POINT ( 'NONE',  ( -96.32500000000001705, 92.29496732002878900, 84.81416666666666515 ) ) ;
#20313=AXIS2_PLACEMENT_3D ( 'NONE', #11200, #27747, #34126 ) ;
#20320=ORIENTED_EDGE ( 'NONE', *, *, #17223, .F. ) ;
#20322=CARTESIAN_POINT ( 'NONE',  ( 93.84685191531249870, -208.0026889286704943, 81.28197916753380525 ) ) ;
#20323=CARTESIAN_POINT ( 'NONE',  ( 97.30629616937498838, -208.6684592857803295, 83.82197916753382572 ) ) ;
#20325=CARTESIAN_POINT ( 'NONE',  ( 97.30629616937498838, -208.6684592857803011, 85.72697916753381264 ) ) ;
#20329=CARTESIAN_POINT ( 'NONE',  ( -93.84685191531252713, 88.00268892867056536, 78.58322916753382970 ) ) ;
#20334=CARTESIAN_POINT ( 'NONE',  ( -2.500000000000015543, -73.00000000000001421, -204.9999999999999716 ) ) ;
#20341=EDGE_LOOP ( 'NONE', ( #4915, #11263, #59812, #64820 ) ) ;
#20343=EDGE_CURVE ( 'NONE', #67844, #10235, #34024, .T. ) ;
#20347=CARTESIAN_POINT ( 'NONE',  ( 95.00000000000000000, -212.6630814284392557, 79.00656250086713328 ) ) ;
#20348=DIRECTION ( 'NONE',  ( -0.000000000000000000, -0.000000000000000000, -1.000000000000000000 ) ) ;
#20357=VECTOR ( 'NONE', #57933, 1000.000000000000000 ) ;
#20359=DIRECTION ( 'NONE',  ( 1.000000000000000000, 0.000000000000000000, 0.000000000000000000 ) ) ;
#20362=CARTESIAN_POINT ( 'NONE',  ( -96.15314808468751551, 88.00268892867056536, 80.38239583420048007 ) ) ;
#20364=CARTESIAN_POINT ( 'NONE',  ( 97.30629616937498838, 90.00000000000002842, 76.62531250086713897 ) ) ;
#20367=CARTESIAN_POINT ( 'NONE',  ( -94.99999999999997158, -212.6630814284392557, 87.89656250086713385 ) ) ;
#20371=CARTESIAN_POINT ( 'NONE',  ( -97.30629616937497417, -211.3315407142195852, 82.07572916753382231 ) ) ;
#20373=ADVANCED_FACE ( 'NONE', ( #40156 ), #27371, .F. ) ;
#20380=VERTEX_POINT ( 'NONE', #44696 ) ;
#20386=CARTESIAN_POINT ( 'NONE',  ( -96.15314808468752972, 91.99731107132950569, 86.36197916753381776 ) ) ;
#20387=CARTESIAN_POINT ( 'NONE',  ( -95.67252605959615153, -207.6887180216938020, 74.85222950654856788 ) ) ;
#20402=CARTESIAN_POINT ( 'NONE',  ( -92.69370383062498320, -209.9999999999999716, 83.76906250086716454 ) ) ;
#20406=VECTOR ( 'NONE', #60999, 1000.000000000000000 ) ;
#20407=CARTESIAN_POINT ( 'NONE',  ( -93.33921851433959205, -211.6002521295065435, 74.80065602173004891 ) ) ;
#20408=CARTESIAN_POINT ( 'NONE',  ( -92.34999999999998010, 88.47002178664760663, 88.99458333333333826 ) ) ;
#20410=EDGE_CURVE ( 'NONE', #23771, #2356, #69820, .T. ) ;
#20411=CARTESIAN_POINT ( 'NONE',  ( -92.34999999999999432, -211.5299782133524218, 82.08895833506764461 ) ) ;
#20422=VERTEX_POINT ( 'NONE', #53281 ) ;
#20425=FACE_BOUND ( 'NONE', #4201, .T. ) ;
#20434=CYLINDRICAL_SURFACE ( 'NONE', #67150, 2.649999999999999467 ) ;
#20437=CARTESIAN_POINT ( 'NONE',  ( 92.69370383062498320, 90.00000000000002842, 75.19656250086714522 ) ) ;
#20441=VERTEX_POINT ( 'NONE', #52916 ) ;
#20446=CARTESIAN_POINT ( 'NONE',  ( 92.69370383062501162, -211.3315407142195852, 89.06072916753379332 ) ) ;
#20450=CARTESIAN_POINT ( 'NONE',  ( -97.51367041768835975, 89.99999999999990052, 74.91808492278043730 ) ) ;
#20453=DIRECTION ( 'NONE',  ( -0.000000000000000000, -0.000000000000000000, 1.000000000000000000 ) ) ;
#20457=CARTESIAN_POINT ( 'NONE',  ( -96.32499999999996021, -212.2949673200287179, 77.48520833506763950 ) ) ;
#20458=CARTESIAN_POINT ( 'NONE',  ( -92.69370383062502583, 88.66845928578038638, 88.16114583420048234 ) ) ;
#20460=CARTESIAN_POINT ( 'NONE',  ( 97.30629616937498838, 88.66845928578037217, 88.63739583420047552 ) ) ;
#20461=CARTESIAN_POINT ( 'NONE',  ( -92.69370383062502583, 88.66845928578038638, 87.36739583420047950 ) ) ;
#20463=CARTESIAN_POINT ( 'NONE',  ( 92.69370383062498320, 90.00000000000002842, 76.46656250086715545 ) ) ;
#20465=CARTESIAN_POINT ( 'NONE',  ( 95.00000000000000000, -209.9999999999999716, 90.00000000000000000 ) ) ;
#20466=CARTESIAN_POINT ( 'NONE',  ( -97.64999999999996305, -209.9999999999999716, 86.82500000000000284 ) ) ;
#20481=CARTESIAN_POINT ( 'NONE',  ( -92.69370383062498320, -208.6684592857803011, 74.93197916753381094 ) ) ;
#20482=( BOUNDED_CURVE ( )  B_SPLINE_CURVE ( 2, ( #25530, #13868, #8622, #19515, #14620, #19883, #48098 ),
 .UNSPECIFIED., .F., .F. ) 
 B_SPLINE_CURVE_WITH_KNOTS ( ( 3, 2, 2, 3 ),
 ( 0.1270039290051390157, 0.1340595452767650575, 0.1411153108176474713, 0.1481709449575358828 ),
 .UNSPECIFIED. ) 
 CURVE ( )  GEOMETRIC_REPRESENTATION_ITEM ( )  RATIONAL_B_SPLINE_CURVE ( ( 0.9999943314824852880, 0.8660282381031578769, 1.000000000000000000, 0.8660254037844387076, 1.000000000000000000, 0.8660278988213007123, 0.9999950100192072089 ) ) 
 REPRESENTATION_ITEM ( '' )  );
#20484=CARTESIAN_POINT ( 'NONE',  ( -92.69370383062504004, 90.00000000000004263, 82.34031250086714238 ) ) ;
#20494=CARTESIAN_POINT ( 'NONE',  ( -97.64999999999996305, -209.9999999999999716, 87.45999999999999375 ) ) ;
#20497=CARTESIAN_POINT ( 'NONE',  ( -97.64999999993855795, 90.00001182123732235, 81.82400613091868991 ) ) ;
#20499=CARTESIAN_POINT ( 'NONE',  ( 94.99999999999998579, 92.66308142843932671, 79.48281250086715488 ) ) ;
#20500=CARTESIAN_POINT ( 'NONE',  ( -93.84685191531248449, -208.0026889286704943, 84.50989583420049200 ) ) ;
#20503=CARTESIAN_POINT ( 'NONE',  ( -92.34999999999993747, -211.5299782133523934, 81.37458333333333371 ) ) ;
#20504=CARTESIAN_POINT ( 'NONE',  ( -96.32499999999996021, -207.7050326799711968, 77.19416666666666060 ) ) ;
#20506=CARTESIAN_POINT ( 'NONE',  ( 96.15314808468748708, -208.0026889286704943, 82.44614583420046472 ) ) ;
#20508=CARTESIAN_POINT ( 'NONE',  ( 97.30629616937500259, 90.00000000000002842, 74.79348190356851944 ) ) ;
#20509=ORIENTED_EDGE ( 'NONE', *, *, #50735, .F. ) ;
#20514=CARTESIAN_POINT ( 'NONE',  ( -94.99999999999997158, -209.9999999999999716, 90.00000000000000000 ) ) ;
#20517=CARTESIAN_POINT ( 'NONE',  ( 97.30629616937498838, -211.3315407142195852, 78.63614583420046245 ) ) ;
#20519=CARTESIAN_POINT ( 'NONE',  ( -92.35000000000400178, 89.99999541993113894, 76.42687486206344261 ) ) ;
#20520=CARTESIAN_POINT ( 'NONE',  ( -97.51895106303135208, 89.82936612246383845, 74.92125785461006160 ) ) ;
#20523=CARTESIAN_POINT ( 'NONE',  ( 95.00000000000000000, -213.0599564267049857, 79.99874999999998693 ) ) ;
#20527=EDGE_LOOP ( 'NONE', ( #22232, #50764, #19785, #43190 ) ) ;
#20530=DIRECTION ( 'NONE',  ( -0.000000000000000000, -0.000000000000000000, 1.000000000000000000 ) ) ;
#20533=CARTESIAN_POINT ( 'NONE',  ( -95.00000000000002842, 92.66308142843932671, 83.29281250086717137 ) ) ;
#20535=CARTESIAN_POINT ( 'NONE',  ( -96.32500000000001705, 87.70503267997129626, 81.93020833506763267 ) ) ;
#20540=ADVANCED_FACE ( 'NONE', ( #23977 ), #69460, .F. ) ;
#20541=EDGE_LOOP ( 'NONE', ( #45021, #49319, #33171, #13226 ) ) ;
#20542=CARTESIAN_POINT ( 'NONE',  ( -97.64999999999994884, -208.4700217866474645, 84.94645833506763211 ) ) ;
#20546=CARTESIAN_POINT ( 'NONE',  ( -93.67500000000003979, 92.29496732002878900, 82.24770833506762813 ) ) ;
#20549=CARTESIAN_POINT ( 'NONE',  ( 92.69370383062498320, 88.66845928578037217, 87.31447916753381833 ) ) ;
#20555=ORIENTED_EDGE ( 'NONE', *, *, #52004, .T. ) ;
#20562=EDGE_CURVE ( 'NONE', #66356, #17407, #59691, .T. ) ;
#20565=CARTESIAN_POINT ( 'NONE',  ( -92.69370383062498320, -211.3315407142195852, 84.35114583420049428 ) ) ;
#20566=ORIENTED_EDGE ( 'NONE', *, *, #68576, .T. ) ;
#20569=AXIS2_PLACEMENT_3D ( 'NONE', #35920, #18992, #29530 ) ;
#20574=EDGE_CURVE ( 'NONE', #6723, #5282, #44640, .T. ) ;
#20578=CARTESIAN_POINT ( 'NONE',  ( 92.69370383062498320, 90.00000000000002842, 78.84781250086714977 ) ) ;
#20580=CARTESIAN_POINT ( 'NONE',  ( 92.35001072511518316, 91.52998440550067016, 86.85145790673759336 ) ) ;
#20586=CARTESIAN_POINT ( 'NONE',  ( -2.499999999999965361, 90.00000000000000000, -310.0000000000000000 ) ) ;
#20589=CARTESIAN_POINT ( 'NONE',  ( -92.69370383062505425, 88.66845928578038638, 83.55739583420047722 ) ) ;
#20597=CARTESIAN_POINT ( 'NONE',  ( -90.00000000000002842, 85.00000000000002842, -80.00000000000000000 ) ) ;
#20598=CARTESIAN_POINT ( 'NONE',  ( 96.74471819418077700, 88.31889241252949319, 74.86350982016037392 ) ) ;
#20601=CARTESIAN_POINT ( 'NONE',  ( 95.00000000000000000, -212.6630814284392557, 79.16531250086715943 ) ) ;
#20604=ORIENTED_EDGE ( 'NONE', *, *, #28534, .F. ) ;
#20607=DIRECTION ( 'NONE',  ( -1.000000000000000000, -0.000000000000000000, -0.000000000000000000 ) ) ;
#20610=CARTESIAN_POINT ( 'NONE',  ( 97.30629616937498838, -209.9999999999999716, 76.78406250086715090 ) ) ;
#20622=CARTESIAN_POINT ( 'NONE',  ( 92.35000000000002274, -211.5299782133524502, 79.97229166840095615 ) ) ;
#20623=CARTESIAN_POINT ( 'NONE',  ( 97.64999999999997726, 91.52997821335252127, 86.56041666666665435 ) ) ;
#20627=CARTESIAN_POINT ( 'NONE',  ( -97.64999999954989107, -210.0000310946949753, 88.81037122969127040 ) ) ;
#20629=CARTESIAN_POINT ( 'NONE',  ( 92.34999999999999432, 90.00000000000002842, 84.36437500173430237 ) ) ;
#20631=CARTESIAN_POINT ( 'NONE',  ( -95.00000000000002842, 87.33691857156074434, 85.51531250086715374 ) ) ;
#20633=CARTESIAN_POINT ( 'NONE',  ( 93.84685191531248449, 88.00268892867053694, 80.85864583420047325 ) ) ;
#20636=ORIENTED_EDGE ( 'NONE', *, *, #18471, .F. ) ;
#20651=CARTESIAN_POINT ( 'NONE',  ( -92.69370383062498320, -208.6684592857803011, 79.21822916753380639 ) ) ;
#20656=CARTESIAN_POINT ( 'NONE',  ( -92.35000000000003695, 90.00000000000004263, 90.00000000000000000 ) ) ;
#20658=CARTESIAN_POINT ( 'NONE',  ( 95.00000000000000000, -206.9400435732949575, 83.57062500173429953 ) ) ;
#20660=CARTESIAN_POINT ( 'NONE',  ( 97.64999999999999147, 90.00000000000002842, 77.61749999999999261 ) ) ;
#20661=CARTESIAN_POINT ( 'NONE',  ( -94.99999999999997158, -209.9999999999999716, 90.00000000000000000 ) ) ;
#20666=CARTESIAN_POINT ( 'NONE',  ( -93.67500000000003979, 87.70503267997129626, 87.75104166840095843 ) ) ;
#20673=FACE_OUTER_BOUND ( 'NONE', #4348, .T. ) ;
#20674=CARTESIAN_POINT ( 'NONE',  ( -97.64999999999996305, -209.9999999999999716, 88.09499999999999886 ) ) ;
#20677=AXIS2_PLACEMENT_3D ( 'NONE', #9643, #66430, #55510 ) ;
#20678=( BOUNDED_CURVE ( )  B_SPLINE_CURVE ( 2, ( #73104, #59346, #67485, #55084, #60744, #54720, #15974 ),
 .UNSPECIFIED., .F., .F. ) 
 B_SPLINE_CURVE_WITH_KNOTS ( ( 3, 2, 2, 3 ),
 ( 0.8890265259402125864, 0.8960822236964605114, 0.9031379892373780915, 0.9101937466136234001 ),
 .UNSPECIFIED. ) 
 CURVE ( )  GEOMETRIC_REPRESENTATION_ITEM ( )  RATIONAL_B_SPLINE_CURVE ( ( 0.9999974258394913607, 0.8660266908770580807, 1.000000000000000000, 0.8660254037844387076, 1.000000000000000000, 0.8660254037844387076, 1.000000000000000000 ) ) 
 REPRESENTATION_ITEM ( '' )  );
#20682=CARTESIAN_POINT ( 'NONE',  ( -92.35000000000003695, 90.00000000000004263, 76.34749999999999659 ) ) ;
#20689=ADVANCED_FACE ( 'NONE', ( #55873 ), #5132, .F. ) ;
#20692=CARTESIAN_POINT ( 'NONE',  ( 97.30629616937498838, -211.3315407142195852, 82.92239583420045790 ) ) ;
#20693=CARTESIAN_POINT ( 'NONE',  ( 92.69370383062501162, -209.9999999999999716, 84.08656250086716000 ) ) ;
#20695=CARTESIAN_POINT ( 'NONE',  ( 92.69370383062501162, -209.9999999999999716, 87.89656250086714806 ) ) ;
#20701=CARTESIAN_POINT ( 'NONE',  ( -93.84685191531252713, 88.00268892867056536, 77.31322916753381946 ) ) ;
#20709=CARTESIAN_POINT ( 'NONE',  ( -95.00000000000002842, 90.00000000000004263, 90.00000000000000000 ) ) ;
#20711=CARTESIAN_POINT ( 'NONE',  ( 93.67500000000001137, -212.2949673200287179, 81.29520833506762756 ) ) ;
#20713=ORIENTED_EDGE ( 'NONE', *, *, #12207, .F. ) ;
#20714=VERTEX_POINT ( 'NONE', #21267 ) ;
#20716=CARTESIAN_POINT ( 'NONE',  ( 92.69370383062501162, -209.9999999999999716, 77.57781250086713953 ) ) ;
#20717=CARTESIAN_POINT ( 'NONE',  ( 92.34999999999999432, 90.00000000000002842, 89.44437500173430067 ) ) ;
#20724=CARTESIAN_POINT ( 'NONE',  ( -92.69370383062502583, 91.33154071421968467, 78.10697916753383652 ) ) ;
#20730=CARTESIAN_POINT ( 'NONE',  ( 97.30629616937498838, 91.33154071421968467, 76.04322916753380923 ) ) ;
#20732=ORIENTED_EDGE ( 'NONE', *, *, #4015, .T. ) ;
#20738=CARTESIAN_POINT ( 'NONE',  ( -92.69370383062498320, -211.3315407142195852, 80.38239583420049428 ) ) ;
#20749=CARTESIAN_POINT ( 'NONE',  ( -92.69370383062502583, 91.33154071421968467, 86.20322916753382003 ) ) ;
#20750=LINE ( 'NONE', #60620, #17829 ) ;
#20757=FACE_OUTER_BOUND ( 'NONE', #44749, .T. ) ;
#20759=CARTESIAN_POINT ( 'NONE',  ( -92.69370383062498320, -208.6684592857803011, 83.18697916753382060 ) ) ;
#20760=CARTESIAN_POINT ( 'NONE',  ( 93.67499999999999716, 87.70503267997126784, 76.21520833506762926 ) ) ;
#20764=CARTESIAN_POINT ( 'NONE',  ( -92.34999999999999432, -209.9999999999999716, 78.88750000000000284 ) ) ;
#20766=ORIENTED_EDGE ( 'NONE', *, *, #4589, .F. ) ;
#20778=ORIENTED_EDGE ( 'NONE', *, *, #25873, .F. ) ;
#20781=CARTESIAN_POINT ( 'NONE',  ( -99.99999999999997158, -204.9999999999999716, 90.00000000000000000 ) ) ;
#20785=ADVANCED_FACE ( 'NONE', ( #28401 ), #22030, .T. ) ;
#20790=ORIENTED_EDGE ( 'NONE', *, *, #36098, .T. ) ;
#20793=ORIENTED_EDGE ( 'NONE', *, *, #40594, .F. ) ;
#20798=CARTESIAN_POINT ( 'NONE',  ( 97.30629616937498838, 90.00000000000002842, 76.14906250086716000 ) ) ;
#20805=CARTESIAN_POINT ( 'NONE',  ( 93.84685191531248449, 91.99731107132950569, 86.99697916753380866 ) ) ;
#20807=ORIENTED_EDGE ( 'NONE', *, *, #21925, .F. ) ;
#20808=CARTESIAN_POINT ( 'NONE',  ( 97.30629616937498838, -211.3315407142195852, 88.63739583420047552 ) ) ;
#20813=CARTESIAN_POINT ( 'NONE',  ( -97.64999999999996305, -209.9999999999999716, 81.74500000000000455 ) ) ;
#20814=CARTESIAN_POINT ( 'NONE',  ( -97.64999999999990621, -208.4700217866474361, 82.96208333333332519 ) ) ;
#20816=CARTESIAN_POINT ( 'NONE',  ( -92.34999999999999432, -211.5299782133524502, 75.10395833506764518 ) ) ;
#20817=CARTESIAN_POINT ( 'NONE',  ( -97.30629616937501680, 91.33154071421968467, 89.11364583420049712 ) ) ;
#20820=CARTESIAN_POINT ( 'NONE',  ( 92.69370383062498320, 90.00000000000002842, 87.10281250086714522 ) ) ;
#20821=CARTESIAN_POINT ( 'NONE',  ( -92.69370383062504004, 90.00000000000004263, 86.78531250086714977 ) ) ;
#20823=CARTESIAN_POINT ( 'NONE',  ( 97.30629616937498838, 90.00000000000002842, 74.87906250086714977 ) ) ;
#20828=ADVANCED_FACE ( 'NONE', ( #12227 ), #625, .F. ) ;
#20836=CARTESIAN_POINT ( 'NONE',  ( -95.00000000000002842, 86.94004357329504273, 81.90374999999998806 ) ) ;
#20838=CARTESIAN_POINT ( 'NONE',  ( 93.67500000000001137, -212.2949673200287179, 75.58020833506763836 ) ) ;
#20839=CARTESIAN_POINT ( 'NONE',  ( 100.0000000000000000, -214.9999999999999716, 90.00000000000000000 ) ) ;
#20842=CARTESIAN_POINT ( 'NONE',  ( -93.84685191531248449, -208.0026889286704943, 75.61989583420049144 ) ) ;
#20845=CARTESIAN_POINT ( 'NONE',  ( -92.69370383062502583, 88.66845928578038638, 81.65239583420049030 ) ) ;
#20855=CARTESIAN_POINT ( 'NONE',  ( 93.84685191531248449, 91.99731107132950569, 78.90072916753382515 ) ) ;
#20857=CARTESIAN_POINT ( 'NONE',  ( -96.15314808468745866, -211.9973110713294489, 84.82739583420048746 ) ) ;
#20861=CARTESIAN_POINT ( 'NONE',  ( -92.34999999999999432, -211.5299782133524502, 76.29458333333333542 ) ) ;
#20864=EDGE_CURVE ( 'NONE', #74311, #73251, #22001, .T. ) ;
#20865=EDGE_CURVE ( 'NONE', #52132, #48511, #65273, .T. ) ;
#20867=CARTESIAN_POINT ( 'NONE',  ( 92.69370383062501162, -211.3315407142195852, 83.34572916753380412 ) ) ;
#20878=CARTESIAN_POINT ( 'NONE',  ( 93.84685191531249870, -208.0026889286704943, 76.99572916753382401 ) ) ;
#20882=( BOUNDED_CURVE ( )  B_SPLINE_CURVE ( 2, ( #50597, #61522, #10006, #45732, #22032, #32925, #55875 ),
 .UNSPECIFIED., .F., .F. ) 
 B_SPLINE_CURVE_WITH_KNOTS ( ( 3, 2, 2, 3 ),
 ( 0.1250000000000002220, 0.1319444444444446418, 0.1388888888888890338, 0.1458333333333334536 ),
 .UNSPECIFIED. ) 
 CURVE ( )  GEOMETRIC_REPRESENTATION_ITEM ( )  RATIONAL_B_SPLINE_CURVE ( ( 0.9999999999999956701, 0.8660254037844430375, 1.000000000000000000, 0.8660254037844387076, 1.000000000000000000, 0.8660254037844365982, 1.000000000000002220 ) ) 
 REPRESENTATION_ITEM ( '' )  );
#20883=CARTESIAN_POINT ( 'NONE',  ( 95.00000000000000000, -213.0599564267049857, 83.80875000000000341 ) ) ;
#20884=CARTESIAN_POINT ( 'NONE',  ( 97.30629616937498838, 90.00000000000002842, 85.67406250086715147 ) ) ;
#20886=CARTESIAN_POINT ( 'NONE',  ( 97.65000000000000568, 88.47002178664752137, 75.10395833506764518 ) ) ;
#20887=CARTESIAN_POINT ( 'NONE',  ( 92.35000000000002274, -211.5299782133524502, 81.79791666666666572 ) ) ;
#20893=CARTESIAN_POINT ( 'NONE',  ( 95.00000000000000000, -206.9400435732949575, 89.20624999999999716 ) ) ;
#20898=CARTESIAN_POINT ( 'NONE',  ( -92.69370383062502583, 91.33154071421968467, 85.72697916753381264 ) ) ;
#20899=CARTESIAN_POINT ( 'NONE',  ( 2.499999999999982681, -79.99999999999998579, -310.0000000000000000 ) ) ;
#20901=CARTESIAN_POINT ( 'NONE',  ( -94.99999999999997158, -213.0599564267049857, 88.33312500173431658 ) ) ;
#20903=EDGE_LOOP ( 'NONE', ( #58911, #46520, #34391, #53379 ) ) ;
#20904=CARTESIAN_POINT ( 'NONE',  ( -97.64999999999996305, -209.9999999999999716, 87.53937500173429953 ) ) ;
#20909=CARTESIAN_POINT ( 'NONE',  ( -97.65000000000001990, 88.47002178664754979, 83.14729166840096752 ) ) ;
#20911=CARTESIAN_POINT ( 'NONE',  ( 94.99999999999998579, 92.66308142843935514, 85.83281250086714920 ) ) ;
#20916=CARTESIAN_POINT ( 'NONE',  ( -100.0000000000000142, 95.00000000000002842, -90.00000000000000000 ) ) ;
#20920=LINE ( 'NONE', #72048, #49138 ) ;
#20927=CARTESIAN_POINT ( 'NONE',  ( -96.15314808468745866, -211.9973110713294489, 86.09739583420049769 ) ) ;
#20931=DIRECTION ( 'NONE',  ( -0.000000000000000000, -0.000000000000000000, 1.000000000000000000 ) ) ;
#20934=CARTESIAN_POINT ( 'NONE',  ( 97.64999999999999147, -210.0000058630886031, 82.77687479895030265 ) ) ;
#20935=CARTESIAN_POINT ( 'NONE',  ( 92.69370383062498320, 90.00000000000002842, 76.94281250086713442 ) ) ;
#20941=CARTESIAN_POINT ( 'NONE',  ( -94.99999999999997158, -213.0599564267049857, 86.98374999999998636 ) ) ;
#20943=CARTESIAN_POINT ( 'NONE',  ( -92.93550210798944988, -208.9360650323627624, 74.79348190356850523 ) ) ;
#20947=CARTESIAN_POINT ( 'NONE',  ( -95.00000000000002842, 87.33691857156074434, 82.18156250086715886 ) ) ;
#20951=EDGE_CURVE ( 'NONE', #70455, #35173, #70958, .T. ) ;
#20955=EDGE_CURVE ( 'NONE', #6931, #21000, #19711, .T. ) ;
#20956=DIRECTION ( 'NONE',  ( 1.000000000000000000, 0.000000000000000000, 0.000000000000000000 ) ) ;
#20962=CARTESIAN_POINT ( 'NONE',  ( 97.30629616937498838, -209.9999999999999716, 78.68906250086715204 ) ) ;
#20964=ORIENTED_EDGE ( 'NONE', *, *, #21115, .T. ) ;
#20972=CARTESIAN_POINT ( 'NONE',  ( 92.69370383062501162, -211.3315407142195852, 75.88447916753382572 ) ) ;
#20974=CARTESIAN_POINT ( 'NONE',  ( -93.67499999999998295, -207.7050326799711968, 87.88333333333332575 ) ) ;
#20984=CARTESIAN_POINT ( 'NONE',  ( 96.32499999999998863, -207.7050326799711968, 80.34270833506762699 ) ) ;
#20985=CARTESIAN_POINT ( 'NONE',  ( 92.34999999999999432, 90.00000000000002842, 86.18999999999999773 ) ) ;
#20988=CARTESIAN_POINT ( 'NONE',  ( -92.98549755320793508, -211.1324117838502161, 74.79348190356850523 ) ) ;
#20989=ORIENTED_EDGE ( 'NONE', *, *, #15039, .F. ) ;
#20991=CARTESIAN_POINT ( 'NONE',  ( -93.84685191531254134, 91.99731107132950569, 85.14489583420048291 ) ) ;
#20993=CARTESIAN_POINT ( 'NONE',  ( 93.84685191531248449, 88.00268892867053694, 83.39864583420047950 ) ) ;
#21000=VERTEX_POINT ( 'NONE', #59581 ) ;
#21003=CARTESIAN_POINT ( 'NONE',  ( 93.67499999999998295, 92.29496732002878900, 79.09916666666666174 ) ) ;
#21004=ORIENTED_EDGE ( 'NONE', *, *, #34235, .F. ) ;
#21006=CARTESIAN_POINT ( 'NONE',  ( 96.32499999999998863, 87.70503267997126784, 88.38604166840097776 ) ) ;
#21009=CARTESIAN_POINT ( 'NONE',  ( -93.84685191531248449, -208.0026889286704943, 78.00114583420048575 ) ) ;
#21013=CARTESIAN_POINT ( 'NONE',  ( -93.67499999999998295, -207.7050326799711968, 89.23270833506762756 ) ) ;
#21017=CARTESIAN_POINT ( 'NONE',  ( 96.15314808468748708, 88.00268892867053694, 86.67947916753381321 ) ) ;
#21021=( BOUNDED_CURVE ( )  B_SPLINE_CURVE ( 2, ( #22716, #17068, #55804, #5063, #16320, #67452, #27962 ),
 .UNSPECIFIED., .F., .F. ) 
 B_SPLINE_CURVE_WITH_KNOTS ( ( 3, 2, 2, 3 ),
 ( 0.6666666666666667407, 0.6736111111111112715, 0.6805555555555555802, 0.6875000000000000000 ),
 .UNSPECIFIED. ) 
 CURVE ( )  GEOMETRIC_REPRESENTATION_ITEM ( )  RATIONAL_B_SPLINE_CURVE ( ( 0.9999999999999978906, 0.8660254037844408170, 1.000000000000000000, 0.8660254037844387076, 1.000000000000000000, 0.8660254037844387076, 1.000000000000000000 ) ) 
 REPRESENTATION_ITEM ( '' )  );
#21022=CARTESIAN_POINT ( 'NONE',  ( -97.65000000000001990, 90.00000000000004263, 88.80937500173430976 ) ) ;
#21026=CARTESIAN_POINT ( 'NONE',  ( 94.99999999999998579, 86.94004357329502852, 77.45874999999999488 ) ) ;
#21028=CARTESIAN_POINT ( 'NONE',  ( 96.32499999999998863, -207.7050326799711968, 75.18333333333332291 ) ) ;
#21031=CARTESIAN_POINT ( 'NONE',  ( 94.99999999999998579, 90.00000000000002842, 90.00000000000000000 ) ) ;
#21034=EDGE_CURVE ( 'NONE', #21161, #30764, #27253, .T. ) ;
#21035=CARTESIAN_POINT ( 'NONE',  ( -94.99999999999997158, -213.0599564267049857, 84.44375000000000853 ) ) ;
#21036=DIRECTION ( 'NONE',  ( -0.000000000000000000, -0.000000000000000000, 1.000000000000000000 ) ) ;
#21041=CARTESIAN_POINT ( 'NONE',  ( -100.0000000000000142, 95.00000000000002842, 90.00000000000000000 ) ) ;
#21044=EDGE_LOOP ( 'NONE', ( #6442, #33576, #55751, #47285 ) ) ;
#21051=ORIENTED_EDGE ( 'NONE', *, *, #43208, .T. ) ;
#21053=CARTESIAN_POINT ( 'NONE',  ( 96.15314808468750130, -211.9973110713294489, 82.23447916753380582 ) ) ;
#21054=CARTESIAN_POINT ( 'NONE',  ( 95.00000000000000000, -207.3369185715606307, 85.19781250086714408 ) ) ;
#21055=EDGE_LOOP ( 'NONE', ( #13443, #10931, #9721, #63458 ) ) ;
#21057=CARTESIAN_POINT ( 'NONE',  ( 95.00000000000000000, -212.6630814284392557, 84.88031250086714863 ) ) ;
#21061=CARTESIAN_POINT ( 'NONE',  ( -97.30629616937501680, 90.00000000000004263, 76.46656250086715545 ) ) ;
#21072=EDGE_LOOP ( 'NONE', ( #18748, #51518, #15989, #51428 ) ) ;
#21075=CARTESIAN_POINT ( 'NONE',  ( 93.84685191531251292, -211.9973110713294489, 75.14364583420046984 ) ) ;
#21076=DIRECTION ( 'NONE',  ( -3.061616997868382648E-16, -1.000000000000000000, 0.000000000000000000 ) ) ;
#21082=CARTESIAN_POINT ( 'NONE',  ( -95.00000000000002842, 93.05995642670501411, 89.84125000000000227 ) ) ;
#21085=CARTESIAN_POINT ( 'NONE',  ( 97.30629616937498838, 90.00000000000002842, 77.26031250086714408 ) ) ;
#21088=CARTESIAN_POINT ( 'NONE',  ( -97.30629616937497417, -211.3315407142195852, 89.06072916753379332 ) ) ;
#21093=CARTESIAN_POINT ( 'NONE',  ( -96.15314808468745866, -211.9973110713294489, 79.58864583420047722 ) ) ;
#21106=CARTESIAN_POINT ( 'NONE',  ( 97.65000000000000568, 88.47002178664752137, 80.18395833506764347 ) ) ;
#21107=CARTESIAN_POINT ( 'NONE',  ( -92.69370383062502583, 91.33154071421968467, 83.02822916753379445 ) ) ;
#21112=( BOUNDED_CURVE ( )  B_SPLINE_CURVE ( 2, ( #38256, #1594, #61199, #19204, #53059, #9686, #66470, #32609, #60466 ),
 .UNSPECIFIED., .F., .F. ) 
 B_SPLINE_CURVE_WITH_KNOTS ( ( 3, 2, 2, 2, 3 ),
 ( 0.4021785743327794815, 0.4021786358302962827, 0.4092344013711782802, 0.4162901669120601666, 0.4233457466685775494 ),
 .UNSPECIFIED. ) 
 CURVE ( )  GEOMETRIC_REPRESENTATION_ITEM ( )  RATIONAL_B_SPLINE_CURVE ( ( 0.9999976645955351851, 0.9999988322875899005, 1.000000000000000000, 0.8660254037844387076, 1.000000000000000000, 0.8660254037844387076, 1.000000000000000000, 0.8660289314505841274, 0.9999929448534821130 ) ) 
 REPRESENTATION_ITEM ( '' )  );
#21115=EDGE_CURVE ( 'NONE', #45794, #52450, #68115, .T. ) ;
#21116=EDGE_CURVE ( 'NONE', #2269, #39726, #16304, .T. ) ;
#21121=CARTESIAN_POINT ( 'NONE',  ( 96.32499999999998863, -207.7050326799711968, 88.59770833506763665 ) ) ;
#21122=CARTESIAN_POINT ( 'NONE',  ( -92.69370383062498320, -208.6684592857803011, 81.91697916753381037 ) ) ;
#21128=DIRECTION ( 'NONE',  ( 0.000000000000000000, 1.000000000000000000, 0.000000000000000000 ) ) ;
#21136=EDGE_CURVE ( 'NONE', #21245, #6700, #32530, .T. ) ;
#21156=AXIS2_PLACEMENT_3D ( 'NONE', #95, #34246, #56068 ) ;
#21158=CARTESIAN_POINT ( 'NONE',  ( 93.84685191531248449, 91.99731107132950569, 76.99572916753382401 ) ) ;
#21161=VERTEX_POINT ( 'NONE', #41730 ) ;
#21163=ORIENTED_EDGE ( 'NONE', *, *, #8942, .T. ) ;
#21164=CARTESIAN_POINT ( 'NONE',  ( 92.69370383062498320, 91.33154071421968467, 87.68489583420047495 ) ) ;
#21166=CARTESIAN_POINT ( 'NONE',  ( 97.30629616937498838, -211.3315407142195852, 84.82739583420045903 ) ) ;
#21172=CARTESIAN_POINT ( 'NONE',  ( -97.30629616937495996, -209.9999999999999716, 88.37281250086715545 ) ) ;
#21173=CARTESIAN_POINT ( 'NONE',  ( -93.84685191531252713, 88.00268892867056536, 88.74322916753382628 ) ) ;
#21175=CARTESIAN_POINT ( 'NONE',  ( 97.30629616937498838, 88.66845928578037217, 88.00239583420047040 ) ) ;
#21176=CARTESIAN_POINT ( 'NONE',  ( -97.30629616937501680, 88.66845928578038638, 89.06072916753379332 ) ) ;
#21178=CARTESIAN_POINT ( 'NONE',  ( 92.35000000019411459, -210.0000198431783929, 84.36502760998391182 ) ) ;
#21182=CARTESIAN_POINT ( 'NONE',  ( -94.99999999999997158, -207.3369185715606307, 88.84906250086713442 ) ) ;
#21183=CARTESIAN_POINT ( 'NONE',  ( -95.00000000000002842, 93.05995642670504253, 89.20624999999999716 ) ) ;
#21190=CARTESIAN_POINT ( 'NONE',  ( -92.35000000000005116, 88.47002178664754979, 82.00958333333332462 ) ) ;
#21192=DIRECTION ( 'NONE',  ( 1.000000000000000000, 0.000000000000000000, 0.000000000000000000 ) ) ;
#21200=CARTESIAN_POINT ( 'NONE',  ( -92.69370383062502583, 91.33154071421968467, 81.12322916753382174 ) ) ;
#21206=FACE_OUTER_BOUND ( 'NONE', #9045, .T. ) ;
#21208=CARTESIAN_POINT ( 'NONE',  ( -96.32499999999996021, -207.7050326799711968, 87.35416666666665719 ) ) ;
#21215=CARTESIAN_POINT ( 'NONE',  ( 93.84685191531248449, 91.99731107132950569, 79.53572916753381605 ) ) ;
#21216=CARTESIAN_POINT ( 'NONE',  ( -97.30629616937495996, -209.9999999999999716, 82.81656250086714977 ) ) ;
#21220=CARTESIAN_POINT ( 'NONE',  ( -92.34999999999999432, -211.5299782133524502, 79.46958333333333258 ) ) ;
#21221=CARTESIAN_POINT ( 'NONE',  ( 92.34999999999995168, -208.4700217866474929, 78.51708333333334622 ) ) ;
#21224=CARTESIAN_POINT ( 'NONE',  ( -92.69370383062505425, 88.66845928578038638, 79.27114583420048177 ) ) ;
#21225=CARTESIAN_POINT ( 'NONE',  ( 96.15314808468748708, -208.0026889286704943, 84.98614583420047097 ) ) ;
#21233=DIRECTION ( 'NONE',  ( -0.000000000000000000, -0.000000000000000000, 1.000000000000000000 ) ) ;
#21240=CARTESIAN_POINT ( 'NONE',  ( 92.69370383062498320, 91.33154071421968467, 87.20864583420049598 ) ) ;
#21242=CARTESIAN_POINT ( 'NONE',  ( 93.67499999999999716, 87.70503267997126784, 80.66020833506763665 ) ) ;
#21243=CARTESIAN_POINT ( 'NONE',  ( 93.67500000000001137, -207.7050326799711968, 77.19416666666666060 ) ) ;
#21245=VERTEX_POINT ( 'NONE', #25189 ) ;
#21252=DIRECTION ( 'NONE',  ( -0.000000000000000000, -0.000000000000000000, 1.000000000000000000 ) ) ;
#21253=CARTESIAN_POINT ( 'NONE',  ( -96.32499999999996021, -212.2949673200287179, 88.28020833506764120 ) ) ;
#21256=CARTESIAN_POINT ( 'NONE',  ( -97.64999999999994884, -208.4700217866474645, 86.21645833506764234 ) ) ;
#21261=CARTESIAN_POINT ( 'NONE',  ( -95.00000000000002842, 86.94004357329504273, 84.52312500173428589 ) ) ;
#21263=CARTESIAN_POINT ( 'NONE',  ( 94.99999999999998579, 92.66308142843935514, 82.02281250086714692 ) ) ;
#21266=EDGE_CURVE ( 'NONE', #50963, #57918, #43462, .T. ) ;
#21267=CARTESIAN_POINT ( 'NONE',  ( -89.99999999999998579, -204.9999999999999716, -80.00000000000000000 ) ) ;
#21282=DIRECTION ( 'NONE',  ( 1.000000000000000000, 0.000000000000000000, 0.000000000000000000 ) ) ;
#21284=CARTESIAN_POINT ( 'NONE',  ( -93.84685191531248449, -208.0026889286704943, 83.23989583420049598 ) ) ;
#21286=DIRECTION ( 'NONE',  ( -0.000000000000000000, -0.000000000000000000, 1.000000000000000000 ) ) ;
#21291=CARTESIAN_POINT ( 'NONE',  ( 92.35000000000000853, -209.9999999999999716, 83.09437500173430635 ) ) ;
#21292=CARTESIAN_POINT ( 'NONE',  ( 94.99999999999998579, 87.33691857156068750, 79.64156250086713840 ) ) ;
#21296=CARTESIAN_POINT ( 'NONE',  ( 94.32747394040349320, 92.31128197830615534, 74.85222950654856788 ) ) ;
#21303=ORIENTED_EDGE ( 'NONE', *, *, #54341, .F. ) ;
#21304=CARTESIAN_POINT ( 'NONE',  ( -97.30629616937501680, 88.66845928578038638, 82.71072916753378479 ) ) ;
#21308=VECTOR ( 'NONE', #8079, 1000.000000000000000 ) ;
#21313=( BOUNDED_CURVE ( )  B_SPLINE_CURVE ( 2, ( #31401, #21221, #38156, #43458, #38536, #61474, #27230 ),
 .UNSPECIFIED., .F., .F. ) 
 B_SPLINE_CURVE_WITH_KNOTS ( ( 3, 2, 2, 3 ),
 ( 0.7499999999999996669, 0.7569444444444439757, 0.7638888888888883955, 0.7708333333333328152 ),
 .UNSPECIFIED. ) 
 CURVE ( )  GEOMETRIC_REPRESENTATION_ITEM ( )  RATIONAL_B_SPLINE_CURVE ( ( 1.000000000000006439, 0.8660254037844322683, 1.000000000000000000, 0.8660254037844387076, 1.000000000000000000, 0.8660254037844493658, 0.9999999999999893419 ) ) 
 REPRESENTATION_ITEM ( '' )  );
#21314=CARTESIAN_POINT ( 'NONE',  ( 94.99999999999998579, 90.00000000000002842, 90.00000000000000000 ) ) ;
#21317=CYLINDRICAL_SURFACE ( 'NONE', #52341, 2.649999999999985700 ) ;
#21318=CARTESIAN_POINT ( 'NONE',  ( 93.84685191531249870, -208.0026889286704943, 80.17072916753382117 ) ) ;
#21320=VECTOR ( 'NONE', #33332, 1000.000000000000000 ) ;
#21322=VERTEX_POINT ( 'NONE', #55977 ) ;
#21330=CARTESIAN_POINT ( 'NONE',  ( 93.84685191531251292, -211.9973110713294489, 76.57239583420049200 ) ) ;
#21336=CARTESIAN_POINT ( 'NONE',  ( -97.65000000000001990, 91.52997821335253548, 89.39145833506763950 ) ) ;
#21339=CARTESIAN_POINT ( 'NONE',  ( 95.00000000000000000, -206.9400435732949575, 79.76062500173429726 ) ) ;
#21340=CARTESIAN_POINT ( 'NONE',  ( 96.32499999999998863, 87.70503267997126784, 82.59166666666665435 ) ) ;
#21341=ORIENTED_EDGE ( 'NONE', *, *, #69362, .F. ) ;
#21343=ORIENTED_EDGE ( 'NONE', *, *, #20102, .F. ) ;
#21344=CARTESIAN_POINT ( 'NONE',  ( -97.64996030324587650, -211.5300011322840987, 88.86229325377448163 ) ) ;
#21347=CARTESIAN_POINT ( 'NONE',  ( -92.69370383062505425, 91.33154071421968467, 85.72697916753381264 ) ) ;
#21349=CARTESIAN_POINT ( 'NONE',  ( 93.84685191531248449, 91.99731107132950569, 78.10697916753380809 ) ) ;
#21356=CARTESIAN_POINT ( 'NONE',  ( -97.30629616937497417, -211.3315407142195852, 79.53572916753380184 ) ) ;
#21367=CARTESIAN_POINT ( 'NONE',  ( 96.32499999999997442, 92.29496732002878900, 89.23270833506762756 ) ) ;
#21369=CARTESIAN_POINT ( 'NONE',  ( -94.99999999999997158, -212.6630814284392557, 78.37156250086714238 ) ) ;
#21371=CARTESIAN_POINT ( 'NONE',  ( 92.34999999999999432, 90.00000000000002842, 88.80937500173430976 ) ) ;
#21372=FACE_OUTER_BOUND ( 'NONE', #47191, .T. ) ;
#21373=DIRECTION ( 'NONE',  ( -0.000000000000000000, -0.000000000000000000, 1.000000000000000000 ) ) ;
#21378=CARTESIAN_POINT ( 'NONE',  ( 92.69370383062498320, 90.00000000000002842, 88.37281250086715545 ) ) ;
#21381=CARTESIAN_POINT ( 'NONE',  ( 92.35000000052950497, 90.00003365185392568, 81.18829462297337329 ) ) ;
#21382=AXIS2_PLACEMENT_3D ( 'NONE', #21990, #44937, #39292 ) ;
#21383=CARTESIAN_POINT ( 'NONE',  ( -97.65000000000001990, 90.00000000000004263, 86.82500000000000284 ) ) ;
#21387=EDGE_CURVE ( 'NONE', #48269, #31307, #72909, .T. ) ;
#21394=ADVANCED_FACE ( 'NONE', ( #9743 ), #26283, .F. ) ;
#21396=LINE ( 'NONE', #26673, #10692 ) ;
#21397=CARTESIAN_POINT ( 'NONE',  ( -92.34999999999999432, -211.5299782133524502, 85.81958333333331268 ) ) ;
#21398=DIRECTION ( 'NONE',  ( -0.000000000000000000, -0.000000000000000000, 1.000000000000000000 ) ) ;
#21401=CARTESIAN_POINT ( 'NONE',  ( -2.499999999999970690, 73.00000000000001421, -204.9999999999999716 ) ) ;
#21406=CARTESIAN_POINT ( 'NONE',  ( 92.69370383062501162, -211.3315407142195852, 89.21947916753381946 ) ) ;
#21407=CIRCLE ( 'NONE', #49066, 3.299999999999983391 ) ;
#21413=ORIENTED_EDGE ( 'NONE', *, *, #24894, .F. ) ;
#21414=CARTESIAN_POINT ( 'NONE',  ( 96.15314808468750130, -211.9973110713294489, 79.05947916753380866 ) ) ;
#21415=CARTESIAN_POINT ( 'NONE',  ( 97.30629616937498838, -211.3315407142195852, 86.25614583420048120 ) ) ;
#21417=B_SPLINE_CURVE_WITH_KNOTS ( 'NONE', 3,
 ( #59702, #8182, #20943, #43898, #31849, #66816 ),
 .UNSPECIFIED., .F., .F.,
 ( 4, 2, 4 ),
 ( 0.000000000000000000, 0.0008269033587275169102, 0.001653806717455033820 ),
 .UNSPECIFIED. ) ;
#21418=CARTESIAN_POINT ( 'NONE',  ( 92.69370383062501162, -211.3315407142195852, 87.94947916753382344 ) ) ;
#21422=ORIENTED_EDGE ( 'NONE', *, *, #19082, .F. ) ;
#21430=CARTESIAN_POINT ( 'NONE',  ( 96.32499999999998863, -212.2949673200287179, 89.02104166840096866 ) ) ;
#21440=CARTESIAN_POINT ( 'NONE',  ( 92.69370383062501162, -208.6684592857803011, 76.25489583420049655 ) ) ;
#21448=( BOUNDED_CURVE ( )  B_SPLINE_CURVE ( 2, ( #28438, #69050, #35194, #22068, #5168, #28067, #45011, #67938, #16427, #73932, #34084, #57029, #51010, #22443, #45387, #16804, #62690, #11161, #5540, #51371, #22822, #74308, #45760, #11517, #68685, #17170, #40104, #63058, #34450, #42327, #18633, #41572, #65260, #69772, #35562, #53974, #64513, #29539, #31022, #7369, #25018, #47222, #19741, #41211, #29911, #47959, #70877, #52477, #2134, #13733, #12991, #58492, #19376, #1767, #24654, #24295, #71236, #36670, #59616, #8099, #47585, #35928, #25400, #2518, #48327, #42690, #65628, #1402, #14099, #37049, #1028, #58877, #52863, #46861, #6628, #59242, #30287, #70489, #53231, #23919, #18274, #41954, #19002, #70132, #64149, #12624, #64892, #6988, #13366, #36299, #53595, #7734, #30649, #60363, #20857, #31393, #60730, #59995, #21594, #44549, #20500, #8480, #44170, #43073, #25762, #32127, #71985, #67468, #38531, #27224, #66005, #73092, #49431, #55818, #67093, #15960, #43451, #72710, #9208, #54345, #14851, #49060, #9586, #26125, #32506, #31762, #4331, #72360, #2869, #50158, #61467, #37798, #21216, #48691, #55072, #61090, #43813, #66371, #55446, #3603, #3965, #26864, #26503, #66731, #8848, #15594, #15220, #71615, #20112, #38151, #49790, #14479, #9947, #32869, #37431, #54705, #3234, #27612, #29083, #27976, #50914, #16334, #50541, #68216, #34740, #73836, #63325, #5814, #51659, #46390, #62592, #11071, #45670, #51281, #69317, #33994, #34361, #57682, #38900, #67842, #22348, #68595, #68960, #39276, #73464, #10320, #17082, #11787, #10693, #33237, #21973, #39647, #56577, #74215, #40017, #61837, #45297, #22732, #62206, #28721, #33620, #16711, #6185, #207, #23099, #52019, #568, #56189, #4710, #44922, #23461, #5076, #56941, #5449, #28345, #62971, #11427, #57304, #46030, #17445, #40374, #59526, #69688, #17809, #30564, #8012, #36578, #36211, #1679, #64802, #47862, #63697, #12538, #29819, #7644, #24930, #47500, #40758, #18910, #64426, #65171, #30929, #35473, #41855, #70785, #47137, #53509, #59153, #52774, #24568, #13279, #70401, #42240, #19289, #2044, #23828, #53877, #2423, #18185, #13645, #58404, #46769, #29446, #12170, #25312, #48242, #64063, #35108, #6544, #18549, #6904, #30199, #58038, #52389, #1317, #937, #41129, #24210, #70045, #41484, #12902, #35835, #58784, #7281, #53139, #20407, #27132 ),
 .UNSPECIFIED., .F., .F. ) 
 B_SPLINE_CURVE_WITH_KNOTS ( ( 3, 2, 2, 2, 2, 2, 2, 2, 2, 2, 2, 2, 2, 2, 2, 2, 2, 2, 2, 2, 2, 2, 2, 2, 2, 2, 2, 2, 2, 2, 2, 2, 2, 2, 2, 2, 2, 2, 2, 2, 2, 2, 2, 2, 2, 2, 2, 2, 2, 2, 2, 2, 2, 2, 2, 2, 2, 2, 2, 2, 2, 2, 2, 2, 2, 2, 2, 2, 2, 2, 2, 2, 2, 2, 2, 2, 2, 2, 2, 2, 2, 2, 2, 2, 2, 2, 2, 2, 2, 2, 2, 2, 2, 2, 2, 2, 2, 2, 2, 2, 2, 2, 2, 2, 2, 2, 2, 2, 2, 2, 2, 2, 2, 2, 2, 2, 2, 2, 2, 2, 2, 2, 2, 2, 2, 2, 2, 2, 2, 2, 2, 2, 2, 2, 2, 2, 2, 2, 2, 2, 2, 2, 2, 3 ),
 ( 0.000000000000000000, 0.007055764916269566256, 0.01411152983253913251, 0.02116729474880869877, 0.02822305966507826502, 0.03527882458134783822, 0.04233458949761739754, 0.04939035441388697073, 0.05644611933015653005, 0.06350188424642609630, 0.07055764916269567644, 0.07761341407896524269, 0.08466917899523479507, 0.09172494391150436133, 0.09878070882777394146, 0.1058364737440435077, 0.1128922386603130601, 0.1199480035765826264, 0.1270037684928521926, 0.1340595334091217727, 0.1411152983253913529, 0.1481710632416609053, 0.1552268281579304854, 0.1622825930742000100, 0.1693383579904695901, 0.1763941229067391703, 0.1834498878230087227, 0.1905056527392783028, 0.1975614176555478829, 0.2046171825718174353, 0.2116729474880870154, 0.2187287124043565678, 0.2257844773206261202, 0.2328402422368957003, 0.2398960071531652527, 0.2469517720694348328, 0.2540075369857043852, 0.2610633019019739653, 0.2681190668182435455, 0.2751748317345130701, 0.2822305966507827057, 0.2892863615670522304, 0.2963421264833218105, 0.3033978913995913906, 0.3104536563158609708, 0.3175094212321304954, 0.3245651861484000200, 0.3316209510646696557, 0.3386767159809391803, 0.3457324808972087604, 0.3527882458134783406, 0.3598440107297479207, 0.3668997756460174453, 0.3739555405622870810, 0.3810113054785566056, 0.3880670703948261302, 0.3951228353110957658, 0.4021786002273652905, 0.4092343651436348706, 0.4162901300599044507, 0.4233458949761740309, 0.4304016598924435555, 0.4374574248087131356, 0.4445131897249827158, 0.4515689546412522404, 0.4586247195575218205, 0.4656804844737914006, 0.4727362493900609808, 0.4797920143063305054, 0.4868477792226001410, 0.4939035441388696657, 0.5009593090551393013, 0.5080150739714087704, 0.5150708388876783506, 0.5221266038039479307, 0.5291823687202175108, 0.5362381336364870910, 0.5432938985527566711, 0.5503496634690261402, 0.5574054283852958314, 0.5644611933015654115, 0.5715169582178348806, 0.5785727231341044607, 0.5856284880503740409, 0.5926842529666436210, 0.5997400178829132011, 0.6067957827991827813, 0.6138515477154522504, 0.6209073126317219415, 0.6279630775479914107, 0.6350188424642609908, 0.6420746073805305709, 0.6491303722968000400, 0.6561861372130697312, 0.6632419021293393113, 0.6702976670456087804, 0.6773534319618783606, 0.6844091968781480517, 0.6914649617944175208, 0.6985207267106871010, 0.7055764916269566811, 0.7126322565432261502, 0.7196880214594958414, 0.7267437863757654215, 0.7337995512920348906, 0.7408553162083044707, 0.7479110811245741619, 0.7549668460408436310, 0.7620226109571132111, 0.7690783758733827913, 0.7761341407896522604, 0.7831899057059219516, 0.7902456706221915317, 0.7973014355384610008, 0.8043572004547305809, 0.8114129653710002721, 0.8184687302872697412, 0.8255244952035393213, 0.8325802601198089015, 0.8396360250360783706, 0.8466917899523480617, 0.8537475548686176419, 0.8608033197848871110, 0.8678590847011566911, 0.8749148496174262712, 0.8819706145336958514, 0.8890263794499654315, 0.8960821443662349006, 0.9031379092825044808, 0.9101936741987741719, 0.9172494391150436410, 0.9243052040313132212, 0.9313609689475828013, 0.9384167338638523814, 0.9454724987801219616, 0.9525282636963915417, 0.9595840286126610108, 0.9666397935289305909, 0.9736955584452002821, 0.9807513233614697512, 0.9878070882777393313, 0.9948628531940089115, 0.9999999123559573100, 1.000000000000000000 ),
 .UNSPECIFIED. ) 
 CURVE ( )  GEOMETRIC_REPRESENTATION_ITEM ( )  RATIONAL_B_SPLINE_CURVE ( ( 1.000000000000000000, 0.8660254037844387076, 1.000000000000000000, 0.8660254037844387076, 1.000000000000000000, 0.8660254037844387076, 1.000000000000000000, 0.8660254037844387076, 1.000000000000000000, 0.8660254037844387076, 1.000000000000000000, 0.8660254037844387076, 1.000000000000000000, 0.8660254037844387076, 1.000000000000000000, 0.8660254037844387076, 1.000000000000000000, 0.8660254037844387076, 1.000000000000000000, 0.8660254037844387076, 1.000000000000000000, 0.8660254037844387076, 1.000000000000000000, 0.8660254037844387076, 1.000000000000000000, 0.8660254037844387076, 1.000000000000000000, 0.8660254037844387076, 1.000000000000000000, 0.8660254037844387076, 1.000000000000000000, 0.8660254037844387076, 1.000000000000000000, 0.8660254037844387076, 1.000000000000000000, 0.8660254037844387076, 1.000000000000000000, 0.8660254037844387076, 1.000000000000000000, 0.8660254037844387076, 1.000000000000000000, 0.8660254037844387076, 1.000000000000000000, 0.8660254037844387076, 1.000000000000000000, 0.8660254037844387076, 1.000000000000000000, 0.8660254037844387076, 1.000000000000000000, 0.8660254037844387076, 1.000000000000000000, 0.8660254037844387076, 1.000000000000000000, 0.8660254037844387076, 1.000000000000000000, 0.8660254037844387076, 1.000000000000000000, 0.8660254037844387076, 1.000000000000000000, 0.8660254037844387076, 1.000000000000000000, 0.8660254037844387076, 1.000000000000000000, 0.8660254037844387076, 1.000000000000000000, 0.8660254037844387076, 1.000000000000000000, 0.8660254037844387076, 1.000000000000000000, 0.8660254037844387076, 1.000000000000000000, 0.8660254037844387076, 1.000000000000000000, 0.8660254037844387076, 1.000000000000000000, 0.8660254037844387076, 1.000000000000000000, 0.8660254037844387076, 1.000000000000000000, 0.8660254037844387076, 1.000000000000000000, 0.8660254037844387076, 1.000000000000000000, 0.8660254037844387076, 1.000000000000000000, 0.8660254037844387076, 1.000000000000000000, 0.8660254037844387076, 1.000000000000000000, 0.8660254037844387076, 1.000000000000000000, 0.8660254037844387076, 1.000000000000000000, 0.8660254037844387076, 1.000000000000000000, 0.8660254037844387076, 1.000000000000000000, 0.8660254037844387076, 1.000000000000000000, 0.8660254037844387076, 1.000000000000000000, 0.8660254037844387076, 1.000000000000000000, 0.8660254037844387076, 1.000000000000000000, 0.8660254037844387076, 1.000000000000000000, 0.8660254037844387076, 1.000000000000000000, 0.8660254037844387076, 1.000000000000000000, 0.8660254037844387076, 1.000000000000000000, 0.8660254037844387076, 1.000000000000000000, 0.8660254037844387076, 1.000000000000000000, 0.8660254037844387076, 1.000000000000000000, 0.8660254037844387076, 1.000000000000000000, 0.8660254037844387076, 1.000000000000000000, 0.8660254037844387076, 1.000000000000000000, 0.8660254037844387076, 1.000000000000000000, 0.8660254037844387076, 1.000000000000000000, 0.8660254037844387076, 1.000000000000000000, 0.8660254037844387076, 1.000000000000000000, 0.8660254037844387076, 1.000000000000000000, 0.8660254037844387076, 1.000000000000000000, 0.8660254037844387076, 1.000000000000000000, 0.8660254037844387076, 1.000000000000000000, 0.8660254037844387076, 1.000000000000000000, 0.8660254037844387076, 1.000000000000000000, 0.8660254037844387076, 1.000000000000000000, 0.8660254037844387076, 1.000000000000000000, 0.8660254037844387076, 1.000000000000000000, 0.8660254037844387076, 1.000000000000000000, 0.8660254037844387076, 1.000000000000000000, 0.8660254037844387076, 1.000000000000000000, 0.8660254037844387076, 1.000000000000000000, 0.8660254037844387076, 1.000000000000000000, 0.8660254037844387076, 1.000000000000000000, 0.8660254037844387076, 1.000000000000000000, 0.8660254037844387076, 1.000000000000000000, 0.8660254037844387076, 1.000000000000000000, 0.8660254037844387076, 1.000000000000000000, 0.8660254037844387076, 1.000000000000000000, 0.8660254037844387076, 1.000000000000000000, 0.8660254037844387076, 1.000000000000000000, 0.8660254037844387076, 1.000000000000000000, 0.8660254037844387076, 1.000000000000000000, 0.8660254037844387076, 1.000000000000000000, 0.8660254037844387076, 1.000000000000000000, 0.8660254037844387076, 1.000000000000000000, 0.8660254037844387076, 1.000000000000000000, 0.8660254037844387076, 1.000000000000000000, 0.8660254037844387076, 1.000000000000000000, 0.8660254037844387076, 1.000000000000000000, 0.8660254037844387076, 1.000000000000000000, 0.8660254037844387076, 1.000000000000000000, 0.8660254037844387076, 1.000000000000000000, 0.8660254037844387076, 1.000000000000000000, 0.8660254037844387076, 1.000000000000000000, 0.8660254037844387076, 1.000000000000000000, 0.8660254037844387076, 1.000000000000000000, 0.8660254037844387076, 1.000000000000000000, 0.8660254037844387076, 1.000000000000000000, 0.8660254037844387076, 1.000000000000000000, 0.8660254037844387076, 1.000000000000000000, 0.8660254037844387076, 1.000000000000000000, 0.8660254037844387076, 1.000000000000000000, 0.8660254037844387076, 1.000000000000000000, 0.8660254037844387076, 1.000000000000000000, 0.8660254037844387076, 1.000000000000000000, 0.8660254037844387076, 1.000000000000000000, 0.8660254037844387076, 1.000000000000000000, 0.8660254037844387076, 1.000000000000000000, 0.8660254037844387076, 1.000000000000000000, 0.8660254037844387076, 1.000000000000000000, 0.8660254037844387076, 1.000000000000000000, 0.8660254037844387076, 1.000000000000000000, 0.8660254037844387076, 1.000000000000000000, 0.8660254037844387076, 1.000000000000000000, 0.8660254037844387076, 1.000000000000000000, 0.8660254037844387076, 1.000000000000000000, 0.8660254037844387076, 1.000000000000000000, 0.8660254037844387076, 1.000000000000000000, 0.8660254037844387076, 1.000000000000000000, 0.8660254037844387076, 1.000000000000000000, 0.8660254037844387076, 1.000000000000000000, 0.8660254037844387076, 1.000000000000000000, 0.8660254037844387076, 1.000000000000000000, 0.8660254037844387076, 1.000000000000000000, 0.8660254037844387076, 1.000000000000000000, 0.8660254037844387076, 1.000000000000000000, 0.8660254037844387076, 1.000000000000000000, 0.8660254037844387076, 1.000000000000000000, 0.8660254037844387076, 1.000000000000000000, 0.8660254037844387076, 1.000000000000000000, 0.8660254037844387076, 1.000000000000000000, 0.8660254037844387076, 1.000000000000000000, 0.8660254037844387076, 1.000000000000000000, 0.9024577157650887083, 0.9469497795711399046, 0.9469497795711399046, 0.9469497795711399046 ) ) 
 REPRESENTATION_ITEM ( '' )  );
#21452=CARTESIAN_POINT ( 'NONE',  ( -96.32500000000001705, 87.70503267997129626, 89.47083333333333144 ) ) ;
#21454=CARTESIAN_POINT ( 'NONE',  ( 92.69370383062498320, 90.00000000000002842, 78.84781250086714977 ) ) ;
#21456=FACE_OUTER_BOUND ( 'NONE', #25020, .T. ) ;
#21461=PLANE ( 'NONE',  #6780 ) ;
#21463=CARTESIAN_POINT ( 'NONE',  ( -94.99999999999997158, -212.6630814284392557, 78.37156250086714238 ) ) ;
#21466=LINE ( 'NONE', #3842, #59070 ) ;
#21468=CARTESIAN_POINT ( 'NONE',  ( -97.64999999999999147, -208.4700217866474929, 84.23208333333334963 ) ) ;
#21473=VECTOR ( 'NONE', #62879, 1000.000000000000000 ) ;
#21474=CARTESIAN_POINT ( 'NONE',  ( -92.34999999999990905, -211.5299782133524502, 88.99458333333333826 ) ) ;
#21476=LINE ( 'NONE', #56830, #15151 ) ;
#21478=CARTESIAN_POINT ( 'NONE',  ( -96.15314808468751551, 88.00268892867056536, 81.49364583420047836 ) ) ;
#21490=CARTESIAN_POINT ( 'NONE',  ( -97.30629616937497417, -208.6684592857803011, 78.95364583420048632 ) ) ;
#21497=CARTESIAN_POINT ( 'NONE',  ( 92.35000000039373447, 90.00002930740642171, 76.74344264317738862 ) ) ;
#21503=ORIENTED_EDGE ( 'NONE', *, *, #54481, .F. ) ;
#21505=CARTESIAN_POINT ( 'NONE',  ( -97.64999999993855795, 90.00001182178863246, 76.10900611559313234 ) ) ;
#21510=CARTESIAN_POINT ( 'NONE',  ( -95.00000000000002842, 93.05995642670504253, 77.77624999999999034 ) ) ;
#21518=CARTESIAN_POINT ( 'NONE',  ( -92.35000000000003695, 90.00000000000004263, 76.98250000000000171 ) ) ;
#21529=CARTESIAN_POINT ( 'NONE',  ( 92.69370383062498320, 90.00000000000002842, 77.10156250086714635 ) ) ;
#21538=CARTESIAN_POINT ( 'NONE',  ( 97.30629616937498838, -209.9999999999999716, 86.15031250086714465 ) ) ;
#21540=VECTOR ( 'NONE', #9269, 1000.000000000000114 ) ;
#21542=DIRECTION ( 'NONE',  ( -0.000000000000000000, -0.000000000000000000, 1.000000000000000000 ) ) ;
#21543=CARTESIAN_POINT ( 'NONE',  ( -94.99999999999997158, -209.9999999999999716, 90.00000000000000000 ) ) ;
#21546=CYLINDRICAL_SURFACE ( 'NONE', #54035, 2.649999999999999467 ) ;
#21550=CARTESIAN_POINT ( 'NONE',  ( -93.84685191531248449, -208.0026889286704943, 88.16114583420046813 ) ) ;
#21551=CARTESIAN_POINT ( 'NONE',  ( -97.30629616937501680, 88.66845928578038638, 84.13947916753383538 ) ) ;
#21553=CARTESIAN_POINT ( 'NONE',  ( 93.84685191531248449, 88.00268892867053694, 86.57364583420047666 ) ) ;
#21554=CARTESIAN_POINT ( 'NONE',  ( -97.30629616937501680, 88.66845928578038638, 86.52072916753381548 ) ) ;
#21555=( BOUNDED_CURVE ( )  B_SPLINE_CURVE ( 2, ( #56341, #40521, #22499, #45814, #50684, #45440, #57086 ),
 .UNSPECIFIED., .F., .F. ) 
 B_SPLINE_CURVE_WITH_KNOTS ( ( 3, 2, 2, 3 ),
 ( 0.02116741234826875415, 0.02822306216352945749, 0.03527882770441185395, 0.04233441017594429673 ),
 .UNSPECIFIED. ) 
 CURVE ( )  GEOMETRIC_REPRESENTATION_ITEM ( )  RATIONAL_B_SPLINE_CURVE ( ( 0.9999956052850527133, 0.8660276011779528549, 1.000000000000000000, 0.8660254037844387076, 1.000000000000000000, 0.8660288798979939306, 0.9999930479532725958 ) ) 
 REPRESENTATION_ITEM ( '' )  );
#21563=CYLINDRICAL_SURFACE ( 'NONE', #54675, 2.649999999999985700 ) ;
#21565=LINE ( 'NONE', #62565, #7062 ) ;
#21568=CARTESIAN_POINT ( 'NONE',  ( -97.65000000000001990, 90.00000000000004263, 83.01499999999998636 ) ) ;
#21571=EDGE_CURVE ( 'NONE', #43311, #36423, #34965, .T. ) ;
#21572=CARTESIAN_POINT ( 'NONE',  ( -96.32500000000001705, 87.70503267997129626, 78.67583333333332973 ) ) ;
#21575=CARTESIAN_POINT ( 'NONE',  ( 93.67499999999998295, 92.29496732002878900, 87.43354166840096298 ) ) ;
#21576=LINE ( 'NONE', #15576, #61363 ) ;
#21579=ADVANCED_FACE ( 'NONE', ( #5986 ), #2115, .F. ) ;
#21581=CARTESIAN_POINT ( 'NONE',  ( -92.69370383062502583, 91.33154071421968467, 82.39322916753381776 ) ) ;
#21584=CARTESIAN_POINT ( 'NONE',  ( -95.00000000000002842, 86.94004357329504273, 85.71374999999999034 ) ) ;
#21588=DIRECTION ( 'NONE',  ( -3.069126149805119941E-16, -1.000000000000000000, 0.000000000000000000 ) ) ;
#21589=CARTESIAN_POINT ( 'NONE',  ( -94.99999999999997158, -212.6630814284392557, 89.32531250086715602 ) ) ;
#21593=CARTESIAN_POINT ( 'NONE',  ( 92.69370383062498320, 91.33154071421968467, 82.12864583420048348 ) ) ;
#21594=CARTESIAN_POINT ( 'NONE',  ( -96.15314808468747287, -208.0026889286704943, 84.61572916753381435 ) ) ;
#21598=CARTESIAN_POINT ( 'NONE',  ( -92.35000000045957336, 90.00004935162611730, 87.22187670868784437 ) ) ;
#21599=CARTESIAN_POINT ( 'NONE',  ( -92.34999999999999432, -211.5299782133524502, 77.56458333333333144 ) ) ;
#21606=CARTESIAN_POINT ( 'NONE',  ( -93.84685191531252713, 88.00268892867056536, 79.85322916753381151 ) ) ;
#21607=CARTESIAN_POINT ( 'NONE',  ( 97.30629616937498838, -209.9999999999999716, 80.43531250086714124 ) ) ;
#21611=CARTESIAN_POINT ( 'NONE',  ( 92.35000000052950497, 90.00003365185392568, 81.18829462297337329 ) ) ;
#21614=CARTESIAN_POINT ( 'NONE',  ( 97.64999999999999147, -209.9999999999999716, 90.00000000000000000 ) ) ;
#21617=EDGE_CURVE ( 'NONE', #46834, #48739, #6636, .T. ) ;
#21619=CARTESIAN_POINT ( 'NONE',  ( 96.15314808468748708, -208.0026889286704943, 75.61989583420049144 ) ) ;
#21624=CARTESIAN_POINT ( 'NONE',  ( 94.99999999999998579, 87.33691857156068750, 87.42031250086715488 ) ) ;
#21627=CARTESIAN_POINT ( 'NONE',  ( 92.35000000000000853, -209.9999999999999716, 76.66499999999999204 ) ) ;
#21629=EDGE_CURVE ( 'NONE', #9811, #18134, #43050, .T. ) ;
#21640=FACE_OUTER_BOUND ( 'NONE', #6906, .T. ) ;
#21641=LINE ( 'NONE', #34783, #57299 ) ;
#21643=CARTESIAN_POINT ( 'NONE',  ( -97.64999999999994884, -211.5299782133524502, 81.24229166840098060 ) ) ;
#21647=CARTESIAN_POINT ( 'NONE',  ( 94.99999999999998579, 93.05995642670504253, 81.03062500173430749 ) ) ;
#21648=CARTESIAN_POINT ( 'NONE',  ( -92.35000000000005116, 91.52997821335253548, 83.46479166840096298 ) ) ;
#21650=CARTESIAN_POINT ( 'NONE',  ( 94.99999999999998579, 92.66308142843935514, 83.29281250086717137 ) ) ;
#21651=EDGE_CURVE ( 'NONE', #5520, #2120, #31656, .T. ) ;
#21653=CARTESIAN_POINT ( 'NONE',  ( -93.67499999999998295, -212.2949673200287179, 82.67104166840096013 ) ) ;
#21658=ORIENTED_EDGE ( 'NONE', *, *, #62312, .T. ) ;
#21659=CARTESIAN_POINT ( 'NONE',  ( 97.65000000000004832, -208.4700217866475214, 77.67041666666666799 ) ) ;
#21661=AXIS2_PLACEMENT_3D ( 'NONE', #8242, #48471, #54124 ) ;
#21670=CARTESIAN_POINT ( 'NONE',  ( -97.65000000000001990, 90.00000000000004263, 90.00000000000000000 ) ) ;
#21671=CARTESIAN_POINT ( 'NONE',  ( -97.30629616937495996, -209.9999999999999716, 80.91156250086716284 ) ) ;
#21677=CARTESIAN_POINT ( 'NONE',  ( -94.99999999999997158, -213.0599564267049857, 76.26812500173430465 ) ) ;
#21678=CARTESIAN_POINT ( 'NONE',  ( 96.15314808468748708, 91.99731107132950569, 77.36614583420046642 ) ) ;
#21685=CARTESIAN_POINT ( 'NONE',  ( 92.34999999999995168, -211.5299782133524218, 83.06791666666666174 ) ) ;
#21686=CARTESIAN_POINT ( 'NONE',  ( 92.69370383062498320, 90.00000000000002842, 89.16656250086715829 ) ) ;
#21690=AXIS2_PLACEMENT_3D ( 'NONE', #22435, #45380, #56278 ) ;
#21691=CARTESIAN_POINT ( 'NONE',  ( -92.69370383062505425, 91.33154071421968467, 82.39322916753381776 ) ) ;
#21704=CARTESIAN_POINT ( 'NONE',  ( 95.00000000000000000, -207.3369185715606307, 78.84781250086714977 ) ) ;
#21715=CARTESIAN_POINT ( 'NONE',  ( 97.64999999999324132, -209.9999940177821713, 82.14187520865721126 ) ) ;
#21716=CARTESIAN_POINT ( 'NONE',  ( 97.64999999999999147, -209.9999999999999716, 87.14249999999999829 ) ) ;
#21718=ORIENTED_EDGE ( 'NONE', *, *, #45073, .T. ) ;
#21725=CARTESIAN_POINT ( 'NONE',  ( 92.35001943615621656, -208.4700105651774606, 78.59645755884378104 ) ) ;
#21726=CARTESIAN_POINT ( 'NONE',  ( 92.35000000000002274, -208.4700217866474645, 81.13645833506764404 ) ) ;
#21727=CARTESIAN_POINT ( 'NONE',  ( 96.32499999999998863, 87.70503267997126784, 81.95666666666666345 ) ) ;
#21730=ORIENTED_EDGE ( 'NONE', *, *, #9397, .F. ) ;
#21732=EDGE_CURVE ( 'NONE', #50224, #14612, #60433, .T. ) ;
#21733=VERTEX_POINT ( 'NONE', #43435 ) ;
#21735=CARTESIAN_POINT ( 'NONE',  ( -92.69370383062504004, 90.00000000000004263, 85.67406250086715147 ) ) ;
#21736=CARTESIAN_POINT ( 'NONE',  ( 97.30629616937498838, 91.33154071421968467, 79.21822916753380639 ) ) ;
#21741=DIRECTION ( 'NONE',  ( -0.000000000000000000, -0.000000000000000000, 1.000000000000000000 ) ) ;
#21745=ORIENTED_EDGE ( 'NONE', *, *, #39498, .T. ) ;
#21750=CARTESIAN_POINT ( 'NONE',  ( -93.84685191531248449, -208.0026889286704943, 81.81114583420047381 ) ) ;
#21753=FACE_OUTER_BOUND ( 'NONE', #26107, .T. ) ;
#21756=FACE_OUTER_BOUND ( 'NONE', #40870, .T. ) ;
#21759=CARTESIAN_POINT ( 'NONE',  ( -92.69370383062498320, -211.3315407142195852, 75.93739583420047268 ) ) ;
#21763=FACE_OUTER_BOUND ( 'NONE', #29032, .T. ) ;
#21769=CARTESIAN_POINT ( 'NONE',  ( 93.84685191531248449, 91.99731107132950569, 88.26697916753380468 ) ) ;
#21775=CARTESIAN_POINT ( 'NONE',  ( 97.64999999999999147, -209.9999999999999716, 78.25249999999999773 ) ) ;
#21776=CARTESIAN_POINT ( 'NONE',  ( 95.00000000000000000, -209.9999999999999716, 90.00000000000000000 ) ) ;
#21778=( BOUNDED_CURVE ( )  B_SPLINE_CURVE ( 2, ( #47748, #47025, #24822, #19542, #7896, #36105, #42492, #18798, #53032, #54146, #65430 ),
 .UNSPECIFIED., .F., .F. ) 
 B_SPLINE_CURVE_WITH_KNOTS ( ( 3, 2, 2, 2, 2, 3 ),
 ( 0.4233457466685775494, 0.4233459324529421086, 0.4304016979938243836, 0.4374574635347067142, 0.4445132290755889337, 0.4445132602971398339 ),
 .UNSPECIFIED. ) 
 CURVE ( )  GEOMETRIC_REPRESENTATION_ITEM ( )  RATIONAL_B_SPLINE_CURVE ( ( 0.9999929448534821130, 0.9999964723338545802, 1.000000000000000000, 0.8660254037844387076, 1.000000000000000000, 0.8660254037844387076, 1.000000000000000000, 0.8660254037844387076, 1.000000000000000000, 0.9999994071664300987, 0.9999988143381067784 ) ) 
 REPRESENTATION_ITEM ( '' )  );
#21781=CARTESIAN_POINT ( 'NONE',  ( 92.35000000000002274, -208.4700217866474361, 84.86708333333332632 ) ) ;
#21784=CARTESIAN_POINT ( 'NONE',  ( -93.67499999999998295, -212.2949673200287179, 84.49666666666666970 ) ) ;
#21787=CARTESIAN_POINT ( 'NONE',  ( -95.00000000000002842, 93.05995642670504253, 77.14124999999999943 ) ) ;
#21795=CARTESIAN_POINT ( 'NONE',  ( 92.69370383062501162, -209.9999999999999716, 89.16656250086715829 ) ) ;
#21806=CARTESIAN_POINT ( 'NONE',  ( 92.69370383062501162, -208.6684592857803295, 76.88989583420047325 ) ) ;
#21808=CARTESIAN_POINT ( 'NONE',  ( 97.30629616937498838, -211.3315407142195852, 83.08114583420048405 ) ) ;
#21813=CARTESIAN_POINT ( 'NONE',  ( -92.69370383062502583, 91.33154071421968467, 75.56697916753383026 ) ) ;
#21819=CARTESIAN_POINT ( 'NONE',  ( 97.64999999999999147, 90.00000000000002842, 85.87249999999998806 ) ) ;
#21829=CARTESIAN_POINT ( 'NONE',  ( 97.30629616937498838, -209.9999999999999716, 75.35531250086714294 ) ) ;
#21831=EDGE_CURVE ( 'NONE', #2794, #65091, #39361, .T. ) ;
#21833=LINE ( 'NONE', #60944, #58198 ) ;
#21836=VERTEX_POINT ( 'NONE', #11410 ) ;
#21839=CARTESIAN_POINT ( 'NONE',  ( -92.69370383062502583, 91.33154071421968467, 74.93197916753381094 ) ) ;
#21841=CARTESIAN_POINT ( 'NONE',  ( 92.69370383062498320, 90.00000000000002842, 76.30781250086714351 ) ) ;
#21843=CARTESIAN_POINT ( 'NONE',  ( 97.64999999999999147, 90.00000000000002842, 78.33187500173430351 ) ) ;
#21844=CARTESIAN_POINT ( 'NONE',  ( -92.69370383062498320, -209.9999999999999716, 88.05531250086713158 ) ) ;
#21849=CARTESIAN_POINT ( 'NONE',  ( -96.15314808468745866, -211.9973110713294489, 78.31864583420048120 ) ) ;
#21859=CARTESIAN_POINT ( 'NONE',  ( -96.32499999999996021, -212.2949673200287179, 88.83583333333334053 ) ) ;
#21862=CARTESIAN_POINT ( 'NONE',  ( -97.30629616937501680, 88.66845928578038638, 80.80572916753382628 ) ) ;
#21866=VERTEX_POINT ( 'NONE', #44900 ) ;
#21874=CYLINDRICAL_SURFACE ( 'NONE', #46027, 2.649999999999985700 ) ;
#21875=CARTESIAN_POINT ( 'NONE',  ( -97.30629616937497417, -208.6684592857803011, 80.85864583420048746 ) ) ;
#21884=EDGE_CURVE ( 'NONE', #70651, #47514, #24417, .T. ) ;
#21888=EDGE_CURVE ( 'NONE', #13854, #64948, #190, .T. ) ;
#21893=CARTESIAN_POINT ( 'NONE',  ( 93.84685191531251292, -211.9973110713294489, 88.47864583420047779 ) ) ;
#21894=CARTESIAN_POINT ( 'NONE',  ( -97.64999999969889188, -209.9999754409357422, 87.53856274002470172 ) ) ;
#21895=ORIENTED_EDGE ( 'NONE', *, *, #70274, .T. ) ;
#21901=CYLINDRICAL_SURFACE ( 'NONE', #34669, 2.649999999999985700 ) ;
#21913=CARTESIAN_POINT ( 'NONE',  ( 97.30629616937498838, 91.33154071421968467, 75.56697916753383026 ) ) ;
#21919=CARTESIAN_POINT ( 'NONE',  ( 94.99999999999998579, 87.33691857156068750, 87.26156250086714294 ) ) ;
#21922=CARTESIAN_POINT ( 'NONE',  ( 95.00000000000000000, -207.3369185715606307, 84.40406250086712703 ) ) ;
#21925=EDGE_CURVE ( 'NONE', #73949, #33726, #47918, .T. ) ;
#21933=CARTESIAN_POINT ( 'NONE',  ( -92.69370383062498320, -211.3315407142195852, 89.27239583420048064 ) ) ;
#21934=CARTESIAN_POINT ( 'NONE',  ( -97.30629616937501680, 91.33154071421968467, 85.30364583420048064 ) ) ;
#21936=CARTESIAN_POINT ( 'NONE',  ( 94.99999999999998579, 92.66308142843935514, 86.30906250086715659 ) ) ;
#21937=CARTESIAN_POINT ( 'NONE',  ( -95.00000000000002842, 87.33691857156074434, 85.35656250086714181 ) ) ;
#21940=CARTESIAN_POINT ( 'NONE',  ( -97.64999999999996305, -209.9999999999999716, 80.55437500173430010 ) ) ;
#21948=ORIENTED_EDGE ( 'NONE', *, *, #26501, .T. ) ;
#21950=CARTESIAN_POINT ( 'NONE',  ( -97.65000000000001990, 91.52997821335253548, 82.32708333333332007 ) ) ;
#21952=CARTESIAN_POINT ( 'NONE',  ( 96.32499999999998863, -207.7050326799711968, 75.81833333333332803 ) ) ;
#21959=CARTESIAN_POINT ( 'NONE',  ( -95.00000000000002842, 92.66308142843932671, 80.59406250086715318 ) ) ;
#21962=AXIS2_PLACEMENT_3D ( 'NONE', #11442, #17459, #4724 ) ;
#21965=LINE ( 'NONE', #50536, #22083 ) ;
#21966=CARTESIAN_POINT ( 'NONE',  ( -92.69370383062498320, -211.3315407142195852, 88.16114583420048234 ) ) ;
#21971=CARTESIAN_POINT ( 'NONE',  ( 94.99999999999998579, 87.33691857156068750, 81.70531250086715147 ) ) ;
#21973=CARTESIAN_POINT ( 'NONE',  ( -96.15314808468745866, -211.9973110713294489, 79.74739583420048916 ) ) ;
#21982=CARTESIAN_POINT ( 'NONE',  ( -96.15314808468751551, 88.00268892867056536, 77.84239583420048803 ) ) ;
#21983=CARTESIAN_POINT ( 'NONE',  ( 97.30629616937498838, -208.6684592857803011, 79.85322916753379729 ) ) ;
#21985=CARTESIAN_POINT ( 'NONE',  ( -92.35000000000003695, 90.00000000000004263, 75.07749999999998636 ) ) ;
#21990=CARTESIAN_POINT ( 'NONE',  ( -6.938893903907228378E-15, 80.00000000000000000, -110.0000000000000000 ) ) ;
#21992=ORIENTED_EDGE ( 'NONE', *, *, #46120, .T. ) ;
#21997=EDGE_LOOP ( 'NONE', ( #69555, #69360, #42248, #39610 ) ) ;
#22000=DIRECTION ( 'NONE',  ( -0.000000000000000000, -0.000000000000000000, 1.000000000000000000 ) ) ;
#22001=( BOUNDED_CURVE ( )  B_SPLINE_CURVE ( 2, ( #41918, #11487, #46828, #40432, #23514, #64119, #12955, #24621, #46447 ),
 .UNSPECIFIED., .F., .F. ) 
 B_SPLINE_CURVE_WITH_KNOTS ( ( 3, 2, 2, 2, 3 ),
 ( 0.6561861948910820974, 0.6632419608429419577, 0.6702977263838236777, 0.6773534919247052866, 0.6773535682752289677 ),
 .UNSPECIFIED. ) 
 CURVE ( )  GEOMETRIC_REPRESENTATION_ITEM ( )  RATIONAL_B_SPLINE_CURVE ( ( 1.000000000000000000, 0.8660254037844387076, 1.000000000000000000, 0.8660254037844387076, 1.000000000000000000, 0.8660254037844387076, 1.000000000000000000, 0.9999985502592857456, 0.9999971005499468379 ) ) 
 REPRESENTATION_ITEM ( '' )  );
#22002=CARTESIAN_POINT ( 'NONE',  ( 97.30629616937498838, 90.00000000000002842, 87.57906250086715261 ) ) ;
#22004=CARTESIAN_POINT ( 'NONE',  ( 92.35000000000002274, -208.4700217866474645, 76.61208333333333087 ) ) ;
#22005=ORIENTED_EDGE ( 'NONE', *, *, #27975, .F. ) ;
#22009=VERTEX_POINT ( 'NONE', #26018 ) ;
#22010=CARTESIAN_POINT ( 'NONE',  ( 97.64999999999990621, -208.4700217866474361, 89.10041666666667481 ) ) ;
#22011=VECTOR ( 'NONE', #26235, 1000.000000000000000 ) ;
#22018=CARTESIAN_POINT ( 'NONE',  ( -97.64999999999994884, -211.5299782133524502, 81.87729166840097150 ) ) ;
#22022=CARTESIAN_POINT ( 'NONE',  ( 92.34999999999999432, 91.52997821335252127, 83.04145833506763097 ) ) ;
#22023=CARTESIAN_POINT ( 'NONE',  ( -95.00000000000002842, 86.94004357329504273, 83.25312500173430408 ) ) ;
#22026=CARTESIAN_POINT ( 'NONE',  ( 97.30629616937498838, 91.33154071421968467, 83.82197916753382572 ) ) ;
#22029=CARTESIAN_POINT ( 'NONE',  ( -97.64999999950704535, 89.99996796756893502, 85.63541623677065218 ) ) ;
#22030=PLANE ( 'NONE',  #13378 ) ;
#22032=CARTESIAN_POINT ( 'NONE',  ( 96.32499999999997442, 92.29496732002878900, 87.88333333333332575 ) ) ;
#22034=CARTESIAN_POINT ( 'NONE',  ( -92.35000000000003695, 89.99999997928479445, 80.87187500099602744 ) ) ;
#22044=CARTESIAN_POINT ( 'NONE',  ( -97.65000000000001990, 90.00000000000004263, 90.00000000000000000 ) ) ;
#22046=CARTESIAN_POINT ( 'NONE',  ( -97.30629616937495996, -209.9999999999999716, 82.18156250086715886 ) ) ;
#22049=EDGE_LOOP ( 'NONE', ( #54563, #43345, #50477, #50571 ) ) ;
#22051=CARTESIAN_POINT ( 'NONE',  ( -96.32499999999996021, -212.2949673200287179, 77.48520833506763950 ) ) ;
#22052=CARTESIAN_POINT ( 'NONE',  ( 92.35000000006144205, 90.00001182123735077, 81.82400613091868991 ) ) ;
#22068=CARTESIAN_POINT ( 'NONE',  ( -94.99999999999997158, -207.3369185715606307, 89.64281250086715147 ) ) ;
#22070=ORIENTED_EDGE ( 'NONE', *, *, #70430, .F. ) ;
#22072=DIRECTION ( 'NONE',  ( 1.000000000000000000, 0.000000000000000000, 0.000000000000000000 ) ) ;
#22073=CARTESIAN_POINT ( 'NONE',  ( -96.15314808468751551, 88.00268892867056536, 78.95364583420047211 ) ) ;
#22075=CARTESIAN_POINT ( 'NONE',  ( 93.84685191531249870, -208.0026889286704943, 89.53697916753381492 ) ) ;
#22076=ORIENTED_EDGE ( 'NONE', *, *, #4899, .F. ) ;
#22078=CARTESIAN_POINT ( 'NONE',  ( 92.35000000000000853, -211.5299782133524218, 79.97229166840095615 ) ) ;
#22080=CARTESIAN_POINT ( 'NONE',  ( 97.65000000000009095, 88.47002178664759242, 83.27958333333332064 ) ) ;
#22081=EDGE_CURVE ( 'NONE', #11565, #14594, #60621, .T. ) ;
#22082=CARTESIAN_POINT ( 'NONE',  ( -97.64999999999996305, -209.9999999999999716, 90.00000000000000000 ) ) ;
#22083=VECTOR ( 'NONE', #5441, 1000.000000000000000 ) ;
#22086=CARTESIAN_POINT ( 'NONE',  ( 92.69370383062501162, -208.6684592857803011, 76.41364583420049428 ) ) ;
#22095=CARTESIAN_POINT ( 'NONE',  ( 93.67500000000001137, -212.2949673200287179, 81.93020833506763267 ) ) ;
#22096=CARTESIAN_POINT ( 'NONE',  ( 97.64999999999997726, -208.4700217866474645, 89.10041666666667481 ) ) ;
#22099=CARTESIAN_POINT ( 'NONE',  ( 95.00000000000000000, -209.9999999999999716, 73.40771935957695860 ) ) ;
#22106=CARTESIAN_POINT ( 'NONE',  ( 92.35000000000002274, -208.4700217866474645, 77.32645833506762756 ) ) ;
#22107=CARTESIAN_POINT ( 'NONE',  ( 92.34999999999999432, 88.47002178664753558, 81.16291666666666060 ) ) ;
#22113=ORIENTED_EDGE ( 'NONE', *, *, #31067, .F. ) ;
#22115=CARTESIAN_POINT ( 'NONE',  ( -93.84685191531254134, 91.99731107132950569, 85.77989583420048803 ) ) ;
#22116=CARTESIAN_POINT ( 'NONE',  ( 92.69370383062498320, 91.33154071421968467, 77.52489583420046415 ) ) ;
#22125=CARTESIAN_POINT ( 'NONE',  ( -93.84685191531248449, -208.0026889286704943, 79.27114583420046756 ) ) ;
#22129=PLANE ( 'NONE',  #48122 ) ;
#22136=CARTESIAN_POINT ( 'NONE',  ( -97.30629616937497417, -208.6684592857803011, 89.74864583420048803 ) ) ;
#22142=CARTESIAN_POINT ( 'NONE',  ( -92.34999999999999432, -208.4700217866474645, 89.17979166840096639 ) ) ;
#22148=CARTESIAN_POINT ( 'NONE',  ( 94.99999999999998579, 87.33691857156068750, 83.45156250086714067 ) ) ;
#22153=CARTESIAN_POINT ( 'NONE',  ( 93.67500000000001137, -207.7050326799711968, 86.71916666666666629 ) ) ;
#22163=CARTESIAN_POINT ( 'NONE',  ( -95.00000000000002842, 92.66308142843932671, 89.48406250086713953 ) ) ;
#22165=CARTESIAN_POINT ( 'NONE',  ( -97.64999999999996305, -209.9999999999999716, 85.55499999999999261 ) ) ;
#22170=CARTESIAN_POINT ( 'NONE',  ( -0.0004442498525516064278, 0.001194404164626844313, -64.00000000000000000 ) ) ;
#22175=CARTESIAN_POINT ( 'NONE',  ( 97.30629616937498838, -211.3315407142195852, 86.25614583420048120 ) ) ;
#22182=CARTESIAN_POINT ( 'NONE',  ( 97.30629616937498838, -208.6684592857803295, 76.67822916753378593 ) ) ;
#22186=CARTESIAN_POINT ( 'NONE',  ( 92.69370383062501162, -209.9999999999999716, 84.08656250086716000 ) ) ;
#22187=EDGE_LOOP ( 'NONE', ( #8531, #61499, #54122, #37565 ) ) ;
#22192=CARTESIAN_POINT ( 'NONE',  ( -92.34999999999999432, -209.9999999999999716, 77.61749999999999261 ) ) ;
#22206=CARTESIAN_POINT ( 'NONE',  ( 96.15314808468748708, -208.0026889286704943, 76.73114583420047552 ) ) ;
#22214=CARTESIAN_POINT ( 'NONE',  ( -96.15314808468751551, 88.00268892867056536, 76.57239583420049200 ) ) ;
#22216=CARTESIAN_POINT ( 'NONE',  ( 94.99999999999998579, 92.66308142843935514, 75.51406250086714067 ) ) ;
#22218=( BOUNDED_CURVE ( )  B_SPLINE_CURVE ( 2, ( #69191, #40619, #73702, #78, #34596, #22971, #17313 ),
 .UNSPECIFIED., .F., .F. ) 
 B_SPLINE_CURVE_WITH_KNOTS ( ( 3, 2, 2, 3 ),
 ( 0.8958333333333331483, 0.9027777777777775681, 0.9097222222222218768, 0.9166666666666662966 ),
 .UNSPECIFIED. ) 
 CURVE ( )  GEOMETRIC_REPRESENTATION_ITEM ( )  RATIONAL_B_SPLINE_CURVE ( ( 1.000000000000004219, 0.8660254037844343777, 1.000000000000000000, 0.8660254037844387076, 1.000000000000000000, 0.8660254037844451469, 0.9999999999999935607 ) ) 
 REPRESENTATION_ITEM ( '' )  );
#22220=CARTESIAN_POINT ( 'NONE',  ( -94.99999999999997158, -207.3369185715606307, 87.57906250086713840 ) ) ;
#22223=DIRECTION ( 'NONE',  ( -1.343011723336883198E-16, 1.000000000000000000, 0.000000000000000000 ) ) ;
#22225=CARTESIAN_POINT ( 'NONE',  ( -93.84685191531248449, -208.0026889286704943, 79.90614583420047268 ) ) ;
#22232=ORIENTED_EDGE ( 'NONE', *, *, #27848, .F. ) ;
#22233=CARTESIAN_POINT ( 'NONE',  ( -97.65000000000001990, 90.00000929204281874, 84.99937468035460597 ) ) ;
#22237=CARTESIAN_POINT ( 'NONE',  ( -92.69370383062504004, 90.00000000000004263, 81.70531250086713726 ) ) ;
#22251=CARTESIAN_POINT ( 'NONE',  ( -96.15314808468745866, -211.9973110713294489, 81.01739583420049939 ) ) ;
#22253=CYLINDRICAL_SURFACE ( 'NONE', #58472, 2.649999999999985700 ) ;
#22272=CARTESIAN_POINT ( 'NONE',  ( 93.84685191531251292, -211.9973110713294489, 87.20864583420046756 ) ) ;
#22273=CARTESIAN_POINT ( 'NONE',  ( 96.32499999999998863, -207.7050326799711968, 85.97833333333332462 ) ) ;
#22278=ORIENTED_EDGE ( 'NONE', *, *, #20562, .T. ) ;
#22287=CARTESIAN_POINT ( 'NONE',  ( 92.34999999999999432, 88.47002178664753558, 88.78291666666667936 ) ) ;
#22293=CARTESIAN_POINT ( 'NONE',  ( 96.15314808468748708, 91.99731107132950569, 84.98614583420047097 ) ) ;
#22296=CARTESIAN_POINT ( 'NONE',  ( 97.30629616937498838, -208.6684592857803011, 85.56822916753380071 ) ) ;
#22298=DIRECTION ( 'NONE',  ( 1.000000000000000000, 0.000000000000000000, 0.000000000000000000 ) ) ;
#22299=CARTESIAN_POINT ( 'NONE',  ( -97.64999999999996305, -209.9999999999999716, 80.47499999999999432 ) ) ;
#22305=CARTESIAN_POINT ( 'NONE',  ( -92.69370383062498320, -209.9999999999999716, 87.42031250086714067 ) ) ;
#22306=CARTESIAN_POINT ( 'NONE',  ( -97.30629616937501680, 91.33154071421968467, 87.20864583420049598 ) ) ;
#22309=CARTESIAN_POINT ( 'NONE',  ( 96.15314808468748708, 91.99731107132950569, 83.08114583420048405 ) ) ;
#22310=CARTESIAN_POINT ( 'NONE',  ( -96.15314808468751551, 88.00268892867056536, 85.30364583420046642 ) ) ;
#22317=CARTESIAN_POINT ( 'NONE',  ( -96.15314808468747287, -208.0026889286704943, 88.26697916753380468 ) ) ;
#22318=DIRECTION ( 'NONE',  ( -0.000000000000000000, -0.000000000000000000, 1.000000000000000000 ) ) ;
#22327=CARTESIAN_POINT ( 'NONE',  ( -95.00000000000002842, 86.94004357329504273, 82.53874999999999318 ) ) ;
#22337=CARTESIAN_POINT ( 'NONE',  ( -95.00000000000002842, 87.33691857156074434, 78.37156250086714238 ) ) ;
#22339=DIRECTION ( 'NONE',  ( 1.000000000000000000, 0.000000000000000000, 0.000000000000000000 ) ) ;
#22342=CARTESIAN_POINT ( 'NONE',  ( -97.65000000000001990, 90.00000000000004263, 82.37999999999999545 ) ) ;
#22343=CARTESIAN_POINT ( 'NONE',  ( -99.99999999999997158, -214.9999999999999716, -90.00000000000000000 ) ) ;
#22347=CARTESIAN_POINT ( 'NONE',  ( 96.15314808468748708, 91.99731107132950569, 78.79489583420048859 ) ) ;
#22348=CARTESIAN_POINT ( 'NONE',  ( -97.30629616937495996, -209.9999999999999716, 80.27656250086714351 ) ) ;
#22349=CARTESIAN_POINT ( 'NONE',  ( -93.67500000000003979, 92.29496732002878900, 84.78770833506763438 ) ) ;
#22350=VERTEX_POINT ( 'NONE', #73724 ) ;
#22352=CARTESIAN_POINT ( 'NONE',  ( -92.34999999999998010, -211.0689551420226735, 75.04052853044679239 ) ) ;
#22353=FACE_OUTER_BOUND ( 'NONE', #45209, .T. ) ;
#22358=CARTESIAN_POINT ( 'NONE',  ( -93.84685191531252713, 88.00268892867056536, 77.94822916753382458 ) ) ;
#22359=CARTESIAN_POINT ( 'NONE',  ( 95.00000000000000000, -207.3369185715606307, 79.32406250086714294 ) ) ;
#22360=ORIENTED_EDGE ( 'NONE', *, *, #44469, .F. ) ;
#22368=VECTOR ( 'NONE', #18462, 1000.000000000000000 ) ;
#22372=CARTESIAN_POINT ( 'NONE',  ( 92.69370383062501162, -209.9999999999999716, 76.46656250086715545 ) ) ;
#22376=CARTESIAN_POINT ( 'NONE',  ( 97.30629616937498838, 90.00000000000002842, 88.21406250086714351 ) ) ;
#22378=CARTESIAN_POINT ( 'NONE',  ( 96.32499999999998863, -207.7050326799711968, 78.99333333333332519 ) ) ;
#22382=EDGE_LOOP ( 'NONE', ( #48468, #39797, #72217, #6831, #63349, #67024, #32809, #41912, #52402, #7870, #1617, #32138, #73872, #49926, #25887, #6053, #36359, #20790, #64544, #9323, #5599, #5843, #21745, #20555, #66564, #16026, #38452, #40769, #25534, #25264, #14508, #44707, #35749, #68876, #23386, #52539, #67964, #42907, #53433, #64860, #37987, #11100, #56866, #3262, #10385, #67712, #8027, #61351, #59213, #14960 ) ) ;
#22392=CARTESIAN_POINT ( 'NONE',  ( -94.99999999999997158, -213.0599564267049857, 81.98312500173430806 ) ) ;
#22397=CARTESIAN_POINT ( 'NONE',  ( 92.34999999999999432, 88.47002178664753558, 83.14729166840096752 ) ) ;
#22398=CARTESIAN_POINT ( 'NONE',  ( -97.65000000000001990, 88.47002178664754979, 79.33729166840096525 ) ) ;
#22400=CARTESIAN_POINT ( 'NONE',  ( 96.15314808468748708, 91.99731107132950569, 83.23989583420049598 ) ) ;
#22407=CARTESIAN_POINT ( 'NONE',  ( -97.64999999953492704, -210.0000309987302956, 83.09538598079114990 ) ) ;
#22408=VERTEX_POINT ( 'NONE', #24103 ) ;
#22410=CARTESIAN_POINT ( 'NONE',  ( -97.64999999960637922, 90.00002930319634231, 82.45844277051273252 ) ) ;
#22411=DIRECTION ( 'NONE',  ( -0.000000000000000000, -0.000000000000000000, 1.000000000000000000 ) ) ;
#22419=CARTESIAN_POINT ( 'NONE',  ( 2.499999999999984457, -73.00000000000001421, -251.7000000000000455 ) ) ;
#22421=CARTESIAN_POINT ( 'NONE',  ( -92.35000000000005116, 88.47002178664754979, 80.18395833506764347 ) ) ;
#22423=CARTESIAN_POINT ( 'NONE',  ( -97.30629616937497417, -208.6684592857803011, 80.22364583420048234 ) ) ;
#22426=CARTESIAN_POINT ( 'NONE',  ( -97.30629616937501680, 88.66845928578038638, 88.42572916753380241 ) ) ;
#22427=EDGE_LOOP ( 'NONE', ( #11270, #44103, #73410, #25981 ) ) ;
#22432=CARTESIAN_POINT ( 'NONE',  ( 94.99999999999998579, 92.66308142843932671, 74.87906250086713555 ) ) ;
#22435=CARTESIAN_POINT ( 'NONE',  ( -95.00000000000002842, 90.00000000000004263, 90.00000000000000000 ) ) ;
#22442=CARTESIAN_POINT ( 'NONE',  ( 97.30629616937498838, 91.33154071421968467, 89.53697916753382913 ) ) ;
#22443=CARTESIAN_POINT ( 'NONE',  ( -97.30629616937497417, -208.6684592857803295, 89.11364583420049712 ) ) ;
#22447=CARTESIAN_POINT ( 'NONE',  ( -92.69370383062505425, 91.33154071421968467, 79.85322916753379729 ) ) ;
#22451=( BOUNDED_CURVE ( )  B_SPLINE_CURVE ( 2, ( #37780, #8826, #48677, #65987, #14462, #71217, #42670, #49416, #72692 ),
 .UNSPECIFIED., .F., .F. ) 
 B_SPLINE_CURVE_WITH_KNOTS ( ( 3, 2, 2, 2, 3 ),
 ( 0.8678591737214811364, 0.8749149270694133174, 0.8819706926102951483, 0.8890264581511769792, 0.8890265259358467453 ),
 .UNSPECIFIED. ) 
 CURVE ( )  GEOMETRIC_REPRESENTATION_ITEM ( )  RATIONAL_B_SPLINE_CURVE ( ( 1.000000000000000000, 0.8660254037844387076, 1.000000000000000000, 0.8660254037844387076, 1.000000000000000000, 0.8660254037844387076, 1.000000000000000000, 0.9999987129073784065, 0.9999974258394870308 ) ) 
 REPRESENTATION_ITEM ( '' )  );
#22452=DIRECTION ( 'NONE',  ( -0.000000000000000000, -0.000000000000000000, 1.000000000000000000 ) ) ;
#22453=DIRECTION ( 'NONE',  ( -0.000000000000000000, -0.000000000000000000, 1.000000000000000000 ) ) ;
#22458=CARTESIAN_POINT ( 'NONE',  ( 92.69370383062501162, -211.3315407142195852, 75.24947916753383481 ) ) ;
#22463=CARTESIAN_POINT ( 'NONE',  ( 97.30629616937497417, -209.9999999999998863, 74.79348190356849102 ) ) ;
#22469=LINE ( 'NONE', #51034, #63331 ) ;
#22470=CARTESIAN_POINT ( 'NONE',  ( 93.67500000000001137, -207.7050326799711968, 86.71916666666666629 ) ) ;
#22475=ORIENTED_EDGE ( 'NONE', *, *, #13651, .F. ) ;
#22481=EDGE_LOOP ( 'NONE', ( #56405, #37114, #62885, #42899 ) ) ;
#22483=CARTESIAN_POINT ( 'NONE',  ( 95.00000000000000000, -213.0599564267049857, 75.63312500173429953 ) ) ;
#22484=CARTESIAN_POINT ( 'NONE',  ( 94.99999999999998579, 86.94004357329500010, 82.53874999999999318 ) ) ;
#22488=CARTESIAN_POINT ( 'NONE',  ( 95.00000000000000000, -206.9400435732949575, 75.31562500173430408 ) ) ;
#22492=CARTESIAN_POINT ( 'NONE',  ( 97.64999017507813051, -211.5299838857737029, 88.43895794268867405 ) ) ;
#22493=CARTESIAN_POINT ( 'NONE',  ( -97.30629616937501680, 91.33154071421968467, 80.22364583420048234 ) ) ;
#22494=CARTESIAN_POINT ( 'NONE',  ( 94.99999999999998579, 92.66308142843935514, 79.32406250086714294 ) ) ;
#22499=CARTESIAN_POINT ( 'NONE',  ( 96.32499999999998863, 87.70503267997126784, 89.02104166840096866 ) ) ;
#22503=CARTESIAN_POINT ( 'NONE',  ( -92.69370383062498320, -211.3315407142195852, 77.84239583420045960 ) ) ;
#22506=CARTESIAN_POINT ( 'NONE',  ( 97.65000000000000568, 91.52997821335252127, 75.20979166840096752 ) ) ;
#22512=CARTESIAN_POINT ( 'NONE',  ( -97.30629616937497417, -211.3315407142195852, 75.72572916753381378 ) ) ;
#22514=CARTESIAN_POINT ( 'NONE',  ( -97.64999999999996305, -209.9999999999999716, 81.74500000000000455 ) ) ;
#22515=EDGE_CURVE ( 'NONE', #11290, #26437, #58669, .T. ) ;
#22519=CARTESIAN_POINT ( 'NONE',  ( 92.35000000000000853, -209.9999999999999716, 81.74500000000000455 ) ) ;
#22522=CARTESIAN_POINT ( 'NONE',  ( 95.00000000000000000, -206.9400435732949575, 86.11062500173430578 ) ) ;
#22523=CARTESIAN_POINT ( 'NONE',  ( 97.30629616937498838, 90.00000000000002842, 86.15031250086714465 ) ) ;
#22524=VECTOR ( 'NONE', #3958, 1000.000000000000000 ) ;
#22527=CARTESIAN_POINT ( 'NONE',  ( 92.35000000000000853, -209.9999999999999716, 86.82500000000000284 ) ) ;
#22531=CARTESIAN_POINT ( 'NONE',  ( 97.65000000000000568, -211.5299782133524218, 87.80395833506766223 ) ) ;
#22540=CARTESIAN_POINT ( 'NONE',  ( -94.99999999999997158, -206.9400435732949575, 83.49125000000000796 ) ) ;
#22542=CARTESIAN_POINT ( 'NONE',  ( -93.67500000000003979, 87.70503267997129626, 80.05166666666666231 ) ) ;
#22548=CARTESIAN_POINT ( 'NONE',  ( 92.69370383062501162, -209.9999999999999716, 85.35656250086715602 ) ) ;
#22554=CARTESIAN_POINT ( 'NONE',  ( 95.00000000000000000, -207.3369185715606307, 77.41906250086714181 ) ) ;
#22557=CARTESIAN_POINT ( 'NONE',  ( 93.84685191531251292, -211.9973110713294489, 82.28739583420048120 ) ) ;
#22560=EDGE_CURVE ( 'NONE', #33726, #26516, #47044, .T. ) ;
#22569=ORIENTED_EDGE ( 'NONE', *, *, #20343, .F. ) ;
#22570=CARTESIAN_POINT ( 'NONE',  ( 93.67500000000001137, -207.7050326799711968, 86.79854166840097207 ) ) ;
#22579=ORIENTED_EDGE ( 'NONE', *, *, #63115, .T. ) ;
#22589=CARTESIAN_POINT ( 'NONE',  ( -0.0004442498525516064278, 0.001194404164626844313, -80.00000000000001421 ) ) ;
#22592=CARTESIAN_POINT ( 'NONE',  ( -97.30629616937501680, 88.66845928578038638, 76.51947916753381662 ) ) ;
#22595=LINE ( 'NONE', #23697, #65944 ) ;
#22599=CARTESIAN_POINT ( 'NONE',  ( -94.99999999999997158, -212.6630814284392557, 86.62656250086715204 ) ) ;
#22603=CARTESIAN_POINT ( 'NONE',  ( 93.32700159667696482, -211.9834083483116274, 74.96344747200082281 ) ) ;
#22604=CARTESIAN_POINT ( 'NONE',  ( 92.34999999999999432, 90.00000000000002842, 81.10999999999999943 ) ) ;
#22612=CARTESIAN_POINT ( 'NONE',  ( -93.84685191531254134, 91.99731107132950569, 81.17614583420048291 ) ) ;
#22625=CARTESIAN_POINT ( 'NONE',  ( -97.30629616937495996, -209.9999999999999716, 80.27656250086714351 ) ) ;
#22627=DIRECTION ( 'NONE',  ( 1.000000000000000000, 0.000000000000000000, 0.000000000000000000 ) ) ;
#22628=ORIENTED_EDGE ( 'NONE', *, *, #8942, .F. ) ;
#22630=CARTESIAN_POINT ( 'NONE',  ( 97.65000000000000568, 91.52997821335252127, 76.47979166840096354 ) ) ;
#22643=CARTESIAN_POINT ( 'NONE',  ( 97.30629616937498838, -208.6684592857803295, 89.37822916753378877 ) ) ;
#22644=CARTESIAN_POINT ( 'NONE',  ( -93.67500000000003979, 92.29496732002878900, 82.24770833506762813 ) ) ;
#22647=CARTESIAN_POINT ( 'NONE',  ( 97.64999999999999147, -209.9999999999999716, 75.07749999999998636 ) ) ;
#22651=CARTESIAN_POINT ( 'NONE',  ( -97.64999999999996305, -209.9999999999999716, 79.91937500173429498 ) ) ;
#22653=ORIENTED_EDGE ( 'NONE', *, *, #49158, .F. ) ;
#22659=EDGE_LOOP ( 'NONE', ( #34670, #49029, #15935, #50528 ) ) ;
#22661=( BOUNDED_CURVE ( )  B_SPLINE_CURVE ( 2, ( #69776, #6275, #52867, #47588, #1405, #69053, #70135, #34837, #18277 ),
 .UNSPECIFIED., .F., .F. ) 
 B_SPLINE_CURVE_WITH_KNOTS ( ( 3, 2, 2, 2, 3 ),
 ( 0.4021785743327781493, 0.4021786358302961717, 0.4092344013711782247, 0.4162901669120602222, 0.4233457466685775494 ),
 .UNSPECIFIED. ) 
 CURVE ( )  GEOMETRIC_REPRESENTATION_ITEM ( )  RATIONAL_B_SPLINE_CURVE ( ( 0.9999976645954902210, 0.9999988322875673630, 1.000000000000000000, 0.8660254037844387076, 1.000000000000000000, 0.8660254037844387076, 1.000000000000000000, 0.8660289314505862368, 0.9999929448534778942 ) ) 
 REPRESENTATION_ITEM ( '' )  );
#22662=CARTESIAN_POINT ( 'NONE',  ( 97.64999999999997726, 91.52997821335252127, 89.10041666666667481 ) ) ;
#22665=DIRECTION ( 'NONE',  ( -0.000000000000000000, -0.000000000000000000, 1.000000000000000000 ) ) ;
#22672=CARTESIAN_POINT ( 'NONE',  ( 92.69370383062498320, 90.00000000000002842, 85.19781250086714408 ) ) ;
#22674=CARTESIAN_POINT ( 'NONE',  ( 96.15314808468748708, -208.0026889286704943, 83.71614583420047495 ) ) ;
#22679=CARTESIAN_POINT ( 'NONE',  ( -92.35000000000005116, 91.52997821335253548, 77.74979166840097378 ) ) ;
#22684=CARTESIAN_POINT ( 'NONE',  ( -92.69370383062498320, -209.9999999999999716, 86.15031250086714465 ) ) ;
#22685=CARTESIAN_POINT ( 'NONE',  ( -93.84685191531254134, 91.99731107132950569, 85.14489583420048291 ) ) ;
#22688=CARTESIAN_POINT ( 'NONE',  ( 97.30629616937498838, 88.66845928578037217, 84.19239583420046813 ) ) ;
#22689=CARTESIAN_POINT ( 'NONE',  ( -96.15314808468752972, 91.99731107132950569, 83.82197916753381151 ) ) ;
#22695=CARTESIAN_POINT ( 'NONE',  ( 94.99999999999998579, 93.05995642670504253, 87.30124999999999602 ) ) ;
#22697=CARTESIAN_POINT ( 'NONE',  ( -92.69370383062498320, -211.3315407142195852, 86.73239583420047438 ) ) ;
#22698=CARTESIAN_POINT ( 'NONE',  ( -94.99999999999997158, -213.0599564267049857, 81.90375000000000227 ) ) ;
#22700=CARTESIAN_POINT ( 'NONE',  ( -92.35002509397746451, 88.47000729863293600, 89.07395733288676354 ) ) ;
#22704=CARTESIAN_POINT ( 'NONE',  ( 92.34999999999999432, 90.00000000000002842, 89.36499999999999488 ) ) ;
#22709=CARTESIAN_POINT ( 'NONE',  ( -96.32500000000001705, 92.29496732002878900, 79.09916666666666174 ) ) ;
#22714=CARTESIAN_POINT ( 'NONE',  ( -92.34999999999999432, -209.9999999999999716, 89.68250000000000455 ) ) ;
#22716=CARTESIAN_POINT ( 'NONE',  ( -97.64999999999996305, -209.9999999999999716, 79.83999999999998920 ) ) ;
#22719=CARTESIAN_POINT ( 'NONE',  ( -93.84685191531254134, 91.99731107132950569, 78.00114583420048575 ) ) ;
#22729=CARTESIAN_POINT ( 'NONE',  ( 96.15314808468748708, 88.00268892867053694, 77.94822916753382458 ) ) ;
#22732=CARTESIAN_POINT ( 'NONE',  ( -92.69370383062498320, -208.6684592857803295, 79.37697916753381833 ) ) ;
#22741=CARTESIAN_POINT ( 'NONE',  ( 93.84685191531251292, -211.9973110713294489, 81.49364583420047836 ) ) ;
#22748=EDGE_CURVE ( 'NONE', #73349, #42391, #1415, .T. ) ;
#22763=CARTESIAN_POINT ( 'NONE',  ( 93.84685191531248449, 91.99731107132950569, 82.07572916753382231 ) ) ;
#22764=CARTESIAN_POINT ( 'NONE',  ( 97.64999999999999147, -209.9999999999999716, 78.25249999999999773 ) ) ;
#22765=ORIENTED_EDGE ( 'NONE', *, *, #49900, .F. ) ;
#22766=VERTEX_POINT ( 'NONE', #67646 ) ;
#22767=EDGE_LOOP ( 'NONE', ( #28120, #26012, #43756, #2547, #52416 ) ) ;
#22774=CARTESIAN_POINT ( 'NONE',  ( -92.34999999999999432, -209.9999999999999716, 87.14249999999999829 ) ) ;
#22778=CARTESIAN_POINT ( 'NONE',  ( -94.99999999999997158, -206.9400435732949575, 81.66562500173431260 ) ) ;
#22782=CARTESIAN_POINT ( 'NONE',  ( 94.99999999999998579, 93.05995642670504253, 77.85562500173429612 ) ) ;
#22783=CARTESIAN_POINT ( 'NONE',  ( -92.35000000000003695, 90.00000000000004263, 78.96687500173429441 ) ) ;
#22786=CARTESIAN_POINT ( 'NONE',  ( 96.15314808468748708, 88.00268892867053694, 82.39322916753381776 ) ) ;
#22788=LINE ( 'NONE', #4764, #15087 ) ;
#22790=DIRECTION ( 'NONE',  ( 0.000000000000000000, 1.000000000000000000, 0.000000000000000000 ) ) ;
#22791=CARTESIAN_POINT ( 'NONE',  ( 97.64999999999447766, 89.99999459739470353, 81.50687481489491404 ) ) ;
#22794=VERTEX_POINT ( 'NONE', #3769 ) ;
#22798=EDGE_CURVE ( 'NONE', #58538, #38048, #9039, .T. ) ;
#22805=LINE ( 'NONE', #21670, #46161 ) ;
#22806=CARTESIAN_POINT ( 'NONE',  ( -96.15314808468745866, -211.9973110713294489, 81.65239583420049030 ) ) ;
#22814=FACE_OUTER_BOUND ( 'NONE', #71969, .T. ) ;
#22816=CARTESIAN_POINT ( 'NONE',  ( 93.67499999999999716, 87.70503267997126784, 78.12020833506763040 ) ) ;
#22821=CARTESIAN_POINT ( 'NONE',  ( 93.84685191531248449, 91.99731107132950569, 85.88572916753381037 ) ) ;
#22822=CARTESIAN_POINT ( 'NONE',  ( -93.84685191531247028, -211.9973110713294489, 88.74322916753382628 ) ) ;
#22823=CARTESIAN_POINT ( 'NONE',  ( 92.34999999999999432, 90.00000000000002842, 82.37999999999999545 ) ) ;
#22826=CARTESIAN_POINT ( 'NONE',  ( -92.69370383062505425, 88.66845928578038638, 78.47739583420047893 ) ) ;
#22827=CARTESIAN_POINT ( 'NONE',  ( 96.15314808468748708, -208.0026889286704943, 89.43114583420047836 ) ) ;
#22840=ORIENTED_EDGE ( 'NONE', *, *, #9985, .F. ) ;
#22843=CARTESIAN_POINT ( 'NONE',  ( 97.30629616937498838, -208.6684592857803295, 85.72697916753381264 ) ) ;
#22844=CARTESIAN_POINT ( 'NONE',  ( 92.35000000000000853, -209.9999999999999716, 89.44437500173430067 ) ) ;
#22846=CARTESIAN_POINT ( 'NONE',  ( -96.32499999999996021, -207.7050326799711968, 85.52854166840096184 ) ) ;
#22850=CARTESIAN_POINT ( 'NONE',  ( 97.64999999999997726, -211.5299782133524502, 89.62958333333332916 ) ) ;
#22863=CARTESIAN_POINT ( 'NONE',  ( 97.64999999999997726, -211.5299782133524502, 77.00895833506763211 ) ) ;
#22864=CARTESIAN_POINT ( 'NONE',  ( 97.64999999999997726, 91.52997821335252127, 83.38541666666667140 ) ) ;
#22871=DIRECTION ( 'NONE',  ( 1.000000000000000000, 0.000000000000000000, 0.000000000000000000 ) ) ;
#22874=CARTESIAN_POINT ( 'NONE',  ( -97.30629616937501680, 90.00000000000004263, 82.18156250086715886 ) ) ;
#22875=CARTESIAN_POINT ( 'NONE',  ( 97.30629616937498838, 91.33154071421968467, 76.67822916753378593 ) ) ;
#22877=CYLINDRICAL_SURFACE ( 'NONE', #8135, 2.649999999999985700 ) ;
#22879=FACE_OUTER_BOUND ( 'NONE', #64258, .T. ) ;
#22880=CARTESIAN_POINT ( 'NONE',  ( -92.34999999999993747, -208.4700217866475214, 77.67041666666666799 ) ) ;
#22885=CARTESIAN_POINT ( 'NONE',  ( -94.99999999999997158, -207.3369185715606307, 76.14906250086716000 ) ) ;
#22886=ORIENTED_EDGE ( 'NONE', *, *, #10382, .F. ) ;
#22891=CARTESIAN_POINT ( 'NONE',  ( -97.64999999999996305, -209.9999999999999716, 77.93499999999998806 ) ) ;
#22893=CARTESIAN_POINT ( 'NONE',  ( -92.69370383062498320, -211.3315407142195852, 75.30239583420048177 ) ) ;
#22894=ORIENTED_EDGE ( 'NONE', *, *, #6858, .F. ) ;
#22895=LINE ( 'NONE', #63856, #5081 ) ;
#22896=CARTESIAN_POINT ( 'NONE',  ( 97.64999999999999147, 90.00000000000002842, 83.96750000000000114 ) ) ;
#22897=CARTESIAN_POINT ( 'NONE',  ( -93.08359813425039420, -211.8303114255588753, 74.99954695036822727 ) ) ;
#22904=CARTESIAN_POINT ( 'NONE',  ( 92.69370383062498320, 91.33154071421968467, 83.87489583420047268 ) ) ;
#22912=( BOUNDED_CURVE ( )  B_SPLINE_CURVE ( 2, ( #37423, #3222, #65997, #32495, #8470, #26493, #48683 ),
 .UNSPECIFIED., .F., .F. ) 
 B_SPLINE_CURVE_WITH_KNOTS ( ( 3, 2, 2, 3 ),
 ( 0.7083333333333331483, 0.7152777777777775681, 0.7222222222222220989, 0.7291666666666665186 ),
 .UNSPECIFIED. ) 
 CURVE ( )  GEOMETRIC_REPRESENTATION_ITEM ( )  RATIONAL_B_SPLINE_CURVE ( ( 1.000000000000004219, 0.8660254037844343777, 1.000000000000000000, 0.8660254037844387076, 1.000000000000000000, 0.8660254037844408170, 0.9999999999999978906 ) ) 
 REPRESENTATION_ITEM ( '' )  );
#22915=VECTOR ( 'NONE', #55238, 1000.000000000000000 ) ;
#22917=CARTESIAN_POINT ( 'NONE',  ( -92.69370383062504004, 90.00000000000004263, 89.32531250086714181 ) ) ;
#22930=CARTESIAN_POINT ( 'NONE',  ( 2.499999999999979572, -80.00000000000000000, -280.0000000000000000 ) ) ;
#22932=CARTESIAN_POINT ( 'NONE',  ( 97.30629616937498838, -209.9999999999999716, 85.67406250086715147 ) ) ;
#22938=CARTESIAN_POINT ( 'NONE',  ( 97.30629616937498838, -209.9999999999999716, 77.89531250086714920 ) ) ;
#22940=ORIENTED_EDGE ( 'NONE', *, *, #63102, .T. ) ;
#22941=CARTESIAN_POINT ( 'NONE',  ( 92.69370383062501162, -211.3315407142195852, 84.13947916753383538 ) ) ;
#22944=CARTESIAN_POINT ( 'NONE',  ( -96.32499999999996021, -212.2949673200287179, 88.20083333333332121 ) ) ;
#22945=ORIENTED_EDGE ( 'NONE', *, *, #73510, .T. ) ;
#22951=CARTESIAN_POINT ( 'NONE',  ( -92.35000000000003695, 90.00000000000004263, 77.61749999999999261 ) ) ;
#22952=CARTESIAN_POINT ( 'NONE',  ( 96.32499999999998863, -207.7050326799711968, 87.32770833506762642 ) ) ;
#22957=ORIENTED_EDGE ( 'NONE', *, *, #13312, .T. ) ;
#22961=AXIS2_PLACEMENT_3D ( 'NONE', #65335, #58956, #35628 ) ;
#22971=CARTESIAN_POINT ( 'NONE',  ( 92.35000000000009379, -211.5299782133524502, 76.08291666666664810 ) ) ;
#22974=CARTESIAN_POINT ( 'NONE',  ( -95.00000000000002842, 93.05995642670501411, 86.66624999999999091 ) ) ;
#22979=CARTESIAN_POINT ( 'NONE',  ( -97.30629616937497417, -208.6684592857803011, 84.50989583420046358 ) ) ;
#22984=CARTESIAN_POINT ( 'NONE',  ( -97.30629616937495996, -209.9999999999999716, 75.03781250086713328 ) ) ;
#22991=CARTESIAN_POINT ( 'NONE',  ( -95.00000000000002842, 92.66308142843932671, 77.41906250086714181 ) ) ;
#22995=CARTESIAN_POINT ( 'NONE',  ( 93.67499999999999716, 87.70503267997126784, 79.39020833506762642 ) ) ;
#22996=VECTOR ( 'NONE', #8841, 1000.000000000000000 ) ;
#22999=CARTESIAN_POINT ( 'NONE',  ( 92.35000000000000853, -209.9999999999999716, 89.44437500173430067 ) ) ;
#23004=CARTESIAN_POINT ( 'NONE',  ( -93.84685191531248449, -208.0026889286704943, 78.79489583420048859 ) ) ;
#23007=AXIS2_PLACEMENT_3D ( 'NONE', #58459, #6954, #34798 ) ;
#23010=FACE_OUTER_BOUND ( 'NONE', #6656, .T. ) ;
#23011=LINE ( 'NONE', #51567, #21473 ) ;
#23023=CARTESIAN_POINT ( 'NONE',  ( 92.69370383062501162, -208.6684592857803295, 87.68489583420047495 ) ) ;
#23024=CARTESIAN_POINT ( 'NONE',  ( -93.67499999999998295, -207.7050326799711968, 83.51770833506763836 ) ) ;
#23025=ADVANCED_FACE ( 'NONE', ( #30734 ), #7453, .F. ) ;
#23047=CARTESIAN_POINT ( 'NONE',  ( 97.30629616937498838, 88.66845928578037217, 86.73239583420047438 ) ) ;
#23049=CARTESIAN_POINT ( 'NONE',  ( 93.84685191531249870, -208.0026889286704943, 82.55197916753380127 ) ) ;
#23053=LINE ( 'NONE', #28668, #48605 ) ;
#23055=CARTESIAN_POINT ( 'NONE',  ( -93.67499999999998295, -207.7050326799711968, 89.15333333333333599 ) ) ;
#23056=CARTESIAN_POINT ( 'NONE',  ( 97.64999999999999147, 90.00000000000002842, 90.00000000000000000 ) ) ;
#23058=CARTESIAN_POINT ( 'NONE',  ( -93.84685191531247028, -211.9973110713294489, 85.40947916753380298 ) ) ;
#23059=CARTESIAN_POINT ( 'NONE',  ( -93.84685191531252713, 88.00268892867056536, 83.66322916753382799 ) ) ;
#23062=CARTESIAN_POINT ( 'NONE',  ( 93.84685191531248449, 91.99731107132950569, 85.72697916753379843 ) ) ;
#23063=CARTESIAN_POINT ( 'NONE',  ( -97.30629616937501680, 88.66845928578038638, 84.61572916753380014 ) ) ;
#23066=CARTESIAN_POINT ( 'NONE',  ( -92.35000000000003695, 90.00000000000004263, 78.96687500173429441 ) ) ;
#23067=CARTESIAN_POINT ( 'NONE',  ( 95.00000000000000000, -213.0599564267049857, 76.26812500173430465 ) ) ;
#23070=CARTESIAN_POINT ( 'NONE',  ( -92.69370383062498320, -209.9999999999999716, 87.42031250086714067 ) ) ;
#23075=CARTESIAN_POINT ( 'NONE',  ( 96.32499999999998863, 87.70503267997126784, 89.57666666666666799 ) ) ;
#23077=ORIENTED_EDGE ( 'NONE', *, *, #16325, .T. ) ;
#23079=CARTESIAN_POINT ( 'NONE',  ( -93.67500000000003979, 87.70503267997129626, 76.87666666666666515 ) ) ;
#23080=CARTESIAN_POINT ( 'NONE',  ( 97.64999999999999147, -209.9999999999999716, 90.00000000000000000 ) ) ;
#23087=VERTEX_POINT ( 'NONE', #19094 ) ;
#23088=CARTESIAN_POINT ( 'NONE',  ( -97.30629616937501680, 90.00000000000004263, 76.94281250086713442 ) ) ;
#23092=EDGE_CURVE ( 'NONE', #61621, #58605, #11897, .T. ) ;
#23096=CARTESIAN_POINT ( 'NONE',  ( -92.69370383062498320, -211.3315407142195852, 88.79614583420050167 ) ) ;
#23098=CARTESIAN_POINT ( 'NONE',  ( 97.30629616937498838, 91.33154071421968467, 78.10697916753383652 ) ) ;
#23099=CARTESIAN_POINT ( 'NONE',  ( -97.30629616937495996, -209.9999999999999716, 79.00656250086716170 ) ) ;
#23103=CARTESIAN_POINT ( 'NONE',  ( 97.65000000000000568, 88.47002178664752137, 87.80395833506766223 ) ) ;
#23105=CARTESIAN_POINT ( 'NONE',  ( -96.32499999999996021, -207.7050326799711968, 75.28916666666665947 ) ) ;
#23106=CARTESIAN_POINT ( 'NONE',  ( -94.99999999999997158, -209.9999999999999716, 90.00000000000000000 ) ) ;
#23108=CARTESIAN_POINT ( 'NONE',  ( -95.00000000000002842, 87.33691857156074434, 75.35531250086715715 ) ) ;
#23109=CARTESIAN_POINT ( 'NONE',  ( 95.00000000000000000, -207.3369185715606307, 81.86406250086714920 ) ) ;
#23114=ORIENTED_EDGE ( 'NONE', *, *, #49334, .F. ) ;
#23116=( BOUNDED_CURVE ( )  B_SPLINE_CURVE ( 2, ( #1169, #39876, #62820, #11284, #3000, #37563, #60496, #1900, #8616, #54466, #66136, #70630, #24785, #2270, #48823, #42090, #47716, #71740, #3365, #8230, #19145, #13505, #30780, #65029, #36431, #36800, #31902, #26256, #2644, #31162, #59376, #49194, #42456, #14614, #18768, #7864, #53725, #60134, #54839, #25894, #20243, #25166, #41705, #14237, #48092, #71006, #31527, #43214, #19509, #59747, #64644, #13861, #13129, #65394, #8976, #36067, #53359, #54112, #59011, #7504, #25523, #48457, #30414, #37191, #71369, #19876, #42824, #65753, #45054, #9337, #67981, #15347, #72848, #28118, #49932, #66502, #22115, #21347, #21735, #61977, #50300, #20631, #32638, #38291, #73235, #72121, #44692, #67607, #20991, #44306, #60858, #73605, #32263, #4852, #43945, #37927, #33373, #16100, #16475, #67238, #55211, #27365, #39412, #27753, #43585, #14983, #5217, #3730, #9719, #26632, #49562, #62357, #39038, #10458, #15734, #72491, #50678, #55583, #55955, #66861, #4102, #61238, #38670, #56334, #10840, #26997, #33761, #61600, #10086, #56718, #33007, #4471, #40898, #346, #63833, #17217, #1078, #57441, #23237, #704, #51418, #45433, #6674, #44889, #22874, #68362, #12307, #69453, #51797, #68734, #5587, #39787, #40152, #16857, #23598, #35245, #11206, #63105, #40516, #52160, #58176, #11935, #29221, #63460, #11563, #46165, #5958, #57080, #34498, #51053, #62738, #29580, #28866, #34133, #17584, #46527, #52525, #73978, #69097, #28482, #45809, #22493, #34882, #17953, #57815, #6321, #27232, #50164, #21606, #28353, #56196, #27985, #39283, #62215, #27624, #16343, #73843, #62598, #32874, #21224, #55825, #50547, #32512, #4342, #38908, #56583, #73099, #44556, #10702, #55457, #15227, #15967, #5085, #33631, #67477, #73473, #61844, #66741, #44175, #50921, #10328, #33246, #4718, #45304, #22358, #74221, #21982, #3973, #44927, #38538, #67851, #67101, #72720, #68222, #56948, #51290, #16723, #39659, #15607, #43821, #11079, #34001, #5457, #38157, #61099, #61475, #9597, #26870, #49800, #9956, #58792, #18193, #46038, #51669, #12547, #29825, #68966, #216, #35481, #52783, #40382, #12176, #18555, #6191, #53148, #69324, #35114, #6910, #17452, #34751, #1327, #35841, #24216, #23108, #47146, #41136, #17090, #63333, #11435, #23835, #70054, #34370, #41494, #64434, #28730, #57692, #46777 ),
 .UNSPECIFIED., .F., .F. ) 
 B_SPLINE_CURVE_WITH_KNOTS ( ( 3, 2, 2, 2, 2, 2, 2, 2, 2, 2, 2, 2, 2, 2, 2, 2, 2, 2, 2, 2, 2, 2, 2, 2, 2, 2, 2, 2, 2, 2, 2, 2, 2, 2, 2, 2, 2, 2, 2, 2, 2, 2, 2, 2, 2, 2, 2, 2, 2, 2, 2, 2, 2, 2, 2, 2, 2, 2, 2, 2, 2, 2, 2, 2, 2, 2, 2, 2, 2, 2, 2, 2, 2, 2, 2, 2, 2, 2, 2, 2, 2, 2, 2, 2, 2, 2, 2, 2, 2, 2, 2, 2, 2, 2, 2, 2, 2, 2, 2, 2, 2, 2, 2, 2, 2, 2, 2, 2, 2, 2, 2, 2, 2, 2, 2, 2, 2, 2, 2, 2, 2, 2, 2, 2, 2, 2, 2, 2, 2, 2, 2, 2, 2, 2, 2, 2, 2, 2, 2, 2, 2, 2, 2, 3 ),
 ( 0.000000000000000000, 0.007055764916269566256, 0.01411152983253913251, 0.02116729474880869877, 0.02822305966507826502, 0.03527882458134783822, 0.04233458949761739754, 0.04939035441388697073, 0.05644611933015653005, 0.06350188424642609630, 0.07055764916269567644, 0.07761341407896524269, 0.08466917899523479507, 0.09172494391150436133, 0.09878070882777394146, 0.1058364737440435077, 0.1128922386603130601, 0.1199480035765826264, 0.1270037684928521926, 0.1340595334091217727, 0.1411152983253913529, 0.1481710632416609053, 0.1552268281579304854, 0.1622825930742000100, 0.1693383579904695901, 0.1763941229067391703, 0.1834498878230087227, 0.1905056527392783028, 0.1975614176555478829, 0.2046171825718174353, 0.2116729474880870154, 0.2187287124043565678, 0.2257844773206261202, 0.2328402422368957003, 0.2398960071531652527, 0.2469517720694348328, 0.2540075369857043852, 0.2610633019019739653, 0.2681190668182435455, 0.2751748317345130701, 0.2822305966507827057, 0.2892863615670522304, 0.2963421264833218105, 0.3033978913995913906, 0.3104536563158609708, 0.3175094212321304954, 0.3245651861484000200, 0.3316209510646696557, 0.3386767159809391803, 0.3457324808972087604, 0.3527882458134783406, 0.3598440107297479207, 0.3668997756460174453, 0.3739555405622870810, 0.3810113054785566056, 0.3880670703948261302, 0.3951228353110957658, 0.4021786002273652905, 0.4092343651436348706, 0.4162901300599044507, 0.4233458949761740309, 0.4304016598924435555, 0.4374574248087131356, 0.4445131897249827158, 0.4515689546412522404, 0.4586247195575218205, 0.4656804844737914006, 0.4727362493900609808, 0.4797920143063305054, 0.4868477792226001410, 0.4939035441388696657, 0.5009593090551393013, 0.5080150739714087704, 0.5150708388876783506, 0.5221266038039479307, 0.5291823687202175108, 0.5362381336364870910, 0.5432938985527566711, 0.5503496634690261402, 0.5574054283852958314, 0.5644611933015654115, 0.5715169582178348806, 0.5785727231341044607, 0.5856284880503740409, 0.5926842529666436210, 0.5997400178829132011, 0.6067957827991827813, 0.6138515477154522504, 0.6209073126317219415, 0.6279630775479914107, 0.6350188424642609908, 0.6420746073805305709, 0.6491303722968000400, 0.6561861372130697312, 0.6632419021293393113, 0.6702976670456087804, 0.6773534319618783606, 0.6844091968781480517, 0.6914649617944175208, 0.6985207267106871010, 0.7055764916269566811, 0.7126322565432261502, 0.7196880214594958414, 0.7267437863757654215, 0.7337995512920348906, 0.7408553162083044707, 0.7479110811245741619, 0.7549668460408436310, 0.7620226109571132111, 0.7690783758733827913, 0.7761341407896522604, 0.7831899057059219516, 0.7902456706221915317, 0.7973014355384610008, 0.8043572004547305809, 0.8114129653710002721, 0.8184687302872697412, 0.8255244952035393213, 0.8325802601198089015, 0.8396360250360783706, 0.8466917899523480617, 0.8537475548686176419, 0.8608033197848871110, 0.8678590847011566911, 0.8749148496174262712, 0.8819706145336958514, 0.8890263794499654315, 0.8960821443662349006, 0.9031379092825044808, 0.9101936741987741719, 0.9172494391150436410, 0.9243052040313132212, 0.9313609689475828013, 0.9384167338638523814, 0.9454724987801219616, 0.9525282636963915417, 0.9595840286126610108, 0.9666397935289305909, 0.9736955584452002821, 0.9807513233614697512, 0.9878070882777393313, 0.9948628531940089115, 0.9999999123559573100, 1.000000000000000000 ),
 .UNSPECIFIED. ) 
 CURVE ( )  GEOMETRIC_REPRESENTATION_ITEM ( )  RATIONAL_B_SPLINE_CURVE ( ( 1.000000000000000000, 0.8660254037844387076, 1.000000000000000000, 0.8660254037844387076, 1.000000000000000000, 0.8660254037844387076, 1.000000000000000000, 0.8660254037844387076, 1.000000000000000000, 0.8660254037844387076, 1.000000000000000000, 0.8660254037844387076, 1.000000000000000000, 0.8660254037844387076, 1.000000000000000000, 0.8660254037844387076, 1.000000000000000000, 0.8660254037844387076, 1.000000000000000000, 0.8660254037844387076, 1.000000000000000000, 0.8660254037844387076, 1.000000000000000000, 0.8660254037844387076, 1.000000000000000000, 0.8660254037844387076, 1.000000000000000000, 0.8660254037844387076, 1.000000000000000000, 0.8660254037844387076, 1.000000000000000000, 0.8660254037844387076, 1.000000000000000000, 0.8660254037844387076, 1.000000000000000000, 0.8660254037844387076, 1.000000000000000000, 0.8660254037844387076, 1.000000000000000000, 0.8660254037844387076, 1.000000000000000000, 0.8660254037844387076, 1.000000000000000000, 0.8660254037844387076, 1.000000000000000000, 0.8660254037844387076, 1.000000000000000000, 0.8660254037844387076, 1.000000000000000000, 0.8660254037844387076, 1.000000000000000000, 0.8660254037844387076, 1.000000000000000000, 0.8660254037844387076, 1.000000000000000000, 0.8660254037844387076, 1.000000000000000000, 0.8660254037844387076, 1.000000000000000000, 0.8660254037844387076, 1.000000000000000000, 0.8660254037844387076, 1.000000000000000000, 0.8660254037844387076, 1.000000000000000000, 0.8660254037844387076, 1.000000000000000000, 0.8660254037844387076, 1.000000000000000000, 0.8660254037844387076, 1.000000000000000000, 0.8660254037844387076, 1.000000000000000000, 0.8660254037844387076, 1.000000000000000000, 0.8660254037844387076, 1.000000000000000000, 0.8660254037844387076, 1.000000000000000000, 0.8660254037844387076, 1.000000000000000000, 0.8660254037844387076, 1.000000000000000000, 0.8660254037844387076, 1.000000000000000000, 0.8660254037844387076, 1.000000000000000000, 0.8660254037844387076, 1.000000000000000000, 0.8660254037844387076, 1.000000000000000000, 0.8660254037844387076, 1.000000000000000000, 0.8660254037844387076, 1.000000000000000000, 0.8660254037844387076, 1.000000000000000000, 0.8660254037844387076, 1.000000000000000000, 0.8660254037844387076, 1.000000000000000000, 0.8660254037844387076, 1.000000000000000000, 0.8660254037844387076, 1.000000000000000000, 0.8660254037844387076, 1.000000000000000000, 0.8660254037844387076, 1.000000000000000000, 0.8660254037844387076, 1.000000000000000000, 0.8660254037844387076, 1.000000000000000000, 0.8660254037844387076, 1.000000000000000000, 0.8660254037844387076, 1.000000000000000000, 0.8660254037844387076, 1.000000000000000000, 0.8660254037844387076, 1.000000000000000000, 0.8660254037844387076, 1.000000000000000000, 0.8660254037844387076, 1.000000000000000000, 0.8660254037844387076, 1.000000000000000000, 0.8660254037844387076, 1.000000000000000000, 0.8660254037844387076, 1.000000000000000000, 0.8660254037844387076, 1.000000000000000000, 0.8660254037844387076, 1.000000000000000000, 0.8660254037844387076, 1.000000000000000000, 0.8660254037844387076, 1.000000000000000000, 0.8660254037844387076, 1.000000000000000000, 0.8660254037844387076, 1.000000000000000000, 0.8660254037844387076, 1.000000000000000000, 0.8660254037844387076, 1.000000000000000000, 0.8660254037844387076, 1.000000000000000000, 0.8660254037844387076, 1.000000000000000000, 0.8660254037844387076, 1.000000000000000000, 0.8660254037844387076, 1.000000000000000000, 0.8660254037844387076, 1.000000000000000000, 0.8660254037844387076, 1.000000000000000000, 0.8660254037844387076, 1.000000000000000000, 0.8660254037844387076, 1.000000000000000000, 0.8660254037844387076, 1.000000000000000000, 0.8660254037844387076, 1.000000000000000000, 0.8660254037844387076, 1.000000000000000000, 0.8660254037844387076, 1.000000000000000000, 0.8660254037844387076, 1.000000000000000000, 0.8660254037844387076, 1.000000000000000000, 0.8660254037844387076, 1.000000000000000000, 0.8660254037844387076, 1.000000000000000000, 0.8660254037844387076, 1.000000000000000000, 0.8660254037844387076, 1.000000000000000000, 0.8660254037844387076, 1.000000000000000000, 0.8660254037844387076, 1.000000000000000000, 0.8660254037844387076, 1.000000000000000000, 0.8660254037844387076, 1.000000000000000000, 0.8660254037844387076, 1.000000000000000000, 0.8660254037844387076, 1.000000000000000000, 0.8660254037844387076, 1.000000000000000000, 0.8660254037844387076, 1.000000000000000000, 0.8660254037844387076, 1.000000000000000000, 0.8660254037844387076, 1.000000000000000000, 0.8660254037844387076, 1.000000000000000000, 0.8660254037844387076, 1.000000000000000000, 0.8660254037844387076, 1.000000000000000000, 0.8660254037844387076, 1.000000000000000000, 0.8660254037844387076, 1.000000000000000000, 0.8660254037844387076, 1.000000000000000000, 0.8660254037844387076, 1.000000000000000000, 0.8660254037844387076, 1.000000000000000000, 0.8660254037844387076, 1.000000000000000000, 0.8660254037844387076, 1.000000000000000000, 0.8660254037844387076, 1.000000000000000000, 0.8660254037844387076, 1.000000000000000000, 0.8660254037844387076, 1.000000000000000000, 0.8660254037844387076, 1.000000000000000000, 0.8660254037844387076, 1.000000000000000000, 0.8660254037844387076, 1.000000000000000000, 0.8660254037844387076, 1.000000000000000000, 0.8660254037844387076, 1.000000000000000000, 0.8660254037844387076, 1.000000000000000000, 0.8660254037844387076, 1.000000000000000000, 0.8660254037844387076, 1.000000000000000000, 0.8660254037844387076, 1.000000000000000000, 0.8660254037844387076, 1.000000000000000000, 0.8660254037844387076, 1.000000000000000000, 0.8660254037844387076, 1.000000000000000000, 0.8660254037844387076, 1.000000000000000000, 0.8660254037844387076, 1.000000000000000000, 0.8660254037844387076, 1.000000000000000000, 0.8660254037844387076, 1.000000000000000000, 0.8660254037844387076, 1.000000000000000000, 0.8660254037844387076, 1.000000000000000000, 0.8660254037844387076, 1.000000000000000000, 0.8660254037844387076, 1.000000000000000000, 0.8660254037844387076, 1.000000000000000000, 0.8660254037844387076, 1.000000000000000000, 0.8660254037844387076, 1.000000000000000000, 0.8660254037844387076, 1.000000000000000000, 0.8660254037844387076, 1.000000000000000000, 0.8660254037844387076, 1.000000000000000000, 0.8660254037844387076, 1.000000000000000000, 0.9024577157650887083, 0.9469497795711399046, 0.9469497795711399046, 0.9469497795711399046 ) ) 
 REPRESENTATION_ITEM ( '' )  );
#23130=ORIENTED_EDGE ( 'NONE', *, *, #9865, .T. ) ;
#23131=CARTESIAN_POINT ( 'NONE',  ( 97.30629616937498838, 88.66845928578037217, 83.71614583420050337 ) ) ;
#23140=CARTESIAN_POINT ( 'NONE',  ( 92.34999999999995168, 91.52997821335250705, 84.23208333333334963 ) ) ;
#23145=DIRECTION ( 'NONE',  ( 1.000000000000000000, 0.000000000000000000, 0.000000000000000000 ) ) ;
#23147=CARTESIAN_POINT ( 'NONE',  ( -92.34999999999999432, -209.9999999999999716, 81.50687500173430067 ) ) ;
#23151=CARTESIAN_POINT ( 'NONE',  ( 97.64999999999997726, 88.47002178664753558, 77.64395833506762301 ) ) ;
#23152=CARTESIAN_POINT ( 'NONE',  ( -95.00000000000002842, 86.94004357329504273, 79.44312500173428759 ) ) ;
#23154=CARTESIAN_POINT ( 'NONE',  ( 97.30629616937498838, 91.33154071421968467, 80.01197916753380923 ) ) ;
#23158=CARTESIAN_POINT ( 'NONE',  ( 92.35000000006144205, 90.00001182123735077, 81.82400613091868991 ) ) ;
#23161=CARTESIAN_POINT ( 'NONE',  ( -97.64999999999994884, 91.52997821335257811, 80.42208333333330472 ) ) ;
#23169=DIRECTION ( 'NONE',  ( -1.000000000000000000, 0.000000000000000000, 0.000000000000000000 ) ) ;
#23170=CARTESIAN_POINT ( 'NONE',  ( -92.69370383062498320, -209.9999999999999716, 79.95906250086714806 ) ) ;
#23177=EDGE_CURVE ( 'NONE', #45415, #27271, #5851, .T. ) ;
#23187=CARTESIAN_POINT ( 'NONE',  ( 97.30629616937498838, 88.66845928578035796, 88.16114583420048234 ) ) ;
#23191=CARTESIAN_POINT ( 'NONE',  ( -92.35000000000003695, 90.00000000000004263, 78.25249999999999773 ) ) ;
#23192=CARTESIAN_POINT ( 'NONE',  ( -92.69370383062505425, 91.33154071421968467, 80.48822916753380241 ) ) ;
#23198=FACE_OUTER_BOUND ( 'NONE', #24666, .T. ) ;
#23201=CARTESIAN_POINT ( 'NONE',  ( 96.32499999999998863, -212.2949673200287179, 85.84604166840097150 ) ) ;
#23204=CARTESIAN_POINT ( 'NONE',  ( 92.69370383062501162, -208.6684592857803011, 75.77864583420048916 ) ) ;
#23207=ORIENTED_EDGE ( 'NONE', *, *, #58810, .T. ) ;
#23209=CARTESIAN_POINT ( 'NONE',  ( 95.00000000000000000, -207.3369185715606307, 80.75281250086716511 ) ) ;
#23214=CARTESIAN_POINT ( 'NONE',  ( -97.64999999953586496, -210.0000309672219601, 77.38038495123339544 ) ) ;
#23215=CARTESIAN_POINT ( 'NONE',  ( 92.34999999999999432, 89.99996406046703612, 83.72937624475873974 ) ) ;
#23218=CARTESIAN_POINT ( 'NONE',  ( 97.64999999999997726, -208.4700217866474645, 87.19541666666667368 ) ) ;
#23219=ORIENTED_EDGE ( 'NONE', *, *, #24676, .F. ) ;
#23224=VERTEX_POINT ( 'NONE', #6224 ) ;
#23226=VECTOR ( 'NONE', #29531, 1000.000000000000000 ) ;
#23227=CARTESIAN_POINT ( 'NONE',  ( -92.69370383062504004, 90.00000000000004263, 86.30906250086715659 ) ) ;
#23229=CARTESIAN_POINT ( 'NONE',  ( 96.32499999999998863, -207.7050326799711968, 77.80270833506763495 ) ) ;
#23230=CARTESIAN_POINT ( 'NONE',  ( 92.34999999999999432, 91.52997821335252127, 79.78708333333332803 ) ) ;
#23231=ORIENTED_EDGE ( 'NONE', *, *, #37192, .F. ) ;
#23236=CARTESIAN_POINT ( 'NONE',  ( 93.67500000000001137, -212.2949673200287179, 88.28020833506764120 ) ) ;
#23237=CARTESIAN_POINT ( 'NONE',  ( -92.69370383062504004, 90.00000000000004263, 82.49906250086715431 ) ) ;
#23238=CARTESIAN_POINT ( 'NONE',  ( 92.69370383062498320, 88.66845928578037217, 89.21947916753381946 ) ) ;
#23246=CARTESIAN_POINT ( 'NONE',  ( -94.99999999999997158, -212.6630814284392557, 77.73656250086713726 ) ) ;
#23248=EDGE_LOOP ( 'NONE', ( #44367, #47919, #20320, #3890 ) ) ;
#23254=CARTESIAN_POINT ( 'NONE',  ( -92.69370383062498320, -208.6684592857803011, 77.31322916753380525 ) ) ;
#23258=CARTESIAN_POINT ( 'NONE',  ( 92.34999999999999432, -208.4700217866474645, 81.69208333333332916 ) ) ;
#23265=CARTESIAN_POINT ( 'NONE',  ( 97.64999999999999147, -210.0000000198592716, 85.95187500101400246 ) ) ;
#23266=CARTESIAN_POINT ( 'NONE',  ( 97.30629616937498838, 91.33154071421968467, 83.66322916753381378 ) ) ;
#23268=CARTESIAN_POINT ( 'NONE',  ( -97.65000000000007674, 88.47002178664759242, 88.14791666666667425 ) ) ;
#23269=FACE_OUTER_BOUND ( 'NONE', #62047, .T. ) ;
#23284=CARTESIAN_POINT ( 'NONE',  ( -26.50044424985255276, 0.001194404164626844313, -64.00000000000000000 ) ) ;
#23285=EDGE_CURVE ( 'NONE', #47150, #64948, #15376, .T. ) ;
#23294=CARTESIAN_POINT ( 'NONE',  ( 92.69370383062501162, -208.6684592857803011, 84.66864583420047552 ) ) ;
#23295=ORIENTED_EDGE ( 'NONE', *, *, #67253, .F. ) ;
#23297=CARTESIAN_POINT ( 'NONE',  ( -94.99999999999997158, -206.9400435732949575, 86.03125000000000000 ) ) ;
#23298=VERTEX_POINT ( 'NONE', #65581 ) ;
#23300=CARTESIAN_POINT ( 'NONE',  ( -97.64999999978461176, -209.9999789922612479, 79.91868729551984529 ) ) ;
#23301=DIRECTION ( 'NONE',  ( -0.000000000000000000, -0.000000000000000000, 1.000000000000000000 ) ) ;
#23302=ORIENTED_EDGE ( 'NONE', *, *, #51264, .F. ) ;
#23303=CARTESIAN_POINT ( 'NONE',  ( 93.84685191531249870, -208.0026889286704943, 82.07572916753382231 ) ) ;
#23305=CARTESIAN_POINT ( 'NONE',  ( -97.65000000000003411, -211.5299782133523934, 88.14791666666667425 ) ) ;
#23311=CARTESIAN_POINT ( 'NONE',  ( -94.99999999999997158, -209.9999999999999716, 90.00000000000000000 ) ) ;
#23313=CARTESIAN_POINT ( 'NONE',  ( -93.67500000000003979, 87.70503267997129626, 77.51166666666665606 ) ) ;
#23314=CARTESIAN_POINT ( 'NONE',  ( 95.00000000000000000, -206.9400435732949575, 86.11062500173430578 ) ) ;
#23318=( BOUNDED_CURVE ( )  B_SPLINE_CURVE ( 2, ( #55774, #166, #51613, #32823, #61795, #39231, #11025, #73422, #45987 ),
 .UNSPECIFIED., .F., .F. ) 
 B_SPLINE_CURVE_WITH_KNOTS ( ( 3, 2, 2, 2, 3 ),
 ( 0.2751748541904413536, 0.2822306216352944985, 0.2892863871761765515, 0.2963421527170586600, 0.2963422021981248489 ),
 .UNSPECIFIED. ) 
 CURVE ( )  GEOMETRIC_REPRESENTATION_ITEM ( )  RATIONAL_B_SPLINE_CURVE ( ( 1.000000000000000000, 0.8660254037844387076, 1.000000000000000000, 0.8660254037844387076, 1.000000000000000000, 0.8660254037844387076, 1.000000000000000000, 0.9999990604554780393, 0.9999981209241337599 ) ) 
 REPRESENTATION_ITEM ( '' )  );
#23324=CARTESIAN_POINT ( 'NONE',  ( -97.64998927314393029, -211.5299844065056334, 78.06729209680057124 ) ) ;
#23334=CARTESIAN_POINT ( 'NONE',  ( -93.67500000000003979, 87.70503267997129626, 88.94166666666666288 ) ) ;
#23336=CARTESIAN_POINT ( 'NONE',  ( 96.15314808468748708, 88.00268892867053694, 75.88447916753381151 ) ) ;
#23340=( BOUNDED_CURVE ( )  B_SPLINE_CURVE ( 2, ( #6428, #51904, #23344, #46271, #17694, #40631, #29328, #52272, #815 ),
 .UNSPECIFIED., .F., .F. ) 
 B_SPLINE_CURVE_WITH_KNOTS ( ( 3, 2, 2, 2, 3 ),
 ( 0.6561861948943049638, 0.6632419608461993521, 0.6702977263871157110, 0.6773534919280320699, 0.6773535682785479795 ),
 .UNSPECIFIED. ) 
 CURVE ( )  GEOMETRIC_REPRESENTATION_ITEM ( )  RATIONAL_B_SPLINE_CURVE ( ( 1.000000000000000000, 0.8660254037844387076, 1.000000000000000000, 0.8660254037844387076, 1.000000000000000000, 0.8660254037844387076, 1.000000000000000000, 0.9999985502594314069, 0.9999971005502381605 ) ) 
 REPRESENTATION_ITEM ( '' )  );
#23342=CARTESIAN_POINT ( 'NONE',  ( -96.15314808468747287, -208.0026889286704943, 86.36197916753381776 ) ) ;
#23344=CARTESIAN_POINT ( 'NONE',  ( -93.67499999999998295, -212.2949673200287179, 79.49604166840096298 ) ) ;
#23347=CARTESIAN_POINT ( 'NONE',  ( -92.69370383062498320, -208.6684592857803295, 76.04322916753380923 ) ) ;
#23354=CARTESIAN_POINT ( 'NONE',  ( -92.35000000000003695, 90.00000000000004263, 90.00000000000000000 ) ) ;
#23356=CARTESIAN_POINT ( 'NONE',  ( -97.30629616937501680, 90.00000000000004263, 76.94281250086713442 ) ) ;
#23369=CARTESIAN_POINT ( 'NONE',  ( -97.30629616937497417, -211.3315407142195852, 76.51947916753381662 ) ) ;
#23386=ORIENTED_EDGE ( 'NONE', *, *, #32057, .T. ) ;
#23388=CARTESIAN_POINT ( 'NONE',  ( 95.00000000000000000, -212.6630814284392557, 85.35656250086714181 ) ) ;
#23396=CARTESIAN_POINT ( 'NONE',  ( -97.30629616937501680, 90.00000000000004263, 82.18156250086715886 ) ) ;
#23397=ORIENTED_EDGE ( 'NONE', *, *, #33273, .T. ) ;
#23398=DIRECTION ( 'NONE',  ( 1.000000000000000000, 0.000000000000000000, 0.000000000000000000 ) ) ;
#23400=VERTEX_POINT ( 'NONE', #46406 ) ;
#23401=DIRECTION ( 'NONE',  ( -1.000000000000000000, 0.000000000000000000, 0.000000000000000000 ) ) ;
#23405=CARTESIAN_POINT ( 'NONE',  ( 97.65000000000000568, -211.5299782133524218, 80.81895833506763438 ) ) ;
#23408=CARTESIAN_POINT ( 'NONE',  ( 92.69370383062498320, 88.66845928578037217, 86.52072916753381548 ) ) ;
#23410=CARTESIAN_POINT ( 'NONE',  ( 97.30629616937498838, -211.3315407142195852, 82.92239583420045790 ) ) ;
#23413=CARTESIAN_POINT ( 'NONE',  ( -97.64999999947046661, -209.9999663481462164, 81.18829462297327382 ) ) ;
#23414=CARTESIAN_POINT ( 'NONE',  ( -93.09170270117142820, -211.8387227684682159, 74.99954709728268654 ) ) ;
#23415=CARTESIAN_POINT ( 'NONE',  ( 94.99999999999998579, 86.94004357329502852, 85.07875000000001364 ) ) ;
#23417=ADVANCED_FACE ( 'NONE', ( #34006 ), #46045, .F. ) ;
#23418=CARTESIAN_POINT ( 'NONE',  ( -95.00000000000002842, 86.94004357329504273, 79.36374999999996760 ) ) ;
#23419=CARTESIAN_POINT ( 'NONE',  ( -92.69370383062498320, -209.9999999999999716, 83.61031250086713840 ) ) ;
#23420=EDGE_CURVE ( 'NONE', #29989, #68978, #6213, .T. ) ;
#23421=CARTESIAN_POINT ( 'NONE',  ( -97.30629616937501680, 90.00000000000004263, 81.54656250086715374 ) ) ;
#23423=CARTESIAN_POINT ( 'NONE',  ( 93.84685191531248449, 91.99731107132950569, 85.09197916753380753 ) ) ;
#23431=CARTESIAN_POINT ( 'NONE',  ( -93.84685191531248449, -208.0026889286704943, 87.52614583420047722 ) ) ;
#23440=ORIENTED_EDGE ( 'NONE', *, *, #4280, .F. ) ;
#23442=CARTESIAN_POINT ( 'NONE',  ( -92.35000000000003695, 90.00000000000004263, 78.88750000000000284 ) ) ;
#23443=CARTESIAN_POINT ( 'NONE',  ( 92.35000000000000853, -209.9999999999999716, 88.73000000000000398 ) ) ;
#23444=CARTESIAN_POINT ( 'NONE',  ( 92.35000000000000853, -209.9999999999999716, 81.10999999999999943 ) ) ;
#23450=CARTESIAN_POINT ( 'NONE',  ( -97.30629616937501680, 91.33154071421968467, 79.42989583420046529 ) ) ;
#23456=CARTESIAN_POINT ( 'NONE',  ( -97.30629616937495996, -209.9999999999999716, 86.62656250086715204 ) ) ;
#23460=CARTESIAN_POINT ( 'NONE',  ( 94.99999999999998579, 87.33691857156068750, 76.62531250086715318 ) ) ;
#23461=CARTESIAN_POINT ( 'NONE',  ( -92.69370383062498320, -209.9999999999999716, 78.68906250086715204 ) ) ;
#23469=CARTESIAN_POINT ( 'NONE',  ( 95.00000000000000000, -207.3369185715606307, 78.05406250086714692 ) ) ;
#23470=VERTEX_POINT ( 'NONE', #5828 ) ;
#23471=CARTESIAN_POINT ( 'NONE',  ( -92.34999999999998010, 91.52997821335249284, 75.13041666666666174 ) ) ;
#23486=CARTESIAN_POINT ( 'NONE',  ( 92.69370383062498320, 91.33154071421968467, 83.39864583420050792 ) ) ;
#23487=CARTESIAN_POINT ( 'NONE',  ( 95.00000000000000000, -213.0599564267049857, 75.55375000000000796 ) ) ;
#23490=ADVANCED_FACE ( 'NONE', ( #51674 ), #222, .F. ) ;
#23493=DIRECTION ( 'NONE',  ( -2.628368902995175337E-16, -1.000000000000000000, 0.000000000000000000 ) ) ;
#23498=DIRECTION ( 'NONE',  ( -0.000000000000000000, -0.000000000000000000, 1.000000000000000000 ) ) ;
#23503=CARTESIAN_POINT ( 'NONE',  ( -97.64999999999994884, -211.5299782133524502, 78.70229166840096013 ) ) ;
#23504=ORIENTED_EDGE ( 'NONE', *, *, #49900, .T. ) ;
#23507=ORIENTED_EDGE ( 'NONE', *, *, #21266, .F. ) ;
#23508=CARTESIAN_POINT ( 'NONE',  ( 97.64999999999997726, 88.47002178664753558, 80.18395833506764347 ) ) ;
#23509=CARTESIAN_POINT ( 'NONE',  ( -97.65000000000001990, 91.52997821335253548, 79.23145833506762870 ) ) ;
#23511=CARTESIAN_POINT ( 'NONE',  ( 94.99999999999998579, 87.33691857156068750, 79.16531250086715943 ) ) ;
#23512=CARTESIAN_POINT ( 'NONE',  ( -94.99999999999997158, -206.9400435732949575, 82.22124999999999773 ) ) ;
#23514=CARTESIAN_POINT ( 'NONE',  ( 93.67500000000001137, -212.2949673200287179, 79.39020833506762642 ) ) ;
#23516=EDGE_CURVE ( 'NONE', #33091, #2294, #70419, .T. ) ;
#23519=CARTESIAN_POINT ( 'NONE',  ( 96.32499999999998863, -207.7050326799711968, 77.08833333333332405 ) ) ;
#23520=CARTESIAN_POINT ( 'NONE',  ( -92.35000000000179909, 90.00000306648279036, 75.79187510780352000 ) ) ;
#23526=CARTESIAN_POINT ( 'NONE',  ( -93.33864827736697123, -211.6008015735577033, 74.79754476654878204 ) ) ;
#23527=CARTESIAN_POINT ( 'NONE',  ( -94.99999999999997158, -212.6630814284392557, 77.26031250086714408 ) ) ;
#23536=CARTESIAN_POINT ( 'NONE',  ( 96.73972734126400042, 91.51405112163766375, 74.79348190356853365 ) ) ;
#23543=CARTESIAN_POINT ( 'NONE',  ( 92.35000000052950497, -209.9999663481461027, 81.18829462297289012 ) ) ;
#23544=EDGE_CURVE ( 'NONE', #43675, #71815, #36333, .T. ) ;
#23547=( BOUNDED_CURVE ( )  B_SPLINE_CURVE ( 2, ( #29411, #46361, #52359, #11039, #35077, #17414, #23792 ),
 .UNSPECIFIED., .F., .F. ) 
 B_SPLINE_CURVE_WITH_KNOTS ( ( 3, 2, 2, 3 ),
 ( 0.2916666666666669072, 0.2986111111111113270, 0.3055555555555557468, 0.3125000000000001665 ),
 .UNSPECIFIED. ) 
 CURVE ( )  GEOMETRIC_REPRESENTATION_ITEM ( )  RATIONAL_B_SPLINE_CURVE ( ( 0.9999999999999956701, 0.8660254037844430375, 1.000000000000000000, 0.8660254037844387076, 1.000000000000000000, 0.8660254037844354880, 1.000000000000003109 ) ) 
 REPRESENTATION_ITEM ( '' )  );
#23548=CARTESIAN_POINT ( 'NONE',  ( 96.15314808468748708, 88.00268892867053694, 88.74322916753382628 ) ) ;
#23553=CARTESIAN_POINT ( 'NONE',  ( -92.69370383062505425, 91.33154071421968467, 79.21822916753380639 ) ) ;
#23554=VECTOR ( 'NONE', #28264, 1000.000000000000000 ) ;
#23555=CARTESIAN_POINT ( 'NONE',  ( 96.15314808468748708, -208.0026889286704943, 88.16114583420046813 ) ) ;
#23557=CARTESIAN_POINT ( 'NONE',  ( 97.65000000000000568, -211.5299782133524218, 80.18395833506764347 ) ) ;
#23565=CARTESIAN_POINT ( 'NONE',  ( 97.30629616937498838, -209.9999999999999716, 81.22906250086715829 ) ) ;
#23572=CARTESIAN_POINT ( 'NONE',  ( 92.35000000000002274, -208.4700217866474645, 84.86708333333334053 ) ) ;
#23574=VERTEX_POINT ( 'NONE', #70801 ) ;
#23580=CARTESIAN_POINT ( 'NONE',  ( -93.84685191531254134, 91.99731107132950569, 85.77989583420048803 ) ) ;
#23586=CARTESIAN_POINT ( 'NONE',  ( 93.67500000000001137, -212.2949673200287179, 76.21520833506762926 ) ) ;
#23588=CARTESIAN_POINT ( 'NONE',  ( 93.67499999999999716, 87.70503267997126784, 78.04083333333333883 ) ) ;
#23590=CARTESIAN_POINT ( 'NONE',  ( -92.34999999999999432, -211.5299782133524502, 89.07395833506762983 ) ) ;
#23596=CARTESIAN_POINT ( 'NONE',  ( -96.32500000000001705, 92.29496732002878900, 88.06854166840095388 ) ) ;
#23598=CARTESIAN_POINT ( 'NONE',  ( -96.15314808468751551, 88.00268892867056536, 81.65239583420049030 ) ) ;
#23599=CARTESIAN_POINT ( 'NONE',  ( 97.30629616937498838, 90.00000000000002842, 88.84906250086716284 ) ) ;
#23601=CARTESIAN_POINT ( 'NONE',  ( -92.34999999999999432, -209.9999999999999716, 84.60249999999999204 ) ) ;
#23608=CARTESIAN_POINT ( 'NONE',  ( -97.30629616937497417, -211.3315407142195852, 78.26572916753380582 ) ) ;
#23612=CARTESIAN_POINT ( 'NONE',  ( 97.64999999999999147, 90.00002660292301471, 78.96687592183759818 ) ) ;
#23617=CARTESIAN_POINT ( 'NONE',  ( -92.69370383062498320, -211.3315407142195852, 89.43114583420049257 ) ) ;
#23628=CARTESIAN_POINT ( 'NONE',  ( 97.30629616937498838, 91.33154071421968467, 84.29822916753380468 ) ) ;
#23631=DIRECTION ( 'NONE',  ( -0.000000000000000000, -0.000000000000000000, 1.000000000000000000 ) ) ;
#23634=CARTESIAN_POINT ( 'NONE',  ( 92.35000000000000853, -211.5299782133524218, 87.59229166840096070 ) ) ;
#23638=CARTESIAN_POINT ( 'NONE',  ( -92.34999999999999432, -209.9999999999999716, 85.23749999999999716 ) ) ;
#23647=LINE ( 'NONE', #36767, #7185 ) ;
#23651=CARTESIAN_POINT ( 'NONE',  ( 92.69370383062501162, -211.3315407142195852, 85.40947916753380298 ) ) ;
#23657=CARTESIAN_POINT ( 'NONE',  ( 96.32499999999998863, -207.7050326799711968, 88.51833333333333087 ) ) ;
#23658=LINE ( 'NONE', #29287, #42413 ) ;
#23659=VERTEX_POINT ( 'NONE', #3884 ) ;
#23660=CARTESIAN_POINT ( 'NONE',  ( 97.30629616937498838, -208.6684592857803011, 78.74197916753382742 ) ) ;
#23661=EDGE_LOOP ( 'NONE', ( #61330, #46600, #66400, #71545 ) ) ;
#23666=CARTESIAN_POINT ( 'NONE',  ( 2.500000000000034639, 90.00000000000000000, -310.0000000000000000 ) ) ;
#23668=( LENGTH_UNIT ( ) NAMED_UNIT ( * ) SI_UNIT ( .MILLI., .METRE. ) );
#23670=ORIENTED_EDGE ( 'NONE', *, *, #14406, .F. ) ;
#23672=CARTESIAN_POINT ( 'NONE',  ( 96.32499999999998863, -207.7050326799711968, 86.05770833506763040 ) ) ;
#23675=VERTEX_POINT ( 'NONE', #31688 ) ;
#23680=ORIENTED_EDGE ( 'NONE', *, *, #26501, .F. ) ;
#23682=CARTESIAN_POINT ( 'NONE',  ( 96.32499999999998863, 87.70503267997126784, 84.57604166840096127 ) ) ;
#23688=VERTEX_POINT ( 'NONE', #4254 ) ;
#23692=CARTESIAN_POINT ( 'NONE',  ( 93.67499999999998295, 92.29496732002878900, 79.81354166840095843 ) ) ;
#23693=CARTESIAN_POINT ( 'NONE',  ( 94.99999999999998579, 90.00000000000002842, 90.00000000000000000 ) ) ;
#23694=EDGE_CURVE ( 'NONE', #6687, #21322, #37356, .T. ) ;
#23695=CARTESIAN_POINT ( 'NONE',  ( -92.35000000000003695, 90.00000000000004263, 87.77749999999998920 ) ) ;
#23697=CARTESIAN_POINT ( 'NONE',  ( -97.64999999999996305, -209.9999999999999716, 90.00000000000000000 ) ) ;
#23700=CARTESIAN_POINT ( 'NONE',  ( -93.84685191531247028, -211.9973110713294489, 84.13947916753380696 ) ) ;
#23705=CARTESIAN_POINT ( 'NONE',  ( -93.26027265873587169, -208.4859488783624215, 74.79348190356851944 ) ) ;
#23716=CARTESIAN_POINT ( 'NONE',  ( -95.00000000000002842, 92.66308142843932671, 76.78406250086712248 ) ) ;
#23725=CYLINDRICAL_SURFACE ( 'NONE', #36392, 12.75000000000000000 ) ;
#23726=CARTESIAN_POINT ( 'NONE',  ( -97.30629616937497417, -208.6684592857803011, 77.04864583420048518 ) ) ;
#23740=VERTEX_POINT ( 'NONE', #43734 ) ;
#23741=( BOUNDED_CURVE ( )  B_SPLINE_CURVE ( 2, ( #64805, #23103, #58407, #68963, #41487, #17448, #57686, #6188, #14759 ),
 .UNSPECIFIED., .F., .F. ) 
 B_SPLINE_CURVE_WITH_KNOTS ( ( 3, 2, 2, 2, 3 ),
 ( 0.1058364832022827134, 0.1128922486541179548, 0.1199480141950002993, 0.1270037797358826437, 0.1270039290051391268 ),
 .UNSPECIFIED. ) 
 CURVE ( )  GEOMETRIC_REPRESENTATION_ITEM ( )  RATIONAL_B_SPLINE_CURVE ( ( 1.000000000000000000, 0.8660254037844387076, 1.000000000000000000, 0.8660254037844387076, 1.000000000000000000, 0.8660254037844387076, 1.000000000000000000, 0.9999971656812787213, 0.9999943314824810692 ) ) 
 REPRESENTATION_ITEM ( '' )  );
#23742=CARTESIAN_POINT ( 'NONE',  ( 96.15314808468750130, -211.9973110713294489, 85.40947916753380298 ) ) ;
#23751=CARTESIAN_POINT ( 'NONE',  ( -92.69370383062502583, 88.66845928578038638, 80.54114583420049200 ) ) ;
#23755=ORIENTED_EDGE ( 'NONE', *, *, #44211, .T. ) ;
#23757=VECTOR ( 'NONE', #21233, 1000.000000000000000 ) ;
#23759=LINE ( 'NONE', #13578, #44939 ) ;
#23761=AXIS2_PLACEMENT_3D ( 'NONE', #33138, #4603, #48947 ) ;
#23768=( BOUNDED_CURVE ( )  B_SPLINE_CURVE ( 2, ( #19254, #37671, #42205, #65140, #13613, #42566, #10191 ),
 .UNSPECIFIED., .F., .F. ) 
 B_SPLINE_CURVE_WITH_KNOTS ( ( 3, 2, 2, 3 ),
 ( 0.7831899741065913023, 0.7902457405788253508, 0.7973015061197076259, 0.8043570860654228882 ),
 .UNSPECIFIED. ) 
 CURVE ( )  GEOMETRIC_REPRESENTATION_ITEM ( )  RATIONAL_B_SPLINE_CURVE ( ( 1.000000000000000000, 0.8660254037844387076, 1.000000000000000000, 0.8660254037844387076, 1.000000000000000000, 0.8660289278581101424, 0.9999929520380519410 ) ) 
 REPRESENTATION_ITEM ( '' )  );
#23769=CARTESIAN_POINT ( 'NONE',  ( 95.00000000000000000, -213.0599564267049857, 80.71312500173429783 ) ) ;
#23771=VERTEX_POINT ( 'NONE', #61390 ) ;
#23774=CARTESIAN_POINT ( 'NONE',  ( 97.30629616937498838, -211.3315407142195852, 82.28739583420048120 ) ) ;
#23777=DIRECTION ( 'NONE',  ( -0.000000000000000000, -0.000000000000000000, 1.000000000000000000 ) ) ;
#23781=CARTESIAN_POINT ( 'NONE',  ( -97.65000000000001990, 90.00000000000004263, 82.37999999999999545 ) ) ;
#23782=CARTESIAN_POINT ( 'NONE',  ( -94.99999999999997158, -212.6630814284392557, 85.35656250086714181 ) ) ;
#23784=CARTESIAN_POINT ( 'NONE',  ( -97.30629616937501680, 90.00000000000004263, 80.91156250086716284 ) ) ;
#23787=CARTESIAN_POINT ( 'NONE',  ( 92.69370383062498320, 88.66845928578037217, 84.61572916753380014 ) ) ;
#23792=CARTESIAN_POINT ( 'NONE',  ( 97.64999999999999147, -209.9999999999999716, 85.23749999999999716 ) ) ;
#23793=CARTESIAN_POINT ( 'NONE',  ( -97.30629616937497417, -211.3315407142195852, 85.25072916753379104 ) ) ;
#23804=CARTESIAN_POINT ( 'NONE',  ( -92.35000000000005116, 91.52997821335253548, 77.03541666666666288 ) ) ;
#23806=CARTESIAN_POINT ( 'NONE',  ( -97.30629616937501680, 90.00000000000004263, 87.10281250086714522 ) ) ;
#23812=CARTESIAN_POINT ( 'NONE',  ( -97.30629616937501680, 90.00000000000004263, 80.11781250086713158 ) ) ;
#23820=CARTESIAN_POINT ( 'NONE',  ( -96.15314808468745866, -211.9973110713294489, 84.82739583420048746 ) ) ;
#23826=CARTESIAN_POINT ( 'NONE',  ( 92.69370383062498320, 88.66845928578035796, 77.78947916753381264 ) ) ;
#23828=CARTESIAN_POINT ( 'NONE',  ( -94.99999999999997158, -207.3369185715606307, 76.30781250086715772 ) ) ;
#23834=EDGE_CURVE ( 'NONE', #50224, #5801, #13860, .T. ) ;
#23835=CARTESIAN_POINT ( 'NONE',  ( -95.00000000000002842, 92.66308142843932671, 75.03781250086714749 ) ) ;
#23836=CARTESIAN_POINT ( 'NONE',  ( 96.15314808468750130, -211.9973110713294489, 77.15447916753380753 ) ) ;
#23842=DIRECTION ( 'NONE',  ( -2.628368902995175337E-16, -1.000000000000000000, 0.000000000000000000 ) ) ;
#23849=ORIENTED_EDGE ( 'NONE', *, *, #26845, .T. ) ;
#23855=CARTESIAN_POINT ( 'NONE',  ( 97.30629616937498838, 88.66845928578037217, 84.35114583420049428 ) ) ;
#23868=CARTESIAN_POINT ( 'NONE',  ( -92.34999999999995168, -208.4700217866474929, 85.29041666666665833 ) ) ;
#23877=CARTESIAN_POINT ( 'NONE',  ( -92.34999999999999432, -208.4700217866474645, 77.74979166840097378 ) ) ;
#23883=CARTESIAN_POINT ( 'NONE',  ( 97.64999999999999147, 90.00000000000002842, 80.87187500173430976 ) ) ;
#23884=CARTESIAN_POINT ( 'NONE',  ( -92.35000000000003695, 90.00000000000004263, 80.87187500173430976 ) ) ;
#23887=EDGE_CURVE ( 'NONE', #6682, #65091, #23658, .T. ) ;
#23888=CARTESIAN_POINT ( 'NONE',  ( 93.84685191531248449, 91.99731107132950569, 81.44072916753381719 ) ) ;
#23896=ORIENTED_EDGE ( 'NONE', *, *, #10535, .T. ) ;
#23900=CARTESIAN_POINT ( 'NONE',  ( -93.25528180581923721, -211.6811075874705352, 74.86350982016035971 ) ) ;
#23901=CARTESIAN_POINT ( 'NONE',  ( -97.30629616937497417, -208.6684592857803011, 78.31864583420050963 ) ) ;
#23908=CARTESIAN_POINT ( 'NONE',  ( 97.64999999999999147, 89.99999998014077107, 85.95187500101400246 ) ) ;
#23914=CARTESIAN_POINT ( 'NONE',  ( 93.67499999999998295, 92.29496732002878900, 86.16354166840096696 ) ) ;
#23917=CARTESIAN_POINT ( 'NONE',  ( 92.69370383062498320, 88.66845928578035796, 87.31447916753381833 ) ) ;
#23919=CARTESIAN_POINT ( 'NONE',  ( -92.69370383062498320, -211.3315407142195852, 85.62114583420047609 ) ) ;
#23923=EDGE_CURVE ( 'NONE', #1787, #41677, #30395, .T. ) ;
#23925=CARTESIAN_POINT ( 'NONE',  ( -94.99999999999997158, -213.0599564267049857, 80.63375000000000625 ) ) ;
#23928=AXIS2_PLACEMENT_3D ( 'NONE', #15279, #38593, #32929 ) ;
#23931=CARTESIAN_POINT ( 'NONE',  ( 96.15314808468748708, -208.0026889286704943, 86.25614583420048120 ) ) ;
#23942=CARTESIAN_POINT ( 'NONE',  ( 92.69370383062501162, -208.6684592857803295, 82.76364583420048859 ) ) ;
#23948=ADVANCED_FACE ( 'NONE', ( #37540 ), #59726, .F. ) ;
#23950=CARTESIAN_POINT ( 'NONE',  ( 97.64999999999999147, -209.9999999999999716, 85.23749999999999716 ) ) ;
#23960=CARTESIAN_POINT ( 'NONE',  ( -97.30629616937501680, 88.66845928578038638, 86.67947916753382742 ) ) ;
#23964=CARTESIAN_POINT ( 'NONE',  ( 95.00000000000000000, -207.3369185715606307, 88.21406250086714351 ) ) ;
#23965=CARTESIAN_POINT ( 'NONE',  ( 97.64999999999997726, 91.52997821335252127, 79.57541666666665492 ) ) ;
#23968=VERTEX_POINT ( 'NONE', #60111 ) ;
#23972=ORIENTED_EDGE ( 'NONE', *, *, #17167, .F. ) ;
#23973=CARTESIAN_POINT ( 'NONE',  ( -97.65000000000001990, 91.52997821335253548, 88.12145833506762926 ) ) ;
#23974=CARTESIAN_POINT ( 'NONE',  ( 92.69370383062498320, 91.33154071421968467, 76.25489583420049655 ) ) ;
#23975=EDGE_LOOP ( 'NONE', ( #678, #256, #4406, #4352 ) ) ;
#23977=FACE_OUTER_BOUND ( 'NONE', #24947, .T. ) ;
#23979=CYLINDRICAL_SURFACE ( 'NONE', #47385, 2.649999999999985700 ) ;
#23994=ORIENTED_EDGE ( 'NONE', *, *, #8345, .T. ) ;
#23995=( BOUNDED_CURVE ( )  B_SPLINE_CURVE ( 2, ( #49919, #21336, #44293, #42814, #48812, #55940, #49552, #14973, #61224 ),
 .UNSPECIFIED., .F., .F. ) 
 B_SPLINE_CURVE_WITH_KNOTS ( ( 3, 2, 2, 2, 3 ),
 ( 0.000000000000000000, 0.007055765540882369576, 0.01411153108176473915, 0.02116729662264710959, 0.02116741234826251261 ),
 .UNSPECIFIED. ) 
 CURVE ( )  GEOMETRIC_REPRESENTATION_ITEM ( )  RATIONAL_B_SPLINE_CURVE ( ( 1.000000000000000000, 0.8660254037844387076, 1.000000000000000000, 0.8660254037844387076, 1.000000000000000000, 0.8660254037844387076, 1.000000000000000000, 0.9999978026066050907, 0.9999956052852916333 ) ) 
 REPRESENTATION_ITEM ( '' )  );
#23996=CARTESIAN_POINT ( 'NONE',  ( -92.69370383062498320, -208.6684592857803011, 88.90197916753382401 ) ) ;
#24004=CARTESIAN_POINT ( 'NONE',  ( 94.99999999999998579, 87.33691857156068750, 82.18156250086715886 ) ) ;
#24010=CARTESIAN_POINT ( 'NONE',  ( 92.35000000000000853, -209.9999999999999716, 90.00000000000000000 ) ) ;
#24018=CARTESIAN_POINT ( 'NONE',  ( -95.00000000000002842, 92.66308142843932671, 86.94406250086714749 ) ) ;
#24022=EDGE_CURVE ( 'NONE', #54357, #62567, #31136, .T. ) ;
#24028=CARTESIAN_POINT ( 'NONE',  ( 92.34999999999999432, 90.00000000000002842, 77.29999999999999716 ) ) ;
#24030=DIRECTION ( 'NONE',  ( -3.061616997868382648E-16, -1.000000000000000000, -5.966227995846078450E-16 ) ) ;
#24034=CARTESIAN_POINT ( 'NONE',  ( 92.69370383062501162, -209.9999999999999716, 80.91156250086716284 ) ) ;
#24040=ORIENTED_EDGE ( 'NONE', *, *, #60381, .F. ) ;
#24043=CARTESIAN_POINT ( 'NONE',  ( 96.15314808468750130, -211.9973110713294489, 76.51947916753380241 ) ) ;
#24046=CARTESIAN_POINT ( 'NONE',  ( 93.84685191531251292, -211.9973110713294489, 81.01739583420049939 ) ) ;
#24052=ORIENTED_EDGE ( 'NONE', *, *, #15712, .F. ) ;
#24054=SURFACE_STYLE_FILL_AREA ( #1525 ) ;
#24058=CARTESIAN_POINT ( 'NONE',  ( 96.32499999999998863, -207.7050326799711968, 85.42270833506762528 ) ) ;
#24059=CARTESIAN_POINT ( 'NONE',  ( 92.34999999999999432, 88.47002178664753558, 87.51291666666666913 ) ) ;
#24063=LINE ( 'NONE', #13126, #39343 ) ;
#24064=ORIENTED_EDGE ( 'NONE', *, *, #6461, .F. ) ;
#24067=EDGE_LOOP ( 'NONE', ( #24441, #13023, #24540, #20713 ) ) ;
#24068=CARTESIAN_POINT ( 'NONE',  ( 92.34999999999999432, 91.52997821335252127, 86.85145833506763324 ) ) ;
#24071=ORIENTED_EDGE ( 'NONE', *, *, #47204, .T. ) ;
#24076=ORIENTED_EDGE ( 'NONE', *, *, #64799, .T. ) ;
#24082=CARTESIAN_POINT ( 'NONE',  ( -97.65000000000001990, 90.00000000000004263, 88.09499999999999886 ) ) ;
#24084=CARTESIAN_POINT ( 'NONE',  ( -92.35000000000003695, 90.00000000000004263, 90.00000000000000000 ) ) ;
#24087=CARTESIAN_POINT ( 'NONE',  ( 92.35000000000005116, 91.52997821335254969, 75.34208333333333485 ) ) ;
#24088=CARTESIAN_POINT ( 'NONE',  ( -97.30629616937497417, -211.3315407142195852, 83.98072916753380923 ) ) ;
#24090=CARTESIAN_POINT ( 'NONE',  ( -93.09170270117147084, 88.16127723153178408, 74.99954709728267233 ) ) ;
#24093=CARTESIAN_POINT ( 'NONE',  ( -96.15314808468747287, -208.0026889286704943, 76.20197916753380696 ) ) ;
#24097=CARTESIAN_POINT ( 'NONE',  ( 2.500000000000029754, 73.00000000000001421, -251.7000000000000455 ) ) ;
#24099=CARTESIAN_POINT ( 'NONE',  ( 92.35000000003290666, -209.9999916046337205, 84.99910573348564924 ) ) ;
#24101=CARTESIAN_POINT ( 'NONE',  ( -95.00000000000002842, 92.66308142843932671, 78.05406250086714692 ) ) ;
#24103=CARTESIAN_POINT ( 'NONE',  ( -97.65000000000001990, 90.00000000000004263, 76.03000000000000114 ) ) ;
#24106=B_SPLINE_CURVE_WITH_KNOTS ( 'NONE', 1,
 ( #16954, #39891 ),
 .UNSPECIFIED., .F., .F.,
 ( 2, 2 ),
 ( 0.000000000000000000, 1.000000000000000000 ),
 .UNSPECIFIED. ) ;
#24107=EDGE_CURVE ( 'NONE', #50232, #13102, #55559, .T. ) ;
#24110=DIRECTION ( 'NONE',  ( 1.000000000000000000, 0.000000000000000000, 0.000000000000000000 ) ) ;
#24112=CARTESIAN_POINT ( 'NONE',  ( 96.32499999999998863, -212.2949673200287179, 75.05104166840095559 ) ) ;
#24113=CARTESIAN_POINT ( 'NONE',  ( -95.00000000000002842, 93.05995642670504253, 87.38062500173430180 ) ) ;
#24114=CARTESIAN_POINT ( 'NONE',  ( -92.69370383062498320, -211.3315407142195852, 75.46114583420049371 ) ) ;
#24116=EDGE_CURVE ( 'NONE', #62043, #18290, #63307, .T. ) ;
#24117=CYLINDRICAL_SURFACE ( 'NONE', #5685, 2.649999999999999467 ) ;
#24131=CARTESIAN_POINT ( 'NONE',  ( 97.30629616937498838, -209.9999999999999716, 86.15031250086714465 ) ) ;
#24134=CARTESIAN_POINT ( 'NONE',  ( 92.69370383062501162, -211.3315407142195852, 89.21947916753381946 ) ) ;
#24142=CARTESIAN_POINT ( 'NONE',  ( -93.84685191531252713, 88.00268892867056536, 79.85322916753381151 ) ) ;
#24150=VERTEX_POINT ( 'NONE', #61578 ) ;
#24153=CARTESIAN_POINT ( 'NONE',  ( 92.35000000009274856, -209.9999861897330788, 80.55392363656960697 ) ) ;
#24157=CARTESIAN_POINT ( 'NONE',  ( 92.69370383062501162, -208.6684592857803011, 80.69989583420048973 ) ) ;
#24162=CARTESIAN_POINT ( 'NONE',  ( 99.99999999999997158, -90.00000000000000000, -90.00000000000014211 ) ) ;
#24164=CARTESIAN_POINT ( 'NONE',  ( -97.30629616937497417, -211.3315407142195852, 83.98072916753380923 ) ) ;
#24165=CARTESIAN_POINT ( 'NONE',  ( -92.69370383062502583, 91.33154071421968467, 83.82197916753382572 ) ) ;
#24167=CARTESIAN_POINT ( 'NONE',  ( 97.30629616937498838, 88.66845928578037217, 82.28739583420048120 ) ) ;
#24169=CARTESIAN_POINT ( 'NONE',  ( -97.65000000000001990, 90.00000000000004263, 78.64937500173429896 ) ) ;
#24170=LINE ( 'NONE', #70371, #1200 ) ;
#24173=CARTESIAN_POINT ( 'NONE',  ( -97.30629616937497417, -211.3315407142195852, 87.15572916753380639 ) ) ;
#24176=AXIS2_PLACEMENT_3D ( 'NONE', #42296, #7696, #8447 ) ;
#24177=CARTESIAN_POINT ( 'NONE',  ( -95.00000000000002842, 90.00000000000004263, 90.00000000000000000 ) ) ;
#24178=CARTESIAN_POINT ( 'NONE',  ( -97.65000000000001990, 90.00000000000004263, 87.45999999999999375 ) ) ;
#24184=CARTESIAN_POINT ( 'NONE',  ( -92.35000000000003695, 90.00000000000004263, 79.52249999999999375 ) ) ;
#24186=CARTESIAN_POINT ( 'NONE',  ( -93.84685191531252713, 88.00268892867056536, 88.58447916753381435 ) ) ;
#24188=CARTESIAN_POINT ( 'NONE',  ( 92.34999999999993747, 91.52997821335250705, 76.61208333333333087 ) ) ;
#24190=CARTESIAN_POINT ( 'NONE',  ( -92.34999999999999432, -209.9999999999999716, 78.25249999999999773 ) ) ;
#24202=CARTESIAN_POINT ( 'NONE',  ( -97.30629616937495996, -209.9999999999999716, 85.99156250086716113 ) ) ;
#24204=ADVANCED_FACE ( 'NONE', ( #62713 ), #61949, .F. ) ;
#24206=( BOUNDED_CURVE ( )  B_SPLINE_CURVE ( 2, ( #6136, #6853, #51608, #519, #34312, #11379, #51231, #45624, #23413 ),
 .UNSPECIFIED., .F., .F. ) 
 B_SPLINE_CURVE_WITH_KNOTS ( ( 3, 2, 2, 2, 3 ),
 ( 0.5291824299534890752, 0.5362381811096936790, 0.5432939466506105930, 0.5503497121915276180, 0.5503499107253647660 ),
 .UNSPECIFIED. ) 
 CURVE ( )  GEOMETRIC_REPRESENTATION_ITEM ( )  RATIONAL_B_SPLINE_CURVE ( ( 1.000000000000000000, 0.8660254037844387076, 1.000000000000000000, 0.8660254037844387076, 1.000000000000000000, 0.8660254037844387076, 1.000000000000000000, 0.9999962302473756059, 0.9999924607068964022 ) ) 
 REPRESENTATION_ITEM ( '' )  );
#24210=CARTESIAN_POINT ( 'NONE',  ( -97.30629616937497417, -208.6684592857803295, 75.14364583420049826 ) ) ;
#24216=CARTESIAN_POINT ( 'NONE',  ( -93.84685191531252713, 88.00268892867056536, 75.40822916753381833 ) ) ;
#24217=CARTESIAN_POINT ( 'NONE',  ( 97.30629616937498838, -209.9999999999999716, 77.26031250086714408 ) ) ;
#24219=VERTEX_POINT ( 'NONE', #50276 ) ;
#24226=CARTESIAN_POINT ( 'NONE',  ( -92.35003071823130938, 91.52999594853163501, 79.01979289519825045 ) ) ;
#24228=EDGE_CURVE ( 'NONE', #29135, #2794, #29238, .T. ) ;
#24237=CARTESIAN_POINT ( 'NONE',  ( 97.30629616937498838, 91.33154071421968467, 79.37697916753381833 ) ) ;
#24238=CARTESIAN_POINT ( 'NONE',  ( -93.67500000000003979, 87.70503267997129626, 81.40104166840096411 ) ) ;
#24239=CARTESIAN_POINT ( 'NONE',  ( 97.64999999999997726, -208.4700217866474645, 75.13041666666666174 ) ) ;
#24245=AXIS2_PLACEMENT_3D ( 'NONE', #17578, #28479, #22871 ) ;
#24247=CARTESIAN_POINT ( 'NONE',  ( -93.67499999999998295, -207.7050326799711968, 75.26270833506764291 ) ) ;
#24253=CARTESIAN_POINT ( 'NONE',  ( -97.64999999999994884, -211.5299782133524502, 79.33729166840096525 ) ) ;
#24257=CARTESIAN_POINT ( 'NONE',  ( 94.99999999999998579, 93.05995642670504253, 79.76062500173429726 ) ) ;
#24258=CARTESIAN_POINT ( 'NONE',  ( -92.35000000000005116, 88.47002178664754979, 75.73895833506765030 ) ) ;
#24260=CARTESIAN_POINT ( 'NONE',  ( 96.15314808468748708, 91.99731107132950569, 79.42989583420049371 ) ) ;
#24261=CARTESIAN_POINT ( 'NONE',  ( -0.0004442498525516064278, 0.001194404164626844313, -80.00000000000000000 ) ) ;
#24267=DIRECTION ( 'NONE',  ( 1.000000000000000000, 0.000000000000000000, 0.000000000000000000 ) ) ;
#24270=EDGE_CURVE ( 'NONE', #66690, #35348, #62876, .T. ) ;
#24276=CARTESIAN_POINT ( 'NONE',  ( -97.30629616937495996, -209.9999999999999716, 77.73656250086715147 ) ) ;
#24283=DIRECTION ( 'NONE',  ( -0.000000000000000000, -0.000000000000000000, 1.000000000000000000 ) ) ;
#24285=DIRECTION ( 'NONE',  ( -0.000000000000000000, -0.000000000000000000, 1.000000000000000000 ) ) ;
#24289=CARTESIAN_POINT ( 'NONE',  ( -92.35000000000006537, -209.9999992849074317, 85.31687502647974952 ) ) ;
#24294=CARTESIAN_POINT ( 'NONE',  ( 92.69370383062498320, 91.33154071421968467, 85.93864583420051417 ) ) ;
#24295=CARTESIAN_POINT ( 'NONE',  ( -92.69370383062498320, -211.3315407142195852, 86.89114583420048632 ) ) ;
#24296=CARTESIAN_POINT ( 'NONE',  ( 93.67500000000001137, -212.2949673200287179, 83.83520833506763381 ) ) ;
#24299=CARTESIAN_POINT ( 'NONE',  ( -93.67499999999998295, -212.2949673200287179, 80.05166666666666231 ) ) ;
#24300=CARTESIAN_POINT ( 'NONE',  ( -93.84685191531254134, 91.99731107132950569, 75.46114583420047950 ) ) ;
#24303=CARTESIAN_POINT ( 'NONE',  ( 97.30629616937498838, -208.6684592857803011, 85.56822916753380071 ) ) ;
#24309=FACE_OUTER_BOUND ( 'NONE', #38170, .T. ) ;
#24313=CARTESIAN_POINT ( 'NONE',  ( 96.15314808468748708, -208.0026889286704943, 81.96989583420048575 ) ) ;
#24314=CARTESIAN_POINT ( 'NONE',  ( 94.99999999999998579, 93.05995642670504253, 89.84125000000000227 ) ) ;
#24319=CARTESIAN_POINT ( 'NONE',  ( 96.32499999999998863, -207.7050326799711968, 85.97833333333332462 ) ) ;
#24323=ORIENTED_EDGE ( 'NONE', *, *, #35646, .F. ) ;
#24326=CARTESIAN_POINT ( 'NONE',  ( -97.30629616937501680, 91.33154071421968467, 88.47864583420047779 ) ) ;
#24329=CARTESIAN_POINT ( 'NONE',  ( 96.32499999999998863, -207.7050326799711968, 74.62770833506762358 ) ) ;
#24330=CARTESIAN_POINT ( 'NONE',  ( 93.67499999999998295, 92.29496732002878900, 78.46416666666667084 ) ) ;
#24332=CARTESIAN_POINT ( 'NONE',  ( -97.64999999999994884, -208.4700217866474645, 89.39145833506763950 ) ) ;
#24334=ORIENTED_EDGE ( 'NONE', *, *, #26060, .T. ) ;
#24337=CARTESIAN_POINT ( 'NONE',  ( -97.65000000000001990, 88.47002178664754979, 86.95729166840096980 ) ) ;
#24339=CARTESIAN_POINT ( 'NONE',  ( 92.69370383062498320, 91.33154071421968467, 74.98489583420048632 ) ) ;
#24341=FACE_OUTER_BOUND ( 'NONE', #59560, .T. ) ;
#24344=CARTESIAN_POINT ( 'NONE',  ( -95.00000000000002842, 90.00000000000004263, 90.00000000000000000 ) ) ;
#24345=ORIENTED_EDGE ( 'NONE', *, *, #46673, .F. ) ;
#24350=ORIENTED_EDGE ( 'NONE', *, *, #7280, .F. ) ;
#24358=CARTESIAN_POINT ( 'NONE',  ( -96.15314808468745866, -211.9973110713294489, 89.27239583420049485 ) ) ;
#24363=EDGE_CURVE ( 'NONE', #9807, #6402, #50326, .T. ) ;
#24367=CARTESIAN_POINT ( 'NONE',  ( 94.99999999999998579, 92.66308142843932671, 83.13406250086714522 ) ) ;
#24370=CARTESIAN_POINT ( 'NONE',  ( 94.99999999999998579, 90.00000000000002842, 90.00000000000000000 ) ) ;
#24378=CARTESIAN_POINT ( 'NONE',  ( -92.69370383062504004, 90.00000000000004263, 86.78531250086714977 ) ) ;
#24393=CARTESIAN_POINT ( 'NONE',  ( 97.30629616937498838, -211.3315407142195852, 83.08114583420048405 ) ) ;
#24397=LINE ( 'NONE', #35313, #67766 ) ;
#24400=CARTESIAN_POINT ( 'NONE',  ( 96.15314808468750130, -211.9973110713294489, 79.21822916753382060 ) ) ;
#24404=ORIENTED_EDGE ( 'NONE', *, *, #71596, .T. ) ;
#24405=CARTESIAN_POINT ( 'NONE',  ( 93.67500000000001137, -207.7050326799711968, 86.79854166840097207 ) ) ;
#24408=CARTESIAN_POINT ( 'NONE',  ( -93.67500000000003979, 92.29496732002878900, 84.07333333333333769 ) ) ;
#24409=CARTESIAN_POINT ( 'NONE',  ( 93.67500000000001137, -212.2949673200287179, 83.20020833506764291 ) ) ;
#24410=CARTESIAN_POINT ( 'NONE',  ( 96.32499999999998863, 87.70503267997126784, 89.57666666666666799 ) ) ;
#24417=( BOUNDED_CURVE ( )  B_SPLINE_CURVE ( 2, ( #62185, #33598, #27959, #17429, #24545, #40736, #51640 ),
 .UNSPECIFIED., .F., .F. ) 
 B_SPLINE_CURVE_WITH_KNOTS ( ( 3, 2, 2, 3 ),
 ( 0.6350190250571088324, 0.6420746642202955767, 0.6491304297611778518, 0.6561861948910822084 ),
 .UNSPECIFIED. ) 
 CURVE ( )  GEOMETRIC_REPRESENTATION_ITEM ( )  RATIONAL_B_SPLINE_CURVE ( ( 0.9999952007766184092, 0.8660278034391103441, 1.000000000000000000, 0.8660254037844387076, 1.000000000000000000, 0.8660254037844387076, 1.000000000000000000 ) ) 
 REPRESENTATION_ITEM ( '' )  );
#24420=CARTESIAN_POINT ( 'NONE',  ( 94.99999999999998579, 86.94004357329500010, 87.69812500173429726 ) ) ;
#24422=ORIENTED_EDGE ( 'NONE', *, *, #38002, .T. ) ;
#24430=CARTESIAN_POINT ( 'NONE',  ( -96.32500000000001705, 92.29496732002878900, 86.08416666666666117 ) ) ;
#24432=DIRECTION ( 'NONE',  ( -0.000000000000000000, -0.000000000000000000, -1.000000000000000000 ) ) ;
#24433=CARTESIAN_POINT ( 'NONE',  ( -97.65000000000001990, 88.47002178664754979, 87.51291666666666913 ) ) ;
#24438=ORIENTED_EDGE ( 'NONE', *, *, #57368, .F. ) ;
#24439=FACE_OUTER_BOUND ( 'NONE', #30389, .T. ) ;
#24440=CARTESIAN_POINT ( 'NONE',  ( -93.84685191531248449, -208.0026889286704943, 84.35114583420048007 ) ) ;
#24441=ORIENTED_EDGE ( 'NONE', *, *, #214, .F. ) ;
#24447=EDGE_CURVE ( 'NONE', #64948, #37629, #63731, .T. ) ;
#24450=AXIS2_PLACEMENT_3D ( 'NONE', #5532, #288, #73550 ) ;
#24456=CARTESIAN_POINT ( 'NONE',  ( -95.00000000000002842, 87.33691857156074434, 77.73656250086713726 ) ) ;
#24463=VECTOR ( 'NONE', #68367, 1000.000000000000000 ) ;
#24465=CARTESIAN_POINT ( 'NONE',  ( -97.64997399466339800, -211.5299932275404728, 84.41729270697886989 ) ) ;
#24470=CARTESIAN_POINT ( 'NONE',  ( -94.53673242685059108, -212.8430781844921569, 74.72378867588408013 ) ) ;
#24471=CARTESIAN_POINT ( 'NONE',  ( -95.00000000000002842, 90.00000000000004263, 90.00000000000000000 ) ) ;
#24473=ORIENTED_EDGE ( 'NONE', *, *, #38044, .T. ) ;
#24479=VECTOR ( 'NONE', #64636, 1000.000000000000000 ) ;
#24481=VERTEX_POINT ( 'NONE', #67869 ) ;
#24485=AXIS2_PLACEMENT_3D ( 'NONE', #7580, #1976, #24864 ) ;
#24486=CARTESIAN_POINT ( 'NONE',  ( 93.84685191531251292, -211.9973110713294489, 84.66864583420047552 ) ) ;
#24487=CARTESIAN_POINT ( 'NONE',  ( 92.69370383062501162, -211.3315407142195852, 87.31447916753381833 ) ) ;
#24490=ORIENTED_EDGE ( 'NONE', *, *, #15432, .F. ) ;
#24495=CARTESIAN_POINT ( 'NONE',  ( -93.84685191531254134, 91.99731107132950569, 80.69989583420047552 ) ) ;
#24511=CARTESIAN_POINT ( 'NONE',  ( 92.69370383062501162, -209.9999999999999716, 82.02281250086714692 ) ) ;
#24512=CARTESIAN_POINT ( 'NONE',  ( -97.65000000000010516, 91.52997821335250705, 83.59708333333334451 ) ) ;
#24513=CARTESIAN_POINT ( 'NONE',  ( -94.99999999999997158, -213.0599564267049857, 85.79312500173431033 ) ) ;
#24514=EDGE_CURVE ( 'NONE', #3169, #32383, #29665, .T. ) ;
#24515=DIRECTION ( 'NONE',  ( -0.000000000000000000, -0.000000000000000000, 1.000000000000000000 ) ) ;
#24521=CARTESIAN_POINT ( 'NONE',  ( -96.15314808468745866, -211.9973110713294489, 84.03364583420047040 ) ) ;
#24522=CARTESIAN_POINT ( 'NONE',  ( -97.30629616937501680, 90.00000000000004263, 82.81656250086714977 ) ) ;
#24525=CARTESIAN_POINT ( 'NONE',  ( 92.69370383062498320, 90.00000000000002842, 79.48281250086714067 ) ) ;
#24531=LINE ( 'NONE', #11397, #30746 ) ;
#24533=CARTESIAN_POINT ( 'NONE',  ( -93.84685191531248449, -208.0026889286704943, 83.08114583420048405 ) ) ;
#24540=ORIENTED_EDGE ( 'NONE', *, *, #18471, .T. ) ;
#24543=CARTESIAN_POINT ( 'NONE',  ( -95.00000000000002842, 92.66308142843932671, 88.21406250086714351 ) ) ;
#24545=CARTESIAN_POINT ( 'NONE',  ( -93.67500000000003979, 92.29496732002878900, 79.70770833506762187 ) ) ;
#24551=ADVANCED_FACE ( 'NONE', ( #72380 ), #49818, .F. ) ;
#24552=CARTESIAN_POINT ( 'NONE',  ( -96.15314808468751551, 88.00268892867056536, 76.41364583420048007 ) ) ;
#24556=EDGE_CURVE ( 'NONE', #55829, #15433, #62428, .T. ) ;
#24561=CARTESIAN_POINT ( 'NONE',  ( -92.69370383062498320, -211.3315407142195852, 85.62114583420047609 ) ) ;
#24566=CARTESIAN_POINT ( 'NONE',  ( 97.30629616937498838, 89.06968786819598449, 74.84209103131392737 ) ) ;
#24568=CARTESIAN_POINT ( 'NONE',  ( -94.99999999999997158, -212.6630814284392557, 76.62531250086715318 ) ) ;
#24572=CARTESIAN_POINT ( 'NONE',  ( 96.32499999999997442, 92.29496732002878900, 75.81833333333332803 ) ) ;
#24575=CARTESIAN_POINT ( 'NONE',  ( 93.84685191531249870, -208.0026889286704943, 76.83697916753381207 ) ) ;
#24583=VECTOR ( 'NONE', #64190, 1000.000000000000000 ) ;
#24590=CARTESIAN_POINT ( 'NONE',  ( 92.69370383062498320, 90.00000000000002842, 81.54656250086715374 ) ) ;
#24592=CARTESIAN_POINT ( 'NONE',  ( -95.00000000000002842, 86.94004357329504273, 81.34812500173430294 ) ) ;
#24597=ORIENTED_EDGE ( 'NONE', *, *, #19411, .T. ) ;
#24598=DIRECTION ( 'NONE',  ( 1.000000000000000000, 0.000000000000000000, 0.000000000000000000 ) ) ;
#24603=CARTESIAN_POINT ( 'NONE',  ( -96.13030974027475395, 92.14422361751735480, 74.86230178910948041 ) ) ;
#24607=CARTESIAN_POINT ( 'NONE',  ( 96.32499999999997442, 92.29496732002878900, 77.72333333333332916 ) ) ;
#24608=EDGE_CURVE ( 'NONE', #16444, #23574, #66510, .T. ) ;
#24609=CARTESIAN_POINT ( 'NONE',  ( -94.99999999999997158, -213.0599564267049857, 78.80812500173429669 ) ) ;
#24612=CARTESIAN_POINT ( 'NONE',  ( 92.34999999999999432, 90.00000000000002842, 75.47437500173430180 ) ) ;
#24613=CARTESIAN_POINT ( 'NONE',  ( -97.65000000000001990, 90.00000000000004263, 75.47437500173430180 ) ) ;
#24616=CARTESIAN_POINT ( 'NONE',  ( 96.15314808468748708, 88.00268892867053694, 77.31322916753381946 ) ) ;
#24617=CARTESIAN_POINT ( 'NONE',  ( -97.64999999999996305, -208.4700217866474645, 82.32708333333334849 ) ) ;
#24621=CARTESIAN_POINT ( 'NONE',  ( 92.35000000000000853, -209.9999856621383003, 79.28437450583713542 ) ) ;
#24635=( BOUNDED_CURVE ( )  B_SPLINE_CURVE ( 2, ( #6087, #12072, #16982, #16231, #68490, #17343, #51556 ),
 .UNSPECIFIED., .F., .F. ) 
 B_SPLINE_CURVE_WITH_KNOTS ( ( 3, 2, 2, 3 ),
 ( 0.1905056698837211959, 0.1975614351447063655, 0.2046172006855887515, 0.2116728463006670169 ),
 .UNSPECIFIED. ) 
 CURVE ( )  GEOMETRIC_REPRESENTATION_ITEM ( )  RATIONAL_B_SPLINE_CURVE ( ( 1.000000000000000000, 0.8660254037844387076, 1.000000000000000000, 0.8660254037844387076, 1.000000000000000000, 0.8660276809308509183, 0.9999954457845842137 ) ) 
 REPRESENTATION_ITEM ( '' )  );
#24636=CARTESIAN_POINT ( 'NONE',  ( -97.30629616937497417, -208.6684592857803011, 77.04864583420048518 ) ) ;
#24653=CARTESIAN_POINT ( 'NONE',  ( 92.69370383062498320, 91.33154071421968467, 85.30364583420048064 ) ) ;
#24654=CARTESIAN_POINT ( 'NONE',  ( -92.69370383062498320, -209.9999999999999716, 86.94406250086716170 ) ) ;
#24656=ORIENTED_EDGE ( 'NONE', *, *, #59319, .T. ) ;
#24657=CARTESIAN_POINT ( 'NONE',  ( -92.35000000000009379, 91.52997821335256390, 81.48041666666665606 ) ) ;
#24658=CARTESIAN_POINT ( 'NONE',  ( -97.64999999999994884, -208.4700217866474645, 82.32708333333332007 ) ) ;
#24659=CARTESIAN_POINT ( 'NONE',  ( -96.15314808468752972, 91.99731107132950569, 77.47197916753380298 ) ) ;
#24660=VECTOR ( 'NONE', #11898, 1000.000000000000000 ) ;
#24662=CARTESIAN_POINT ( 'NONE',  ( 95.00000000000000000, -212.6630814284392557, 87.89656250086713385 ) ) ;
#24666=EDGE_LOOP ( 'NONE', ( #27491, #13938, #42584, #38000 ) ) ;
#24673=CARTESIAN_POINT ( 'NONE',  ( 95.00000000000000000, -207.3369185715606307, 82.65781250086715204 ) ) ;
#24676=EDGE_CURVE ( 'NONE', #15642, #44823, #23759, .T. ) ;
#24677=CARTESIAN_POINT ( 'NONE',  ( 93.67500000000001137, -212.2949673200287179, 80.58083333333331666 ) ) ;
#24678=CARTESIAN_POINT ( 'NONE',  ( 92.35000000000003695, 88.47002178664747873, 76.71791666666666742 ) ) ;
#24680=CARTESIAN_POINT ( 'NONE',  ( 96.32499999999998863, -212.2949673200287179, 84.49666666666666970 ) ) ;
#24688=CARTESIAN_POINT ( 'NONE',  ( -97.30629616937501680, 88.66845928578038638, 87.94947916753382344 ) ) ;
#24691=CARTESIAN_POINT ( 'NONE',  ( -92.35000000000003695, 90.00000000000004263, 83.96750000000000114 ) ) ;
#24692=CARTESIAN_POINT ( 'NONE',  ( 96.15314808468748708, -208.0026889286704943, 87.52614583420047722 ) ) ;
#24693=CARTESIAN_POINT ( 'NONE',  ( 94.99999999999998579, 86.94004357329500010, 79.99874999999998693 ) ) ;
#24696=CARTESIAN_POINT ( 'NONE',  ( -96.32499999999996021, -207.7050326799711968, 88.70354166840097321 ) ) ;
#24698=CARTESIAN_POINT ( 'NONE',  ( 96.32499999999998863, -212.2949673200287179, 80.05166666666666231 ) ) ;
#24700=CARTESIAN_POINT ( 'NONE',  ( -96.32500000000001705, 92.29496732002878900, 86.16354166840096696 ) ) ;
#24702=CARTESIAN_POINT ( 'NONE',  ( 96.15314808468748708, 91.99731107132950569, 89.58989583420049030 ) ) ;
#24710=CYLINDRICAL_SURFACE ( 'NONE', #17098, 2.649999999999999467 ) ;
#24712=CARTESIAN_POINT ( 'NONE',  ( -96.15314808468745866, -211.9973110713294489, 75.14364583420046984 ) ) ;
#24718=EDGE_CURVE ( 'NONE', #72660, #74057, #40234, .T. ) ;
#24723=CARTESIAN_POINT ( 'NONE',  ( -97.30629616937497417, -211.3315407142195852, 87.31447916753381833 ) ) ;
#24729=CARTESIAN_POINT ( 'NONE',  ( -97.65000000000001990, 90.00000000000004263, 86.82500000000000284 ) ) ;
#24730=AXIS2_PLACEMENT_3D ( 'NONE', #25585, #48518, #14307 ) ;
#24732=CARTESIAN_POINT ( 'NONE',  ( 92.69370383062498320, 90.00000000000002842, 82.02281250086714692 ) ) ;
#24734=FACE_BOUND ( 'NONE', #34859, .T. ) ;
#24735=CARTESIAN_POINT ( 'NONE',  ( -95.00000000000002842, 93.05995642670504253, 85.39624999999998067 ) ) ;
#24740=CARTESIAN_POINT ( 'NONE',  ( 93.67500000000001137, -207.7050326799711968, 85.52854166840096184 ) ) ;
#24743=CARTESIAN_POINT ( 'NONE',  ( -97.30629616937501680, 91.33154071421968467, 86.41489583420047893 ) ) ;
#24753=CARTESIAN_POINT ( 'NONE',  ( 96.15314808468748708, -208.0026889286704943, 81.33489583420049485 ) ) ;
#24761=ORIENTED_EDGE ( 'NONE', *, *, #4506, .F. ) ;
#24765=CARTESIAN_POINT ( 'NONE',  ( 92.69370383062501162, -211.3315407142195852, 75.72572916753381378 ) ) ;
#24767=CARTESIAN_POINT ( 'NONE',  ( 97.30629616937498838, -209.9999999999999716, 79.95906250086714806 ) ) ;
#24778=CARTESIAN_POINT ( 'NONE',  ( 95.00000000000000000, -206.9400435732949575, 83.57062500173429953 ) ) ;
#24779=CARTESIAN_POINT ( 'NONE',  ( 96.32499999999997442, 92.29496732002878900, 89.15333333333333599 ) ) ;
#24785=CARTESIAN_POINT ( 'NONE',  ( -97.30629616937501680, 90.00000000000004263, 89.16656250086715829 ) ) ;
#24787=CARTESIAN_POINT ( 'NONE',  ( 92.69370383062498320, 88.66845928578037217, 83.98072916753380923 ) ) ;
#24789=CARTESIAN_POINT ( 'NONE',  ( 96.32499999999998863, 87.70503267997126784, 85.84604166840097150 ) ) ;
#24791=ORIENTED_EDGE ( 'NONE', *, *, #60381, .T. ) ;
#24793=CARTESIAN_POINT ( 'NONE',  ( 92.35000000021533140, 90.00002100773845370, 79.91868729553033290 ) ) ;
#24799=CARTESIAN_POINT ( 'NONE',  ( -97.65000000000001990, 90.00000000000004263, 84.92000000000000171 ) ) ;
#24803=CARTESIAN_POINT ( 'NONE',  ( 94.99999999999998579, 86.94004357329502852, 81.90375000000000227 ) ) ;
#24807=CARTESIAN_POINT ( 'NONE',  ( -92.69370383062498320, -209.9999999999999716, 83.61031250086713840 ) ) ;
#24822=CARTESIAN_POINT ( 'NONE',  ( 92.34999999999999432, 90.00000000000002842, 83.09437500173430635 ) ) ;
#24824=CARTESIAN_POINT ( 'NONE',  ( -93.84685191531254134, 91.99731107132950569, 76.09614583420047040 ) ) ;
#24829=PLANE ( 'NONE',  #72515 ) ;
#24831=CARTESIAN_POINT ( 'NONE',  ( 93.67500000000001137, -212.2949673200287179, 77.40583333333331950 ) ) ;
#24833=CARTESIAN_POINT ( 'NONE',  ( 96.32499999999998863, 87.70503267997126784, 75.68604166840097491 ) ) ;
#24834=CARTESIAN_POINT ( 'NONE',  ( -97.30629616937497417, -211.3315407142195852, 75.24947916753383481 ) ) ;
#24838=CARTESIAN_POINT ( 'NONE',  ( 97.64999999999992042, -211.5299782133524786, 88.35958333333334735 ) ) ;
#24846=EDGE_CURVE ( 'NONE', #21322, #32442, #34089, .T. ) ;
#24849=( BOUNDED_CURVE ( )  B_SPLINE_CURVE ( 2, ( #4026, #38964, #37854, #31818, #3657, #26557, #22034 ),
 .UNSPECIFIED., .F., .F. ) 
 B_SPLINE_CURVE_WITH_KNOTS ( ( 3, 2, 2, 3 ),
 ( 0.5503499107226623721, 0.5574054777297072771, 0.5644612432705895522, 0.5715170088666297055 ),
 .UNSPECIFIED. ) 
 CURVE ( )  GEOMETRIC_REPRESENTATION_ITEM ( )  RATIONAL_B_SPLINE_CURVE ( ( 0.9999924607068793048, 0.8660291735370716504, 1.000000000000000000, 0.8660254037844387076, 1.000000000000000000, 0.8660254037844387076, 1.000000000000000000 ) ) 
 REPRESENTATION_ITEM ( '' )  );
#24850=CARTESIAN_POINT ( 'NONE',  ( 95.00000000000000000, -212.6630814284392557, 84.08656250086714579 ) ) ;
#24860=CARTESIAN_POINT ( 'NONE',  ( -95.00000000000002842, 87.33691857156074434, 81.70531250086715147 ) ) ;
#24864=DIRECTION ( 'NONE',  ( 0.000000000000000000, 0.000000000000000000, 1.000000000000000000 ) ) ;
#24873=VERTEX_POINT ( 'NONE', #37998 ) ;
#24878=VERTEX_POINT ( 'NONE', #45889 ) ;
#24879=CARTESIAN_POINT ( 'NONE',  ( 92.69370383062501162, -209.9999999999999716, 79.48281250086714067 ) ) ;
#24885=CARTESIAN_POINT ( 'NONE',  ( -97.64999999999996305, -209.9999999999999716, 90.00000000000000000 ) ) ;
#24888=CARTESIAN_POINT ( 'NONE',  ( -89.99999999999998579, -124.0000000000000142, 39.99999999999996447 ) ) ;
#24889=CARTESIAN_POINT ( 'NONE',  ( -96.15314808468745866, -211.9973110713294489, 80.22364583420046813 ) ) ;
#24890=VECTOR ( 'NONE', #49192, 1000.000000000000000 ) ;
#24891=CARTESIAN_POINT ( 'NONE',  ( -93.84685191531254134, 91.99731107132950569, 80.69989583420047552 ) ) ;
#24894=EDGE_CURVE ( 'NONE', #48383, #60757, #65709, .T. ) ;
#24895=CARTESIAN_POINT ( 'NONE',  ( 94.99999999999998579, 87.33691857156068750, 80.91156250086714863 ) ) ;
#24897=CARTESIAN_POINT ( 'NONE',  ( 94.99999999999998579, 90.00000000000002842, 73.40771935957695860 ) ) ;
#24901=CARTESIAN_POINT ( 'NONE',  ( -94.99999999999997158, -212.6630814284392557, 83.45156250086714067 ) ) ;
#24904=DIRECTION ( 'NONE',  ( 1.000000000000000000, 0.000000000000000000, 0.000000000000000000 ) ) ;
#24910=CARTESIAN_POINT ( 'NONE',  ( -92.69370383062502583, 88.66845928578038638, 84.82739583420045903 ) ) ;
#24911=CARTESIAN_POINT ( 'NONE',  ( -97.50991008589724629, -209.8784921249854563, 74.91582548749271098 ) ) ;
#24923=CARTESIAN_POINT ( 'NONE',  ( 96.32499999999998863, -207.7050326799711968, 84.15270833506762926 ) ) ;
#24925=CARTESIAN_POINT ( 'NONE',  ( -97.30629616937497417, -208.6684592857803011, 85.30364583420048064 ) ) ;
#24930=CARTESIAN_POINT ( 'NONE',  ( -92.69370383062498320, -211.3315407142195852, 77.36614583420048064 ) ) ;
#24933=DIRECTION ( 'NONE',  ( -0.000000000000000000, -0.000000000000000000, 1.000000000000000000 ) ) ;
#24934=CARTESIAN_POINT ( 'NONE',  ( 92.34999999999999432, 90.00000000000002842, 76.03000000000000114 ) ) ;
#24940=CARTESIAN_POINT ( 'NONE',  ( 96.15314808468750130, -211.9973110713294489, 75.88447916753381151 ) ) ;
#24944=EDGE_LOOP ( 'NONE', ( #56353, #29882, #41366, #74135 ) ) ;
#24947=EDGE_LOOP ( 'NONE', ( #12377, #9601, #53016, #22475 ) ) ;
#24953=CARTESIAN_POINT ( 'NONE',  ( -92.35000000000003695, 90.00000000000004263, 90.00000000000000000 ) ) ;
#24954=VERTEX_POINT ( 'NONE', #45515 ) ;
#24955=EDGE_CURVE ( 'NONE', #45415, #19936, #73368, .T. ) ;
#24957=CARTESIAN_POINT ( 'NONE',  ( 93.84685191531248449, 91.99731107132950569, 79.53572916753381605 ) ) ;
#24958=CARTESIAN_POINT ( 'NONE',  ( 97.64997490601828645, -211.5299927013694798, 89.07395733288659301 ) ) ;
#24960=ADVANCED_FACE ( 'NONE', ( #38746 ), #17292, .F. ) ;
#24961=CARTESIAN_POINT ( 'NONE',  ( -97.65000000000001990, 91.52997821335253548, 88.12145833506765769 ) ) ;
#24966=CARTESIAN_POINT ( 'NONE',  ( 92.34999999999999432, 90.00000000000002842, 90.00000000000000000 ) ) ;
#24969=EDGE_CURVE ( 'NONE', #49448, #41714, #32094, .T. ) ;
#24977=CARTESIAN_POINT ( 'NONE',  ( -92.34999999999999432, -209.9999999999999716, 79.60187500173429953 ) ) ;
#24980=CARTESIAN_POINT ( 'NONE',  ( 94.99999999999998579, 93.05995642670504253, 77.22062500173429100 ) ) ;
#24981=CARTESIAN_POINT ( 'NONE',  ( -93.67500000000003979, 87.70503267997129626, 75.68604166840097491 ) ) ;
#24983=CARTESIAN_POINT ( 'NONE',  ( 92.69370383062498320, 91.33154071421968467, 77.04864583420048518 ) ) ;
#24987=CARTESIAN_POINT ( 'NONE',  ( 96.32499999999998863, -212.2949673200287179, 77.59104166840097605 ) ) ;
#24995=ORIENTED_EDGE ( 'NONE', *, *, #63794, .T. ) ;
#24999=CARTESIAN_POINT ( 'NONE',  ( 92.35000000000002274, -210.0000065184971163, 88.17437522718662990 ) ) ;
#25001=DIRECTION ( 'NONE',  ( 0.000000000000000000, 0.000000000000000000, 1.000000000000000000 ) ) ;
#25002=CARTESIAN_POINT ( 'NONE',  ( -96.15314808468747287, -208.0026889286704943, 75.09072916753380866 ) ) ;
#25005=DIRECTION ( 'NONE',  ( 1.000000000000000000, 0.000000000000000000, 0.000000000000000000 ) ) ;
#25009=CARTESIAN_POINT ( 'NONE',  ( -95.00000000000002842, 90.00000000000004263, 90.00000000000000000 ) ) ;
#25012=CARTESIAN_POINT ( 'NONE',  ( -93.67499999999998295, -212.2949673200287179, 85.21104166840096639 ) ) ;
#25013=CARTESIAN_POINT ( 'NONE',  ( -97.64999999999997726, -210.0000092897485899, 78.01437532303467037 ) ) ;
#25015=CARTESIAN_POINT ( 'NONE',  ( 92.69370383062498320, 91.33154071421968467, 83.39864583420049371 ) ) ;
#25018=CARTESIAN_POINT ( 'NONE',  ( -93.84685191531248449, -208.0026889286704943, 87.68489583420048916 ) ) ;
#25020=EDGE_LOOP ( 'NONE', ( #3371, #31580, #68801, #56902, #28771 ) ) ;
#25022=CARTESIAN_POINT ( 'NONE',  ( -97.64999999999996305, -209.9999999999999716, 79.83999999999998920 ) ) ;
#25024=CARTESIAN_POINT ( 'NONE',  ( -92.69370383062505425, 91.33154071421968467, 75.40822916753381833 ) ) ;
#25028=EDGE_CURVE ( 'NONE', #70067, #21866, #53717, .T. ) ;
#25029=EDGE_CURVE ( 'NONE', #26516, #43747, #7856, .T. ) ;
#25030=CARTESIAN_POINT ( 'NONE',  ( 95.00000000000000000, -212.6630814284392557, 85.99156250086714692 ) ) ;
#25036=CARTESIAN_POINT ( 'NONE',  ( 95.00000000000000000, -206.9400435732949575, 84.12624999999999886 ) ) ;
#25039=ORIENTED_EDGE ( 'NONE', *, *, #65686, .T. ) ;
#25044=CARTESIAN_POINT ( 'NONE',  ( 93.84685191531251292, -211.9973110713294489, 77.84239583420048803 ) ) ;
#25046=CARTESIAN_POINT ( 'NONE',  ( -92.35000000000005116, 91.52997821335253548, 76.47979166840096354 ) ) ;
#25051=CARTESIAN_POINT ( 'NONE',  ( 97.64999999999999147, -209.9999999999999716, 83.33250000000001023 ) ) ;
#25056=CARTESIAN_POINT ( 'NONE',  ( -97.64999999980587120, -210.0000198427943587, 86.27002759516035724 ) ) ;
#25059=CARTESIAN_POINT ( 'NONE',  ( -93.84685191531252713, 88.00268892867056536, 84.93322916753382401 ) ) ;
#25068=VERTEX_POINT ( 'NONE', #35327 ) ;
#25069=CARTESIAN_POINT ( 'NONE',  ( -92.35000000000005116, 88.47002178664754979, 85.26395833506762756 ) ) ;
#25070=( BOUNDED_CURVE ( )  B_SPLINE_CURVE ( 2, ( #322, #23215, #63441, #11910, #34854, #57794, #29195, #46503, #683 ),
 .UNSPECIFIED., .F., .F. ) 
 B_SPLINE_CURVE_WITH_KNOTS ( ( 3, 2, 2, 2, 3 ),
 ( 0.3810111478265181262, 0.3810113392076479033, 0.3880671047485306779, 0.3951228702894135081, 0.4021785743327794815 ),
 .UNSPECIFIED. ) 
 CURVE ( )  GEOMETRIC_REPRESENTATION_ITEM ( )  RATIONAL_B_SPLINE_CURVE ( ( 0.9999927323225317188, 0.9999963660626987050, 1.000000000000000000, 0.8660254037844387076, 1.000000000000000000, 0.8660254037844387076, 1.000000000000000000, 0.8660265714968488071, 0.9999976645955351851 ) ) 
 REPRESENTATION_ITEM ( '' )  );
#25072=CARTESIAN_POINT ( 'NONE',  ( 97.30629616937498838, 90.00000000000002842, 85.67406250086715147 ) ) ;
#25077=CARTESIAN_POINT ( 'NONE',  ( -97.64998056384295921, -208.4700105651770627, 78.59645755884375262 ) ) ;
#25081=CARTESIAN_POINT ( 'NONE',  ( -93.33921309982507353, -211.6002465100980316, 74.64190636928354650 ) ) ;
#25084=ORIENTED_EDGE ( 'NONE', *, *, #46082, .F. ) ;
#25086=CARTESIAN_POINT ( 'NONE',  ( 96.32499999999998863, 87.70503267997126784, 78.86104166840097207 ) ) ;
#25089=CARTESIAN_POINT ( 'NONE',  ( -92.69370383062498320, -209.9999999999999716, 88.84906250086716284 ) ) ;
#25091=DIRECTION ( 'NONE',  ( -0.000000000000000000, -0.000000000000000000, 1.000000000000000000 ) ) ;
#25099=CARTESIAN_POINT ( 'NONE',  ( 94.99999999999998579, 87.33691857156068750, 89.32531250086715602 ) ) ;
#25100=CARTESIAN_POINT ( 'NONE',  ( 97.64999999999999147, 89.99999990163419739, 80.23687499810812085 ) ) ;
#25101=CARTESIAN_POINT ( 'NONE',  ( 92.69370383062498320, 88.66845928578035796, 82.71072916753378479 ) ) ;
#25112=DIRECTION ( 'NONE',  ( -0.000000000000000000, -0.000000000000000000, 1.000000000000000000 ) ) ;
#25118=CARTESIAN_POINT ( 'NONE',  ( -95.00000000000002842, 87.33691857156074434, 87.89656250086713385 ) ) ;
#25133=CARTESIAN_POINT ( 'NONE',  ( 97.30629616937498838, -209.9999999999999716, 81.22906250086715829 ) ) ;
#25137=EDGE_CURVE ( 'NONE', #40132, #68971, #39806, .T. ) ;
#25144=CARTESIAN_POINT ( 'NONE',  ( 95.00000000000000000, -207.3369185715606307, 79.48281250086715488 ) ) ;
#25149=ORIENTED_EDGE ( 'NONE', *, *, #4899, .T. ) ;
#25159=CARTESIAN_POINT ( 'NONE',  ( 96.32499999999998863, -212.2949673200287179, 84.57604166840096127 ) ) ;
#25160=CARTESIAN_POINT ( 'NONE',  ( 93.67499999999998295, 92.29496732002878900, 86.08416666666666117 ) ) ;
#25164=ORIENTED_EDGE ( 'NONE', *, *, #13890, .T. ) ;
#25166=CARTESIAN_POINT ( 'NONE',  ( -92.69370383062505425, 91.33154071421968467, 87.63197916753381378 ) ) ;
#25167=CARTESIAN_POINT ( 'NONE',  ( 96.15314808468748708, 88.00268892867053694, 81.59947916753381492 ) ) ;
#25169=CARTESIAN_POINT ( 'NONE',  ( 93.67499999999998295, 92.29496732002878900, 86.16354166840096696 ) ) ;
#25172=ORIENTED_EDGE ( 'NONE', *, *, #31795, .T. ) ;
#25177=CARTESIAN_POINT ( 'NONE',  ( -93.67500000000003979, 92.29496732002878900, 83.43833333333333258 ) ) ;
#25179=DIRECTION ( 'NONE',  ( 0.000000000000000000, 0.000000000000000000, -1.000000000000000000 ) ) ;
#25183=CARTESIAN_POINT ( 'NONE',  ( -97.30629616937497417, -208.6684592857803011, 81.96989583420048575 ) ) ;
#25186=CARTESIAN_POINT ( 'NONE',  ( -92.35000000000003695, 90.00000000000004263, 82.69749999999999091 ) ) ;
#25189=CARTESIAN_POINT ( 'NONE',  ( -97.30629616937495996, -209.9999999999999716, 89.64281250086713726 ) ) ;
#25201=CARTESIAN_POINT ( 'NONE',  ( -97.30629616937501680, 91.33154071421968467, 89.74864583420048803 ) ) ;
#25209=CARTESIAN_POINT ( 'NONE',  ( -96.32499999999996021, -212.2949673200287179, 84.47020833506762472 ) ) ;
#25213=CARTESIAN_POINT ( 'NONE',  ( 97.64999999999993463, -211.5299782133524786, 77.56458333333333144 ) ) ;
#25217=CARTESIAN_POINT ( 'NONE',  ( -96.32499999999996021, -212.2949673200287179, 86.93083333333332519 ) ) ;
#25219=VECTOR ( 'NONE', #65725, 1000.000000000000000 ) ;
#25233=CARTESIAN_POINT ( 'NONE',  ( 92.69370383062501162, -211.3315407142195852, 82.71072916753378479 ) ) ;
#25237=CARTESIAN_POINT ( 'NONE',  ( 95.00000000000000000, -212.6630814284392557, 88.69031250086716511 ) ) ;
#25240=CARTESIAN_POINT ( 'NONE',  ( -97.65000000000003411, -211.5299782133524502, 80.52791666666665549 ) ) ;
#25241=ORIENTED_EDGE ( 'NONE', *, *, #56544, .T. ) ;
#25243=CARTESIAN_POINT ( 'NONE',  ( -97.30629616937501680, 91.33154071421968467, 76.41364583420049428 ) ) ;
#25244=ORIENTED_EDGE ( 'NONE', *, *, #29877, .T. ) ;
#25256=AXIS2_PLACEMENT_3D ( 'NONE', #54956, #9095, #55329 ) ;
#25260=CARTESIAN_POINT ( 'NONE',  ( 92.69370383062501162, -209.9999999999999716, 78.84781250086714977 ) ) ;
#25264=ORIENTED_EDGE ( 'NONE', *, *, #15039, .T. ) ;
#25265=CARTESIAN_POINT ( 'NONE',  ( -97.64999999999994884, -209.9999831677324664, 78.64937441956425346 ) ) ;
#25271=CARTESIAN_POINT ( 'NONE',  ( -96.15314808468745866, -211.9973110713294489, 82.12864583420046927 ) ) ;
#25272=CARTESIAN_POINT ( 'NONE',  ( -92.69370383062502583, 91.33154071421968467, 80.01197916753380923 ) ) ;
#25275=CARTESIAN_POINT ( 'NONE',  ( 93.84685191531248449, 88.00268892867053694, 79.58864583420047722 ) ) ;
#25277=CARTESIAN_POINT ( 'NONE',  ( 94.99999999999998579, 93.05995642670504253, 78.49062500173430124 ) ) ;
#25279=CARTESIAN_POINT ( 'NONE',  ( -93.67499999999998295, -212.2949673200287179, 83.30604166840096525 ) ) ;
#25282=CARTESIAN_POINT ( 'NONE',  ( -97.30629616937497417, -208.6684592857803295, 83.87489583420047268 ) ) ;
#25284=LINE ( 'NONE', #66968, #52302 ) ;
#25290=CARTESIAN_POINT ( 'NONE',  ( -95.84368202074679743, 85.30516711421526566, 74.84535815546854565 ) ) ;
#25293=CARTESIAN_POINT ( 'NONE',  ( -93.84685191531254134, 91.99731107132950569, 86.89114583420047211 ) ) ;
#25294=CARTESIAN_POINT ( 'NONE',  ( -97.51367041768831712, -210.0000000000000284, 74.91808492278045151 ) ) ;
#25298=CARTESIAN_POINT ( 'NONE',  ( -93.84685191531252713, 88.00268892867056536, 75.24947916753380639 ) ) ;
#25300=EDGE_CURVE ( 'NONE', #71848, #67219, #48084, .T. ) ;
#25307=CARTESIAN_POINT ( 'NONE',  ( -92.69370383062498320, -211.3315407142195852, 83.71614583420050337 ) ) ;
#25309=( BOUNDED_CURVE ( )  B_SPLINE_CURVE ( 2, ( #44840, #16627, #68131, #21510, #15135, #72636, #38821 ),
 .UNSPECIFIED., .F., .F. ) 
 B_SPLINE_CURVE_WITH_KNOTS ( ( 3, 2, 2, 3 ),
 ( 0.7916666666666669627, 0.7986111111111114935, 0.8055555555555558023, 0.8125000000000002220 ),
 .UNSPECIFIED. ) 
 CURVE ( )  GEOMETRIC_REPRESENTATION_ITEM ( )  RATIONAL_B_SPLINE_CURVE ( ( 0.9999999999999935607, 0.8660254037844451469, 1.000000000000000000, 0.8660254037844387076, 1.000000000000000000, 0.8660254037844343777, 1.000000000000004219 ) ) 
 REPRESENTATION_ITEM ( '' )  );
#25312=CARTESIAN_POINT ( 'NONE',  ( -97.30629616937495996, -209.9999999999999716, 75.83156250086716454 ) ) ;
#25315=FACE_OUTER_BOUND ( 'NONE', #49360, .T. ) ;
#25322=CARTESIAN_POINT ( 'NONE',  ( 96.15314808468748708, -208.0026889286704943, 74.82614583420047438 ) ) ;
#25325=EDGE_CURVE ( 'NONE', #44494, #52144, #47486, .T. ) ;
#25333=VERTEX_POINT ( 'NONE', #4842 ) ;
#25334=ORIENTED_EDGE ( 'NONE', *, *, #24955, .T. ) ;
#25340=CARTESIAN_POINT ( 'NONE',  ( 97.30629616937498838, 91.33154071421968467, 81.28197916753381946 ) ) ;
#25341=FACE_BOUND ( 'NONE', #19211, .T. ) ;
#25342=CARTESIAN_POINT ( 'NONE',  ( -95.00000000000002842, 86.94004357329504273, 85.07875000000001364 ) ) ;
#25343=ORIENTED_EDGE ( 'NONE', *, *, #54013, .T. ) ;
#25352=CARTESIAN_POINT ( 'NONE',  ( -94.70223316839030758, 92.36156954995054491, 74.83035915144986916 ) ) ;
#25357=CARTESIAN_POINT ( 'NONE',  ( -97.64999999999994884, -211.5299782133524502, 74.89229166840097207 ) ) ;
#25358=CARTESIAN_POINT ( 'NONE',  ( -97.30629616937501680, 91.33154071421968467, 88.47864583420047779 ) ) ;
#25361=CARTESIAN_POINT ( 'NONE',  ( 92.34999999999999432, 91.52997821335252127, 75.42145833506764063 ) ) ;
#25362=CARTESIAN_POINT ( 'NONE',  ( -93.67500000000003979, 87.70503267997129626, 76.95604166840095672 ) ) ;
#25364=CARTESIAN_POINT ( 'NONE',  ( 96.15314808468748708, 91.99731107132950569, 76.88989583420048746 ) ) ;
#25365=FACE_OUTER_BOUND ( 'NONE', #30633, .T. ) ;
#25374=DIRECTION ( 'NONE',  ( 0.000000000000000000, 0.000000000000000000, -1.000000000000000000 ) ) ;
#25399=CARTESIAN_POINT ( 'NONE',  ( 96.15314808468748708, 88.00268892867053694, 85.56822916753381492 ) ) ;
#25400=CARTESIAN_POINT ( 'NONE',  ( -96.15314808468747287, -208.0026889286704943, 86.52072916753382970 ) ) ;
#25401=CARTESIAN_POINT ( 'NONE',  ( 96.32499999999998863, -212.2949673200287179, 83.94104166840097037 ) ) ;
#25405=CARTESIAN_POINT ( 'NONE',  ( -93.67499999999998295, -212.2949673200287179, 82.59166666666665435 ) ) ;
#25406=CARTESIAN_POINT ( 'NONE',  ( -97.30629616937501680, 88.66845928578038638, 76.36072916753381890 ) ) ;
#25409=CARTESIAN_POINT ( 'NONE',  ( 97.30629616937498838, -208.6684592857803011, 84.29822916753380468 ) ) ;
#25411=AXIS2_PLACEMENT_3D ( 'NONE', #8150, #65677, #31813 ) ;
#25415=EDGE_CURVE ( 'NONE', #55326, #49491, #5576, .T. ) ;
#25423=CARTESIAN_POINT ( 'NONE',  ( 93.84685191531249870, -208.0026889286704943, 78.26572916753382003 ) ) ;
#25425=DIRECTION ( 'NONE',  ( -0.000000000000000000, -0.000000000000000000, 1.000000000000000000 ) ) ;
#25426=CARTESIAN_POINT ( 'NONE',  ( 92.35000000000000853, -209.9999999999999716, 80.47499999999999432 ) ) ;
#25429=CARTESIAN_POINT ( 'NONE',  ( 93.67500000000001137, -207.7050326799711968, 82.90916666666666401 ) ) ;
#25433=VERTEX_POINT ( 'NONE', #61591 ) ;
#25434=CARTESIAN_POINT ( 'NONE',  ( -97.30629616937501680, 91.33154071421968467, 83.39864583420050792 ) ) ;
#25435=CARTESIAN_POINT ( 'NONE',  ( -92.34999999999999432, -209.9999999999999716, 76.98250000000000171 ) ) ;
#25437=CARTESIAN_POINT ( 'NONE',  ( 96.32499999999997442, 92.29496732002878900, 76.45333333333333314 ) ) ;
#25439=CARTESIAN_POINT ( 'NONE',  ( -94.99999999999997158, -206.9400435732949575, 84.84062500173429555 ) ) ;
#25443=CARTESIAN_POINT ( 'NONE',  ( -97.65000000000001990, 90.00000000000004263, 86.90437500173429441 ) ) ;
#25444=CARTESIAN_POINT ( 'NONE',  ( 96.15314808468748708, 91.99731107132950569, 87.68489583420048916 ) ) ;
#25447=CARTESIAN_POINT ( 'NONE',  ( -92.34999999999999432, -208.4700217866474645, 78.38479166840096468 ) ) ;
#25450=EDGE_CURVE ( 'NONE', #58350, #47426, #3795, .T. ) ;
#25452=ORIENTED_EDGE ( 'NONE', *, *, #29175, .T. ) ;
#25460=EDGE_CURVE ( 'NONE', #17976, #2629, #6309, .T. ) ;
#25462=CARTESIAN_POINT ( 'NONE',  ( 2.499999999999979572, -90.00000000000000000, -310.0000000000000000 ) ) ;
#25465=CARTESIAN_POINT ( 'NONE',  ( -92.69370383062498320, -209.9999999999999716, 83.13406250086715943 ) ) ;
#25472=VECTOR ( 'NONE', #60255, 1000.000000000000000 ) ;
#25474=CARTESIAN_POINT ( 'NONE',  ( 93.84685191531248449, 91.99731107132950569, 82.55197916753380127 ) ) ;
#25483=CARTESIAN_POINT ( 'NONE',  ( -95.00000000000002842, 92.66308142843932671, 87.57906250086713840 ) ) ;
#25491=CARTESIAN_POINT ( 'NONE',  ( 26.49955575014745079, 0.001194404164630089764, -64.00000000000000000 ) ) ;
#25494=CARTESIAN_POINT ( 'NONE',  ( 97.30629616937498838, -209.9999999999999716, 80.59406250086715318 ) ) ;
#25496=ORIENTED_EDGE ( 'NONE', *, *, #13291, .T. ) ;
#25500=CYLINDRICAL_SURFACE ( 'NONE', #38949, 3.299999999999969624 ) ;
#25502=( BOUNDED_CURVE ( )  B_SPLINE_CURVE ( 2, ( #35851, #1697, #46408, #34759, #69334, #24226, #953 ),
 .UNSPECIFIED., .F., .F. ) 
 B_SPLINE_CURVE_WITH_KNOTS ( ( 3, 2, 2, 3 ),
 ( 0.6773535682752291898, 0.6844092574655884498, 0.6914650230064715020, 0.6985206468843497829 ),
 .UNSPECIFIED. ) 
 CURVE ( )  GEOMETRIC_REPRESENTATION_ITEM ( )  RATIONAL_B_SPLINE_CURVE ( ( 0.9999971005499384002, 0.8660268535251571809, 1.000000000000000000, 0.8660254037844387076, 1.000000000000000000, 0.8660280936759529036, 0.9999946203249847620 ) ) 
 REPRESENTATION_ITEM ( '' )  );
#25505=CARTESIAN_POINT ( 'NONE',  ( 95.00000000000000000, -207.3369185715606307, 75.03781250086714749 ) ) ;
#25516=CARTESIAN_POINT ( 'NONE',  ( 97.64999999999999147, -209.9999999999999716, 82.77687500173431090 ) ) ;
#25517=CARTESIAN_POINT ( 'NONE',  ( 92.34999999999999432, 91.52997821335252127, 83.59708333333334451 ) ) ;
#25523=CARTESIAN_POINT ( 'NONE',  ( -97.30629616937501680, 90.00000000000004263, 86.62656250086715204 ) ) ;
#25524=CARTESIAN_POINT ( 'NONE',  ( 97.30629616937498838, 90.00000000000002842, 81.07031250086714635 ) ) ;
#25526=CARTESIAN_POINT ( 'NONE',  ( 96.32499999999998863, 87.70503267997126784, 83.94104166840097037 ) ) ;
#25530=CARTESIAN_POINT ( 'NONE',  ( 92.35000000030107969, -209.9999754409356854, 87.53856274002261273 ) ) ;
#25533=ADVANCED_FACE ( 'NONE', ( #36336 ), #6665, .F. ) ;
#25534=ORIENTED_EDGE ( 'NONE', *, *, #33712, .T. ) ;
#25535=CARTESIAN_POINT ( 'NONE',  ( -92.35000000000003695, 90.00000000000004263, 85.87249999999998806 ) ) ;
#25538=CARTESIAN_POINT ( 'NONE',  ( -97.65000000000001990, 91.52997821335253548, 83.59708333333334451 ) ) ;
#25540=CARTESIAN_POINT ( 'NONE',  ( 97.30629616937497417, 90.27617560457109391, 74.79348190356854786 ) ) ;
#25544=CARTESIAN_POINT ( 'NONE',  ( -92.69370383062498320, -211.3315407142195852, 78.47739583420047893 ) ) ;
#25545=EDGE_CURVE ( 'NONE', #68971, #73338, #11455, .T. ) ;
#25558=CARTESIAN_POINT ( 'NONE',  ( 97.65000000000000568, 88.47002178664752137, 86.53395833506763779 ) ) ;
#25560=CARTESIAN_POINT ( 'NONE',  ( -96.15314808468751551, 88.00268892867056536, 76.41364583420048007 ) ) ;
#25569=CARTESIAN_POINT ( 'NONE',  ( 94.99999999999998579, 92.66308142843932671, 89.00781250086716057 ) ) ;
#25572=EDGE_CURVE ( 'NONE', #6029, #7101, #18308, .T. ) ;
#25575=CARTESIAN_POINT ( 'NONE',  ( 97.64999999999999147, 90.00000000000002842, 86.50750000000000739 ) ) ;
#25576=CARTESIAN_POINT ( 'NONE',  ( -92.34999999999999432, -209.9999999999999716, 87.77749999999998920 ) ) ;
#25581=( LENGTH_UNIT ( ) NAMED_UNIT ( * ) SI_UNIT ( .MILLI., .METRE. ) );
#25582=CARTESIAN_POINT ( 'NONE',  ( -93.67500000000003979, 92.29496732002878900, 84.70833333333332860 ) ) ;
#25583=EDGE_LOOP ( 'NONE', ( #2279, #43858, #29037, #54963, #61403 ) ) ;
#25585=CARTESIAN_POINT ( 'NONE',  ( -2.500000000000015543, -73.00000000000001421, -255.0000000000000000 ) ) ;
#25588=CARTESIAN_POINT ( 'NONE',  ( 92.69370383062501162, -211.3315407142195852, 82.07572916753382231 ) ) ;
#25589=CARTESIAN_POINT ( 'NONE',  ( 97.30629616937498838, -209.9999999999999716, 89.48406250086715374 ) ) ;
#25596=CARTESIAN_POINT ( 'NONE',  ( -93.84685191531254134, 91.99731107132950569, 75.61989583420049144 ) ) ;
#25598=ORIENTED_EDGE ( 'NONE', *, *, #1742, .T. ) ;
#25616=CARTESIAN_POINT ( 'NONE',  ( 96.15314808468748708, -208.0026889286704943, 78.00114583420048575 ) ) ;
#25618=CARTESIAN_POINT ( 'NONE',  ( -93.67500000000003979, 92.29496732002878900, 83.43833333333333258 ) ) ;
#25623=CARTESIAN_POINT ( 'NONE',  ( -97.64999999989191792, -209.9999848944890175, 78.64888723590522090 ) ) ;
#25627=DIRECTION ( 'NONE',  ( 1.000000000000000000, 0.000000000000000000, 0.000000000000000000 ) ) ;
#25629=CARTESIAN_POINT ( 'NONE',  ( -97.51367041768835975, 89.99999999999990052, 74.91808492278043730 ) ) ;
#25630=CARTESIAN_POINT ( 'NONE',  ( -96.15314808468745866, -211.9973110713294489, 79.58864583420047722 ) ) ;
#25631=CARTESIAN_POINT ( 'NONE',  ( -96.15314808468752972, 91.99731107132950569, 80.17072916753382117 ) ) ;
#25633=CARTESIAN_POINT ( 'NONE',  ( 93.84685191531248449, 88.00268892867053694, 80.85864583420047325 ) ) ;
#25634=ORIENTED_EDGE ( 'NONE', *, *, #48798, .F. ) ;
#25641=CARTESIAN_POINT ( 'NONE',  ( -92.69370383062498320, -208.6684592857803295, 81.75822916753381264 ) ) ;
#25649=CARTESIAN_POINT ( 'NONE',  ( -97.65000000000001990, 90.00000000000004263, 75.39499999999999602 ) ) ;
#25651=DIRECTION ( 'NONE',  ( -0.000000000000000000, -0.000000000000000000, 1.000000000000000000 ) ) ;
#25653=CARTESIAN_POINT ( 'NONE',  ( -92.69370383062502583, 91.33154071421968467, 83.66322916753379957 ) ) ;
#25658=LINE ( 'NONE', #58391, #26023 ) ;
#25667=CARTESIAN_POINT ( 'NONE',  ( -92.69370383062498320, -211.3315407142195852, 81.17614583420048291 ) ) ;
#25669=CARTESIAN_POINT ( 'NONE',  ( 2.499999999999984457, -73.00000000000001421, -204.9999999999999716 ) ) ;
#25670=AXIS2_PLACEMENT_3D ( 'NONE', #37996, #44764, #60930 ) ;
#25674=CARTESIAN_POINT ( 'NONE',  ( -97.64999999999993463, 88.47002178664749295, 88.78291666666667936 ) ) ;
#25680=FACE_OUTER_BOUND ( 'NONE', #20527, .T. ) ;
#25681=CARTESIAN_POINT ( 'NONE',  ( 97.30629616937497417, -210.9303297190751891, 74.68334033237940162 ) ) ;
#25682=ORIENTED_EDGE ( 'NONE', *, *, #63826, .T. ) ;
#25691=ORIENTED_EDGE ( 'NONE', *, *, #38020, .F. ) ;
#25700=ORIENTED_EDGE ( 'NONE', *, *, #25325, .F. ) ;
#25701=CARTESIAN_POINT ( 'NONE',  ( 94.99999999999998579, 87.33691857156068750, 79.16531250086715943 ) ) ;
#25709=ORIENTED_EDGE ( 'NONE', *, *, #44665, .F. ) ;
#25713=CARTESIAN_POINT ( 'NONE',  ( -97.42291288542705274, 90.60195399605305511, 74.90604073465185309 ) ) ;
#25715=CARTESIAN_POINT ( 'NONE',  ( -96.32499999999996021, -207.7050326799711968, 84.25854166840096582 ) ) ;
#25718=CARTESIAN_POINT ( 'NONE',  ( -92.34999999999999432, -211.5299782133524502, 77.00895833506763211 ) ) ;
#25719=CARTESIAN_POINT ( 'NONE',  ( -92.69370383062504004, 90.00000000000004263, 89.48406250086715374 ) ) ;
#25720=CARTESIAN_POINT ( 'NONE',  ( 97.64999999999999147, 90.00000000000002842, 75.15687500173430635 ) ) ;
#25721=CARTESIAN_POINT ( 'NONE',  ( -96.15314808468751551, 88.00268892867056536, 89.11364583420048291 ) ) ;
#25724=CARTESIAN_POINT ( 'NONE',  ( 97.30629616937498838, 90.00000000000002842, 75.51406250086715488 ) ) ;
#25733=CARTESIAN_POINT ( 'NONE',  ( -92.35000000000000853, -211.5299782133524218, 80.10458333333330927 ) ) ;
#25742=DIRECTION ( 'NONE',  ( -0.000000000000000000, -0.000000000000000000, -1.000000000000000000 ) ) ;
#25746=CARTESIAN_POINT ( 'NONE',  ( -94.99999999999997158, -212.6630814284392557, 75.35531250086715715 ) ) ;
#25747=( BOUNDED_CURVE ( )  B_SPLINE_CURVE ( 2, ( #46107, #17525, #51361, #67927, #22816, #62680, #5528 ),
 .UNSPECIFIED., .F., .F. ) 
 B_SPLINE_CURVE_WITH_KNOTS ( ( 3, 2, 2, 3 ),
 ( 0.7408554641864709689, 0.7479111473335299243, 0.7549669128744133095, 0.7620226289464456793 ),
 .UNSPECIFIED. ) 
 CURVE ( )  GEOMETRIC_REPRESENTATION_ITEM ( )  RATIONAL_B_SPLINE_CURVE ( ( 0.9999968710551943030, 0.8660269682751109421, 1.000000000000000000, 0.8660254037844387076, 1.000000000000000000, 0.8660263430970207565, 0.9999981213880071440 ) ) 
 REPRESENTATION_ITEM ( '' )  );
#25761=CARTESIAN_POINT ( 'NONE',  ( 94.99999999999998579, 87.33691857156068750, 84.24531250086717193 ) ) ;
#25762=CARTESIAN_POINT ( 'NONE',  ( -93.84685191531247028, -211.9973110713294489, 84.29822916753381890 ) ) ;
#25766=CARTESIAN_POINT ( 'NONE',  ( -96.32499999999996021, -212.2949673200287179, 79.31083333333333485 ) ) ;
#25769=CARTESIAN_POINT ( 'NONE',  ( 97.30629616937498838, -211.3315407142195852, 84.82739583420045903 ) ) ;
#25776=ORIENTED_EDGE ( 'NONE', *, *, #38167, .F. ) ;
#25780=ORIENTED_EDGE ( 'NONE', *, *, #52053, .T. ) ;
#25782=CARTESIAN_POINT ( 'NONE',  ( 93.84685191531249870, -208.0026889286704943, 79.53572916753381605 ) ) ;
#25783=ADVANCED_FACE ( 'NONE', ( #28015 ), #44958, .F. ) ;
#25790=CARTESIAN_POINT ( 'NONE',  ( 92.35000000000000853, -209.9999999999999716, 79.83999999999998920 ) ) ;
#25797=CARTESIAN_POINT ( 'NONE',  ( -96.15314808468752972, 91.99731107132950569, 82.71072916753381321 ) ) ;
#25798=CARTESIAN_POINT ( 'NONE',  ( 96.32499999999998863, 87.70503267997126784, 88.38604166840097776 ) ) ;
#25802=VERTEX_POINT ( 'NONE', #22774 ) ;
#25803=CARTESIAN_POINT ( 'NONE',  ( -92.34999999999999432, -211.5299782133524502, 85.26395833506762756 ) ) ;
#25808=CARTESIAN_POINT ( 'NONE',  ( -97.65000000000001990, 90.00000000000004263, 84.99937500173429328 ) ) ;
#25810=CARTESIAN_POINT ( 'NONE',  ( 94.99999999999998579, 87.33691857156068750, 86.78531250086716398 ) ) ;
#25821=ORIENTED_EDGE ( 'NONE', *, *, #37684, .T. ) ;
#25827=CARTESIAN_POINT ( 'NONE',  ( -97.30629616937495996, -209.9999999999999716, 85.35656250086715602 ) ) ;
#25833=CARTESIAN_POINT ( 'NONE',  ( -92.34999999999999432, -209.9999999999999716, 90.00000000000000000 ) ) ;
#25836=CARTESIAN_POINT ( 'NONE',  ( 94.99999999999998579, 92.66308142843932671, 79.32406250086714294 ) ) ;
#25841=CARTESIAN_POINT ( 'NONE',  ( 92.57708711457300410, 90.60195399605306932, 74.90604073465190993 ) ) ;
#25844=DIRECTION ( 'NONE',  ( 1.343011723336882952E-16, -1.000000000000000000, 0.000000000000000000 ) ) ;
#25849=CARTESIAN_POINT ( 'NONE',  ( -92.69370383062505425, 88.66845928578038638, 82.28739583420048120 ) ) ;
#25850=DIRECTION ( 'NONE',  ( 1.343011723336883198E-16, -1.000000000000000000, 0.000000000000000000 ) ) ;
#25853=VERTEX_POINT ( 'NONE', #74254 ) ;
#25856=FACE_OUTER_BOUND ( 'NONE', #32047, .T. ) ;
#25858=AXIS2_PLACEMENT_3D ( 'NONE', #1718, #18589, #58827 ) ;
#25859=CARTESIAN_POINT ( 'NONE',  ( 97.30629616937498838, -211.3315407142195852, 79.27114583420048177 ) ) ;
#25872=CARTESIAN_POINT ( 'NONE',  ( 97.30629616937498838, -208.6684592857803011, 75.56697916753383026 ) ) ;
#25873=EDGE_CURVE ( 'NONE', #63717, #2629, #5340, .T. ) ;
#25882=VECTOR ( 'NONE', #20931, 1000.000000000000000 ) ;
#25885=CARTESIAN_POINT ( 'NONE',  ( 96.32499999999998863, -207.7050326799711968, 83.51770833506763836 ) ) ;
#25886=CARTESIAN_POINT ( 'NONE',  ( 94.99999999999998579, 93.05995642670504253, 86.66624999999999091 ) ) ;
#25887=ORIENTED_EDGE ( 'NONE', *, *, #59928, .T. ) ;
#25889=CARTESIAN_POINT ( 'NONE',  ( -94.99999999999997158, -213.0599564267049857, 88.96812500173430749 ) ) ;
#25894=CARTESIAN_POINT ( 'NONE',  ( -95.00000000000002842, 92.66308142843932671, 87.73781250086715033 ) ) ;
#25895=CARTESIAN_POINT ( 'NONE',  ( 97.30629616937498838, 88.66845928578037217, 82.28739583420048120 ) ) ;
#25898=CARTESIAN_POINT ( 'NONE',  ( 97.64999999999999147, 90.00000000000002842, 84.04687500173430692 ) ) ;
#25903=EDGE_CURVE ( 'NONE', #47350, #23224, #54695, .T. ) ;
#25905=ORIENTED_EDGE ( 'NONE', *, *, #4426, .T. ) ;
#25909=CARTESIAN_POINT ( 'NONE',  ( -92.35000000000005116, 88.47002178664754979, 83.91458333333333997 ) ) ;
#25913=CARTESIAN_POINT ( 'NONE',  ( 92.34999999999999432, 90.00000000000002842, 88.80937500173430976 ) ) ;
#25914=ORIENTED_EDGE ( 'NONE', *, *, #34296, .F. ) ;
#25916=CARTESIAN_POINT ( 'NONE',  ( -97.30629616937495996, -209.9999999999999716, 80.11781250086713158 ) ) ;
#25917=ORIENTED_EDGE ( 'NONE', *, *, #63957, .F. ) ;
#25918=CARTESIAN_POINT ( 'NONE',  ( -0.0004442498525516064278, 0.001194404164626844313, -85.59999999999999432 ) ) ;
#25923=CARTESIAN_POINT ( 'NONE',  ( -92.34999999999999432, -209.9999999999999716, 90.00000000000000000 ) ) ;
#25924=CARTESIAN_POINT ( 'NONE',  ( 97.30629616937498838, 88.66845928578035796, 89.27239583420048064 ) ) ;
#25926=CARTESIAN_POINT ( 'NONE',  ( -92.35000000000000853, 88.47002178664753558, 87.08958333333333712 ) ) ;
#25928=CARTESIAN_POINT ( 'NONE',  ( -92.69370383062502583, 89.06967028092473981, 74.68334033237941583 ) ) ;
#25940=CARTESIAN_POINT ( 'NONE',  ( -93.67499999999998295, -207.7050326799711968, 88.51833333333333087 ) ) ;
#25945=( BOUNDED_CURVE ( )  B_SPLINE_CURVE ( 2, ( #72340, #56554, #73447, #66711, #21952, #4315, #56165 ),
 .UNSPECIFIED., .F., .F. ) 
 B_SPLINE_CURVE_WITH_KNOTS ( ( 3, 2, 2, 3 ),
 ( 0.9166666666666662966, 0.9236111111111108274, 0.9305555555555551361, 0.9374999999999995559 ),
 .UNSPECIFIED. ) 
 CURVE ( )  GEOMETRIC_REPRESENTATION_ITEM ( )  RATIONAL_B_SPLINE_CURVE ( ( 1.000000000000006439, 0.8660254037844322683, 1.000000000000000000, 0.8660254037844387076, 1.000000000000000000, 0.8660254037844472563, 0.9999999999999914513 ) ) 
 REPRESENTATION_ITEM ( '' )  );
#25956=EDGE_CURVE ( 'NONE', #9715, #14143, #44180, .T. ) ;
#25959=ORIENTED_EDGE ( 'NONE', *, *, #10383, .F. ) ;
#25960=CARTESIAN_POINT ( 'NONE',  ( 97.30629616937498838, -208.6684592857803295, 81.75822916753381264 ) ) ;
#25963=CARTESIAN_POINT ( 'NONE',  ( 95.00000000000000000, -212.6630814284392557, 86.78531250086716398 ) ) ;
#25967=CARTESIAN_POINT ( 'NONE',  ( -96.15314808468751551, 88.00268892867056536, 77.20739583420048291 ) ) ;
#25973=CARTESIAN_POINT ( 'NONE',  ( 96.32499999999998863, -212.2949673200287179, 79.41666666666665719 ) ) ;
#25981=ORIENTED_EDGE ( 'NONE', *, *, #17808, .F. ) ;
#25983=CARTESIAN_POINT ( 'NONE',  ( 95.00000000000000000, -207.3369185715606307, 79.32406250086714294 ) ) ;
#25996=CARTESIAN_POINT ( 'NONE',  ( -93.84685191531254134, 91.99731107132950569, 78.79489583420048859 ) ) ;
#25999=CARTESIAN_POINT ( 'NONE',  ( 97.30629616937498838, 91.33154071421968467, 77.94822916753381037 ) ) ;
#26006=CARTESIAN_POINT ( 'NONE',  ( -97.30629616937495996, -209.9999999999999716, 83.92781250086714806 ) ) ;
#26012=ORIENTED_EDGE ( 'NONE', *, *, #13435, .T. ) ;
#26013=CARTESIAN_POINT ( 'NONE',  ( 12.75000000000000000, -120.0000000000000000, -80.00000000000001421 ) ) ;
#26016=CARTESIAN_POINT ( 'NONE',  ( -96.15314808468752972, 91.99731107132950569, 85.09197916753380753 ) ) ;
#26018=CARTESIAN_POINT ( 'NONE',  ( 97.64999999999999147, -209.9999999999999716, 82.69749999999999091 ) ) ;
#26019=LINE ( 'NONE', #15766, #48096 ) ;
#26023=VECTOR ( 'NONE', #58774, 1000.000000000000000 ) ;
#26028=CARTESIAN_POINT ( 'NONE',  ( -97.30629616937497417, -211.3315407142195852, 82.23447916753383424 ) ) ;
#26029=CARTESIAN_POINT ( 'NONE',  ( 97.64999999999601243, 89.99999541993086893, 76.42687486206342840 ) ) ;
#26032=ADVANCED_FACE ( 'NONE', ( #251, #46066, #40414 ), #11828, .T. ) ;
#26060=EDGE_CURVE ( 'NONE', #69330, #27263, #48991, .T. ) ;
#26065=CARTESIAN_POINT ( 'NONE',  ( 92.69370383062498320, 88.66845928578037217, 75.24947916753383481 ) ) ;
#26069=ORIENTED_EDGE ( 'NONE', *, *, #46678, .F. ) ;
#26071=DIRECTION ( 'NONE',  ( -0.000000000000000000, -0.000000000000000000, 1.000000000000000000 ) ) ;
#26073=CARTESIAN_POINT ( 'NONE',  ( 92.69370383062501162, -208.6684592857803011, 87.04989583420048405 ) ) ;
#26082=CARTESIAN_POINT ( 'NONE',  ( -94.99999999999997158, -206.9400435732949575, 76.58562500173430010 ) ) ;
#26083=CARTESIAN_POINT ( 'NONE',  ( -93.84685191531254134, 91.99731107132950569, 88.95489583420049939 ) ) ;
#26084=ORIENTED_EDGE ( 'NONE', *, *, #4247, .T. ) ;
#26085=CARTESIAN_POINT ( 'NONE',  ( 94.99999999999998579, 93.05995642670504253, 74.68062500173429896 ) ) ;
#26086=CARTESIAN_POINT ( 'NONE',  ( -93.84685191531254134, 91.99731107132950569, 88.79614583420047325 ) ) ;
#26088=CARTESIAN_POINT ( 'NONE',  ( 94.99999999999998579, 92.66308142843935514, 75.03781250086714749 ) ) ;
#26091=FACE_OUTER_BOUND ( 'NONE', #18040, .T. ) ;
#26095=CARTESIAN_POINT ( 'NONE',  ( -97.64999999999997726, -211.5299782133524502, 79.89291666666666458 ) ) ;
#26100=VECTOR ( 'NONE', #64056, 1000.000000000000000 ) ;
#26103=CARTESIAN_POINT ( 'NONE',  ( -92.35000000000005116, 91.52997821335253548, 86.00479166840096923 ) ) ;
#26104=CARTESIAN_POINT ( 'NONE',  ( 2.499999999999984457, -73.00000000000001421, -204.9999999999999716 ) ) ;
#26106=CARTESIAN_POINT ( 'NONE',  ( 97.64999999999999147, -209.9999999999999716, 89.04749999999999943 ) ) ;
#26107=EDGE_LOOP ( 'NONE', ( #60759, #74188, #11103, #56239 ) ) ;
#26108=CARTESIAN_POINT ( 'NONE',  ( -92.69370383062502583, 88.66845928578038638, 82.92239583420045790 ) ) ;
#26115=DIRECTION ( 'NONE',  ( 1.000000000000000000, 0.000000000000000000, 0.000000000000000000 ) ) ;
#26118=CARTESIAN_POINT ( 'NONE',  ( -89.99999999999998579, -124.0000000000000142, -40.00000000000002132 ) ) ;
#26123=CARTESIAN_POINT ( 'NONE',  ( 97.30629616937498838, 88.66845928578035796, 84.35114583420050849 ) ) ;
#26125=CARTESIAN_POINT ( 'NONE',  ( -94.99999999999997158, -207.3369185715606307, 83.29281250086715715 ) ) ;
#26128=CARTESIAN_POINT ( 'NONE',  ( -96.32499999999996021, -207.7050326799711968, 78.46416666666667084 ) ) ;
#26130=CARTESIAN_POINT ( 'NONE',  ( 93.84685191531249870, -208.0026889286704943, 82.55197916753380127 ) ) ;
#26138=CARTESIAN_POINT ( 'NONE',  ( 92.34999999999998010, -208.4700217866474929, 84.23208333333334963 ) ) ;
#26141=CARTESIAN_POINT ( 'NONE',  ( 96.15314808468748708, -208.0026889286704943, 76.88989583420048746 ) ) ;
#26143=CARTESIAN_POINT ( 'NONE',  ( -92.34999999999999432, -209.9999999999999716, 80.79249999999998977 ) ) ;
#26144=EDGE_CURVE ( 'NONE', #47974, #12189, #66328, .T. ) ;
#26146=( BOUNDED_CURVE ( )  B_SPLINE_CURVE ( 2, ( #68122, #4988, #44457, #44829, #15126, #38438, #27891, #50816, #32412 ),
 .UNSPECIFIED., .F., .F. ) 
 B_SPLINE_CURVE_WITH_KNOTS ( ( 3, 2, 2, 2, 3 ),
 ( 0.8043570860654228882, 0.8043572716605900119, 0.8114130372014725090, 0.8184688027423547840, 0.8255245790564498254 ),
 .UNSPECIFIED. ) 
 CURVE ( )  GEOMETRIC_REPRESENTATION_ITEM ( )  RATIONAL_B_SPLINE_CURVE ( ( 0.9999929520380519410, 0.9999964759263285652, 1.000000000000000000, 0.8660254037844387076, 1.000000000000000000, 0.8660254037844387076, 1.000000000000000000, 0.8660254037844387076, 1.000000000000000000 ) ) 
 REPRESENTATION_ITEM ( '' )  );
#26151=CARTESIAN_POINT ( 'NONE',  ( 95.00000000000000000, -213.0599564267049857, 81.26874999999999716 ) ) ;
#26152=EDGE_LOOP ( 'NONE', ( #64775, #68533, #36739, #35500 ) ) ;
#26158=CARTESIAN_POINT ( 'NONE',  ( -95.00000000000002842, 87.33691857156074434, 83.61031250086716682 ) ) ;
#26162=CARTESIAN_POINT ( 'NONE',  ( 97.64999999999999147, 90.00000000000002842, 75.71250000000000568 ) ) ;
#26167=CARTESIAN_POINT ( 'NONE',  ( -94.99999999999997158, -206.9400435732949575, 86.74562500173429669 ) ) ;
#26171=CARTESIAN_POINT ( 'NONE',  ( -96.32500000000001705, 92.29496732002878900, 82.35354166840096468 ) ) ;
#26174=CARTESIAN_POINT ( 'NONE',  ( 92.69370383062498320, 90.00000000000002842, 87.89656250086714806 ) ) ;
#26177=CARTESIAN_POINT ( 'NONE',  ( -95.00000000000002842, 86.94004357329504273, 83.88812500173429498 ) ) ;
#26182=LINE ( 'NONE', #37489, #21540 ) ;
#26185=DIRECTION ( 'NONE',  ( -1.000000000000000000, 3.061616997868382648E-16, 0.000000000000000000 ) ) ;
#26186=DIRECTION ( 'NONE',  ( -0.000000000000000000, -0.000000000000000000, 1.000000000000000000 ) ) ;
#26188=CARTESIAN_POINT ( 'NONE',  ( -93.84685191531247028, -211.9973110713294489, 85.56822916753381492 ) ) ;
#26190=FACE_OUTER_BOUND ( 'NONE', #45080, .T. ) ;
#26199=CARTESIAN_POINT ( 'NONE',  ( 93.84685191531248449, 88.00268892867053694, 79.58864583420047722 ) ) ;
#26202=CARTESIAN_POINT ( 'NONE',  ( 97.65000000000000568, 91.52997821335252127, 86.63979166840096013 ) ) ;
#26211=CARTESIAN_POINT ( 'NONE',  ( -96.32500000000001705, 87.70503267997129626, 78.12020833506763040 ) ) ;
#26214=CARTESIAN_POINT ( 'NONE',  ( -96.15314808468752972, 91.99731107132950569, 81.91697916753381037 ) ) ;
#26226=PLANE ( 'NONE',  #46719 ) ;
#26228=CARTESIAN_POINT ( 'NONE',  ( 95.00000000000000000, -212.6630814284392557, 79.80031250086715033 ) ) ;
#26229=VERTEX_POINT ( 'NONE', #20813 ) ;
#26233=EDGE_CURVE ( 'NONE', #49041, #28732, #45220, .T. ) ;
#26235=DIRECTION ( 'NONE',  ( -4.476705744456276711E-17, 1.000000000000000000, -0.000000000000000000 ) ) ;
#26236=CARTESIAN_POINT ( 'NONE',  ( 93.84685191531249870, -208.0026889286704943, 76.99572916753382401 ) ) ;
#26249=CARTESIAN_POINT ( 'NONE',  ( 95.00000000000000000, -206.9400435732949575, 81.03062500173430749 ) ) ;
#26250=CARTESIAN_POINT ( 'NONE',  ( 96.32499999999997442, 92.29496732002878900, 85.97833333333332462 ) ) ;
#26256=CARTESIAN_POINT ( 'NONE',  ( -95.00000000000002842, 92.66308142843932671, 88.37281250086715545 ) ) ;
#26257=CARTESIAN_POINT ( 'NONE',  ( 92.69370383062498320, 88.66845928578037217, 80.17072916753379275 ) ) ;
#26258=VERTEX_POINT ( 'NONE', #49743 ) ;
#26262=EDGE_LOOP ( 'NONE', ( #48076, #44551, #41257, #40395, #52796, #9709 ) ) ;
#26266=ORIENTED_EDGE ( 'NONE', *, *, #12454, .F. ) ;
#26268=CARTESIAN_POINT ( 'NONE',  ( 92.34999999999999432, 90.00000000000002842, 75.47437500173430180 ) ) ;
#26278=CARTESIAN_POINT ( 'NONE',  ( -97.30629616937497417, -208.6684592857803011, 80.69989583420048973 ) ) ;
#26283=CYLINDRICAL_SURFACE ( 'NONE', #53152, 2.649999999999985700 ) ;
#26286=B_SPLINE_CURVE_WITH_KNOTS ( 'NONE', 3,
 ( #32635, #54835, #49559, #66858, #20988, #67233, #49927, #60855 ),
 .UNSPECIFIED., .F., .F.,
 ( 4, 2, 2, 4 ),
 ( 0.001653806717455033820, 0.002539064216007439964, 0.002981692965283634471, 0.003424321714559829845 ),
 .UNSPECIFIED. ) ;
#26288=LINE ( 'NONE', #38322, #22915 ) ;
#26289=CARTESIAN_POINT ( 'NONE',  ( 96.15314808468748708, 91.99731107132950569, 86.89114583420047211 ) ) ;
#26290=CARTESIAN_POINT ( 'NONE',  ( 97.30629616937497417, -209.9999999999998863, 74.79348190356849102 ) ) ;
#26293=( BOUNDED_CURVE ( )  B_SPLINE_CURVE ( 2, ( #11688, #70305, #24112, #41389, #64694 ),
 .UNSPECIFIED., .F., .F. ) 
 B_SPLINE_CURVE_WITH_KNOTS ( ( 3, 2, 3 ),
 ( 0.9525283480321509177, 0.9595841135600021721, 0.9629953541049911525 ),
 .UNSPECIFIED. ) 
 CURVE ( )  GEOMETRIC_REPRESENTATION_ITEM ( )  RATIONAL_B_SPLINE_CURVE ( ( 1.000000000000000000, 0.8660254037844387076, 1.000000000000000000, 0.9352274998423648622, 0.9330859296547732162 ) ) 
 REPRESENTATION_ITEM ( '' )  );
#26294=CARTESIAN_POINT ( 'NONE',  ( 95.39412261730187481, -212.6434372237805803, 75.00000000000001421 ) ) ;
#26306=CARTESIAN_POINT ( 'NONE',  ( 97.30629616937498838, 88.66845928578035796, 89.43114583420049257 ) ) ;
#26310=CARTESIAN_POINT ( 'NONE',  ( -92.34999999999999432, -211.5299782133524502, 87.72458333333332803 ) ) ;
#26311=AXIS2_PLACEMENT_3D ( 'NONE', #21401, #11609, #47324 ) ;
#26317=CARTESIAN_POINT ( 'NONE',  ( 97.64999999981932888, -210.0000309431867436, 78.33187387208516839 ) ) ;
#26318=CARTESIAN_POINT ( 'NONE',  ( 92.35000000006145626, -209.9999881787626919, 81.82400613091914465 ) ) ;
#26324=ORIENTED_EDGE ( 'NONE', *, *, #25415, .F. ) ;
#26333=CARTESIAN_POINT ( 'NONE',  ( 92.69370383062501162, -208.6684592857803295, 82.60489583420049087 ) ) ;
#26334=CARTESIAN_POINT ( 'NONE',  ( 96.15314808468750130, -211.9973110713294489, 86.83822916753382515 ) ) ;
#26336=CARTESIAN_POINT ( 'NONE',  ( 92.69370383062501162, -209.9999999999999716, 85.35656250086715602 ) ) ;
#26341=CARTESIAN_POINT ( 'NONE',  ( -97.30629616937501680, 88.66845928578038638, 77.15447916753382174 ) ) ;
#26351=DIRECTION ( 'NONE',  ( -0.000000000000000000, -0.000000000000000000, 1.000000000000000000 ) ) ;
#26352=AXIS2_PLACEMENT_3D ( 'NONE', #46267, #40254, #63202 ) ;
#26355=ORIENTED_EDGE ( 'NONE', *, *, #19503, .F. ) ;
#26356=ORIENTED_EDGE ( 'NONE', *, *, #55503, .F. ) ;
#26357=CARTESIAN_POINT ( 'NONE',  ( 92.69370383062501162, -211.3315407142195852, 80.17072916753379275 ) ) ;
#26366=CARTESIAN_POINT ( 'NONE',  ( -93.84685191531252713, 88.00268892867056536, 77.94822916753382458 ) ) ;
#26368=CARTESIAN_POINT ( 'NONE',  ( 93.84685191531248449, 91.99731107132950569, 78.74197916753381321 ) ) ;
#26370=FACE_OUTER_BOUND ( 'NONE', #32247, .T. ) ;
#26375=CARTESIAN_POINT ( 'NONE',  ( -97.30629616937495996, -209.9999999999999716, 78.21281250086714465 ) ) ;
#26377=EDGE_CURVE ( 'NONE', #29550, #10929, #51862, .T. ) ;
#26383=ADVANCED_FACE ( 'NONE', ( #35063 ), #11739, .F. ) ;
#26384=ORIENTED_EDGE ( 'NONE', *, *, #70452, .F. ) ;
#26386=VECTOR ( 'NONE', #73959, 1000.000000000000000 ) ;
#26392=CARTESIAN_POINT ( 'NONE',  ( -92.69370383062502583, 88.66845928578038638, 85.46239583420047836 ) ) ;
#26395=( BOUNDED_CURVE ( )  B_SPLINE_CURVE ( 2, ( #27190, #9914, #66697, #72679, #14815, #43780, #56540 ),
 .UNSPECIFIED., .F., .F. ) 
 B_SPLINE_CURVE_WITH_KNOTS ( ( 3, 2, 2, 3 ),
 ( 0.4656806970056960315, 0.4727362912391188110, 0.4797920567800011971, 0.4868478063929146393 ),
 .UNSPECIFIED. ) 
 CURVE ( )  GEOMETRIC_REPRESENTATION_ITEM ( )  RATIONAL_B_SPLINE_CURVE ( ( 0.9999934945994508606, 0.8660286565636877709, 1.000000000000000000, 0.8660254037844387076, 1.000000000000000000, 0.8660254037844387076, 1.000000000000000000 ) ) 
 REPRESENTATION_ITEM ( '' )  );
#26403=CARTESIAN_POINT ( 'NONE',  ( -92.69370383062498320, -208.6684592857803011, 84.45697916753383083 ) ) ;
#26405=CARTESIAN_POINT ( 'NONE',  ( 94.99999999999998579, 86.94004357329502852, 76.26812500173430465 ) ) ;
#26409=PLANE ( 'NONE',  #33351 ) ;
#26411=CARTESIAN_POINT ( 'NONE',  ( -93.67499999999998295, -212.2949673200287179, 82.03604166840096923 ) ) ;
#26416=EDGE_CURVE ( 'NONE', #55326, #11224, #63212, .T. ) ;
#26418=LINE ( 'NONE', #39559, #56424 ) ;
#26420=CARTESIAN_POINT ( 'NONE',  ( 97.64999999999987779, 91.52997821335259232, 78.30541666666667311 ) ) ;
#26424=CARTESIAN_POINT ( 'NONE',  ( -96.32499999999996021, -207.7050326799711968, 87.43354166840096298 ) ) ;
#26437=VERTEX_POINT ( 'NONE', #17763 ) ;
#26438=CARTESIAN_POINT ( 'NONE',  ( 92.35000000039376289, -209.9999706925934504, 76.74344264317686282 ) ) ;
#26441=CARTESIAN_POINT ( 'NONE',  ( 93.84685191531248449, 91.99731107132950569, 78.26572916753382003 ) ) ;
#26443=CARTESIAN_POINT ( 'NONE',  ( -92.35000000000003695, 90.00000000000004263, 85.23749999999999716 ) ) ;
#26447=ORIENTED_EDGE ( 'NONE', *, *, #64244, .T. ) ;
#26448=CARTESIAN_POINT ( 'NONE',  ( 95.00000000000000000, -207.3369185715606307, 88.84906250086713442 ) ) ;
#26451=CARTESIAN_POINT ( 'NONE',  ( -97.65000000000001990, 90.00000000000004263, 77.37937500173428873 ) ) ;
#26456=CARTESIAN_POINT ( 'NONE',  ( -96.32499999999996021, -212.2949673200287179, 76.21520833506762926 ) ) ;
#26457=CARTESIAN_POINT ( 'NONE',  ( -92.69370383062502583, 91.33154071421968467, 89.53697916753382913 ) ) ;
#26459=CARTESIAN_POINT ( 'NONE',  ( 93.84685191531248449, 91.99731107132950569, 87.63197916753379957 ) ) ;
#26460=CARTESIAN_POINT ( 'NONE',  ( -92.69370383062502583, 91.33154071421968467, 87.47322916753381605 ) ) ;
#26478=CARTESIAN_POINT ( 'NONE',  ( -97.65000000000001990, 91.52997821335253548, 81.69208333333332916 ) ) ;
#26480=CARTESIAN_POINT ( 'NONE',  ( 97.64999999999999147, -209.9999999999999716, 82.69749999999999091 ) ) ;
#26487=CARTESIAN_POINT ( 'NONE',  ( -96.15314808468752972, 91.99731107132950569, 82.55197916753380127 ) ) ;
#26493=CARTESIAN_POINT ( 'NONE',  ( -92.35000000000005116, 91.52997821335254969, 78.94041666666664980 ) ) ;
#26501=EDGE_CURVE ( 'NONE', #4344, #70067, #72057, .T. ) ;
#26502=CARTESIAN_POINT ( 'NONE',  ( 93.84685191531248449, 88.00268892867053694, 79.11239583420048405 ) ) ;
#26503=CARTESIAN_POINT ( 'NONE',  ( -96.15314808468745866, -211.9973110713294489, 82.28739583420048120 ) ) ;
#26504=DIRECTION ( 'NONE',  ( -0.000000000000000000, -0.000000000000000000, 1.000000000000000000 ) ) ;
#26507=CARTESIAN_POINT ( 'NONE',  ( -96.32499999999996021, -212.2949673200287179, 78.67583333333332973 ) ) ;
#26511=CARTESIAN_POINT ( 'NONE',  ( 96.15314808468750130, -211.9973110713294489, 85.40947916753380298 ) ) ;
#26512=EDGE_LOOP ( 'NONE', ( #51884, #4777, #70607, #70331 ) ) ;
#26516=VERTEX_POINT ( 'NONE', #14345 ) ;
#26518=CARTESIAN_POINT ( 'NONE',  ( -92.35000000000005116, 88.47002178664754979, 79.54895833506762415 ) ) ;
#26520=CARTESIAN_POINT ( 'NONE',  ( 92.69370383062501162, -209.9999999999999716, 77.10156250086714635 ) ) ;
#26523=CARTESIAN_POINT ( 'NONE',  ( -95.29566955675987572, 87.37275709988156791, 74.99300273738300859 ) ) ;
#26524=CARTESIAN_POINT ( 'NONE',  ( 96.15314808468748708, 91.99731107132950569, 85.14489583420048291 ) ) ;
#26525=CARTESIAN_POINT ( 'NONE',  ( -95.00000000000002842, 90.00000000000004263, 90.00000000000000000 ) ) ;
#26526=CARTESIAN_POINT ( 'NONE',  ( 97.64999999999997726, -211.5299782133524502, 82.00958333333332462 ) ) ;
#26531=CARTESIAN_POINT ( 'NONE',  ( 93.67500000000001137, -207.7050326799711968, 89.25916666666667254 ) ) ;
#26534=CARTESIAN_POINT ( 'NONE',  ( -95.00000000000002842, 92.66308142843932671, 83.92781250086716227 ) ) ;
#26536=VECTOR ( 'NONE', #19466, 1000.000000000000000 ) ;
#26542=CARTESIAN_POINT ( 'NONE',  ( -93.67499999999998295, -212.2949673200287179, 87.11604166840096752 ) ) ;
#26547=CARTESIAN_POINT ( 'NONE',  ( -96.32500000000001705, 87.70503267997129626, 84.47020833506762472 ) ) ;
#26549=CARTESIAN_POINT ( 'NONE',  ( 97.30629616937498838, 88.66845928578037217, 87.52614583420049144 ) ) ;
#26557=CARTESIAN_POINT ( 'NONE',  ( -92.35000000000005116, 91.52997821335253548, 80.92479166840097093 ) ) ;
#26558=CYLINDRICAL_SURFACE ( 'NONE', #23928, 2.649999999999985700 ) ;
#26561=ORIENTED_EDGE ( 'NONE', *, *, #577, .F. ) ;
#26565=CARTESIAN_POINT ( 'NONE',  ( -97.30629616937495996, -209.9999999999999716, 83.45156250086715488 ) ) ;
#26566=EDGE_LOOP ( 'NONE', ( #13004, #36991, #19773, #46989 ) ) ;
#26572=LINE ( 'NONE', #49504, #25882 ) ;
#26576=CARTESIAN_POINT ( 'NONE',  ( 93.84685191531248449, 91.99731107132950569, 78.74197916753381321 ) ) ;
#26582=ADVANCED_FACE ( 'NONE', ( #47453 ), #2740, .F. ) ;
#26583=CARTESIAN_POINT ( 'NONE',  ( -92.34999999999999432, -209.9999999999999716, 87.14249999999999829 ) ) ;
#26586=LINE ( 'NONE', #72799, #56454 ) ;
#26588=ORIENTED_EDGE ( 'NONE', *, *, #71609, .F. ) ;
#26589=CARTESIAN_POINT ( 'NONE',  ( -92.69370383062505425, 88.66845928578038638, 81.65239583420047609 ) ) ;
#26595=( BOUNDED_CURVE ( )  B_SPLINE_CURVE ( 2, ( #44083, #14761, #43725, #48247, #48612, #72271, #66646 ),
 .UNSPECIFIED., .F., .F. ) 
 B_SPLINE_CURVE_WITH_KNOTS ( ( 3, 2, 2, 3 ),
 ( 0.6666666666666667407, 0.6736111111111112715, 0.6805555555555555802, 0.6875000000000000000 ),
 .UNSPECIFIED. ) 
 CURVE ( )  GEOMETRIC_REPRESENTATION_ITEM ( )  RATIONAL_B_SPLINE_CURVE ( ( 0.9999999999999978906, 0.8660254037844408170, 1.000000000000000000, 0.8660254037844387076, 1.000000000000000000, 0.8660254037844387076, 1.000000000000000000 ) ) 
 REPRESENTATION_ITEM ( '' )  );
#26600=CARTESIAN_POINT ( 'NONE',  ( 97.30629616937498838, -208.6684592857803011, 77.47197916753381719 ) ) ;
#26609=CARTESIAN_POINT ( 'NONE',  ( 92.69370383062501162, -209.9999999999999716, 77.10156250086714635 ) ) ;
#26622=CARTESIAN_POINT ( 'NONE',  ( 93.67500000000001137, -212.2949673200287179, 80.66020833506763665 ) ) ;
#26623=CARTESIAN_POINT ( 'NONE',  ( 94.99999999999998579, 93.05995642670504253, 85.39624999999998067 ) ) ;
#26632=CARTESIAN_POINT ( 'NONE',  ( -97.30629616937501680, 91.33154071421968467, 84.03364583420049883 ) ) ;
#26633=CARTESIAN_POINT ( 'NONE',  ( 92.69370383062498320, 88.66845928578037217, 82.07572916753380809 ) ) ;
#26636=EDGE_CURVE ( 'NONE', #29381, #58538, #17273, .T. ) ;
#26648=CARTESIAN_POINT ( 'NONE',  ( 97.64999999999999147, 90.00000000000002842, 88.49187500173430010 ) ) ;
#26650=DIRECTION ( 'NONE',  ( -3.061616997868383141E-16, -1.000000000000000000, 0.000000000000000000 ) ) ;
#26651=CARTESIAN_POINT ( 'NONE',  ( -94.99999999999997158, -212.6630814284392557, 80.27656250086714351 ) ) ;
#26660=CARTESIAN_POINT ( 'NONE',  ( 97.30629616937498838, 90.00000000000002842, 86.78531250086714977 ) ) ;
#26663=CARTESIAN_POINT ( 'NONE',  ( -96.32500000000001705, 92.29496732002878900, 88.70354166840097321 ) ) ;
#26673=CARTESIAN_POINT ( 'NONE',  ( 100.0010000000000900, 64.99999999999997158, -90.00000000000000000 ) ) ;
#26675=CARTESIAN_POINT ( 'NONE',  ( -97.64999999999996305, -209.9999999999999716, 84.92000000000000171 ) ) ;
#26688=CARTESIAN_POINT ( 'NONE',  ( -2.499999999999970690, 73.00000000000001421, -255.0000000000000000 ) ) ;
#26691=CARTESIAN_POINT ( 'NONE',  ( 92.69370383062501162, -209.9999999999999716, 82.02281250086714692 ) ) ;
#26692=CARTESIAN_POINT ( 'NONE',  ( 96.15314808468748708, -208.0026889286704943, 86.41489583420049314 ) ) ;
#26694=CARTESIAN_POINT ( 'NONE',  ( 92.69370383062501162, -208.6684592857803011, 86.57364583420047666 ) ) ;
#26695=EDGE_LOOP ( 'NONE', ( #3807, #44655, #69184, #52615 ) ) ;
#26698=CARTESIAN_POINT ( 'NONE',  ( -92.69370383062504004, 90.00000000000004263, 78.05406250086716113 ) ) ;
#26702=EDGE_CURVE ( 'NONE', #48244, #43660, #30385, .T. ) ;
#26708=CYLINDRICAL_SURFACE ( 'NONE', #40615, 2.649999999999999467 ) ;
#26715=CARTESIAN_POINT ( 'NONE',  ( 93.84685191531249870, -208.0026889286704943, 74.93197916753379673 ) ) ;
#26718=ORIENTED_EDGE ( 'NONE', *, *, #4074, .T. ) ;
#26723=( BOUNDED_SURFACE ( )  B_SPLINE_SURFACE ( 1, 2, ( 
 ( #49301, #72587, #3466, #43685, #56060, #37307, #66605, #61706, #10189, #32739, #33111, #21088, #55689, #32006, #44046, #50410, #4205, #8722, #15457, #15085, #73337, #31638, #48927, #38027, #27097, #44419, #32374, #50029, #67340, #55317, #21844, #65872, #71850, #20367, #51902, #63203, #50781, #63568, #57922, #22220, #45910, #57183, #33869, #68835, #10945, #17322, #16577, #12045, #5688, #29326, #40629, #46268, #74085, #6063, #62081, #45543, #51152, #22599, #444, #40255, #11665, #62464, #23342, #56815, #34605, #16204, #39895, #45161, #56443, #68467, #34987, #51529, #28222, #6425, #812, #10559, #69199, #57554, #28969, #17692, #52270, #44792, #33481, #16958, #67714, #39143, #11306, #4953, #27853, #73708, #86, #68086, #39521, #5324, #62844, #34239, #28590, #22979, #69563, #12413, #24440, #41368, #36090, #30435, #23700, #12778, #7525, #24088, #65051, #69922, #1922, #53022, #42481, #13526, #24807, #2293, #48112, #53749, #58284, #35706, #35360, #59770, #18422, #63938, #59398, #47737, #58653, #18785, #47378, #7886, #71029, #19529, #65419, #1191, #7154, #30073, #47012, #1554, #30800, #36452, #8255, #70650, #18064, #64305, #70282, #25183, #53385, #41725, #13882, #64667, #41006, #6777, #36821, #13150, #29691, #52641, #59037, #19162, #31180, #54132, #46636, #42114, #15751, #66520, #72863, #61253, #38689, #60515, #15367, #26278, #61620, #31920, #65776, #72507, #14262, #43601, #66877, #26651, #8996, #9361, #25916, #32658, #14635, #10106, #44328, #32284, #14999, #48481, #9738, #37943, #55602, #55226, #60154, #37212, #67257, #66159, #37580, #20651, #4122, #8637, #60876, #31545, #54858, #54490, #42844, #49212, #3380, #33030, #27015, #2665, #3024, #25544, #3750, #21369, #49948, #71396, #72141, #38314, #49578, #19896, #21009, #48842, #43960, #71762, #20270, #43234, #5605, #39434, #62761, #4873, #11580, #68000, #63481, #23254, #11223, #68387, #27385, #63127, #16874, #34516, #34155, #39060, #44711, #46186, #45079, #16495, #73998, #40172, #61998, #39807, #10476, #10857, #73252, #5981, #68752, #28501, #57464, #28887, #40533, #21759, #33785, #51439, #2, #22512, #11958, #17240, #69120, #57101, #51819, #33394, #67627, #22893, #16122, #45830, #365, #50327, #56358, #56737, #73623, #17605, #55972, #4488, #62380, #27773, #50700 ),
 ( #5238, #22136, #28137, #51074, #45456, #65327, #46923, #23617, #40917, #30717, #24358, #19442, #52178, #29602, #69837, #70196, #18337, #23996, #25089, #57840, #41281, #59305, #53664, #1831, #7798, #41637, #30351, #35266, #18703, #2201, #53295, #29239, #64574, #12693, #48027, #728, #6342, #52543, #34900, #35622, #46547, #52928, #6696, #63854, #69475, #29986, #17975, #24723, #13061, #35998, #64219, #58946, #1102, #70939, #12329, #7438, #58193, #58559, #7057, #47653, #19071, #1469, #47292, #70556, #42026, #64957, #13440, #42390, #36364, #9277, #20927, #54777, #66437, #49500, #66077, #71680, #72425, #8548, #37498, #55520, #26188, #43876, #8914, #44240, #25827, #2577, #19807, #9654, #3301, #72781, #31090, #31464, #48760, #49129, #20178, #2936, #4037, #36738, #43142, #38220, #32571, #55140, #61167, #20565, #32194, #14168, #72058, #26933, #3671, #8164, #43523, #14546, #49860, #54044, #59681, #54406, #14918, #66800, #60429, #15286, #26565, #31827, #37864, #60795, #21284, #13794, #25465, #48389, #42758, #71304, #65692, #37121, #60072, #5150, #56262, #16786, #33306, #39723, #38974, #11498, #28048, #51734, #63041, #68663, #22046, #28420, #10019, #67915, #73537, #44989, #74288, #68290, #34067, #10394, #22806, #4785, #57012, #38601, #62280, #44622, #4403, #16408, #34431, #73911, #50609, #57375, #51352, #27686, #21671, #5517, #10767, #33695, #39347, #5886, #45746, #62667, #17152, #56647, #45368, #40083, #50989, #22423, #28797, #61908, #11142, #277, #23170, #67168, #15671, #61538, #32937, #55888, #73166, #27297, #50231, #67541, #16032, #40831, #6610, #6970, #58113, #35179, #36282, #69030, #52457, #70475, #41932, #12970, #18981, #52845, #41554, #46462, #29892, #64871, #64493, #40448, #1385, #23901, #13352, #11860, #17515, #63770, #47203, #53212, #1010, #7356, #35907, #29518, #24276, #70115, #18617, #59221, #1749, #58857, #52094, #7717, #30631, #23527, #30268, #58475, #46840, #24636, #12241, #47569, #17883, #53576, #2119, #46098, #63394, #34813, #69756, #57751, #6255, #18253, #41195, #64134, #29156, #638, #69387, #12608, #35539, #37029, #66355, #70858, #20095, #2497, #36652, #54326, #20842, #31746, #8465, #43797, #55430, #25746, #19360, #43053, #71219, #53958, #25002, #65988, #42312, #20481, #60344, #3216, #14083 ) ),
 .UNSPECIFIED., .F., .F., .F. ) 
 B_SPLINE_SURFACE_WITH_KNOTS ( ( 2, 2 ),
 ( 3, 2, 2, 2, 2, 2, 2, 2, 2, 2, 2, 2, 2, 2, 2, 2, 2, 2, 2, 2, 2, 2, 2, 2, 2, 2, 2, 2, 2, 2, 2, 2, 2, 2, 2, 2, 2, 2, 2, 2, 2, 2, 2, 2, 2, 2, 2, 2, 2, 2, 2, 2, 2, 2, 2, 2, 2, 2, 2, 2, 2, 2, 2, 2, 2, 2, 2, 2, 2, 2, 2, 2, 2, 2, 2, 2, 2, 2, 2, 2, 2, 2, 2, 2, 2, 2, 2, 2, 2, 2, 2, 2, 2, 2, 2, 2, 2, 2, 2, 2, 2, 2, 2, 2, 2, 2, 2, 2, 2, 2, 2, 2, 2, 2, 2, 2, 2, 2, 2, 2, 2, 2, 2, 2, 2, 2, 2, 2, 2, 2, 2, 2, 2, 2, 2, 2, 2, 2, 2, 2, 2, 2, 3 ),
 ( 0.000000000000000000, 1.000000000000000000 ),
 ( 0.000000000000000000, 0.006944444444444444059, 0.01388888888888888812, 0.02083333333333333218, 0.02777777777777777624, 0.03472222222222222376, 0.04166666666666666435, 0.04861111111111111188, 0.05555555555555555247, 0.06250000000000000000, 0.06944444444444444753, 0.07638888888888889506, 0.08333333333333332871, 0.09027777777777777624, 0.09722222222222222376, 0.1041666666666666713, 0.1111111111111111049, 0.1180555555555555525, 0.1250000000000000000, 0.1319444444444444475, 0.1388888888888888951, 0.1458333333333333426, 0.1527777777777777901, 0.1597222222222222099, 0.1666666666666666574, 0.1736111111111111049, 0.1805555555555555525, 0.1875000000000000000, 0.1944444444444444475, 0.2013888888888888951, 0.2083333333333333426, 0.2152777777777777901, 0.2222222222222222099, 0.2291666666666666574, 0.2361111111111111049, 0.2430555555555555525, 0.2500000000000000000, 0.2569444444444444198, 0.2638888888888888951, 0.2708333333333333148, 0.2777777777777777901, 0.2847222222222222099, 0.2916666666666666852, 0.2986111111111111049, 0.3055555555555555802, 0.3125000000000000000, 0.3194444444444444198, 0.3263888888888888951, 0.3333333333333333148, 0.3402777777777777901, 0.3472222222222222099, 0.3541666666666666852, 0.3611111111111111049, 0.3680555555555555802, 0.3750000000000000000, 0.3819444444444444198, 0.3888888888888888951, 0.3958333333333333148, 0.4027777777777777901, 0.4097222222222222099, 0.4166666666666666852, 0.4236111111111111049, 0.4305555555555555802, 0.4375000000000000000, 0.4444444444444444198, 0.4513888888888888951, 0.4583333333333333148, 0.4652777777777777901, 0.4722222222222222099, 0.4791666666666666852, 0.4861111111111111049, 0.4930555555555555802, 0.5000000000000000000, 0.5069444444444444198, 0.5138888888888888395, 0.5208333333333333703, 0.5277777777777777901, 0.5347222222222222099, 0.5416666666666666297, 0.5486111111111111605, 0.5555555555555555802, 0.5625000000000000000, 0.5694444444444444198, 0.5763888888888888395, 0.5833333333333333703, 0.5902777777777777901, 0.5972222222222222099, 0.6041666666666666297, 0.6111111111111111605, 0.6180555555555555802, 0.6250000000000000000, 0.6319444444444444198, 0.6388888888888888395, 0.6458333333333333703, 0.6527777777777777901, 0.6597222222222222099, 0.6666666666666666297, 0.6736111111111111605, 0.6805555555555555802, 0.6875000000000000000, 0.6944444444444444198, 0.7013888888888888395, 0.7083333333333333703, 0.7152777777777777901, 0.7222222222222222099, 0.7291666666666666297, 0.7361111111111111605, 0.7430555555555555802, 0.7500000000000000000, 0.7569444444444444198, 0.7638888888888888395, 0.7708333333333333703, 0.7777777777777777901, 0.7847222222222222099, 0.7916666666666666297, 0.7986111111111111605, 0.8055555555555555802, 0.8125000000000000000, 0.8194444444444444198, 0.8263888888888888395, 0.8333333333333333703, 0.8402777777777777901, 0.8472222222222222099, 0.8541666666666666297, 0.8611111111111111605, 0.8680555555555555802, 0.8750000000000000000, 0.8819444444444444198, 0.8888888888888888395, 0.8958333333333333703, 0.9027777777777777901, 0.9097222222222222099, 0.9166666666666666297, 0.9236111111111111605, 0.9305555555555555802, 0.9375000000000000000, 0.9444444444444444198, 0.9513888888888888395, 0.9583333333333333703, 0.9652777777777777901, 0.9722222222222222099, 0.9791666666666666297, 0.9842227634901432598 ),
 .UNSPECIFIED. ) 
 GEOMETRIC_REPRESENTATION_ITEM ( )  RATIONAL_B_SPLINE_SURFACE ( (
 ( 1.000000000000000000, 0.8660254037844387076, 1.000000000000000000, 0.8660254037844387076, 1.000000000000000000, 0.8660254037844387076, 1.000000000000000000, 0.8660254037844387076, 1.000000000000000000, 0.8660254037844387076, 1.000000000000000000, 0.8660254037844387076, 1.000000000000000000, 0.8660254037844387076, 1.000000000000000000, 0.8660254037844387076, 1.000000000000000000, 0.8660254037844387076, 1.000000000000000000, 0.8660254037844387076, 1.000000000000000000, 0.8660254037844387076, 1.000000000000000000, 0.8660254037844387076, 1.000000000000000000, 0.8660254037844387076, 1.000000000000000000, 0.8660254037844387076, 1.000000000000000000, 0.8660254037844387076, 1.000000000000000000, 0.8660254037844387076, 1.000000000000000000, 0.8660254037844387076, 1.000000000000000000, 0.8660254037844387076, 1.000000000000000000, 0.8660254037844387076, 1.000000000000000000, 0.8660254037844387076, 1.000000000000000000, 0.8660254037844387076, 1.000000000000000000, 0.8660254037844387076, 1.000000000000000000, 0.8660254037844387076, 1.000000000000000000, 0.8660254037844387076, 1.000000000000000000, 0.8660254037844387076, 1.000000000000000000, 0.8660254037844387076, 1.000000000000000000, 0.8660254037844387076, 1.000000000000000000, 0.8660254037844387076, 1.000000000000000000, 0.8660254037844387076, 1.000000000000000000, 0.8660254037844387076, 1.000000000000000000, 0.8660254037844387076, 1.000000000000000000, 0.8660254037844387076, 1.000000000000000000, 0.8660254037844387076, 1.000000000000000000, 0.8660254037844387076, 1.000000000000000000, 0.8660254037844387076, 1.000000000000000000, 0.8660254037844387076, 1.000000000000000000, 0.8660254037844387076, 1.000000000000000000, 0.8660254037844387076, 1.000000000000000000, 0.8660254037844387076, 1.000000000000000000, 0.8660254037844387076, 1.000000000000000000, 0.8660254037844387076, 1.000000000000000000, 0.8660254037844387076, 1.000000000000000000, 0.8660254037844387076, 1.000000000000000000, 0.8660254037844387076, 1.000000000000000000, 0.8660254037844387076, 1.000000000000000000, 0.8660254037844387076, 1.000000000000000000, 0.8660254037844387076, 1.000000000000000000, 0.8660254037844387076, 1.000000000000000000, 0.8660254037844387076, 1.000000000000000000, 0.8660254037844387076, 1.000000000000000000, 0.8660254037844387076, 1.000000000000000000, 0.8660254037844387076, 1.000000000000000000, 0.8660254037844387076, 1.000000000000000000, 0.8660254037844387076, 1.000000000000000000, 0.8660254037844387076, 1.000000000000000000, 0.8660254037844387076, 1.000000000000000000, 0.8660254037844387076, 1.000000000000000000, 0.8660254037844387076, 1.000000000000000000, 0.8660254037844387076, 1.000000000000000000, 0.8660254037844387076, 1.000000000000000000, 0.8660254037844387076, 1.000000000000000000, 0.8660254037844387076, 1.000000000000000000, 0.8660254037844387076, 1.000000000000000000, 0.8660254037844387076, 1.000000000000000000, 0.8660254037844387076, 1.000000000000000000, 0.8660254037844387076, 1.000000000000000000, 0.8660254037844387076, 1.000000000000000000, 0.8660254037844387076, 1.000000000000000000, 0.8660254037844387076, 1.000000000000000000, 0.8660254037844387076, 1.000000000000000000, 0.8660254037844387076, 1.000000000000000000, 0.8660254037844387076, 1.000000000000000000, 0.8660254037844387076, 1.000000000000000000, 0.8660254037844387076, 1.000000000000000000, 0.8660254037844387076, 1.000000000000000000, 0.8660254037844387076, 1.000000000000000000, 0.8660254037844387076, 1.000000000000000000, 0.8660254037844387076, 1.000000000000000000, 0.8660254037844387076, 1.000000000000000000, 0.8660254037844387076, 1.000000000000000000, 0.8660254037844387076, 1.000000000000000000, 0.8660254037844387076, 1.000000000000000000, 0.8660254037844387076, 1.000000000000000000, 0.8660254037844387076, 1.000000000000000000, 0.8660254037844387076, 1.000000000000000000, 0.8660254037844387076, 1.000000000000000000, 0.8660254037844387076, 1.000000000000000000, 0.8660254037844387076, 1.000000000000000000, 0.8660254037844387076, 1.000000000000000000, 0.8660254037844387076, 1.000000000000000000, 0.8660254037844387076, 1.000000000000000000, 0.8660254037844387076, 1.000000000000000000, 0.8660254037844387076, 1.000000000000000000, 0.8660254037844387076, 1.000000000000000000, 0.8660254037844387076, 1.000000000000000000, 0.8660254037844387076, 1.000000000000000000, 0.8660254037844387076, 1.000000000000000000, 0.8660254037844387076, 1.000000000000000000, 0.8660254037844387076, 1.000000000000000000, 0.8660254037844387076, 1.000000000000000000, 0.8660254037844387076, 1.000000000000000000, 0.8660254037844387076, 1.000000000000000000, 0.8660254037844387076, 1.000000000000000000, 0.8660254037844387076, 1.000000000000000000, 0.8660254037844387076, 1.000000000000000000, 0.8660254037844387076, 1.000000000000000000, 0.8660254037844387076, 1.000000000000000000, 0.8660254037844387076, 1.000000000000000000, 0.8660254037844387076, 1.000000000000000000, 0.8660254037844387076, 1.000000000000000000, 0.8660254037844387076, 1.000000000000000000, 0.8660254037844387076, 1.000000000000000000, 0.8660254037844387076, 1.000000000000000000, 0.8660254037844387076, 1.000000000000000000, 0.8660254037844387076, 1.000000000000000000, 0.8660254037844387076, 1.000000000000000000, 0.8660254037844387076, 1.000000000000000000, 0.8660254037844387076, 1.000000000000000000, 0.8660254037844387076, 1.000000000000000000, 0.8660254037844387076, 1.000000000000000000, 0.8660254037844387076, 1.000000000000000000, 0.8660254037844387076, 1.000000000000000000, 0.8660254037844387076, 1.000000000000000000, 0.8660254037844387076, 1.000000000000000000, 0.8660254037844387076, 1.000000000000000000, 0.8660254037844387076, 1.000000000000000000, 0.8660254037844387076, 1.000000000000000000, 0.8660254037844387076, 1.000000000000000000, 0.8660254037844387076, 1.000000000000000000, 0.8660254037844387076, 1.000000000000000000, 0.8660254037844387076, 1.000000000000000000, 0.8660254037844387076, 1.000000000000000000, 0.8660254037844387076, 1.000000000000000000, 0.8660254037844387076, 1.000000000000000000, 0.8660254037844387076, 1.000000000000000000, 0.8660254037844387076, 1.000000000000000000, 0.8660254037844387076, 1.000000000000000000, 0.8660254037844387076, 1.000000000000000000, 0.8660254037844387076, 1.000000000000000000, 0.8660254037844387076, 1.000000000000000000, 0.8660254037844387076, 1.000000000000000000, 0.9024560516293040902, 0.9469512977404621612),
 ( 1.000000000000000000, 0.8660254037844387076, 1.000000000000000000, 0.8660254037844387076, 1.000000000000000000, 0.8660254037844387076, 1.000000000000000000, 0.8660254037844387076, 1.000000000000000000, 0.8660254037844387076, 1.000000000000000000, 0.8660254037844387076, 1.000000000000000000, 0.8660254037844387076, 1.000000000000000000, 0.8660254037844387076, 1.000000000000000000, 0.8660254037844387076, 1.000000000000000000, 0.8660254037844387076, 1.000000000000000000, 0.8660254037844387076, 1.000000000000000000, 0.8660254037844387076, 1.000000000000000000, 0.8660254037844387076, 1.000000000000000000, 0.8660254037844387076, 1.000000000000000000, 0.8660254037844387076, 1.000000000000000000, 0.8660254037844387076, 1.000000000000000000, 0.8660254037844387076, 1.000000000000000000, 0.8660254037844387076, 1.000000000000000000, 0.8660254037844387076, 1.000000000000000000, 0.8660254037844387076, 1.000000000000000000, 0.8660254037844387076, 1.000000000000000000, 0.8660254037844387076, 1.000000000000000000, 0.8660254037844387076, 1.000000000000000000, 0.8660254037844387076, 1.000000000000000000, 0.8660254037844387076, 1.000000000000000000, 0.8660254037844387076, 1.000000000000000000, 0.8660254037844387076, 1.000000000000000000, 0.8660254037844387076, 1.000000000000000000, 0.8660254037844387076, 1.000000000000000000, 0.8660254037844387076, 1.000000000000000000, 0.8660254037844387076, 1.000000000000000000, 0.8660254037844387076, 1.000000000000000000, 0.8660254037844387076, 1.000000000000000000, 0.8660254037844387076, 1.000000000000000000, 0.8660254037844387076, 1.000000000000000000, 0.8660254037844387076, 1.000000000000000000, 0.8660254037844387076, 1.000000000000000000, 0.8660254037844387076, 1.000000000000000000, 0.8660254037844387076, 1.000000000000000000, 0.8660254037844387076, 1.000000000000000000, 0.8660254037844387076, 1.000000000000000000, 0.8660254037844387076, 1.000000000000000000, 0.8660254037844387076, 1.000000000000000000, 0.8660254037844387076, 1.000000000000000000, 0.8660254037844387076, 1.000000000000000000, 0.8660254037844387076, 1.000000000000000000, 0.8660254037844387076, 1.000000000000000000, 0.8660254037844387076, 1.000000000000000000, 0.8660254037844387076, 1.000000000000000000, 0.8660254037844387076, 1.000000000000000000, 0.8660254037844387076, 1.000000000000000000, 0.8660254037844387076, 1.000000000000000000, 0.8660254037844387076, 1.000000000000000000, 0.8660254037844387076, 1.000000000000000000, 0.8660254037844387076, 1.000000000000000000, 0.8660254037844387076, 1.000000000000000000, 0.8660254037844387076, 1.000000000000000000, 0.8660254037844387076, 1.000000000000000000, 0.8660254037844387076, 1.000000000000000000, 0.8660254037844387076, 1.000000000000000000, 0.8660254037844387076, 1.000000000000000000, 0.8660254037844387076, 1.000000000000000000, 0.8660254037844387076, 1.000000000000000000, 0.8660254037844387076, 1.000000000000000000, 0.8660254037844387076, 1.000000000000000000, 0.8660254037844387076, 1.000000000000000000, 0.8660254037844387076, 1.000000000000000000, 0.8660254037844387076, 1.000000000000000000, 0.8660254037844387076, 1.000000000000000000, 0.8660254037844387076, 1.000000000000000000, 0.8660254037844387076, 1.000000000000000000, 0.8660254037844387076, 1.000000000000000000, 0.8660254037844387076, 1.000000000000000000, 0.8660254037844387076, 1.000000000000000000, 0.8660254037844387076, 1.000000000000000000, 0.8660254037844387076, 1.000000000000000000, 0.8660254037844387076, 1.000000000000000000, 0.8660254037844387076, 1.000000000000000000, 0.8660254037844387076, 1.000000000000000000, 0.8660254037844387076, 1.000000000000000000, 0.8660254037844387076, 1.000000000000000000, 0.8660254037844387076, 1.000000000000000000, 0.8660254037844387076, 1.000000000000000000, 0.8660254037844387076, 1.000000000000000000, 0.8660254037844387076, 1.000000000000000000, 0.8660254037844387076, 1.000000000000000000, 0.8660254037844387076, 1.000000000000000000, 0.8660254037844387076, 1.000000000000000000, 0.8660254037844387076, 1.000000000000000000, 0.8660254037844387076, 1.000000000000000000, 0.8660254037844387076, 1.000000000000000000, 0.8660254037844387076, 1.000000000000000000, 0.8660254037844387076, 1.000000000000000000, 0.8660254037844387076, 1.000000000000000000, 0.8660254037844387076, 1.000000000000000000, 0.8660254037844387076, 1.000000000000000000, 0.8660254037844387076, 1.000000000000000000, 0.8660254037844387076, 1.000000000000000000, 0.8660254037844387076, 1.000000000000000000, 0.8660254037844387076, 1.000000000000000000, 0.8660254037844387076, 1.000000000000000000, 0.8660254037844387076, 1.000000000000000000, 0.8660254037844387076, 1.000000000000000000, 0.8660254037844387076, 1.000000000000000000, 0.8660254037844387076, 1.000000000000000000, 0.8660254037844387076, 1.000000000000000000, 0.8660254037844387076, 1.000000000000000000, 0.8660254037844387076, 1.000000000000000000, 0.8660254037844387076, 1.000000000000000000, 0.8660254037844387076, 1.000000000000000000, 0.8660254037844387076, 1.000000000000000000, 0.8660254037844387076, 1.000000000000000000, 0.8660254037844387076, 1.000000000000000000, 0.8660254037844387076, 1.000000000000000000, 0.8660254037844387076, 1.000000000000000000, 0.8660254037844387076, 1.000000000000000000, 0.8660254037844387076, 1.000000000000000000, 0.8660254037844387076, 1.000000000000000000, 0.8660254037844387076, 1.000000000000000000, 0.8660254037844387076, 1.000000000000000000, 0.8660254037844387076, 1.000000000000000000, 0.8660254037844387076, 1.000000000000000000, 0.8660254037844387076, 1.000000000000000000, 0.8660254037844387076, 1.000000000000000000, 0.8660254037844387076, 1.000000000000000000, 0.8660254037844387076, 1.000000000000000000, 0.8660254037844387076, 1.000000000000000000, 0.8660254037844387076, 1.000000000000000000, 0.8660254037844387076, 1.000000000000000000, 0.8660254037844387076, 1.000000000000000000, 0.8660254037844387076, 1.000000000000000000, 0.8660254037844387076, 1.000000000000000000, 0.8660254037844387076, 1.000000000000000000, 0.8660254037844387076, 1.000000000000000000, 0.8660254037844387076, 1.000000000000000000, 0.8660254037844387076, 1.000000000000000000, 0.8660254037844387076, 1.000000000000000000, 0.8660254037844387076, 1.000000000000000000, 0.8660254037844387076, 1.000000000000000000, 0.8660254037844387076, 1.000000000000000000, 0.8660254037844387076, 1.000000000000000000, 0.9024560516293040902, 0.9469512977404621612) ) ) 
 REPRESENTATION_ITEM ( '' )  SURFACE ( )  );
#26724=DIRECTION ( 'NONE',  ( -0.000000000000000000, -0.000000000000000000, 1.000000000000000000 ) ) ;
#26725=CARTESIAN_POINT ( 'NONE',  ( -96.15314808468752972, 91.99731107132950569, 75.09072916753380866 ) ) ;
#26729=CARTESIAN_POINT ( 'NONE',  ( 92.69370383062498320, 91.33154071421968467, 78.79489583420047438 ) ) ;
#26739=CARTESIAN_POINT ( 'NONE',  ( -97.30629616937495996, -209.9999999999999716, 79.48281250086714067 ) ) ;
#26752=CARTESIAN_POINT ( 'NONE',  ( -93.84685191531252713, 88.00268892867056536, 81.59947916753381492 ) ) ;
#26756=CARTESIAN_POINT ( 'NONE',  ( 92.34999999999999432, 90.00000000000002842, 81.10999999999999943 ) ) ;
#26758=DIRECTION ( 'NONE',  ( -0.000000000000000000, -0.000000000000000000, 1.000000000000000000 ) ) ;
#26759=CARTESIAN_POINT ( 'NONE',  ( 100.0010000000000190, -123.9999999999999858, -40.00000000000002132 ) ) ;
#26761=CARTESIAN_POINT ( 'NONE',  ( -94.99999999999997158, -207.3369185715606307, 82.02281250086714692 ) ) ;
#26764=ORIENTED_EDGE ( 'NONE', *, *, #57740, .F. ) ;
#26771=CARTESIAN_POINT ( 'NONE',  ( -97.64999999999996305, -209.9999999999999716, 79.20499999999999829 ) ) ;
#26794=VERTEX_POINT ( 'NONE', #55464 ) ;
#26803=CARTESIAN_POINT ( 'NONE',  ( 97.30629616937498838, 90.00000000000002842, 75.51406250086715488 ) ) ;
#26804=CARTESIAN_POINT ( 'NONE',  ( 92.35000000045006630, -210.0000310946952595, 88.81037122969986797 ) ) ;
#26810=CARTESIAN_POINT ( 'NONE',  ( 97.30629616937498838, 90.00000000000002842, 89.32531250086714181 ) ) ;
#26811=ORIENTED_EDGE ( 'NONE', *, *, #23516, .F. ) ;
#26812=CARTESIAN_POINT ( 'NONE',  ( 93.84685191531249870, -208.0026889286704943, 85.09197916753380753 ) ) ;
#26815=DIRECTION ( 'NONE',  ( 1.000000000000000000, 0.000000000000000000, 0.000000000000000000 ) ) ;
#26820=CARTESIAN_POINT ( 'NONE',  ( -92.34999999999999432, -208.4700217866474645, 75.20979166840096752 ) ) ;
#26824=CARTESIAN_POINT ( 'NONE',  ( 96.15314808468748708, 91.99731107132950569, 88.16114583420046813 ) ) ;
#26825=CARTESIAN_POINT ( 'NONE',  ( -93.09170853947344426, 88.16127117233644128, 74.44346887015069569 ) ) ;
#26826=( BOUNDED_CURVE ( )  B_SPLINE_CURVE ( 2, ( #9610, #54730, #2889, #19400, #15241, #25046, #20519 ),
 .UNSPECIFIED., .F., .F. ) 
 B_SPLINE_CURVE_WITH_KNOTS ( ( 3, 2, 2, 3 ),
 ( 0.8466920362367552633, 0.8537476304467667143, 0.8608033959876489893, 0.8678591737214811364 ),
 .UNSPECIFIED. ) 
 CURVE ( )  GEOMETRIC_REPRESENTATION_ITEM ( )  RATIONAL_B_SPLINE_CURVE ( ( 0.9999934937104295596, 0.8660286570082199598, 1.000000000000000000, 0.8660254037844387076, 1.000000000000000000, 0.8660254037844387076, 1.000000000000000000 ) ) 
 REPRESENTATION_ITEM ( '' )  );
#26833=CARTESIAN_POINT ( 'NONE',  ( -97.30629616937495996, -209.9999999999999716, 89.64281250086713726 ) ) ;
#26835=ORIENTED_EDGE ( 'NONE', *, *, #72990, .T. ) ;
#26840=VERTEX_POINT ( 'NONE', #21611 ) ;
#26841=AXIS2_PLACEMENT_3D ( 'NONE', #11178, #57055, #44667 ) ;
#26843=CARTESIAN_POINT ( 'NONE',  ( -92.35000000000005116, 91.52997821335253548, 82.75041666666665208 ) ) ;
#26845=EDGE_CURVE ( 'NONE', #58346, #11208, #20678, .T. ) ;
#26847=CARTESIAN_POINT ( 'NONE',  ( -97.64999999999996305, -211.5299782133524218, 76.79729166840095900 ) ) ;
#26853=CARTESIAN_POINT ( 'NONE',  ( -93.84685191531254134, 91.99731107132950569, 80.54114583420046358 ) ) ;
#26856=FACE_OUTER_BOUND ( 'NONE', #5751, .T. ) ;
#26862=CARTESIAN_POINT ( 'NONE',  ( 94.99999999999998579, 87.33691857156068750, 79.80031250086715033 ) ) ;
#26864=CARTESIAN_POINT ( 'NONE',  ( -94.99999999999997158, -212.6630814284392557, 82.34031250086714238 ) ) ;
#26867=CARTESIAN_POINT ( 'NONE',  ( -92.35000000000005116, 88.47002178664754979, 87.16895833506762870 ) ) ;
#26868=CARTESIAN_POINT ( 'NONE',  ( -94.99999999999997158, -206.9400435732949575, 76.50624999999999432 ) ) ;
#26870=CARTESIAN_POINT ( 'NONE',  ( -92.69370383062505425, 88.66845928578038638, 76.73114583420048973 ) ) ;
#26871=CARTESIAN_POINT ( 'NONE',  ( 92.69370383062501162, -211.3315407142195852, 83.98072916753380923 ) ) ;
#26879=LINE ( 'NONE', #34008, #23757 ) ;
#26889=CARTESIAN_POINT ( 'NONE',  ( -96.53982248244427922, 87.90457393955784937, 74.96680960279263672 ) ) ;
#26890=CARTESIAN_POINT ( 'NONE',  ( 96.15314808468748708, 91.99731107132950569, 87.04989583420048405 ) ) ;
#26893=CARTESIAN_POINT ( 'NONE',  ( 92.35000000000002274, -208.4700217866474645, 81.05708333333333826 ) ) ;
#26895=ORIENTED_EDGE ( 'NONE', *, *, #73653, .T. ) ;
#26902=CARTESIAN_POINT ( 'NONE',  ( -97.65000000000001990, 90.00000000000004263, 81.82437500173429612 ) ) ;
#26905=EDGE_CURVE ( 'NONE', #52144, #30123, #12985, .T. ) ;
#26908=CARTESIAN_POINT ( 'NONE',  ( -97.64999999999996305, -209.9999999999999716, 85.63437500173431260 ) ) ;
#26911=DIRECTION ( 'NONE',  ( -0.000000000000000000, -0.000000000000000000, 1.000000000000000000 ) ) ;
#26914=CARTESIAN_POINT ( 'NONE',  ( -92.35000000000005116, 88.47002178664754979, 81.45395833506763950 ) ) ;
#26915=ORIENTED_EDGE ( 'NONE', *, *, #49563, .F. ) ;
#26916=CARTESIAN_POINT ( 'NONE',  ( 92.69370383062498320, 90.00000000000002842, 82.18156250086715886 ) ) ;
#26917=CARTESIAN_POINT ( 'NONE',  ( -95.00000000000002842, 86.94004357329504273, 76.18874999999999886 ) ) ;
#26919=DIRECTION ( 'NONE',  ( -0.000000000000000000, -0.000000000000000000, 1.000000000000000000 ) ) ;
#26925=ADVANCED_FACE ( 'NONE', ( #40347 ), #28684, .F. ) ;
#26928=ORIENTED_EDGE ( 'NONE', *, *, #4675, .T. ) ;
#26930=AXIS2_PLACEMENT_3D ( 'NONE', #54043, #71303, #21282 ) ;
#26933=CARTESIAN_POINT ( 'NONE',  ( -97.30629616937497417, -211.3315407142195852, 84.13947916753383538 ) ) ;
#26935=CARTESIAN_POINT ( 'NONE',  ( 93.67500000000001137, -212.2949673200287179, 81.21583333333333599 ) ) ;
#26940=CARTESIAN_POINT ( 'NONE',  ( 92.35000000000000853, -208.4700217866474645, 83.04145833506764518 ) ) ;
#26941=CARTESIAN_POINT ( 'NONE',  ( 96.15314808468748708, 88.00268892867053694, 79.05947916753380866 ) ) ;
#26954=CARTESIAN_POINT ( 'NONE',  ( -96.15314808468751551, 88.00268892867056536, 84.66864583420047552 ) ) ;
#26955=AXIS2_PLACEMENT_3D ( 'NONE', #9384, #9017, #31940 ) ;
#26960=DIRECTION ( 'NONE',  ( -0.000000000000000000, -0.000000000000000000, 1.000000000000000000 ) ) ;
#26965=EDGE_CURVE ( 'NONE', #23740, #56929, #534, .T. ) ;
#26967=CARTESIAN_POINT ( 'NONE',  ( 92.69370383062501162, -208.6684592857803011, 77.04864583420048518 ) ) ;
#26971=EDGE_CURVE ( 'NONE', #31889, #52806, #23547, .T. ) ;
#26978=CARTESIAN_POINT ( 'NONE',  ( 95.00000000000000000, -212.6630814284392557, 75.35531250086715715 ) ) ;
#26987=CARTESIAN_POINT ( 'NONE',  ( 92.35000000000000853, -209.9999999999999716, 79.28437500173430408 ) ) ;
#26988=CARTESIAN_POINT ( 'NONE',  ( 92.34999999999999432, 90.00000000000002842, 82.37999999999999545 ) ) ;
#26997=CARTESIAN_POINT ( 'NONE',  ( -92.69370383062505425, 91.33154071421968467, 83.18697916753382060 ) ) ;
#26999=CARTESIAN_POINT ( 'NONE',  ( 93.84685191531248449, 91.99731107132950569, 80.01197916753380923 ) ) ;
#27003=ORIENTED_EDGE ( 'NONE', *, *, #74059, .T. ) ;
#27006=CARTESIAN_POINT ( 'NONE',  ( -97.30629616937495996, -209.9999999999999716, 82.02281250086714692 ) ) ;
#27008=EDGE_LOOP ( 'NONE', ( #63288, #14780, #19431, #64485 ) ) ;
#27010=CARTESIAN_POINT ( 'NONE',  ( 92.34999999999993747, 91.52997821335250705, 79.15208333333333712 ) ) ;
#27012=CARTESIAN_POINT ( 'NONE',  ( -97.64999999947046661, -209.9999663481462164, 81.18829462297327382 ) ) ;
#27015=CARTESIAN_POINT ( 'NONE',  ( -93.84685191531248449, -208.0026889286704943, 78.63614583420047666 ) ) ;
#27021=AXIS2_PLACEMENT_3D ( 'NONE', #70546, #1456, #19059 ) ;
#27024=CARTESIAN_POINT ( 'NONE',  ( 95.00000000000000000, -206.9400435732949575, 82.30062500173427509 ) ) ;
#27025=CARTESIAN_POINT ( 'NONE',  ( 97.30629616937498838, 91.33154071421968467, 88.10822916753380696 ) ) ;
#27028=CARTESIAN_POINT ( 'NONE',  ( -92.35000000005469190, 89.99998298270445218, 88.49187441316097136 ) ) ;
#27032=( BOUNDED_SURFACE ( )  B_SPLINE_SURFACE ( 1, 2, ( 
 ( #58385, #73913, #7263, #62670, #59136, #18889, #29800, #64042, #44991, #30177, #12516, #53121, #1297, #33697, #39349, #41834, #39725, #12146, #69668, #50991, #24186, #50611, #67918, #22426, #1660, #64780, #35453, #24543, #35092, #58017, #47481, #70385, #47121, #70021, #13262, #16410, #36194, #918, #18526, #41467, #62283, #45370, #10769, #68293, #64407, #16788, #6522, #29426, #23806, #46747, #18166, #41109, #25293, #66261, #32022, #14374, #30909, #71871, #2403, #8739, #59882, #49315, #20386, #14735, #72246, #20749, #48221, #48940, #60619, #2026, #36930, #71132, #70766, #37686, #31652, #8370, #31286, #54959, #3482, #26392, #43699, #66621, #7992, #15103, #42957, #9100, #26016, #43341, #37320, #60257, #65891, #24910, #38045, #54599, #60973, #3124, #13624, #19267, #30541, #19634, #42579, #48589, #36553, #53489, #47841, #42223, #59505, #65155, #53855, #65518, #13990, #54240, #2767, #25653, #71500, #19999, #16219, #45560, #32392, #33886, #10207, #27871, #39162, #39534, #38420, #21107, #55333, #62096, #56831, #55707, #3851, #72601, #33130, #27114, #10958, #4221, #45178, #5336, #67732, #9842, #50796, #50047, #10571, #38789, #28234, #73722, #68102, #51169, #74100, #72972, #22237, #62483, #26752, #15857, #21478, #49677, #16590, #33499, #61722, #56077, #22612, #68484, #16972, #39912, #9466, #61356, #44060, #21862, #66977, #4968, #15477, #56464, #32756, #44441, #67354, #27496, #4593, #50433, #73353, #44806, #11320, #63954, #35001, #35722, #62861, #47027, #51547, #12429, #11678, #69214, #47394, #41381, #30089, #45926, #1571, #52285, #58667, #69936, #68853, #46283, #18439, #34620, #57936, #40269, #17337, #34251, #101, #29342, #52654, #35373, #17704, #69579, #57571, #64318, #461, #70295, #53034, #6080, #28602, #24101, #41019, #40640, #63589, #12794, #7172, #24456, #18801, #57196, #63217, #5704, #830, #22991, #58299, #6794, #46648, #29707, #28981, #1207, #6439, #51915, #23356, #12063, #18082, #23716, #54148, #71043, #31563, #41742, #37228, #30452, #25560, #42133, #2306, #43252, #8650, #48856, #24824, #20284, #13897, #3039, #14278, #47751, #30819, #60171, #65065, #19544, #70665, #19181, #13170, #53399, #65432, #42863, #48497, #53764, #31197, #13539, #54509, #59413, #66175, #71779, #8269, #36838, #36107, #25928, #59789 ),
 ( #48131, #25201, #64683, #42494, #59049, #7539, #1937, #36466, #7898, #2679, #71409, #65793, #19908, #70164, #333, #53266, #34486, #63449, #69440, #12662, #693, #47620, #69083, #57803, #1441, #24326, #57429, #29949, #18667, #46514, #11922, #29210, #1802, #12293, #58165, #24688, #47261, #52899, #41609, #1066, #35592, #64549, #35232, #5944, #6663, #29568, #46896, #64929, #28853, #17568, #70529, #19040, #30322, #35964, #63820, #13027, #51784, #52510, #40884, #23960, #58916, #58528, #7407, #52148, #41993, #17943, #23227, #46152, #69805, #7023, #18305, #41248, #40502, #64188, #34867, #6307, #23580, #20898, #37085, #60036, #20146, #7771, #14890, #37832, #55108, #36334, #60763, #14133, #31797, #43108, #43488, #42361, #25059, #59279, #66040, #9242, #59648, #30685, #2172, #8520, #31058, #32162, #8132, #49096, #3635, #71650, #13769, #54742, #54015, #14513, #42725, #26534, #3267, #72020, #49467, #72391, #2553, #26158, #66409, #53630, #19778, #25434, #48000, #20533, #37469, #65659, #31434, #43848, #13405, #70912, #19412, #65299, #36705, #48361, #25797, #71274, #8881, #54375, #60400, #2906, #48727, #47429, #52322, #12832, #23396, #52697, #51951, #13572, #36506, #12469, #18477, #70709, #42168, #24860, #40687, #63632, #13207, #70334, #63990, #58708, #1609, #30125, #1972, #59087, #69972, #36140, #35408, #1245, #58337, #41418, #502, #7207, #24495, #18120, #18840, #23751, #19217, #64358, #6830, #69249, #59453, #47789, #41780, #53074, #64724, #865, #35757, #46321, #24142, #17738, #7937, #12100, #29741, #7577, #65102, #35039, #57972, #6479, #29382, #30493, #53436, #47070, #46692, #69621, #41058, #55286, #37992, #48894, #15054, #65831, #31600, #14318, #20329, #53800, #37634, #54911, #71448, #3435, #2714, #49628, #43288, #15421, #26698, #32342, #60206, #66575, #48169, #54545, #37269, #8688, #60925, #31969, #72193, #48533, #9414, #42906, #20701, #2348, #25967, #26341, #3073, #71818, #38367, #66212, #3804, #43651, #72556, #61308, #14686, #60571, #9048, #49269, #21061, #25243, #44011, #66926, #30854, #59824, #71077, #19580, #19949, #42529, #65472, #54188, #13936, #36876, #8313, #31238, #25596, #21813, #38742, #4544, #51496, #62050, #33451, #56, #74051, #5293, #16930, #50750, #62436, #45510, #10526, #55653, #56413 ) ),
 .UNSPECIFIED., .F., .F., .F. ) 
 B_SPLINE_SURFACE_WITH_KNOTS ( ( 2, 2 ),
 ( 3, 2, 2, 2, 2, 2, 2, 2, 2, 2, 2, 2, 2, 2, 2, 2, 2, 2, 2, 2, 2, 2, 2, 2, 2, 2, 2, 2, 2, 2, 2, 2, 2, 2, 2, 2, 2, 2, 2, 2, 2, 2, 2, 2, 2, 2, 2, 2, 2, 2, 2, 2, 2, 2, 2, 2, 2, 2, 2, 2, 2, 2, 2, 2, 2, 2, 2, 2, 2, 2, 2, 2, 2, 2, 2, 2, 2, 2, 2, 2, 2, 2, 2, 2, 2, 2, 2, 2, 2, 2, 2, 2, 2, 2, 2, 2, 2, 2, 2, 2, 2, 2, 2, 2, 2, 2, 2, 2, 2, 2, 2, 2, 2, 2, 2, 2, 2, 2, 2, 2, 2, 2, 2, 2, 2, 2, 2, 2, 2, 2, 2, 2, 2, 2, 2, 2, 2, 2, 2, 2, 2, 2, 3 ),
 ( 0.000000000000000000, 1.000000000000000000 ),
 ( 0.000000000000000000, 0.006944444444444444059, 0.01388888888888888812, 0.02083333333333333218, 0.02777777777777777624, 0.03472222222222222376, 0.04166666666666666435, 0.04861111111111111188, 0.05555555555555555247, 0.06250000000000000000, 0.06944444444444444753, 0.07638888888888889506, 0.08333333333333332871, 0.09027777777777777624, 0.09722222222222222376, 0.1041666666666666713, 0.1111111111111111049, 0.1180555555555555525, 0.1250000000000000000, 0.1319444444444444475, 0.1388888888888888951, 0.1458333333333333426, 0.1527777777777777901, 0.1597222222222222099, 0.1666666666666666574, 0.1736111111111111049, 0.1805555555555555525, 0.1875000000000000000, 0.1944444444444444475, 0.2013888888888888951, 0.2083333333333333426, 0.2152777777777777901, 0.2222222222222222099, 0.2291666666666666574, 0.2361111111111111049, 0.2430555555555555525, 0.2500000000000000000, 0.2569444444444444198, 0.2638888888888888951, 0.2708333333333333148, 0.2777777777777777901, 0.2847222222222222099, 0.2916666666666666852, 0.2986111111111111049, 0.3055555555555555802, 0.3125000000000000000, 0.3194444444444444198, 0.3263888888888888951, 0.3333333333333333148, 0.3402777777777777901, 0.3472222222222222099, 0.3541666666666666852, 0.3611111111111111049, 0.3680555555555555802, 0.3750000000000000000, 0.3819444444444444198, 0.3888888888888888951, 0.3958333333333333148, 0.4027777777777777901, 0.4097222222222222099, 0.4166666666666666852, 0.4236111111111111049, 0.4305555555555555802, 0.4375000000000000000, 0.4444444444444444198, 0.4513888888888888951, 0.4583333333333333148, 0.4652777777777777901, 0.4722222222222222099, 0.4791666666666666852, 0.4861111111111111049, 0.4930555555555555802, 0.5000000000000000000, 0.5069444444444444198, 0.5138888888888888395, 0.5208333333333333703, 0.5277777777777777901, 0.5347222222222222099, 0.5416666666666666297, 0.5486111111111111605, 0.5555555555555555802, 0.5625000000000000000, 0.5694444444444444198, 0.5763888888888888395, 0.5833333333333333703, 0.5902777777777777901, 0.5972222222222222099, 0.6041666666666666297, 0.6111111111111111605, 0.6180555555555555802, 0.6250000000000000000, 0.6319444444444444198, 0.6388888888888888395, 0.6458333333333333703, 0.6527777777777777901, 0.6597222222222222099, 0.6666666666666666297, 0.6736111111111111605, 0.6805555555555555802, 0.6875000000000000000, 0.6944444444444444198, 0.7013888888888888395, 0.7083333333333333703, 0.7152777777777777901, 0.7222222222222222099, 0.7291666666666666297, 0.7361111111111111605, 0.7430555555555555802, 0.7500000000000000000, 0.7569444444444444198, 0.7638888888888888395, 0.7708333333333333703, 0.7777777777777777901, 0.7847222222222222099, 0.7916666666666666297, 0.7986111111111111605, 0.8055555555555555802, 0.8125000000000000000, 0.8194444444444444198, 0.8263888888888888395, 0.8333333333333333703, 0.8402777777777777901, 0.8472222222222222099, 0.8541666666666666297, 0.8611111111111111605, 0.8680555555555555802, 0.8750000000000000000, 0.8819444444444444198, 0.8888888888888888395, 0.8958333333333333703, 0.9027777777777777901, 0.9097222222222222099, 0.9166666666666666297, 0.9236111111111111605, 0.9305555555555555802, 0.9375000000000000000, 0.9444444444444444198, 0.9513888888888888395, 0.9583333333333333703, 0.9652777777777777901, 0.9722222222222222099, 0.9791666666666666297, 0.9842227634901433708 ),
 .UNSPECIFIED. ) 
 GEOMETRIC_REPRESENTATION_ITEM ( )  RATIONAL_B_SPLINE_SURFACE ( (
 ( 1.000000000000000000, 0.8660254037844387076, 1.000000000000000000, 0.8660254037844387076, 1.000000000000000000, 0.8660254037844387076, 1.000000000000000000, 0.8660254037844387076, 1.000000000000000000, 0.8660254037844387076, 1.000000000000000000, 0.8660254037844387076, 1.000000000000000000, 0.8660254037844387076, 1.000000000000000000, 0.8660254037844387076, 1.000000000000000000, 0.8660254037844387076, 1.000000000000000000, 0.8660254037844387076, 1.000000000000000000, 0.8660254037844387076, 1.000000000000000000, 0.8660254037844387076, 1.000000000000000000, 0.8660254037844387076, 1.000000000000000000, 0.8660254037844387076, 1.000000000000000000, 0.8660254037844387076, 1.000000000000000000, 0.8660254037844387076, 1.000000000000000000, 0.8660254037844387076, 1.000000000000000000, 0.8660254037844387076, 1.000000000000000000, 0.8660254037844387076, 1.000000000000000000, 0.8660254037844387076, 1.000000000000000000, 0.8660254037844387076, 1.000000000000000000, 0.8660254037844387076, 1.000000000000000000, 0.8660254037844387076, 1.000000000000000000, 0.8660254037844387076, 1.000000000000000000, 0.8660254037844387076, 1.000000000000000000, 0.8660254037844387076, 1.000000000000000000, 0.8660254037844387076, 1.000000000000000000, 0.8660254037844387076, 1.000000000000000000, 0.8660254037844387076, 1.000000000000000000, 0.8660254037844387076, 1.000000000000000000, 0.8660254037844387076, 1.000000000000000000, 0.8660254037844387076, 1.000000000000000000, 0.8660254037844387076, 1.000000000000000000, 0.8660254037844387076, 1.000000000000000000, 0.8660254037844387076, 1.000000000000000000, 0.8660254037844387076, 1.000000000000000000, 0.8660254037844387076, 1.000000000000000000, 0.8660254037844387076, 1.000000000000000000, 0.8660254037844387076, 1.000000000000000000, 0.8660254037844387076, 1.000000000000000000, 0.8660254037844387076, 1.000000000000000000, 0.8660254037844387076, 1.000000000000000000, 0.8660254037844387076, 1.000000000000000000, 0.8660254037844387076, 1.000000000000000000, 0.8660254037844387076, 1.000000000000000000, 0.8660254037844387076, 1.000000000000000000, 0.8660254037844387076, 1.000000000000000000, 0.8660254037844387076, 1.000000000000000000, 0.8660254037844387076, 1.000000000000000000, 0.8660254037844387076, 1.000000000000000000, 0.8660254037844387076, 1.000000000000000000, 0.8660254037844387076, 1.000000000000000000, 0.8660254037844387076, 1.000000000000000000, 0.8660254037844387076, 1.000000000000000000, 0.8660254037844387076, 1.000000000000000000, 0.8660254037844387076, 1.000000000000000000, 0.8660254037844387076, 1.000000000000000000, 0.8660254037844387076, 1.000000000000000000, 0.8660254037844387076, 1.000000000000000000, 0.8660254037844387076, 1.000000000000000000, 0.8660254037844387076, 1.000000000000000000, 0.8660254037844387076, 1.000000000000000000, 0.8660254037844387076, 1.000000000000000000, 0.8660254037844387076, 1.000000000000000000, 0.8660254037844387076, 1.000000000000000000, 0.8660254037844387076, 1.000000000000000000, 0.8660254037844387076, 1.000000000000000000, 0.8660254037844387076, 1.000000000000000000, 0.8660254037844387076, 1.000000000000000000, 0.8660254037844387076, 1.000000000000000000, 0.8660254037844387076, 1.000000000000000000, 0.8660254037844387076, 1.000000000000000000, 0.8660254037844387076, 1.000000000000000000, 0.8660254037844387076, 1.000000000000000000, 0.8660254037844387076, 1.000000000000000000, 0.8660254037844387076, 1.000000000000000000, 0.8660254037844387076, 1.000000000000000000, 0.8660254037844387076, 1.000000000000000000, 0.8660254037844387076, 1.000000000000000000, 0.8660254037844387076, 1.000000000000000000, 0.8660254037844387076, 1.000000000000000000, 0.8660254037844387076, 1.000000000000000000, 0.8660254037844387076, 1.000000000000000000, 0.8660254037844387076, 1.000000000000000000, 0.8660254037844387076, 1.000000000000000000, 0.8660254037844387076, 1.000000000000000000, 0.8660254037844387076, 1.000000000000000000, 0.8660254037844387076, 1.000000000000000000, 0.8660254037844387076, 1.000000000000000000, 0.8660254037844387076, 1.000000000000000000, 0.8660254037844387076, 1.000000000000000000, 0.8660254037844387076, 1.000000000000000000, 0.8660254037844387076, 1.000000000000000000, 0.8660254037844387076, 1.000000000000000000, 0.8660254037844387076, 1.000000000000000000, 0.8660254037844387076, 1.000000000000000000, 0.8660254037844387076, 1.000000000000000000, 0.8660254037844387076, 1.000000000000000000, 0.8660254037844387076, 1.000000000000000000, 0.8660254037844387076, 1.000000000000000000, 0.8660254037844387076, 1.000000000000000000, 0.8660254037844387076, 1.000000000000000000, 0.8660254037844387076, 1.000000000000000000, 0.8660254037844387076, 1.000000000000000000, 0.8660254037844387076, 1.000000000000000000, 0.8660254037844387076, 1.000000000000000000, 0.8660254037844387076, 1.000000000000000000, 0.8660254037844387076, 1.000000000000000000, 0.8660254037844387076, 1.000000000000000000, 0.8660254037844387076, 1.000000000000000000, 0.8660254037844387076, 1.000000000000000000, 0.8660254037844387076, 1.000000000000000000, 0.8660254037844387076, 1.000000000000000000, 0.8660254037844387076, 1.000000000000000000, 0.8660254037844387076, 1.000000000000000000, 0.8660254037844387076, 1.000000000000000000, 0.8660254037844387076, 1.000000000000000000, 0.8660254037844387076, 1.000000000000000000, 0.8660254037844387076, 1.000000000000000000, 0.8660254037844387076, 1.000000000000000000, 0.8660254037844387076, 1.000000000000000000, 0.8660254037844387076, 1.000000000000000000, 0.8660254037844387076, 1.000000000000000000, 0.8660254037844387076, 1.000000000000000000, 0.8660254037844387076, 1.000000000000000000, 0.8660254037844387076, 1.000000000000000000, 0.8660254037844387076, 1.000000000000000000, 0.8660254037844387076, 1.000000000000000000, 0.8660254037844387076, 1.000000000000000000, 0.8660254037844387076, 1.000000000000000000, 0.8660254037844387076, 1.000000000000000000, 0.8660254037844387076, 1.000000000000000000, 0.8660254037844387076, 1.000000000000000000, 0.8660254037844387076, 1.000000000000000000, 0.8660254037844387076, 1.000000000000000000, 0.8660254037844387076, 1.000000000000000000, 0.8660254037844387076, 1.000000000000000000, 0.8660254037844387076, 1.000000000000000000, 0.8660254037844387076, 1.000000000000000000, 0.8660254037844387076, 1.000000000000000000, 0.8660254037844387076, 1.000000000000000000, 0.9024560516293018697, 0.9469512977404641596),
 ( 1.000000000000000000, 0.8660254037844387076, 1.000000000000000000, 0.8660254037844387076, 1.000000000000000000, 0.8660254037844387076, 1.000000000000000000, 0.8660254037844387076, 1.000000000000000000, 0.8660254037844387076, 1.000000000000000000, 0.8660254037844387076, 1.000000000000000000, 0.8660254037844387076, 1.000000000000000000, 0.8660254037844387076, 1.000000000000000000, 0.8660254037844387076, 1.000000000000000000, 0.8660254037844387076, 1.000000000000000000, 0.8660254037844387076, 1.000000000000000000, 0.8660254037844387076, 1.000000000000000000, 0.8660254037844387076, 1.000000000000000000, 0.8660254037844387076, 1.000000000000000000, 0.8660254037844387076, 1.000000000000000000, 0.8660254037844387076, 1.000000000000000000, 0.8660254037844387076, 1.000000000000000000, 0.8660254037844387076, 1.000000000000000000, 0.8660254037844387076, 1.000000000000000000, 0.8660254037844387076, 1.000000000000000000, 0.8660254037844387076, 1.000000000000000000, 0.8660254037844387076, 1.000000000000000000, 0.8660254037844387076, 1.000000000000000000, 0.8660254037844387076, 1.000000000000000000, 0.8660254037844387076, 1.000000000000000000, 0.8660254037844387076, 1.000000000000000000, 0.8660254037844387076, 1.000000000000000000, 0.8660254037844387076, 1.000000000000000000, 0.8660254037844387076, 1.000000000000000000, 0.8660254037844387076, 1.000000000000000000, 0.8660254037844387076, 1.000000000000000000, 0.8660254037844387076, 1.000000000000000000, 0.8660254037844387076, 1.000000000000000000, 0.8660254037844387076, 1.000000000000000000, 0.8660254037844387076, 1.000000000000000000, 0.8660254037844387076, 1.000000000000000000, 0.8660254037844387076, 1.000000000000000000, 0.8660254037844387076, 1.000000000000000000, 0.8660254037844387076, 1.000000000000000000, 0.8660254037844387076, 1.000000000000000000, 0.8660254037844387076, 1.000000000000000000, 0.8660254037844387076, 1.000000000000000000, 0.8660254037844387076, 1.000000000000000000, 0.8660254037844387076, 1.000000000000000000, 0.8660254037844387076, 1.000000000000000000, 0.8660254037844387076, 1.000000000000000000, 0.8660254037844387076, 1.000000000000000000, 0.8660254037844387076, 1.000000000000000000, 0.8660254037844387076, 1.000000000000000000, 0.8660254037844387076, 1.000000000000000000, 0.8660254037844387076, 1.000000000000000000, 0.8660254037844387076, 1.000000000000000000, 0.8660254037844387076, 1.000000000000000000, 0.8660254037844387076, 1.000000000000000000, 0.8660254037844387076, 1.000000000000000000, 0.8660254037844387076, 1.000000000000000000, 0.8660254037844387076, 1.000000000000000000, 0.8660254037844387076, 1.000000000000000000, 0.8660254037844387076, 1.000000000000000000, 0.8660254037844387076, 1.000000000000000000, 0.8660254037844387076, 1.000000000000000000, 0.8660254037844387076, 1.000000000000000000, 0.8660254037844387076, 1.000000000000000000, 0.8660254037844387076, 1.000000000000000000, 0.8660254037844387076, 1.000000000000000000, 0.8660254037844387076, 1.000000000000000000, 0.8660254037844387076, 1.000000000000000000, 0.8660254037844387076, 1.000000000000000000, 0.8660254037844387076, 1.000000000000000000, 0.8660254037844387076, 1.000000000000000000, 0.8660254037844387076, 1.000000000000000000, 0.8660254037844387076, 1.000000000000000000, 0.8660254037844387076, 1.000000000000000000, 0.8660254037844387076, 1.000000000000000000, 0.8660254037844387076, 1.000000000000000000, 0.8660254037844387076, 1.000000000000000000, 0.8660254037844387076, 1.000000000000000000, 0.8660254037844387076, 1.000000000000000000, 0.8660254037844387076, 1.000000000000000000, 0.8660254037844387076, 1.000000000000000000, 0.8660254037844387076, 1.000000000000000000, 0.8660254037844387076, 1.000000000000000000, 0.8660254037844387076, 1.000000000000000000, 0.8660254037844387076, 1.000000000000000000, 0.8660254037844387076, 1.000000000000000000, 0.8660254037844387076, 1.000000000000000000, 0.8660254037844387076, 1.000000000000000000, 0.8660254037844387076, 1.000000000000000000, 0.8660254037844387076, 1.000000000000000000, 0.8660254037844387076, 1.000000000000000000, 0.8660254037844387076, 1.000000000000000000, 0.8660254037844387076, 1.000000000000000000, 0.8660254037844387076, 1.000000000000000000, 0.8660254037844387076, 1.000000000000000000, 0.8660254037844387076, 1.000000000000000000, 0.8660254037844387076, 1.000000000000000000, 0.8660254037844387076, 1.000000000000000000, 0.8660254037844387076, 1.000000000000000000, 0.8660254037844387076, 1.000000000000000000, 0.8660254037844387076, 1.000000000000000000, 0.8660254037844387076, 1.000000000000000000, 0.8660254037844387076, 1.000000000000000000, 0.8660254037844387076, 1.000000000000000000, 0.8660254037844387076, 1.000000000000000000, 0.8660254037844387076, 1.000000000000000000, 0.8660254037844387076, 1.000000000000000000, 0.8660254037844387076, 1.000000000000000000, 0.8660254037844387076, 1.000000000000000000, 0.8660254037844387076, 1.000000000000000000, 0.8660254037844387076, 1.000000000000000000, 0.8660254037844387076, 1.000000000000000000, 0.8660254037844387076, 1.000000000000000000, 0.8660254037844387076, 1.000000000000000000, 0.8660254037844387076, 1.000000000000000000, 0.8660254037844387076, 1.000000000000000000, 0.8660254037844387076, 1.000000000000000000, 0.8660254037844387076, 1.000000000000000000, 0.8660254037844387076, 1.000000000000000000, 0.8660254037844387076, 1.000000000000000000, 0.8660254037844387076, 1.000000000000000000, 0.8660254037844387076, 1.000000000000000000, 0.8660254037844387076, 1.000000000000000000, 0.8660254037844387076, 1.000000000000000000, 0.8660254037844387076, 1.000000000000000000, 0.8660254037844387076, 1.000000000000000000, 0.8660254037844387076, 1.000000000000000000, 0.8660254037844387076, 1.000000000000000000, 0.8660254037844387076, 1.000000000000000000, 0.8660254037844387076, 1.000000000000000000, 0.8660254037844387076, 1.000000000000000000, 0.8660254037844387076, 1.000000000000000000, 0.8660254037844387076, 1.000000000000000000, 0.8660254037844387076, 1.000000000000000000, 0.8660254037844387076, 1.000000000000000000, 0.8660254037844387076, 1.000000000000000000, 0.8660254037844387076, 1.000000000000000000, 0.8660254037844387076, 1.000000000000000000, 0.8660254037844387076, 1.000000000000000000, 0.8660254037844387076, 1.000000000000000000, 0.8660254037844387076, 1.000000000000000000, 0.8660254037844387076, 1.000000000000000000, 0.9024560516293018697, 0.9469512977404641596) ) ) 
 REPRESENTATION_ITEM ( '' )  SURFACE ( )  );
#27033=CYLINDRICAL_SURFACE ( 'NONE', #52345, 2.649999999999985700 ) ;
#27034=CARTESIAN_POINT ( 'NONE',  ( 97.65000000000000568, 91.52997821335252127, 75.84479166840098685 ) ) ;
#27038=DIRECTION ( 'NONE',  ( -0.000000000000000000, -0.000000000000000000, 1.000000000000000000 ) ) ;
#27039=CARTESIAN_POINT ( 'NONE',  ( -97.64999999999996305, -209.9999999999999716, 84.28499999999999659 ) ) ;
#27041=EDGE_CURVE ( 'NONE', #71124, #12034, #45997, .T. ) ;
#27051=CARTESIAN_POINT ( 'NONE',  ( 92.69370383062501162, -209.9999999999999716, 87.89656250086714806 ) ) ;
#27054=B_SPLINE_CURVE_WITH_KNOTS ( 'NONE', 3,
 ( #67582, #50274, #33739, #4075, #73950, #22463 ),
 .UNSPECIFIED., .F., .F.,
 ( 4, 2, 4 ),
 ( 0.000000000000000000, 0.0008269033587271741939, 0.001653806717454348388 ),
 .UNSPECIFIED. ) ;
#27058=AXIS2_PLACEMENT_3D ( 'NONE', #6158, #29063, #14914 ) ;
#27059=CARTESIAN_POINT ( 'NONE',  ( 95.00000000000000000, -212.6630814284392557, 79.00656250086714749 ) ) ;
#27060=CARTESIAN_POINT ( 'NONE',  ( 96.15314808468748708, -208.0026889286704943, 83.87489583420048689 ) ) ;
#27064=CARTESIAN_POINT ( 'NONE',  ( 95.00000000000000000, -207.3369185715606307, 86.46781250086716852 ) ) ;
#27082=ORIENTED_EDGE ( 'NONE', *, *, #48658, .T. ) ;
#27092=CARTESIAN_POINT ( 'NONE',  ( -93.84685191531252713, 88.00268892867056536, 77.31322916753381946 ) ) ;
#27094=CARTESIAN_POINT ( 'NONE',  ( 97.30629616937498838, 90.00000000000002842, 79.16531250086714522 ) ) ;
#27097=CARTESIAN_POINT ( 'NONE',  ( -97.30629616937495996, -209.9999999999999716, 88.37281250086715545 ) ) ;
#27102=CARTESIAN_POINT ( 'NONE',  ( -92.69370383062498320, -211.3315407142195852, 78.47739583420047893 ) ) ;
#27113=CARTESIAN_POINT ( 'NONE',  ( 92.54662210827909519, -209.5154774236565061, 74.90854212414865287 ) ) ;
#27114=CARTESIAN_POINT ( 'NONE',  ( -97.30629616937501680, 91.33154071421968467, 82.60489583420047666 ) ) ;
#27124=AXIS2_PLACEMENT_3D ( 'NONE', #56108, #50825, #67764 ) ;
#27126=CARTESIAN_POINT ( 'NONE',  ( -93.84685191531247028, -211.9973110713294489, 79.21822916753382060 ) ) ;
#27129=CARTESIAN_POINT ( 'NONE',  ( -93.67499999999998295, -212.2949673200287179, 87.11604166840096752 ) ) ;
#27132=CARTESIAN_POINT ( 'NONE',  ( -93.33864827736698544, -211.6008015735577033, 74.79754476654878204 ) ) ;
#27135=EDGE_CURVE ( 'NONE', #47166, #39507, #12867, .T. ) ;
#27143=ORIENTED_EDGE ( 'NONE', *, *, #55222, .F. ) ;
#27164=CARTESIAN_POINT ( 'NONE',  ( 93.84685191531248449, 88.00268892867053694, 77.84239583420048803 ) ) ;
#27169=VERTEX_POINT ( 'NONE', #53477 ) ;
#27170=CARTESIAN_POINT ( 'NONE',  ( 93.84685191531248449, 91.99731107132950569, 88.90197916753380980 ) ) ;
#27172=CARTESIAN_POINT ( 'NONE',  ( 93.84685191531249870, -208.0026889286704943, 86.36197916753381776 ) ) ;
#27174=CYLINDRICAL_SURFACE ( 'NONE', #19914, 2.649999999999999467 ) ;
#27179=DIRECTION ( 'NONE',  ( -0.000000000000000000, -0.000000000000000000, 1.000000000000000000 ) ) ;
#27181=CARTESIAN_POINT ( 'NONE',  ( -92.69370383062498320, -208.6684592857803011, 89.37822916753381719 ) ) ;
#27182=CARTESIAN_POINT ( 'NONE',  ( -93.84685191531252713, 88.00268892867056536, 84.93322916753382401 ) ) ;
#27184=CARTESIAN_POINT ( 'NONE',  ( 94.99999999999998579, 92.66308142843935514, 88.21406250086714351 ) ) ;
#27185=CARTESIAN_POINT ( 'NONE',  ( -92.69370383062502583, 91.33154071421968467, 86.83822916753381094 ) ) ;
#27189=CARTESIAN_POINT ( 'NONE',  ( -94.99999999999997158, -209.9999999999999716, 90.00000000000000000 ) ) ;
#27190=CARTESIAN_POINT ( 'NONE',  ( 92.35000000039362078, 90.00002930319625705, 82.45844277051448046 ) ) ;
#27193=CARTESIAN_POINT ( 'NONE',  ( 92.35000000039362078, 90.00002930319625705, 82.45844277051448046 ) ) ;
#27197=CARTESIAN_POINT ( 'NONE',  ( -96.32500000000001705, 87.70503267997129626, 81.21583333333333599 ) ) ;
#27202=LINE ( 'NONE', #66713, #49548 ) ;
#27208=CARTESIAN_POINT ( 'NONE',  ( -93.84685191531252713, 88.00268892867056536, 81.59947916753381492 ) ) ;
#27218=CARTESIAN_POINT ( 'NONE',  ( -97.30629616937497417, -208.6684592857803011, 88.47864583420047779 ) ) ;
#27223=CARTESIAN_POINT ( 'NONE',  ( 92.69370383062498320, 91.33154071421968467, 78.95364583420045790 ) ) ;
#27224=CARTESIAN_POINT ( 'NONE',  ( -97.30629616937497417, -208.6684592857803295, 84.03364583420049883 ) ) ;
#27229=CARTESIAN_POINT ( 'NONE',  ( -97.64999999999996305, -209.9999999999999716, 76.66499999999999204 ) ) ;
#27230=CARTESIAN_POINT ( 'NONE',  ( 97.64999999999999147, -209.9999999999999716, 78.25249999999999773 ) ) ;
#27232=CARTESIAN_POINT ( 'NONE',  ( -92.69370383062504004, 90.00000000000004263, 79.95906250086714806 ) ) ;
#27233=CARTESIAN_POINT ( 'NONE',  ( 92.69370383062501162, -209.9999999999999716, 82.02281250086714692 ) ) ;
#27244=ADVANCED_FACE ( 'NONE', ( #50415 ), #44796, .F. ) ;
#27248=DIRECTION ( 'NONE',  ( -0.000000000000000000, -0.000000000000000000, 1.000000000000000000 ) ) ;
#27253=( BOUNDED_CURVE ( )  B_SPLINE_CURVE ( 2, ( #43033, #49022, #2838, #31731, #48666, #54676, #65975, #71953, #43421 ),
 .UNSPECIFIED., .F., .F. ) 
 B_SPLINE_CURVE_WITH_KNOTS ( ( 3, 2, 2, 2, 3 ),
 ( 0.7196881748034551496, 0.7267438507108833212, 0.7337996162517648191, 0.7408553817926464280, 0.7408554641864648627 ),
 .UNSPECIFIED. ) 
 CURVE ( )  GEOMETRIC_REPRESENTATION_ITEM ( )  RATIONAL_B_SPLINE_CURVE ( ( 0.9999965961303247663, 0.8660271057408972517, 1.000000000000000000, 0.8660254037844387076, 1.000000000000000000, 0.8660254037844387076, 1.000000000000000000, 0.9999984355094434507, 0.9999968710554256734 ) ) 
 REPRESENTATION_ITEM ( '' )  );
#27254=CARTESIAN_POINT ( 'NONE',  ( 94.99999999999998579, 92.66308142843935514, 86.46781250086716852 ) ) ;
#27256=DIRECTION ( 'NONE',  ( 0.000000000000000000, 0.000000000000000000, -1.000000000000000000 ) ) ;
#27257=CARTESIAN_POINT ( 'NONE',  ( 93.67500000000001137, -212.2949673200287179, 76.77083333333332860 ) ) ;
#27263=VERTEX_POINT ( 'NONE', #4581 ) ;
#27269=CARTESIAN_POINT ( 'NONE',  ( -92.35000982493194499, -211.5299838857795862, 88.43895794268827615 ) ) ;
#27271=VERTEX_POINT ( 'NONE', #67344 ) ;
#27272=CARTESIAN_POINT ( 'NONE',  ( -96.32499999999996021, -212.2949673200287179, 81.29520833506762756 ) ) ;
#27277=CARTESIAN_POINT ( 'NONE',  ( 93.67499999999998295, 92.29496732002878900, 84.25854166840096582 ) ) ;
#27278=CARTESIAN_POINT ( 'NONE',  ( -95.00000000000002842, 93.05995642670501411, 82.93562500173429441 ) ) ;
#27280=CARTESIAN_POINT ( 'NONE',  ( 97.30629616937498838, 88.66845928578037217, 84.98614583420047097 ) ) ;
#27295=CARTESIAN_POINT ( 'NONE',  ( -97.65000000000001990, 90.00002373248484844, 79.91937418090955703 ) ) ;
#27296=DIRECTION ( 'NONE',  ( -0.000000000000000000, -0.000000000000000000, -1.000000000000000000 ) ) ;
#27297=CARTESIAN_POINT ( 'NONE',  ( -97.30629616937497417, -208.6684592857803011, 79.58864583420047722 ) ) ;
#27298=ORIENTED_EDGE ( 'NONE', *, *, #32239, .F. ) ;
#27306=CARTESIAN_POINT ( 'NONE',  ( 92.69370383062498320, 91.33154071421968467, 77.52489583420046415 ) ) ;
#27309=CYLINDRICAL_SURFACE ( 'NONE', #21690, 2.649999999999985700 ) ;
#27310=DIRECTION ( 'NONE',  ( -1.000000000000000000, 0.000000000000000000, 0.000000000000000000 ) ) ;
#27315=AXIS2_PLACEMENT_3D ( 'NONE', #37866, #21286, #43879 ) ;
#27316=CARTESIAN_POINT ( 'NONE',  ( 97.64999999999999147, -209.9999999999999716, 83.33250000000001023 ) ) ;
#27321=CARTESIAN_POINT ( 'NONE',  ( -97.30629616937501680, 90.00000000000004263, 83.92781250086714806 ) ) ;
#27335=CARTESIAN_POINT ( 'NONE',  ( 95.00000000000000000, -207.3369185715606307, 80.11781250086714579 ) ) ;
#27338=EDGE_LOOP ( 'NONE', ( #60924, #2809 ) ) ;
#27341=VECTOR ( 'NONE', #4975, 1000.000000000000000 ) ;
#27348=CARTESIAN_POINT ( 'NONE',  ( 93.67500000000001137, -212.2949673200287179, 86.93083333333332519 ) ) ;
#27357=CARTESIAN_POINT ( 'NONE',  ( 92.35000000000002274, -208.4700217866474645, 78.59645833506763779 ) ) ;
#27358=CARTESIAN_POINT ( 'NONE',  ( 92.34999999999999432, 91.52997821335252127, 82.96208333333333940 ) ) ;
#27362=CARTESIAN_POINT ( 'NONE',  ( 97.65000000000000568, 91.52997821335252127, 80.92479166840097093 ) ) ;
#27365=CARTESIAN_POINT ( 'NONE',  ( -92.69370383062505425, 91.33154071421968467, 84.45697916753383083 ) ) ;
#27367=CARTESIAN_POINT ( 'NONE',  ( 92.69370383062498320, 90.00000000000002842, 77.57781250086713953 ) ) ;
#27371=CYLINDRICAL_SURFACE ( 'NONE', #38899, 2.649999999999985700 ) ;
#27376=CARTESIAN_POINT ( 'NONE',  ( -96.15314808468747287, -208.0026889286704943, 81.28197916753380525 ) ) ;
#27377=ORIENTED_EDGE ( 'NONE', *, *, #16476, .T. ) ;
#27380=DIRECTION ( 'NONE',  ( 0.000000000000000000, 0.000000000000000000, -1.000000000000000000 ) ) ;
#27383=CARTESIAN_POINT ( 'NONE',  ( 92.34999999999999432, 88.47002178664753558, 88.86229166840097093 ) ) ;
#27385=CARTESIAN_POINT ( 'NONE',  ( -93.84685191531247028, -211.9973110713294489, 77.15447916753380753 ) ) ;
#27386=ORIENTED_EDGE ( 'NONE', *, *, #70430, .T. ) ;
#27389=DIRECTION ( 'NONE',  ( -0.000000000000000000, -0.000000000000000000, 1.000000000000000000 ) ) ;
#27393=CARTESIAN_POINT ( 'NONE',  ( -92.35000000000000853, 88.47002178664759242, 81.37458333333333371 ) ) ;
#27397=CARTESIAN_POINT ( 'NONE',  ( 93.84685191531248449, 88.00268892867053694, 88.47864583420047779 ) ) ;
#27403=CARTESIAN_POINT ( 'NONE',  ( -92.35000000000002274, 89.99999149135206267, 88.49187470744952577 ) ) ;
#27407=DIRECTION ( 'NONE',  ( 1.000000000000000000, 0.000000000000000000, 0.000000000000000000 ) ) ;
#27410=EDGE_CURVE ( 'NONE', #55837, #42834, #69651, .T. ) ;
#27415=CARTESIAN_POINT ( 'NONE',  ( -92.34999999999999432, -209.9999999999999716, 85.87249999999998806 ) ) ;
#27427=CARTESIAN_POINT ( 'NONE',  ( 93.84685191531251292, -211.9973110713294489, 89.27239583420049485 ) ) ;
#27435=CARTESIAN_POINT ( 'NONE',  ( 97.30629616937498838, -209.9999999999999716, 78.53031250086714010 ) ) ;
#27437=CARTESIAN_POINT ( 'NONE',  ( 92.69370383062501162, -208.6684592857803011, 87.20864583420049598 ) ) ;
#27442=LINE ( 'NONE', #50377, #4537 ) ;
#27446=ORIENTED_EDGE ( 'NONE', *, *, #27984, .F. ) ;
#27451=FACE_OUTER_BOUND ( 'NONE', #45457, .T. ) ;
#27457=VERTEX_POINT ( 'NONE', #91 ) ;
#27464=CYLINDRICAL_SURFACE ( 'NONE', #9644, 2.649999999999985700 ) ;
#27468=CARTESIAN_POINT ( 'NONE',  ( -93.84685191531254134, 91.99731107132950569, 76.25489583420049655 ) ) ;
#27470=CARTESIAN_POINT ( 'NONE',  ( 92.69370383062498320, 88.66845928578037217, 76.99572916753380980 ) ) ;
#27472=( BOUNDED_CURVE ( )  B_SPLINE_CURVE ( 2, ( #70778, #19281, #42235, #65165, #4607, #3866, #61368 ),
 .UNSPECIFIED., .F., .F. ) 
 B_SPLINE_CURVE_WITH_KNOTS ( ( 3, 2, 2, 3 ),
 ( 0.6773535682785479795, 0.6844092574689497610, 0.6914650230098673411, 0.6985206468877303010 ),
 .UNSPECIFIED. ) 
 CURVE ( )  GEOMETRIC_REPRESENTATION_ITEM ( )  RATIONAL_B_SPLINE_CURVE ( ( 0.9999971005502381605, 0.8660268535250073008, 1.000000000000000000, 0.8660254037844387076, 1.000000000000000000, 0.8660280936769018112, 0.9999946203230871689 ) ) 
 REPRESENTATION_ITEM ( '' )  );
#27474=DIRECTION ( 'NONE',  ( -0.000000000000000000, -0.000000000000000000, 1.000000000000000000 ) ) ;
#27481=CARTESIAN_POINT ( 'NONE',  ( -94.99999999999997158, -207.3369185715606307, 78.68906250086713783 ) ) ;
#27482=VECTOR ( 'NONE', #31696, 1000.000000000000000 ) ;
#27487=CARTESIAN_POINT ( 'NONE',  ( -96.32499999999996021, -212.2949673200287179, 79.31083333333333485 ) ) ;
#27489=VECTOR ( 'NONE', #64594, 1000.000000000000000 ) ;
#27490=EDGE_CURVE ( 'NONE', #45343, #423, #41754, .T. ) ;
#27491=ORIENTED_EDGE ( 'NONE', *, *, #19082, .T. ) ;
#27495=PLANE ( 'NONE',  #6739 ) ;
#27496=CARTESIAN_POINT ( 'NONE',  ( -92.69370383062502583, 88.66845928578038638, 80.38239583420049428 ) ) ;
#27501=LINE ( 'NONE', #72978, #36571 ) ;
#27502=CIRCLE ( 'NONE', #37125, 26.50000000000000355 ) ;
#27509=CARTESIAN_POINT ( 'NONE',  ( 95.00000000000000000, -206.9400435732949575, 88.65062500173428361 ) ) ;
#27510=CARTESIAN_POINT ( 'NONE',  ( -96.15314808468745866, -211.9973110713294489, 79.11239583420048405 ) ) ;
#27525=CARTESIAN_POINT ( 'NONE',  ( 94.99999999999998579, 93.05995642670504253, 78.41125000000000966 ) ) ;
#27529=CARTESIAN_POINT ( 'NONE',  ( 97.30629616937498838, -211.3315407142195852, 88.63739583420047552 ) ) ;
#27531=ORIENTED_EDGE ( 'NONE', *, *, #38464, .T. ) ;
#27542=ORIENTED_EDGE ( 'NONE', *, *, #30735, .T. ) ;
#27547=CARTESIAN_POINT ( 'NONE',  ( 97.30629616937498838, 90.00000000000002842, 77.41906250086715602 ) ) ;
#27554=CARTESIAN_POINT ( 'NONE',  ( 92.69370383062498320, 90.00000000000002842, 87.73781250086713612 ) ) ;
#27556=CARTESIAN_POINT ( 'NONE',  ( 95.00000000000000000, -212.6630814284392557, 85.99156250086714692 ) ) ;
#27567=CARTESIAN_POINT ( 'NONE',  ( 92.35000000049316782, -210.0000320386632495, 83.73041644179299681 ) ) ;
#27569=CARTESIAN_POINT ( 'NONE',  ( -94.99999999999997158, -207.3369185715606307, 86.94406250086714749 ) ) ;
#27570=EDGE_CURVE ( 'NONE', #32656, #20380, #71400, .T. ) ;
#27571=CARTESIAN_POINT ( 'NONE',  ( -96.15314808468752972, 91.99731107132950569, 85.88572916753381037 ) ) ;
#27573=CARTESIAN_POINT ( 'NONE',  ( 96.15314808468748708, 91.99731107132950569, 87.52614583420047722 ) ) ;
#27574=CARTESIAN_POINT ( 'NONE',  ( -93.84685191531252713, 88.00268892867056536, 84.77447916753381207 ) ) ;
#27577=CARTESIAN_POINT ( 'NONE',  ( -96.32499999999996021, -212.2949673200287179, 80.66020833506763665 ) ) ;
#27579=CYLINDRICAL_SURFACE ( 'NONE', #2422, 2.649999999999985700 ) ;
#27580=CARTESIAN_POINT ( 'NONE',  ( -94.99999999999997158, -207.3369185715606307, 89.48406250086713953 ) ) ;
#27581=DIRECTION ( 'NONE',  ( 1.000000000000000000, 0.000000000000000000, 0.000000000000000000 ) ) ;
#27588=ORIENTED_EDGE ( 'NONE', *, *, #5627, .T. ) ;
#27589=CARTESIAN_POINT ( 'NONE',  ( -96.32500000000001705, 92.29496732002878900, 81.00416666666666288 ) ) ;
#27590=CARTESIAN_POINT ( 'NONE',  ( -95.00000000000002842, 90.00000000000004263, 90.00000000000000000 ) ) ;
#27600=CARTESIAN_POINT ( 'NONE',  ( -93.84685191531252713, 88.00268892867056536, 80.32947916753380468 ) ) ;
#27603=CARTESIAN_POINT ( 'NONE',  ( -97.65000000000001990, 90.00000000000004263, 88.73000000000000398 ) ) ;
#27607=CARTESIAN_POINT ( 'NONE',  ( -96.15314808468745866, -211.9973110713294489, 88.00239583420048461 ) ) ;
#27611=CARTESIAN_POINT ( 'NONE',  ( 92.69370383062498320, 88.66845928578035796, 81.59947916753382913 ) ) ;
#27612=CARTESIAN_POINT ( 'NONE',  ( -97.30629616937497417, -208.6684592857803295, 81.49364583420049257 ) ) ;
#27617=CARTESIAN_POINT ( 'NONE',  ( -96.32499999999996021, -212.2949673200287179, 76.13583333333333769 ) ) ;
#27618=CARTESIAN_POINT ( 'NONE',  ( 92.35000000000000853, 89.99996406754245015, 85.63437624451401575 ) ) ;
#27624=CARTESIAN_POINT ( 'NONE',  ( -96.15314808468752972, 91.99731107132950569, 79.53572916753381605 ) ) ;
#27625=CARTESIAN_POINT ( 'NONE',  ( 92.69370383062501162, -211.3315407142195852, 80.80572916753382628 ) ) ;
#27632=PLANE ( 'NONE',  #21382 ) ;
#27641=CARTESIAN_POINT ( 'NONE',  ( 94.99999999999998579, 92.66308142843935514, 85.83281250086714920 ) ) ;
#27643=CARTESIAN_POINT ( 'NONE',  ( 92.35000000000002274, -211.5299782133524502, 77.98791666666664923 ) ) ;
#27645=VERTEX_POINT ( 'NONE', #7159 ) ;
#27653=AXIS2_PLACEMENT_3D ( 'NONE', #38297, #61242, #9725 ) ;
#27654=CARTESIAN_POINT ( 'NONE',  ( 97.64999999997404245, -210.0000117261773198, 82.77687459617033028 ) ) ;
#27655=EDGE_CURVE ( 'NONE', #59589, #67219, #46592, .T. ) ;
#27659=CARTESIAN_POINT ( 'NONE',  ( -94.99999999999997158, -213.0599564267049857, 83.25312500173430408 ) ) ;
#27663=CARTESIAN_POINT ( 'NONE',  ( 97.64999999999997726, 88.47002178664753558, 82.08895833506764461 ) ) ;
#27664=CARTESIAN_POINT ( 'NONE',  ( -93.67500000000003979, 87.70503267997129626, 84.57604166840096127 ) ) ;
#27666=CARTESIAN_POINT ( 'NONE',  ( 97.30629616937498838, 91.33154071421968467, 82.55197916753382970 ) ) ;
#27671=CARTESIAN_POINT ( 'NONE',  ( 92.48632958231164025, 89.99999999999990052, 74.91808492278045151 ) ) ;
#27676=CARTESIAN_POINT ( 'NONE',  ( -96.32500000000001705, 87.70503267997129626, 82.56520833506762358 ) ) ;
#27678=CARTESIAN_POINT ( 'NONE',  ( 94.99999999999998579, 90.00000000000002842, 90.00000000000000000 ) ) ;
#27680=ORIENTED_EDGE ( 'NONE', *, *, #52136, .F. ) ;
#27682=LINE ( 'NONE', #67537, #71987 ) ;
#27686=CARTESIAN_POINT ( 'NONE',  ( -97.30629616937497417, -211.3315407142195852, 80.96447916753382401 ) ) ;
#27692=EDGE_CURVE ( 'NONE', #23688, #29022, #72146, .T. ) ;
#27708=VECTOR ( 'NONE', #73923, 1000.000000000000000 ) ;
#27710=CARTESIAN_POINT ( 'NONE',  ( -93.84685191531254134, 91.99731107132950569, 80.54114583420046358 ) ) ;
#27712=CARTESIAN_POINT ( 'NONE',  ( 92.69370383062501162, -208.6684592857803011, 89.58989583420047609 ) ) ;
#27714=( BOUNDED_CURVE ( )  B_SPLINE_CURVE ( 2, ( #62768, #34526, #45465, #68761, #50708, #22522, #39818, #63864, #23265 ),
 .UNSPECIFIED., .F., .F. ) 
 B_SPLINE_CURVE_WITH_KNOTS ( ( 3, 2, 2, 2, 3 ),
 ( 0.2116728463006670169, 0.2116729662264711653, 0.2187287317673535236, 0.2257844973082358264, 0.2328402629019980796 ),
 .UNSPECIFIED. ) 
 CURVE ( )  GEOMETRIC_REPRESENTATION_ITEM ( )  RATIONAL_B_SPLINE_CURVE ( ( 0.9999954457845842137, 0.9999977228535877893, 1.000000000000000000, 0.8660254037844387076, 1.000000000000000000, 0.8660254037844387076, 1.000000000000000000, 0.8660254037844387076, 1.000000000000000000 ) ) 
 REPRESENTATION_ITEM ( '' )  );
#27721=CARTESIAN_POINT ( 'NONE',  ( 93.84685191531251292, -211.9973110713294489, 75.93739583420048689 ) ) ;
#27722=VECTOR ( 'NONE', #24432, 1000.000000000000000 ) ;
#27728=CARTESIAN_POINT ( 'NONE',  ( -94.99999999999997158, -206.9400435732949575, 85.47562500173430067 ) ) ;
#27731=CARTESIAN_POINT ( 'NONE',  ( 92.35000000000000853, -209.9999999999999716, 88.73000000000000398 ) ) ;
#27733=ORIENTED_EDGE ( 'NONE', *, *, #4809, .F. ) ;
#27737=ORIENTED_EDGE ( 'NONE', *, *, #63076, .F. ) ;
#27743=CARTESIAN_POINT ( 'NONE',  ( 92.35000000000000853, -209.9999999999999716, 81.18937500173430521 ) ) ;
#27745=CARTESIAN_POINT ( 'NONE',  ( 94.99999999999998579, 93.05995642670504253, 83.49125000000000796 ) ) ;
#27747=DIRECTION ( 'NONE',  ( -0.000000000000000000, -0.000000000000000000, 1.000000000000000000 ) ) ;
#27752=ADVANCED_FACE ( 'NONE', ( #20274 ), #66164, .F. ) ;
#27753=CARTESIAN_POINT ( 'NONE',  ( -92.69370383062505425, 88.66845928578038638, 84.35114583420050849 ) ) ;
#27754=CARTESIAN_POINT ( 'NONE',  ( 94.99999999999998579, 87.33691857156068750, 78.37156250086714238 ) ) ;
#27757=DIRECTION ( 'NONE',  ( -0.000000000000000000, -0.000000000000000000, 1.000000000000000000 ) ) ;
#27762=CARTESIAN_POINT ( 'NONE',  ( 97.64999999999999147, 90.00000000000002842, 75.07749999999998636 ) ) ;
#27764=CARTESIAN_POINT ( 'NONE',  ( -93.84685191531248449, -208.0026889286704943, 76.09614583420047040 ) ) ;
#27771=CARTESIAN_POINT ( 'NONE',  ( -92.34999999999986642, -211.5299782133523649, 78.19958333333332234 ) ) ;
#27773=CARTESIAN_POINT ( 'NONE',  ( -92.69370383062499741, -210.9303297190751891, 74.68334033237940162 ) ) ;
#27778=CARTESIAN_POINT ( 'NONE',  ( -97.64999999999996305, -208.4700217866474645, 89.39145833506763950 ) ) ;
#27781=ADVANCED_FACE ( 'NONE', ( #21763 ), #31924, .F. ) ;
#27784=CARTESIAN_POINT ( 'NONE',  ( 93.84685191531248449, 91.99731107132950569, 83.82197916753381151 ) ) ;
#27785=CARTESIAN_POINT ( 'NONE',  ( 92.34999999999999432, 90.00000000000002842, 90.00000000000000000 ) ) ;
#27798=CARTESIAN_POINT ( 'NONE',  ( -92.34999999999999432, -209.9999999999999716, 85.23749999999999716 ) ) ;
#27799=CARTESIAN_POINT ( 'NONE',  ( 97.64999999999999147, 90.00000000000002842, 85.87249999999998806 ) ) ;
#27806=CARTESIAN_POINT ( 'NONE',  ( 97.30629616937498838, -209.9999999999999716, 86.30906250086715659 ) ) ;
#27812=ORIENTED_EDGE ( 'NONE', *, *, #53374, .T. ) ;
#27814=CARTESIAN_POINT ( 'NONE',  ( 92.69370383062501162, -208.6684592857803295, 77.52489583420046415 ) ) ;
#27815=ORIENTED_EDGE ( 'NONE', *, *, #38044, .F. ) ;
#27816=CARTESIAN_POINT ( 'NONE',  ( 96.15314808468748708, -208.0026889286704943, 81.33489583420049485 ) ) ;
#27824=FACE_OUTER_BOUND ( 'NONE', #67614, .T. ) ;
#27837=ORIENTED_EDGE ( 'NONE', *, *, #59788, .F. ) ;
#27839=CARTESIAN_POINT ( 'NONE',  ( 97.30629616937498838, -208.6684592857803011, 76.67822916753378593 ) ) ;
#27847=CARTESIAN_POINT ( 'NONE',  ( -92.69370383062504004, 90.00000000000004263, 76.78406250086715090 ) ) ;
#27848=EDGE_CURVE ( 'NONE', #41714, #35387, #50704, .T. ) ;
#27850=CARTESIAN_POINT ( 'NONE',  ( 92.69370383062498320, 88.66845928578037217, 75.72572916753381378 ) ) ;
#27852=CARTESIAN_POINT ( 'NONE',  ( 92.34999999999999432, 90.00000000000002842, 80.47499999999999432 ) ) ;
#27853=CARTESIAN_POINT ( 'NONE',  ( -93.84685191531248449, -208.0026889286704943, 84.98614583420047097 ) ) ;
#27855=CARTESIAN_POINT ( 'NONE',  ( 96.90829729882862864, -211.8387227684681591, 74.99954709728268654 ) ) ;
#27856=FACE_OUTER_BOUND ( 'NONE', #64997, .T. ) ;
#27857=CARTESIAN_POINT ( 'NONE',  ( 96.32499999999998863, 87.70503267997126784, 81.32166666666667254 ) ) ;
#27858=CARTESIAN_POINT ( 'NONE',  ( -96.15314808468747287, -208.0026889286704943, 78.10697916753380809 ) ) ;
#27859=CIRCLE ( 'NONE', #7427, 3.299999999999983391 ) ;
#27871=CARTESIAN_POINT ( 'NONE',  ( -97.30629616937501680, 91.33154071421968467, 83.23989583420046756 ) ) ;
#27884=CARTESIAN_POINT ( 'NONE',  ( -96.15314808468745866, -211.9973110713294489, 79.74739583420048916 ) ) ;
#27891=CARTESIAN_POINT ( 'NONE',  ( 96.32499999999997442, 92.29496732002878900, 77.16770833506762983 ) ) ;
#27892=FACE_OUTER_BOUND ( 'NONE', #38690, .T. ) ;
#27900=CARTESIAN_POINT ( 'NONE',  ( 95.00000000000000000, -207.3369185715606307, 88.21406250086712930 ) ) ;
#27902=ORIENTED_EDGE ( 'NONE', *, *, #38130, .F. ) ;
#27903=EDGE_CURVE ( 'NONE', #69628, #39489, #40897, .T. ) ;
#27906=CARTESIAN_POINT ( 'NONE',  ( -93.67499999999998295, -207.7050326799711968, 84.78770833506763438 ) ) ;
#27919=( BOUNDED_CURVE ( )  B_SPLINE_CURVE ( 2, ( #63968, #74113, #69950, #24113, #16985, #12439, #57586 ),
 .UNSPECIFIED., .F., .F. ) 
 B_SPLINE_CURVE_WITH_KNOTS ( ( 3, 2, 2, 3 ),
 ( 0.1270039290051391268, 0.1340595452767650020, 0.1411153108176473325, 0.1481709449575320525 ),
 .UNSPECIFIED. ) 
 CURVE ( )  GEOMETRIC_REPRESENTATION_ITEM ( )  RATIONAL_B_SPLINE_CURVE ( ( 0.9999943314824810692, 0.8660282381031599863, 1.000000000000000000, 0.8660254037844387076, 1.000000000000000000, 0.8660278988213697682, 0.9999950100190690971 ) ) 
 REPRESENTATION_ITEM ( '' )  );
#27920=CARTESIAN_POINT ( 'NONE',  ( 96.32499999999998863, 87.70503267997126784, 88.94166666666666288 ) ) ;
#27925=VERTEX_POINT ( 'NONE', #39065 ) ;
#27927=CARTESIAN_POINT ( 'NONE',  ( 97.30629616937498838, 88.66845928578037217, 88.63739583420047552 ) ) ;
#27930=CARTESIAN_POINT ( 'NONE',  ( 96.15314808468750130, -211.9973110713294489, 86.04447916753380809 ) ) ;
#27937=CARTESIAN_POINT ( 'NONE',  ( -92.69370383062498320, -208.6684592857803011, 86.83822916753381094 ) ) ;
#27939=CARTESIAN_POINT ( 'NONE',  ( -96.15314808468751551, 88.00268892867056536, 86.09739583420049769 ) ) ;
#27941=VERTEX_POINT ( 'NONE', #62765 ) ;
#27942=CARTESIAN_POINT ( 'NONE',  ( 93.84685191531248449, 91.99731107132950569, 86.36197916753381776 ) ) ;
#27943=CARTESIAN_POINT ( 'NONE',  ( -95.00000000000002842, 87.33691857156074434, 85.99156250086714692 ) ) ;
#27949=DIRECTION ( 'NONE',  ( -0.000000000000000000, -0.000000000000000000, -1.000000000000000000 ) ) ;
#27953=VERTEX_POINT ( 'NONE', #34160 ) ;
#27955=CARTESIAN_POINT ( 'NONE',  ( -92.35000000000003695, 90.00000000000004263, 81.42749999999999488 ) ) ;
#27957=CARTESIAN_POINT ( 'NONE',  ( -97.65000000000001990, 90.00000000000004263, 78.57000000000000739 ) ) ;
#27958=DIRECTION ( 'NONE',  ( -3.061616997868382648E-16, -1.000000000000000000, 0.000000000000000000 ) ) ;
#27959=CARTESIAN_POINT ( 'NONE',  ( -96.32500000000001705, 92.29496732002878900, 79.81354166840095843 ) ) ;
#27961=CARTESIAN_POINT ( 'NONE',  ( -92.34999999999999432, -209.9999999999999716, 90.00000000000000000 ) ) ;
#27962=CARTESIAN_POINT ( 'NONE',  ( -92.34999999999999432, -209.9999999999999716, 79.52249999999999375 ) ) ;
#27964=CARTESIAN_POINT ( 'NONE',  ( -92.69370383062504004, 90.00000000000004263, 78.53031250086714010 ) ) ;
#27969=CARTESIAN_POINT ( 'NONE',  ( -92.34999999999999432, -209.9999999999999716, 82.06250000000000000 ) ) ;
#27971=CARTESIAN_POINT ( 'NONE',  ( -92.69370383062498320, -211.3315407142195852, 89.43114583420049257 ) ) ;
#27974=CARTESIAN_POINT ( 'NONE',  ( 92.69370383062498320, 88.66845928578035796, 80.96447916753382401 ) ) ;
#27975=EDGE_CURVE ( 'NONE', #51621, #74311, #57105, .T. ) ;
#27976=CARTESIAN_POINT ( 'NONE',  ( -94.99999999999997158, -207.3369185715606307, 81.38781250086715602 ) ) ;
#27984=EDGE_CURVE ( 'NONE', #50169, #22009, #56717, .T. ) ;
#27985=CARTESIAN_POINT ( 'NONE',  ( -97.30629616937501680, 88.66845928578038638, 79.69447916753381378 ) ) ;
#27986=CARTESIAN_POINT ( 'NONE',  ( 97.30629616937498838, -211.3315407142195852, 79.11239583420046984 ) ) ;
#28002=CARTESIAN_POINT ( 'NONE',  ( 97.64999999999999147, -209.9999999999999716, 83.96750000000000114 ) ) ;
#28003=CARTESIAN_POINT ( 'NONE',  ( 97.30629616937498838, 88.66845928578037217, 85.62114583420047609 ) ) ;
#28006=CARTESIAN_POINT ( 'NONE',  ( 95.00000000000000000, -213.0599564267049857, 78.09374999999998579 ) ) ;
#28014=CARTESIAN_POINT ( 'NONE',  ( -93.17363653571624127, 88.24022384386938711, 74.93163452119475210 ) ) ;
#28015=FACE_OUTER_BOUND ( 'NONE', #44153, .T. ) ;
#28019=CARTESIAN_POINT ( 'NONE',  ( -96.32499999999996021, -207.7050326799711968, 81.08354166840096866 ) ) ;
#28021=ORIENTED_EDGE ( 'NONE', *, *, #58726, .F. ) ;
#28025=CARTESIAN_POINT ( 'NONE',  ( 96.32499999999997442, 92.29496732002878900, 82.24770833506762813 ) ) ;
#28026=CARTESIAN_POINT ( 'NONE',  ( -96.32500000000001705, 87.70503267997129626, 78.75520833506763552 ) ) ;
#28030=CARTESIAN_POINT ( 'NONE',  ( 93.84685191531248449, 91.99731107132950569, 84.61572916753381435 ) ) ;
#28031=CARTESIAN_POINT ( 'NONE',  ( -94.99999999999997158, -206.9400435732949575, 86.66624999999999091 ) ) ;
#28036=EDGE_LOOP ( 'NONE', ( #7246, #31167, #10079, #71069 ) ) ;
#28044=CYLINDRICAL_SURFACE ( 'NONE', #19164, 2.649999999999985700 ) ;
#28048=CARTESIAN_POINT ( 'NONE',  ( -93.84685191531247028, -211.9973110713294489, 82.39322916753381776 ) ) ;
#28056=CARTESIAN_POINT ( 'NONE',  ( 94.99999999999998579, 87.33691857156068750, 75.19656250086714522 ) ) ;
#28060=DIRECTION ( 'NONE',  ( -0.000000000000000000, -0.000000000000000000, -1.000000000000000000 ) ) ;
#28067=CARTESIAN_POINT ( 'NONE',  ( -92.69370383062498320, -208.6684592857803295, 89.53697916753382913 ) ) ;
#28072=CARTESIAN_POINT ( 'NONE',  ( -97.30629616937501680, 88.66845928578038638, 79.53572916753380184 ) ) ;
#28087=CARTESIAN_POINT ( 'NONE',  ( 95.00000000000000000, -212.6630814284392557, 75.35531250086715715 ) ) ;
#28090=CARTESIAN_POINT ( 'NONE',  ( -92.35000000000547971, -210.0000054026037049, 81.50687481489497088 ) ) ;
#28093=CARTESIAN_POINT ( 'NONE',  ( -92.35000000000006537, -209.9999992849074317, 85.31687502647974952 ) ) ;
#28096=CARTESIAN_POINT ( 'NONE',  ( 92.35000000000000853, -209.9999872712505180, 81.82437456149078514 ) ) ;
#28097=CARTESIAN_POINT ( 'NONE',  ( 96.32499999999998863, -207.7050326799711968, 87.24833333333333485 ) ) ;
#28100=CARTESIAN_POINT ( 'NONE',  ( -92.35000000000005116, 88.47002178664754979, 81.45395833506763950 ) ) ;
#28108=CARTESIAN_POINT ( 'NONE',  ( 92.35000000000002274, -211.5299782133524502, 78.06729166840096923 ) ) ;
#28109=CARTESIAN_POINT ( 'NONE',  ( 92.34999999999999432, 88.47002178664753558, 81.79791666666666572 ) ) ;
#28111=CARTESIAN_POINT ( 'NONE',  ( 96.32499999999998863, -207.7050326799711968, 75.26270833506764291 ) ) ;
#28114=CARTESIAN_POINT ( 'NONE',  ( -92.34999999999999432, -209.9999999999999716, 82.77687500173431090 ) ) ;
#28118=CARTESIAN_POINT ( 'NONE',  ( -97.30629616937501680, 91.33154071421968467, 85.93864583420051417 ) ) ;
#28119=CARTESIAN_POINT ( 'NONE',  ( 97.30629616937498838, 88.66845928578037217, 77.84239583420045960 ) ) ;
#28120=ORIENTED_EDGE ( 'NONE', *, *, #59426, .F. ) ;
#28127=CARTESIAN_POINT ( 'NONE',  ( -92.69370383062498320, -208.6684592857803011, 77.31322916753380525 ) ) ;
#28131=CARTESIAN_POINT ( 'NONE',  ( 97.64999999999997726, 88.47002178664752137, 80.10458333333330927 ) ) ;
#28133=CARTESIAN_POINT ( 'NONE',  ( 92.34999999999999432, 90.00000000000002842, 77.93499999999998806 ) ) ;
#28135=CARTESIAN_POINT ( 'NONE',  ( -94.99999999999997158, -213.0599564267049857, 78.09374999999998579 ) ) ;
#28137=CARTESIAN_POINT ( 'NONE',  ( -96.15314808468747287, -208.0026889286704943, 89.69572916753382685 ) ) ;
#28140=CARTESIAN_POINT ( 'NONE',  ( -92.35000000000003695, 90.00000000000004263, 76.98250000000000171 ) ) ;
#28148=CARTESIAN_POINT ( 'NONE',  ( 96.15314808468748708, 88.00268892867053694, 86.04447916753380809 ) ) ;
#28149=CARTESIAN_POINT ( 'NONE',  ( -93.07557990970624928, -211.8218417373838349, 75.00000000000000000 ) ) ;
#28152=CARTESIAN_POINT ( 'NONE',  ( -95.00000000000002842, 90.00000000000004263, 90.00000000000000000 ) ) ;
#28158=( BOUNDED_CURVE ( )  B_SPLINE_CURVE ( 2, ( #71690, #20580, #61178, #43533, #38234, #26202, #66811 ),
 .UNSPECIFIED., .F., .F. ) 
 B_SPLINE_CURVE_WITH_KNOTS ( ( 3, 2, 2, 3 ),
 ( 0.1693384224419981210, 0.1763941385220586522, 0.1834499040629413158, 0.1905056698837213069 ),
 .UNSPECIFIED. ) 
 CURVE ( )  GEOMETRIC_REPRESENTATION_ITEM ( )  RATIONAL_B_SPLINE_CURVE ( ( 0.9999981216929102468, 0.8660263429445670402, 1.000000000000000000, 0.8660254037844387076, 1.000000000000000000, 0.8660254037844387076, 1.000000000000000000 ) ) 
 REPRESENTATION_ITEM ( '' )  );
#28162=EDGE_CURVE ( 'NONE', #38565, #13389, #25945, .T. ) ;
#28164=CARTESIAN_POINT ( 'NONE',  ( -93.84685191531252713, 88.00268892867056536, 89.21947916753380525 ) ) ;
#28166=EDGE_CURVE ( 'NONE', #54291, #59733, #7731, .T. ) ;
#28167=CARTESIAN_POINT ( 'NONE',  ( -96.32499999999996021, -212.2949673200287179, 83.75583333333332803 ) ) ;
#28170=CARTESIAN_POINT ( 'NONE',  ( 92.34999999999999432, 90.00000000000002842, 85.55499999999999261 ) ) ;
#28173=CARTESIAN_POINT ( 'NONE',  ( -96.32500000000001705, 87.70503267997129626, 77.48520833506763950 ) ) ;
#28174=ADVANCED_FACE ( 'NONE', ( #33219 ), #5058, .F. ) ;
#28176=CARTESIAN_POINT ( 'NONE',  ( 95.00000000000000000, -212.6630814284392557, 85.51531250086713953 ) ) ;
#28178=ORIENTED_EDGE ( 'NONE', *, *, #37797, .T. ) ;
#28179=LINE ( 'NONE', #11619, #49984 ) ;
#28183=CARTESIAN_POINT ( 'NONE',  ( 96.15314808468748708, -208.0026889286704943, 78.63614583420047666 ) ) ;
#28188=CARTESIAN_POINT ( 'NONE',  ( 93.84685191531249870, -208.0026889286704943, 82.71072916753381321 ) ) ;
#28199=CARTESIAN_POINT ( 'NONE',  ( 92.35000000000000853, -211.5299782133524218, 76.79729166840095900 ) ) ;
#28200=CARTESIAN_POINT ( 'NONE',  ( 97.64999999999999147, -209.9999999999999716, 85.31687500173428873 ) ) ;
#28210=CARTESIAN_POINT ( 'NONE',  ( 97.30629616937498838, -211.3315407142195852, 76.57239583420046358 ) ) ;
#28215=EDGE_LOOP ( 'NONE', ( #16713, #24473, #61539, #69549 ) ) ;
#28216=DIRECTION ( 'NONE',  ( 1.000000000000000000, 0.000000000000000000, 0.000000000000000000 ) ) ;
#28217=CARTESIAN_POINT ( 'NONE',  ( -92.69370383062502583, 91.33154071421968467, 76.20197916753382117 ) ) ;
#28219=CARTESIAN_POINT ( 'NONE',  ( 94.99999999999998579, 92.66308142843935514, 74.87906250086713555 ) ) ;
#28222=CARTESIAN_POINT ( 'NONE',  ( -97.30629616937495996, -209.9999999999999716, 85.83281250086714920 ) ) ;
#28226=CARTESIAN_POINT ( 'NONE',  ( 95.00000000000000000, -206.9400435732949575, 87.93624999999998693 ) ) ;
#28227=CARTESIAN_POINT ( 'NONE',  ( -92.69370383062498320, -208.6684592857803295, 77.31322916753380525 ) ) ;
#28232=CARTESIAN_POINT ( 'NONE',  ( -97.65000000000007674, 91.52997821335250705, 76.61208333333333087 ) ) ;
#28233=DIRECTION ( 'NONE',  ( 0.000000000000000000, -0.000000000000000000, -1.000000000000000000 ) ) ;
#28234=CARTESIAN_POINT ( 'NONE',  ( -97.30629616937501680, 90.00000000000004263, 82.02281250086714692 ) ) ;
#28240=EDGE_CURVE ( 'NONE', #40893, #56929, #67237, .T. ) ;
#28242=CARTESIAN_POINT ( 'NONE',  ( 97.64999999999999147, -209.9999999999999716, 89.12687500173430521 ) ) ;
#28243=CARTESIAN_POINT ( 'NONE',  ( 92.35000000000000853, -209.9999999999999716, 90.00000000000000000 ) ) ;
#28246=CARTESIAN_POINT ( 'NONE',  ( -94.99999999999997158, -212.6630814284392557, 79.80031250086715033 ) ) ;
#28249=ADVANCED_FACE ( 'NONE', ( #58386 ), #29070, .F. ) ;
#28254=CARTESIAN_POINT ( 'NONE',  ( -97.65000000000001990, 90.00000000000004263, 80.55437500173430010 ) ) ;
#28256=CARTESIAN_POINT ( 'NONE',  ( -97.64999999980587120, -210.0000198427943587, 86.27002759516035724 ) ) ;
#28264=DIRECTION ( 'NONE',  ( -0.000000000000000000, -0.000000000000000000, 1.000000000000000000 ) ) ;
#28266=CARTESIAN_POINT ( 'NONE',  ( 97.30629616937498838, -208.6684592857803295, 86.83822916753381094 ) ) ;
#28274=CARTESIAN_POINT ( 'NONE',  ( 95.00000000000000000, -213.0599564267049857, 81.90375000000000227 ) ) ;
#28276=CARTESIAN_POINT ( 'NONE',  ( -92.34999999999999432, -209.9999999999999716, 75.07749999999998636 ) ) ;
#28278=VERTEX_POINT ( 'NONE', #64408 ) ;
#28282=CARTESIAN_POINT ( 'NONE',  ( 94.99999999999998579, 86.94004357329500010, 89.52375000000000682 ) ) ;
#28283=CYLINDRICAL_SURFACE ( 'NONE', #60004, 2.649999999999999467 ) ;
#28288=ORIENTED_EDGE ( 'NONE', *, *, #869, .F. ) ;
#28289=CARTESIAN_POINT ( 'NONE',  ( 93.84685191531248449, 91.99731107132950569, 83.82197916753381151 ) ) ;
#28292=CARTESIAN_POINT ( 'NONE',  ( 97.30629616937498838, -208.6684592857803011, 84.93322916753379559 ) ) ;
#28297=CARTESIAN_POINT ( 'NONE',  ( -92.34999999999999432, -209.9999999999999716, 89.04749999999999943 ) ) ;
#28301=CARTESIAN_POINT ( 'NONE',  ( -96.15314808468747287, -208.0026889286704943, 86.99697916753380866 ) ) ;
#28302=CARTESIAN_POINT ( 'NONE',  ( -92.69370383062504004, 90.00000000000004263, 85.67406250086715147 ) ) ;
#28303=ORIENTED_EDGE ( 'NONE', *, *, #8676, .T. ) ;
#28305=CARTESIAN_POINT ( 'NONE',  ( 94.99999999999998579, 87.33691857156068750, 82.81656250086713555 ) ) ;
#28306=CARTESIAN_POINT ( 'NONE',  ( -97.30629616937501680, 91.33154071421968467, 83.87489583420047268 ) ) ;
#28310=DIRECTION ( 'NONE',  ( 1.000000000000000000, 0.000000000000000000, 0.000000000000000000 ) ) ;
#28312=CARTESIAN_POINT ( 'NONE',  ( 97.64999999999999147, 90.00000000000002842, 87.14249999999999829 ) ) ;
#28321=CARTESIAN_POINT ( 'NONE',  ( -96.32500000000001705, 87.70503267997129626, 78.04083333333333883 ) ) ;
#28325=CARTESIAN_POINT ( 'NONE',  ( -93.67499999999998295, -207.7050326799711968, 89.78833333333332689 ) ) ;
#28329=CARTESIAN_POINT ( 'NONE',  ( -96.15314808468752972, 91.99731107132950569, 78.10697916753380809 ) ) ;
#28338=CARTESIAN_POINT ( 'NONE',  ( -97.65000000000001990, 91.52997821335253548, 82.32708333333334849 ) ) ;
#28339=CARTESIAN_POINT ( 'NONE',  ( -94.99999999999997158, -207.3369185715606307, 89.00781250086716057 ) ) ;
#28344=CARTESIAN_POINT ( 'NONE',  ( 97.30629616937498838, 90.00000000000002842, 78.05406250086716113 ) ) ;
#28345=CARTESIAN_POINT ( 'NONE',  ( -96.15314808468745866, -211.9973110713294489, 78.47739583420049314 ) ) ;
#28348=CARTESIAN_POINT ( 'NONE',  ( -97.64999999996715019, 90.00000839192523472, 86.90410584365564262 ) ) ;
#28353=CARTESIAN_POINT ( 'NONE',  ( -95.00000000000002842, 87.33691857156074434, 79.80031250086715033 ) ) ;
#28354=CARTESIAN_POINT ( 'NONE',  ( 96.15314808468750130, -211.9973110713294489, 80.32947916753380468 ) ) ;
#28362=( BOUNDED_CURVE ( )  B_SPLINE_CURVE ( 2, ( #52198, #22531, #10878, #745, #28902, #23634, #45847, #56752, #5996 ),
 .UNSPECIFIED., .F., .F. ) 
 B_SPLINE_CURVE_WITH_KNOTS ( ( 3, 2, 2, 2, 3 ),
 ( 0.1058364832022827828, 0.1128922486541179687, 0.1199480141950002993, 0.1270037797358826437, 0.1270039290051390157 ),
 .UNSPECIFIED. ) 
 CURVE ( )  GEOMETRIC_REPRESENTATION_ITEM ( )  RATIONAL_B_SPLINE_CURVE ( ( 1.000000000000000000, 0.8660254037844387076, 1.000000000000000000, 0.8660254037844387076, 1.000000000000000000, 0.8660254037844387076, 1.000000000000000000, 0.9999971656812808307, 0.9999943314824852880 ) ) 
 REPRESENTATION_ITEM ( '' )  );
#28365=CARTESIAN_POINT ( 'NONE',  ( -97.65000000000001990, 90.00000000000004263, 79.20499999999999829 ) ) ;
#28366=EDGE_CURVE ( 'NONE', #55652, #9807, #2935, .T. ) ;
#28367=EDGE_CURVE ( 'NONE', #6700, #10235, #5785, .T. ) ;
#28371=EDGE_LOOP ( 'NONE', ( #66116, #73531, #570 ) ) ;
#28372=CARTESIAN_POINT ( 'NONE',  ( 93.84685191531251292, -211.9973110713294489, 75.30239583420048177 ) ) ;
#28376=CARTESIAN_POINT ( 'NONE',  ( 93.84685191531248449, 91.99731107132950569, 82.71072916753381321 ) ) ;
#28377=CARTESIAN_POINT ( 'NONE',  ( 92.35000000000002274, -211.5299782133524502, 78.62291666666668277 ) ) ;
#28384=DIRECTION ( 'NONE',  ( -0.000000000000000000, -0.000000000000000000, 1.000000000000000000 ) ) ;
#28389=CARTESIAN_POINT ( 'NONE',  ( -92.34999999999999432, -209.9999999999999716, 83.41187500173430180 ) ) ;
#28393=CARTESIAN_POINT ( 'NONE',  ( 93.67499999999998295, 92.29496732002878900, 79.17854166840096752 ) ) ;
#28394=CARTESIAN_POINT ( 'NONE',  ( -96.32500000000001705, 92.29496732002878900, 80.44854166840097776 ) ) ;
#28396=CARTESIAN_POINT ( 'NONE',  ( 97.30629616937498838, 91.33154071421968467, 85.09197916753380753 ) ) ;
#28399=DIRECTION ( 'NONE',  ( -0.000000000000000000, -0.000000000000000000, 1.000000000000000000 ) ) ;
#28401=FACE_OUTER_BOUND ( 'NONE', #17464, .T. ) ;
#28406=CARTESIAN_POINT ( 'NONE',  ( 97.64999999981932888, -210.0000309431867436, 78.33187387208516839 ) ) ;
#28420=CARTESIAN_POINT ( 'NONE',  ( -97.30629616937497417, -208.6684592857803011, 82.12864583420048348 ) ) ;
#28421=ORIENTED_EDGE ( 'NONE', *, *, #7586, .T. ) ;
#28425=CARTESIAN_POINT ( 'NONE',  ( -94.95306897617061281, -212.6495843973424655, 75.00000002508416230 ) ) ;
#28428=CARTESIAN_POINT ( 'NONE',  ( 94.99999999999998579, 92.66308142843932671, 75.51406250086714067 ) ) ;
#28432=CARTESIAN_POINT ( 'NONE',  ( -97.64999999960622290, -209.9999706925929672, 76.74344264316562203 ) ) ;
#28433=CARTESIAN_POINT ( 'NONE',  ( -92.35000000000003695, 89.99999997442942856, 84.04687500080852658 ) ) ;
#28437=CARTESIAN_POINT ( 'NONE',  ( 96.15314808468748708, 88.00268892867053694, 87.47322916753381605 ) ) ;
#28438=CARTESIAN_POINT ( 'NONE',  ( -97.30629616937495996, -209.9999999999999716, 89.80156250086714920 ) ) ;
#28442=CARTESIAN_POINT ( 'NONE',  ( -93.84685191531252713, 88.00268892867056536, 79.05947916753380866 ) ) ;
#28443=LINE ( 'NONE', #67568, #60996 ) ;
#28447=CARTESIAN_POINT ( 'NONE',  ( 93.67500000000001137, -212.2949673200287179, 80.02520833506763154 ) ) ;
#28449=CARTESIAN_POINT ( 'NONE',  ( 97.64999999999999147, 90.00000000000002842, 83.33250000000001023 ) ) ;
#28453=CARTESIAN_POINT ( 'NONE',  ( 95.00000000000000000, -207.3369185715606307, 76.94281250086714863 ) ) ;
#28456=AXIS2_PLACEMENT_3D ( 'NONE', #35549, #58482, #64502 ) ;
#28458=CARTESIAN_POINT ( 'NONE',  ( 92.69370383062501162, -208.6684592857803295, 85.93864583420051417 ) ) ;
#28464=CARTESIAN_POINT ( 'NONE',  ( 95.00000000000000000, -206.9400435732949575, 88.57124999999999204 ) ) ;
#28471=DIRECTION ( 'NONE',  ( -1.000000000000000000, -0.000000000000000000, -0.000000000000000000 ) ) ;
#28472=CARTESIAN_POINT ( 'NONE',  ( 95.00000000000000000, -213.0599564267049857, 78.17312500173430578 ) ) ;
#28473=CARTESIAN_POINT ( 'NONE',  ( 92.34999999999999432, 90.00000000000002842, 83.01499999999998636 ) ) ;
#28479=DIRECTION ( 'NONE',  ( -0.000000000000000000, -0.000000000000000000, 1.000000000000000000 ) ) ;
#28481=PLANE ( 'NONE',  #6815 ) ;
#28482=CARTESIAN_POINT ( 'NONE',  ( -97.30629616937501680, 88.66845928578038638, 80.32947916753381890 ) ) ;
#28483=CARTESIAN_POINT ( 'NONE',  ( 97.30629616937498838, 90.00000000000002842, 77.89531250086714920 ) ) ;
#28489=ORIENTED_EDGE ( 'NONE', *, *, #169, .T. ) ;
#28491=CARTESIAN_POINT ( 'NONE',  ( -97.30629616937497417, -208.6684592857803011, 78.15989583420048348 ) ) ;
#28501=CARTESIAN_POINT ( 'NONE',  ( -94.99999999999997158, -207.3369185715606307, 76.14906250086716000 ) ) ;
#28513=CARTESIAN_POINT ( 'NONE',  ( 94.99999999999998579, 92.66308142843932671, 84.40406250086714124 ) ) ;
#28526=DIRECTION ( 'NONE',  ( 1.000000000000000000, -0.000000000000000000, 0.000000000000000000 ) ) ;
#28529=CARTESIAN_POINT ( 'NONE',  ( -92.34999999999999432, -211.5299782133524502, 80.73958333333332860 ) ) ;
#28531=CARTESIAN_POINT ( 'NONE',  ( 97.64999999999989200, 88.47002178664747873, 85.81958333333332689 ) ) ;
#28534=EDGE_CURVE ( 'NONE', #60050, #50746, #20750, .T. ) ;
#28536=CARTESIAN_POINT ( 'NONE',  ( -93.67500000000003979, 92.29496732002878900, 77.08833333333332405 ) ) ;
#28537=CARTESIAN_POINT ( 'NONE',  ( 94.99999999999998579, 90.00000000000002842, 90.00000000000000000 ) ) ;
#28539=CARTESIAN_POINT ( 'NONE',  ( -92.35000000000006537, 90.00000034979574082, 77.69687501385438111 ) ) ;
#28540=CARTESIAN_POINT ( 'NONE',  ( 93.84685191531249870, -208.0026889286704943, 85.25072916753381946 ) ) ;
#28546=CARTESIAN_POINT ( 'NONE',  ( 95.00000000000000000, -212.6630814284392557, 78.37156250086714238 ) ) ;
#28549=CARTESIAN_POINT ( 'NONE',  ( 92.69370383062501162, -208.6684592857803011, 81.49364583420047836 ) ) ;
#28550=VECTOR ( 'NONE', #36665, 1000.000000000000000 ) ;
#28558=CARTESIAN_POINT ( 'NONE',  ( 92.35000000000000853, -209.9999678257246103, 76.74437388893714740 ) ) ;
#28559=CARTESIAN_POINT ( 'NONE',  ( 92.35000000000002274, -211.5299782133524502, 85.68729166840097378 ) ) ;
#28564=( BOUNDED_CURVE ( )  B_SPLINE_CURVE ( 2, ( #70272, #18778, #13142, #437, #45904, #35698, #36082 ),
 .UNSPECIFIED., .F., .F. ) 
 B_SPLINE_CURVE_WITH_KNOTS ( ( 3, 2, 2, 3 ),
 ( 0.5416666666666665186, 0.5486111111111110494, 0.5555555555555553582, 0.5624999999999997780 ),
 .UNSPECIFIED. ) 
 CURVE ( )  GEOMETRIC_REPRESENTATION_ITEM ( )  RATIONAL_B_SPLINE_CURVE ( ( 1.000000000000002220, 0.8660254037844365982, 1.000000000000000000, 0.8660254037844387076, 1.000000000000000000, 0.8660254037844430375, 0.9999999999999956701 ) ) 
 REPRESENTATION_ITEM ( '' )  );
#28568=VERTEX_POINT ( 'NONE', #45179 ) ;
#28581=VECTOR ( 'NONE', #68612, 1000.000000000000000 ) ;
#28583=CARTESIAN_POINT ( 'NONE',  ( -93.67500000000003979, 87.70503267997129626, 87.67166666666666686 ) ) ;
#28585=CARTESIAN_POINT ( 'NONE',  ( 92.69370383062498320, 88.66845928578037217, 75.09072916753382287 ) ) ;
#28587=ORIENTED_EDGE ( 'NONE', *, *, #13512, .T. ) ;
#28588=( BOUNDED_CURVE ( )  B_SPLINE_CURVE ( 2, ( #45808, #56714, #52159, #39786, #69816, #34132, #68732 ),
 .UNSPECIFIED., .F., .F. ) 
 B_SPLINE_CURVE_WITH_KNOTS ( ( 3, 2, 2, 3 ),
 ( 0.3175094496506953301, 0.3245652148805889814, 0.3316209804214713674, 0.3386766260338263668 ),
 .UNSPECIFIED. ) 
 CURVE ( )  GEOMETRIC_REPRESENTATION_ITEM ( )  RATIONAL_B_SPLINE_CURVE ( ( 1.000000000000000000, 0.8660254037844387076, 1.000000000000000000, 0.8660254037844387076, 1.000000000000000000, 0.8660276809825581124, 0.9999954456811732673 ) ) 
 REPRESENTATION_ITEM ( '' )  );
#28590=CARTESIAN_POINT ( 'NONE',  ( -97.30629616937495996, -209.9999999999999716, 84.56281250086713897 ) ) ;
#28595=CARTESIAN_POINT ( 'NONE',  ( -93.84685191531247028, -211.9973110713294489, 76.51947916753380241 ) ) ;
#28602=CARTESIAN_POINT ( 'NONE',  ( -96.15314808468752972, 91.99731107132950569, 78.10697916753380809 ) ) ;
#28618=CARTESIAN_POINT ( 'NONE',  ( 97.64999999999821512, 90.00000306648260562, 75.79187510780352000 ) ) ;
#28619=CARTESIAN_POINT ( 'NONE',  ( -96.15314808468747287, -208.0026889286704943, 78.26572916753382003 ) ) ;
#28624=DIRECTION ( 'NONE',  ( 1.000000000000000000, 0.000000000000000000, 0.000000000000000000 ) ) ;
#28639=VERTEX_POINT ( 'NONE', #33131 ) ;
#28644=CARTESIAN_POINT ( 'NONE',  ( -93.67499999999998295, -212.2949673200287179, 80.13104166840095388 ) ) ;
#28661=CARTESIAN_POINT ( 'NONE',  ( 96.15314808468748708, 88.00268892867053694, 86.67947916753381321 ) ) ;
#28663=CARTESIAN_POINT ( 'NONE',  ( 97.30629616937498838, -211.3315407142195852, 80.38239583420049428 ) ) ;
#28668=CARTESIAN_POINT ( 'NONE',  ( -92.34999999999999432, -209.9999999999999716, 90.00000000000000000 ) ) ;
#28669=CARTESIAN_POINT ( 'NONE',  ( 92.35000000000000853, -209.9999999999999716, 82.37999999999999545 ) ) ;
#28675=CARTESIAN_POINT ( 'NONE',  ( -94.99999999999997158, -212.6630814284392557, 89.16656250086712987 ) ) ;
#28676=CARTESIAN_POINT ( 'NONE',  ( -93.84685191531254134, 91.99731107132950569, 87.04989583420048405 ) ) ;
#28678=CARTESIAN_POINT ( 'NONE',  ( 93.84685191531248449, 91.99731107132950569, 84.45697916753380241 ) ) ;
#28679=CARTESIAN_POINT ( 'NONE',  ( -93.84685191531252713, 88.00268892867056536, 86.04447916753380809 ) ) ;
#28681=CARTESIAN_POINT ( 'NONE',  ( -93.67500000000003979, 87.70503267997129626, 78.86104166840097207 ) ) ;
#28684=CYLINDRICAL_SURFACE ( 'NONE', #3268, 2.649999999999985700 ) ;
#28686=CARTESIAN_POINT ( 'NONE',  ( -92.69370383062498320, -208.6684592857803295, 86.83822916753381094 ) ) ;
#28689=CARTESIAN_POINT ( 'NONE',  ( 92.35000000000000853, -209.9999999999999716, 90.00000000000000000 ) ) ;
#28697=EDGE_CURVE ( 'NONE', #11224, #55326, #21407, .T. ) ;
#28699=CARTESIAN_POINT ( 'NONE',  ( -97.65000000000001990, 91.52997821335253548, 78.51708333333334622 ) ) ;
#28701=CARTESIAN_POINT ( 'NONE',  ( -93.59478774260932710, -208.1321859400969174, 74.80441578173234518 ) ) ;
#28705=CARTESIAN_POINT ( 'NONE',  ( -97.64999999999996305, -209.9999999999999716, 78.57000000000000739 ) ) ;
#28708=CARTESIAN_POINT ( 'NONE',  ( -93.84685191531252713, 88.00268892867056536, 77.78947916753381264 ) ) ;
#28716=CARTESIAN_POINT ( 'NONE',  ( -92.69370383062498320, -208.6684592857803011, 88.90197916753382401 ) ) ;
#28717=( BOUNDED_CURVE ( )  B_SPLINE_CURVE ( 2, ( #67371, #44825, #33520, #10979, #56482, #67750, #40289 ),
 .UNSPECIFIED., .F., .F. ) 
 B_SPLINE_CURVE_WITH_KNOTS ( ( 3, 2, 2, 3 ),
 ( 0.08333333333333288462, 0.09027777777777759582, 0.09722222222222230703, 0.1041666666666670182 ),
 .UNSPECIFIED. ) 
 CURVE ( )  GEOMETRIC_REPRESENTATION_ITEM ( )  RATIONAL_B_SPLINE_CURVE ( ( 1.000000000000008660, 0.8660254037844301589, 1.000000000000000000, 0.8660254037844387076, 1.000000000000000000, 0.8660254037844320463, 1.000000000000006661 ) ) 
 REPRESENTATION_ITEM ( '' )  );
#28719=CARTESIAN_POINT ( 'NONE',  ( 92.69370383062498320, 91.33154071421968467, 75.77864583420048916 ) ) ;
#28721=CARTESIAN_POINT ( 'NONE',  ( -92.69370383062498320, -211.3315407142195852, 79.27114583420048177 ) ) ;
#28724=LINE ( 'NONE', #47503, #64116 ) ;
#28725=CARTESIAN_POINT ( 'NONE',  ( -96.32499999999996021, -212.2949673200287179, 75.50083333333331836 ) ) ;
#28728=AXIS2_PLACEMENT_3D ( 'NONE', #53312, #48406, #37142 ) ;
#28730=CARTESIAN_POINT ( 'NONE',  ( -93.33920801875068207, 88.39975876321990711, 74.80065669543250806 ) ) ;
#28731=CARTESIAN_POINT ( 'NONE',  ( 97.30629616937498838, -211.3315407142195852, 81.01739583420048518 ) ) ;
#28732=VERTEX_POINT ( 'NONE', #16973 ) ;
#28738=CARTESIAN_POINT ( 'NONE',  ( 92.35000000000000853, -209.9999999999999716, 77.29999999999999716 ) ) ;
#28746=CARTESIAN_POINT ( 'NONE',  ( 95.00000000000000000, -206.9400435732949575, 79.76062500173429726 ) ) ;
#28750=CARTESIAN_POINT ( 'NONE',  ( 92.69370383062498320, 88.66845928578037217, 84.13947916753383538 ) ) ;
#28751=CARTESIAN_POINT ( 'NONE',  ( 97.64999999999997726, -208.4700217866474645, 78.94041666666666401 ) ) ;
#28764=DIRECTION ( 'NONE',  ( 1.000000000000000000, 0.000000000000000000, 0.000000000000000000 ) ) ;
#28768=CARTESIAN_POINT ( 'NONE',  ( -93.67499999999998295, -212.2949673200287179, 82.67104166840096013 ) ) ;
#28771=ORIENTED_EDGE ( 'NONE', *, *, #44211, .F. ) ;
#28772=CARTESIAN_POINT ( 'NONE',  ( 92.34999999999999432, 91.52997821335252127, 77.96145833506763267 ) ) ;
#28773=CARTESIAN_POINT ( 'NONE',  ( -92.35000000000003695, 90.00000000000004263, 80.23687500173429044 ) ) ;
#28776=ORIENTED_EDGE ( 'NONE', *, *, #48064, .F. ) ;
#28777=CARTESIAN_POINT ( 'NONE',  ( 93.84685191531248449, 88.00268892867053694, 79.74739583420048916 ) ) ;
#28779=CARTESIAN_POINT ( 'NONE',  ( 99.99999999999998579, 95.00000000000001421, -90.00000000000002842 ) ) ;
#28785=LINE ( 'NONE', #10758, #18363 ) ;
#28790=ORIENTED_EDGE ( 'NONE', *, *, #18182, .F. ) ;
#28796=CARTESIAN_POINT ( 'NONE',  ( 95.00000000000000000, -209.9999999999999716, 90.00000000000000000 ) ) ;
#28797=CARTESIAN_POINT ( 'NONE',  ( -96.15314808468747287, -208.0026889286704943, 80.17072916753382117 ) ) ;
#28807=CARTESIAN_POINT ( 'NONE',  ( 96.15314808468748708, 91.99731107132950569, 74.82614583420047438 ) ) ;
#28816=( BOUNDED_CURVE ( )  B_SPLINE_CURVE ( 2, ( #69247, #68520, #46319, #62899, #18475, #17736, #18117, #58335, #46690 ),
 .UNSPECIFIED., .F., .F. ) 
 B_SPLINE_CURVE_WITH_KNOTS ( ( 3, 2, 2, 2, 3 ),
 ( 0.2751748541904411316, 0.2822306216352944985, 0.2892863871761764960, 0.2963421527170585490, 0.2963422021981251264 ),
 .UNSPECIFIED. ) 
 CURVE ( )  GEOMETRIC_REPRESENTATION_ITEM ( )  RATIONAL_B_SPLINE_CURVE ( ( 1.000000000000000000, 0.8660254037844387076, 1.000000000000000000, 0.8660254037844387076, 1.000000000000000000, 0.8660254037844387076, 1.000000000000000000, 0.9999990604554704898, 0.9999981209241187718 ) ) 
 REPRESENTATION_ITEM ( '' )  );
#28817=CARTESIAN_POINT ( 'NONE',  ( 93.84685191531248449, 88.00268892867053694, 88.63739583420048973 ) ) ;
#28821=CARTESIAN_POINT ( 'NONE',  ( -96.15314808468752972, 91.99731107132950569, 81.28197916753380525 ) ) ;
#28826=CARTESIAN_POINT ( 'NONE',  ( 93.67499999999999716, 87.70503267997126784, 83.12083333333332291 ) ) ;
#28828=CIRCLE ( 'NONE', #61260, 3.299999999999997158 ) ;
#28830=CARTESIAN_POINT ( 'NONE',  ( 93.84685191531249870, -208.0026889286704943, 75.72572916753382799 ) ) ;
#28836=CARTESIAN_POINT ( 'NONE',  ( 95.00000000000000000, -212.6630814284392557, 85.51531250086715374 ) ) ;
#28842=CARTESIAN_POINT ( 'NONE',  ( 95.00000000000000000, -213.0599564267049857, 81.98312500173430806 ) ) ;
#28843=CARTESIAN_POINT ( 'NONE',  ( 95.00000000000000000, -206.9400435732949575, 87.30124999999999602 ) ) ;
#28848=ORIENTED_EDGE ( 'NONE', *, *, #18001, .T. ) ;
#28853=CARTESIAN_POINT ( 'NONE',  ( -97.30629616937501680, 90.00000000000004263, 87.26156250086715715 ) ) ;
#28857=CARTESIAN_POINT ( 'NONE',  ( -97.64999999999993463, 88.47002178664750716, 83.70291666666668107 ) ) ;
#28858=CARTESIAN_POINT ( 'NONE',  ( 97.64999999999997726, -208.4700217866474645, 75.84479166840098685 ) ) ;
#28859=CARTESIAN_POINT ( 'NONE',  ( 94.99999999999998579, 86.94004357329500010, 78.09374999999998579 ) ) ;
#28863=CARTESIAN_POINT ( 'NONE',  ( -97.64999999999996305, -209.9999999999999716, 84.28499999999999659 ) ) ;
#28864=ORIENTED_EDGE ( 'NONE', *, *, #61789, .T. ) ;
#28865=CARTESIAN_POINT ( 'NONE',  ( -92.35000000000003695, 90.00000000000004263, 89.12687500173430521 ) ) ;
#28866=CARTESIAN_POINT ( 'NONE',  ( -93.84685191531254134, 91.99731107132950569, 80.69989583420047552 ) ) ;
#28867=ADVANCED_FACE ( 'NONE', ( #70296 ), #48857, .F. ) ;
#28868=CARTESIAN_POINT ( 'NONE',  ( 92.69370383062498320, 90.00000000000002842, 89.80156250086714920 ) ) ;
#28872=CARTESIAN_POINT ( 'NONE',  ( 92.35000000000000853, -209.9999999999999716, 85.55499999999999261 ) ) ;
#28877=CARTESIAN_POINT ( 'NONE',  ( -93.84685191531248449, -208.0026889286704943, 78.00114583420048575 ) ) ;
#28878=ORIENTED_EDGE ( 'NONE', *, *, #30469, .F. ) ;
#28886=ORIENTED_EDGE ( 'NONE', *, *, #20562, .F. ) ;
#28887=CARTESIAN_POINT ( 'NONE',  ( -92.69370383062498320, -208.6684592857803011, 76.04322916753380923 ) ) ;
#28893=AXIS2_PLACEMENT_3D ( 'NONE', #39448, #16888, #62391 ) ;
#28896=CARTESIAN_POINT ( 'NONE',  ( 97.30629616937498838, 88.66845928578035796, 86.09739583420048348 ) ) ;
#28897=CARTESIAN_POINT ( 'NONE',  ( -93.67499999999998295, -212.2949673200287179, 83.86166666666666458 ) ) ;
#28898=CARTESIAN_POINT ( 'NONE',  ( -97.30629616937501680, 90.00000000000004263, 89.64281250086713726 ) ) ;
#28902=CARTESIAN_POINT ( 'NONE',  ( 93.67500000000001137, -212.2949673200287179, 87.64520833506762187 ) ) ;
#28914=CARTESIAN_POINT ( 'NONE',  ( -92.35000000000003695, 90.00000000000004263, 76.98250000000000171 ) ) ;
#28916=DIRECTION ( 'NONE',  ( 1.000000000000000000, 0.000000000000000000, 0.000000000000000000 ) ) ;
#28919=CARTESIAN_POINT ( 'NONE',  ( 93.84685191531249870, -208.0026889286704943, 86.52072916753382970 ) ) ;
#28924=LINE ( 'NONE', #17277, #63175 ) ;
#28925=EDGE_LOOP ( 'NONE', ( #57232, #58744, #56972, #67341 ) ) ;
#28929=CARTESIAN_POINT ( 'NONE',  ( 92.69370383062501162, -211.3315407142195852, 82.23447916753383424 ) ) ;
#28942=CARTESIAN_POINT ( 'NONE',  ( 92.35000000039376289, -209.9999706925934504, 76.74344264317686282 ) ) ;
#28943=CARTESIAN_POINT ( 'NONE',  ( 92.35000000000002274, -211.5299782133524502, 86.95729166840096980 ) ) ;
#28959=CARTESIAN_POINT ( 'NONE',  ( -23.50044424985255276, 0.001194404164626844313, -64.00000000000000000 ) ) ;
#28962=CARTESIAN_POINT ( 'NONE',  ( -97.65000000000001990, 90.00000000000004263, 88.73000000000000398 ) ) ;
#28963=ADVANCED_FACE ( 'NONE', ( #59790 ), #31198, .F. ) ;
#28967=ORIENTED_EDGE ( 'NONE', *, *, #30646, .F. ) ;
#28969=CARTESIAN_POINT ( 'NONE',  ( -92.69370383062498320, -209.9999999999999716, 85.51531250086713953 ) ) ;
#28973=CARTESIAN_POINT ( 'NONE',  ( 92.55058773059857913, -210.6792855350292086, 74.93153462041254897 ) ) ;
#28975=CARTESIAN_POINT ( 'NONE',  ( -97.30629616937497417, -211.3315407142195852, 76.99572916753380980 ) ) ;
#28981=CARTESIAN_POINT ( 'NONE',  ( -93.84685191531252713, 88.00268892867056536, 77.15447916753380753 ) ) ;
#28985=CARTESIAN_POINT ( 'NONE',  ( 92.35000000007821086, 90.00001303125209517, 79.28395951162845279 ) ) ;
#28992=CARTESIAN_POINT ( 'NONE',  ( -93.67500000000003979, 92.29496732002878900, 85.42270833506762528 ) ) ;
#28993=CARTESIAN_POINT ( 'NONE',  ( -97.64999999999994884, -208.4700217866474645, 89.94708333333333883 ) ) ;
#29012=( BOUNDED_CURVE ( )  B_SPLINE_CURVE ( 2, ( #51206, #39942, #10614, #45214, #17734, #11354, #496 ),
 .UNSPECIFIED., .F., .F. ) 
 B_SPLINE_CURVE_WITH_KNOTS ( ( 3, 2, 2, 3 ),
 ( 0.02083333333333322115, 0.02777777777777762705, 0.03472222222222204335, 0.04166666666666644231 ),
 .UNSPECIFIED. ) 
 CURVE ( )  GEOMETRIC_REPRESENTATION_ITEM ( )  RATIONAL_B_SPLINE_CURVE ( ( 1.000000000000002220, 0.8660254037844365982, 1.000000000000000000, 0.8660254037844387076, 1.000000000000000000, 0.8660254037844430375, 0.9999999999999956701 ) ) 
 REPRESENTATION_ITEM ( '' )  );
#29013=CARTESIAN_POINT ( 'NONE',  ( 97.30629616937498838, -211.3315407142195852, 88.00239583420047040 ) ) ;
#29022=VERTEX_POINT ( 'NONE', #15387 ) ;
#29023=VERTEX_POINT ( 'NONE', #60894 ) ;
#29028=( BOUNDED_CURVE ( )  B_SPLINE_CURVE ( 2, ( #50971, #5130, #62266, #33674, #38585, #10750, #17132 ),
 .UNSPECIFIED., .F., .F. ) 
 B_SPLINE_CURVE_WITH_KNOTS ( ( 3, 2, 2, 3 ),
 ( 0.4166666666666662966, 0.4236111111111106609, 0.4305555555555550806, 0.4374999999999994449 ),
 .UNSPECIFIED. ) 
 CURVE ( )  GEOMETRIC_REPRESENTATION_ITEM ( )  RATIONAL_B_SPLINE_CURVE ( ( 1.000000000000007550, 0.8660254037844311581, 1.000000000000000000, 0.8660254037844387076, 1.000000000000000000, 0.8660254037844493658, 0.9999999999999893419 ) ) 
 REPRESENTATION_ITEM ( '' )  );
#29029=CARTESIAN_POINT ( 'NONE',  ( 92.98340954502093325, 88.39448418669219620, 74.95309847082319266 ) ) ;
#29032=EDGE_LOOP ( 'NONE', ( #50297, #39873, #13935, #26069 ) ) ;
#29035=CARTESIAN_POINT ( 'NONE',  ( 93.84685191531248449, 88.00268892867053694, 85.30364583420046642 ) ) ;
#29037=ORIENTED_EDGE ( 'NONE', *, *, #27903, .T. ) ;
#29038=CARTESIAN_POINT ( 'NONE',  ( 92.69370383062501162, -211.3315407142195852, 81.44072916753381719 ) ) ;
#29042=CARTESIAN_POINT ( 'NONE',  ( -94.60587738269659042, -212.6434372237803530, 75.00000000000001421 ) ) ;
#29047=CARTESIAN_POINT ( 'NONE',  ( -92.69370383062498320, -209.9999999999999716, 85.51531250086713953 ) ) ;
#29048=CARTESIAN_POINT ( 'NONE',  ( -96.15314808468751551, 88.00268892867056536, 82.92239583420048632 ) ) ;
#29052=CARTESIAN_POINT ( 'NONE',  ( 97.30629616937498838, 91.33154071421968467, 84.93322916753379559 ) ) ;
#29053=CARTESIAN_POINT ( 'NONE',  ( -97.30629616937501680, 88.66845928578038638, 85.25072916753379104 ) ) ;
#29056=CARTESIAN_POINT ( 'NONE',  ( -93.67500000000003979, 92.29496732002878900, 87.88333333333332575 ) ) ;
#29060=CARTESIAN_POINT ( 'NONE',  ( -94.99999999999997158, -212.6630814284392557, 87.89656250086713385 ) ) ;
#29063=DIRECTION ( 'NONE',  ( -0.000000000000000000, -0.000000000000000000, 1.000000000000000000 ) ) ;
#29068=CARTESIAN_POINT ( 'NONE',  ( -95.00000000000002842, 86.94004357329504273, 76.82374999999998977 ) ) ;
#29069=CARTESIAN_POINT ( 'NONE',  ( 92.35000000000012221, -211.5299782133525071, 88.78291666666667936 ) ) ;
#29070=CYLINDRICAL_SURFACE ( 'NONE', #1034, 2.649999999999985700 ) ;
#29075=CARTESIAN_POINT ( 'NONE',  ( -97.30629616937501680, 90.00000000000004263, 78.84781250086714977 ) ) ;
#29080=CARTESIAN_POINT ( 'NONE',  ( -97.30629616937497417, -208.6684592857803011, 85.93864583420048575 ) ) ;
#29081=CARTESIAN_POINT ( 'NONE',  ( 93.84685191531248449, 88.00268892867053694, 75.93739583420048689 ) ) ;
#29083=CARTESIAN_POINT ( 'NONE',  ( -96.15314808468747287, -208.0026889286704943, 81.44072916753381719 ) ) ;
#29084=CARTESIAN_POINT ( 'NONE',  ( -96.32500000000001705, 92.29496732002878900, 84.89354166840095672 ) ) ;
#29087=CARTESIAN_POINT ( 'NONE',  ( -94.46769236096045574, -213.2667778271279246, 74.92222617501695936 ) ) ;
#29088=CARTESIAN_POINT ( 'NONE',  ( 93.67500000000001137, -212.2949673200287179, 78.75520833506763552 ) ) ;
#29094=CARTESIAN_POINT ( 'NONE',  ( 97.30629616937498838, -208.6684592857803011, 77.31322916753380525 ) ) ;
#29102=ORIENTED_EDGE ( 'NONE', *, *, #7744, .T. ) ;
#29111=ORIENTED_EDGE ( 'NONE', *, *, #37171, .F. ) ;
#29113=CARTESIAN_POINT ( 'NONE',  ( 94.99999999999998579, 87.33691857156068750, 84.24531250086715772 ) ) ;
#29117=ORIENTED_EDGE ( 'NONE', *, *, #13728, .F. ) ;
#29124=CARTESIAN_POINT ( 'NONE',  ( -92.35000000000003695, 90.00000000000004263, 87.77749999999998920 ) ) ;
#29127=CARTESIAN_POINT ( 'NONE',  ( 93.67500000000001137, -212.2949673200287179, 82.56520833506762358 ) ) ;
#29129=CARTESIAN_POINT ( 'NONE',  ( 94.99999999999998579, 90.00000000000002842, 90.00000000000000000 ) ) ;
#29131=CARTESIAN_POINT ( 'NONE',  ( -92.34999999999999432, -208.4700217866474645, 79.65479166840096070 ) ) ;
#29135=VERTEX_POINT ( 'NONE', #29256 ) ;
#29136=CARTESIAN_POINT ( 'NONE',  ( 97.64999999999997726, 91.52997821335252127, 79.65479166840096070 ) ) ;
#29137=CARTESIAN_POINT ( 'NONE',  ( -96.32500000000001705, 87.70503267997129626, 79.39020833506762642 ) ) ;
#29139=CARTESIAN_POINT ( 'NONE',  ( 92.69370383062498320, 91.33154071421968467, 80.85864583420048746 ) ) ;
#29141=CARTESIAN_POINT ( 'NONE',  ( -92.35000000000005116, 91.52997821335253548, 86.63979166840096013 ) ) ;
#29151=( BOUNDED_CURVE ( )  B_SPLINE_CURVE ( 2, ( #4978, #45938, #10218, #15488, #32767, #67742, #55715 ),
 .UNSPECIFIED., .F., .F. ) 
 B_SPLINE_CURVE_WITH_KNOTS ( ( 3, 2, 2, 3 ),
 ( 0.000000000000000000, 0.006944444444444406762, 0.01388888888888881352, 0.02083333333333322115 ),
 .UNSPECIFIED. ) 
 CURVE ( )  GEOMETRIC_REPRESENTATION_ITEM ( )  RATIONAL_B_SPLINE_CURVE ( ( 1.000000000000000000, 0.8660254037844387076, 1.000000000000000000, 0.8660254037844387076, 1.000000000000000000, 0.8660254037844408170, 0.9999999999999978906 ) ) 
 REPRESENTATION_ITEM ( '' )  );
#29153=CARTESIAN_POINT ( 'NONE',  ( 94.99999999999998579, 90.00000000000002842, 90.00000000000000000 ) ) ;
#29156=CARTESIAN_POINT ( 'NONE',  ( -93.84685191531248449, -208.0026889286704943, 76.25489583420049655 ) ) ;
#29157=ORIENTED_EDGE ( 'NONE', *, *, #48863, .T. ) ;
#29161=DIRECTION ( 'NONE',  ( 0.000000000000000000, 0.000000000000000000, 1.000000000000000000 ) ) ;
#29162=CARTESIAN_POINT ( 'NONE',  ( 97.30629616937498838, 88.66845928578035796, 75.30239583420048177 ) ) ;
#29169=CARTESIAN_POINT ( 'NONE',  ( 97.30629616937498838, 90.00000000000002842, 85.67406250086715147 ) ) ;
#29171=CARTESIAN_POINT ( 'NONE',  ( -97.65000000000001990, 90.00000000000004263, 90.00000000000000000 ) ) ;
#29174=CARTESIAN_POINT ( 'NONE',  ( -97.30629616937501680, 90.00000000000004263, 80.11781250086713158 ) ) ;
#29175=EDGE_CURVE ( 'NONE', #2120, #1262, #28362, .T. ) ;
#29178=CARTESIAN_POINT ( 'NONE',  ( 93.84685191531249870, -208.0026889286704943, 86.36197916753381776 ) ) ;
#29182=CARTESIAN_POINT ( 'NONE',  ( 97.64999999999997726, -208.4700217866474929, 87.19541666666667368 ) ) ;
#29189=EDGE_CURVE ( 'NONE', #53667, #6723, #64391, .T. ) ;
#29190=CARTESIAN_POINT ( 'NONE',  ( 97.30629616937498838, -209.9999999999999716, 83.13406250086715943 ) ) ;
#29192=DIRECTION ( 'NONE',  ( -0.000000000000000000, -0.000000000000000000, 1.000000000000000000 ) ) ;
#29195=CARTESIAN_POINT ( 'NONE',  ( 96.32499999999997442, 92.29496732002878900, 83.51770833506763836 ) ) ;
#29198=CARTESIAN_POINT ( 'NONE',  ( 97.64999999999997726, -208.4700217866474645, 84.65541666666666742 ) ) ;
#29210=CARTESIAN_POINT ( 'NONE',  ( -92.69370383062502583, 88.66845928578038638, 88.16114583420048234 ) ) ;
#29213=CARTESIAN_POINT ( 'NONE',  ( 92.35000000000002274, -211.5299782133524502, 76.16229166840095388 ) ) ;
#29214=CARTESIAN_POINT ( 'NONE',  ( 92.34999999999999432, 90.00000000000002842, 79.20499999999999829 ) ) ;
#29220=CARTESIAN_POINT ( 'NONE',  ( -100.0000000000000142, 85.00000000000002842, 90.00000000000000000 ) ) ;
#29221=CARTESIAN_POINT ( 'NONE',  ( -92.69370383062504004, 90.00000000000004263, 81.22906250086715829 ) ) ;
#29222=CARTESIAN_POINT ( 'NONE',  ( 93.84685191531248449, 91.99731107132950569, 89.06072916753382174 ) ) ;
#29230=CARTESIAN_POINT ( 'NONE',  ( -94.99999999999997158, -212.6630814284392557, 77.10156250086711793 ) ) ;
#29238=( BOUNDED_CURVE ( )  B_SPLINE_CURVE ( 2, ( #23214, #34853, #12649, #63810, #45788, #11909, #34475, #17928, #41233 ),
 .UNSPECIFIED., .F., .F. ) 
 B_SPLINE_CURVE_WITH_KNOTS ( ( 3, 2, 2, 2, 3 ),
 ( 0.8043570860693807223, 0.8043572716645402965, 0.8114130372054574325, 0.8184688027463743465, 0.8255245790604923695 ),
 .UNSPECIFIED. ) 
 CURVE ( )  GEOMETRIC_REPRESENTATION_ITEM ( )  RATIONAL_B_SPLINE_CURVE ( ( 0.9999929520383388226, 0.9999964759264720060, 1.000000000000000000, 0.8660254037844387076, 1.000000000000000000, 0.8660254037844387076, 1.000000000000000000, 0.8660254037844387076, 1.000000000000000000 ) ) 
 REPRESENTATION_ITEM ( '' )  );
#29239=CARTESIAN_POINT ( 'NONE',  ( -92.69370383062498320, -211.3315407142195852, 88.16114583420048234 ) ) ;
#29243=ORIENTED_EDGE ( 'NONE', *, *, #6046, .T. ) ;
#29244=CIRCLE ( 'NONE', #50880, 3.299999999999983391 ) ;
#29250=CARTESIAN_POINT ( 'NONE',  ( 96.15314808468748708, 91.99731107132950569, 84.35114583420048007 ) ) ;
#29252=DIRECTION ( 'NONE',  ( -0.000000000000000000, -0.000000000000000000, 1.000000000000000000 ) ) ;
#29256=CARTESIAN_POINT ( 'NONE',  ( -97.64999999953586496, -210.0000309672219601, 77.38038495123339544 ) ) ;
#29262=EDGE_CURVE ( 'NONE', #23771, #16386, #57567, .T. ) ;
#29265=LINE ( 'NONE', #56758, #68993 ) ;
#29268=EDGE_CURVE ( 'NONE', #6402, #47366, #31109, .T. ) ;
#29277=CARTESIAN_POINT ( 'NONE',  ( -92.35000000000005116, 88.47002178664754979, 77.64395833506762301 ) ) ;
#29279=CARTESIAN_POINT ( 'NONE',  ( 92.69370383062501162, -211.3315407142195852, 84.13947916753383538 ) ) ;
#29287=CARTESIAN_POINT ( 'NONE',  ( -97.64999999999996305, -209.9999999999999716, 90.00000000000000000 ) ) ;
#29288=ORIENTED_EDGE ( 'NONE', *, *, #69046, .T. ) ;
#29289=CARTESIAN_POINT ( 'NONE',  ( 96.15314808468748708, -208.0026889286704943, 78.79489583420048859 ) ) ;
#29290=ORIENTED_EDGE ( 'NONE', *, *, #4280, .T. ) ;
#29294=CARTESIAN_POINT ( 'NONE',  ( 97.64999999999999147, -210.0000001051138270, 86.58687499784845443 ) ) ;
#29298=CARTESIAN_POINT ( 'NONE',  ( 92.35000000000002274, -208.4700217866474645, 85.58145833506763722 ) ) ;
#29302=ORIENTED_EDGE ( 'NONE', *, *, #6945, .F. ) ;
#29306=CARTESIAN_POINT ( 'NONE',  ( 92.34999999999999432, 90.00000000000002842, 84.99937500173429328 ) ) ;
#29310=ORIENTED_EDGE ( 'NONE', *, *, #3733, .T. ) ;
#29312=AXIS2_PLACEMENT_3D ( 'NONE', #23106, #40021, #34366 ) ;
#29317=ORIENTED_EDGE ( 'NONE', *, *, #11640, .F. ) ;
#29320=CARTESIAN_POINT ( 'NONE',  ( -93.67500000000003979, 92.29496732002878900, 87.24833333333333485 ) ) ;
#29322=CARTESIAN_POINT ( 'NONE',  ( 95.00000000000000000, -206.9400435732949575, 89.84125000000000227 ) ) ;
#29326=CARTESIAN_POINT ( 'NONE',  ( -97.30629616937497417, -208.6684592857803011, 87.04989583420048405 ) ) ;
#29328=CARTESIAN_POINT ( 'NONE',  ( -97.64999999999996305, -209.9999999999999716, 79.28437500173430408 ) ) ;
#29329=CARTESIAN_POINT ( 'NONE',  ( 93.46017751755566394, -212.0954260604421222, 74.96680960279266515 ) ) ;
#29330=CARTESIAN_POINT ( 'NONE',  ( 94.99999999999998579, 86.94004357329502852, 81.26874999999999716 ) ) ;
#29331=CARTESIAN_POINT ( 'NONE',  ( -97.30629616937495996, -209.9999999999999716, 75.67281250086713840 ) ) ;
#29342=CARTESIAN_POINT ( 'NONE',  ( -95.00000000000002842, 92.66308142843932671, 78.68906250086713783 ) ) ;
#29343=DIRECTION ( 'NONE',  ( -1.000000000000000000, 3.061616997868382648E-16, 0.000000000000000000 ) ) ;
#29355=CARTESIAN_POINT ( 'NONE',  ( -93.84685191531247028, -211.9973110713294489, 76.04322916753382344 ) ) ;
#29373=CARTESIAN_POINT ( 'NONE',  ( 97.30629616937498838, -211.3315407142195852, 84.19239583420048234 ) ) ;
#29378=DIRECTION ( 'NONE',  ( 0.000000000000000000, 0.000000000000000000, 1.000000000000000000 ) ) ;
#29381=VERTEX_POINT ( 'NONE', #30733 ) ;
#29382=CARTESIAN_POINT ( 'NONE',  ( -92.69370383062504004, 90.00000000000004263, 79.32406250086715715 ) ) ;
#29384=EDGE_LOOP ( 'NONE', ( #16358, #38125, #31142, #6491 ) ) ;
#29385=VERTEX_POINT ( 'NONE', #53678 ) ;
#29386=DIRECTION ( 'NONE',  ( -1.000000000000000000, 0.000000000000000000, 0.000000000000000000 ) ) ;
#29390=CARTESIAN_POINT ( 'NONE',  ( 95.04693102382854875, 87.35041560265749183, 75.00000002508419072 ) ) ;
#29394=CARTESIAN_POINT ( 'NONE',  ( 97.30629616937498838, -209.9999999999999716, 81.70531250086713726 ) ) ;
#29402=CARTESIAN_POINT ( 'NONE',  ( -93.84685191531247028, -211.9973110713294489, 86.04447916753380809 ) ) ;
#29403=CARTESIAN_POINT ( 'NONE',  ( -97.30629616937501680, 91.33154071421968467, 83.39864583420050792 ) ) ;
#29405=CARTESIAN_POINT ( 'NONE',  ( 92.69370383062498320, 91.33154071421968467, 85.77989583420048803 ) ) ;
#29407=CARTESIAN_POINT ( 'NONE',  ( -92.35000000000003695, 90.00002660292287260, 78.96687592183759818 ) ) ;
#29409=CARTESIAN_POINT ( 'NONE',  ( -97.30629616937501680, 90.00000000000004263, 89.64281250086713726 ) ) ;
#29411=CARTESIAN_POINT ( 'NONE',  ( 92.35000000000000853, -209.9999999999999716, 85.55499999999999261 ) ) ;
#29412=CARTESIAN_POINT ( 'NONE',  ( -92.69370383062498320, -209.9999999999999716, 86.15031250086714465 ) ) ;
#29418=CARTESIAN_POINT ( 'NONE',  ( -97.65000000000001990, 90.00000000000004263, 77.29999999999999716 ) ) ;
#29423=CARTESIAN_POINT ( 'NONE',  ( -95.00000000000002842, 86.94004357329504273, 78.09374999999998579 ) ) ;
#29426=CARTESIAN_POINT ( 'NONE',  ( -97.30629616937501680, 88.66845928578038638, 87.15572916753380639 ) ) ;
#29429=CARTESIAN_POINT ( 'NONE',  ( 95.00000000000000000, -206.9400435732949575, 77.85562500173431033 ) ) ;
#29432=CARTESIAN_POINT ( 'NONE',  ( -96.15314808468752972, 91.99731107132950569, 79.37697916753380412 ) ) ;
#29433=VECTOR ( 'NONE', #72042, 1000.000000000000000 ) ;
#29441=CARTESIAN_POINT ( 'NONE',  ( -93.84685191531247028, -211.9973110713294489, 84.93322916753382401 ) ) ;
#29442=CARTESIAN_POINT ( 'NONE',  ( 93.67500000000001137, -207.7050326799711968, 79.17854166840096752 ) ) ;
#29443=( BOUNDED_CURVE ( )  B_SPLINE_CURVE ( 2, ( #49592, #25926, #3766, #72881, #61266, #55244, #21383 ),
 .UNSPECIFIED., .F., .F. ) 
 B_SPLINE_CURVE_WITH_KNOTS ( ( 3, 2, 2, 3 ),
 ( 0.1874999999999999167, 0.1944444444444443365, 0.2013888888888887285, 0.2083333333333331483 ),
 .UNSPECIFIED. ) 
 CURVE ( )  GEOMETRIC_REPRESENTATION_ITEM ( )  RATIONAL_B_SPLINE_CURVE ( ( 1.000000000000001554, 0.8660254037844371533, 1.000000000000000000, 0.8660254037844387076, 1.000000000000000000, 0.8660254037844424824, 0.9999999999999962252 ) ) 
 REPRESENTATION_ITEM ( '' )  );
#29444=EDGE_CURVE ( 'NONE', #41704, #18817, #46164, .T. ) ;
#29445=CARTESIAN_POINT ( 'NONE',  ( 97.30629616937498838, 91.33154071421968467, 77.47197916753381719 ) ) ;
#29446=CARTESIAN_POINT ( 'NONE',  ( -96.15314808468745866, -211.9973110713294489, 75.93739583420048689 ) ) ;
#29451=DIRECTION ( 'NONE',  ( -0.000000000000000000, -0.000000000000000000, 1.000000000000000000 ) ) ;
#29454=CARTESIAN_POINT ( 'NONE',  ( 92.69370383062501162, -211.3315407142195852, 75.72572916753381378 ) ) ;
#29467=ORIENTED_EDGE ( 'NONE', *, *, #28366, .F. ) ;
#29469=ORIENTED_EDGE ( 'NONE', *, *, #3733, .F. ) ;
#29475=CARTESIAN_POINT ( 'NONE',  ( 97.30629616937498838, 91.33154071421968467, 83.18697916753382060 ) ) ;
#29477=CARTESIAN_POINT ( 'NONE',  ( 97.64999999999999147, -209.9999999999999716, 75.07749999999998636 ) ) ;
#29479=EDGE_LOOP ( 'NONE', ( #11342, #61871, #41604, #13064 ) ) ;
#29481=B_SPLINE_CURVE_WITH_KNOTS ( 'NONE', 3,
 ( #9984, #28014, #63010, #61878 ),
 .UNSPECIFIED., .F., .F.,
 ( 4, 4 ),
 ( 2.446487931514586224E-06, 1.000000000000000000 ),
 .UNSPECIFIED. ) ;
#29487=CARTESIAN_POINT ( 'NONE',  ( 94.99999999999998579, 93.05995642670504253, 84.12624999999999886 ) ) ;
#29494=CARTESIAN_POINT ( 'NONE',  ( -94.99999999999997158, -213.0599564267049857, 78.17312500173430578 ) ) ;
#29499=CARTESIAN_POINT ( 'NONE',  ( 92.34999999999999432, 88.47002178664753558, 78.06729166840096923 ) ) ;
#29500=CARTESIAN_POINT ( 'NONE',  ( -93.67500000000003979, 87.70503267997129626, 78.86104166840097207 ) ) ;
#29502=CARTESIAN_POINT ( 'NONE',  ( 93.84685191531248449, 88.00268892867053694, 78.47739583420049314 ) ) ;
#29503=DIRECTION ( 'NONE',  ( 0.000000000000000000, -0.000000000000000000, -1.000000000000000000 ) ) ;
#29510=CARTESIAN_POINT ( 'NONE',  ( -94.99999999999997158, -209.9999999999999716, 90.00000000000000000 ) ) ;
#29516=LINE ( 'NONE', #58855, #15031 ) ;
#29518=CARTESIAN_POINT ( 'NONE',  ( -97.30629616937497417, -211.3315407142195852, 77.78947916753381264 ) ) ;
#29530=DIRECTION ( 'NONE',  ( 1.000000000000000000, 0.000000000000000000, 0.000000000000000000 ) ) ;
#29531=DIRECTION ( 'NONE',  ( -0.000000000000000000, -0.000000000000000000, -1.000000000000000000 ) ) ;
#29532=LINE ( 'NONE', #34444, #422 ) ;
#29535=EDGE_CURVE ( 'NONE', #25802, #31031, #36043, .T. ) ;
#29538=CARTESIAN_POINT ( 'NONE',  ( 94.99999999999998579, 92.66308142843932671, 87.73781250086715033 ) ) ;
#29539=CARTESIAN_POINT ( 'NONE',  ( -97.30629616937497417, -208.6684592857803295, 87.84364583420048689 ) ) ;
#29540=LINE ( 'NONE', #65261, #250 ) ;
#29543=CARTESIAN_POINT ( 'NONE',  ( -92.69370383062504004, 90.00000000000004263, 76.62531250086713897 ) ) ;
#29546=CARTESIAN_POINT ( 'NONE',  ( 95.00000000000000000, -207.3369185715606307, 87.57906250086713840 ) ) ;
#29550=VERTEX_POINT ( 'NONE', #11878 ) ;
#29552=CARTESIAN_POINT ( 'NONE',  ( 92.35000000000000853, -209.9999999999999716, 75.39499999999999602 ) ) ;
#29556=CARTESIAN_POINT ( 'NONE',  ( 93.84685191531249870, -208.0026889286704943, 81.44072916753381719 ) ) ;
#29557=DIRECTION ( 'NONE',  ( -0.000000000000000000, -0.000000000000000000, 1.000000000000000000 ) ) ;
#29562=CARTESIAN_POINT ( 'NONE',  ( 93.67500000000001137, -207.7050326799711968, 83.54416666666666913 ) ) ;
#29563=ORIENTED_EDGE ( 'NONE', *, *, #24363, .T. ) ;
#29565=EDGE_LOOP ( 'NONE', ( #58349, #49545, #22940, #66069 ) ) ;
#29568=CARTESIAN_POINT ( 'NONE',  ( -95.00000000000002842, 87.33691857156074434, 87.42031250086715488 ) ) ;
#29570=AXIS2_PLACEMENT_3D ( 'NONE', #10362, #11472, #33281 ) ;
#29571=CARTESIAN_POINT ( 'NONE',  ( 92.35000000000000853, -209.9999999999999716, 90.00000000000000000 ) ) ;
#29572=CARTESIAN_POINT ( 'NONE',  ( 92.35000000000002274, -211.5299782133524502, 76.79729166840095900 ) ) ;
#29573=CARTESIAN_POINT ( 'NONE',  ( 94.99999999999998579, 86.94004357329500010, 76.82374999999998977 ) ) ;
#29575=CARTESIAN_POINT ( 'NONE',  ( -97.64999999999994884, -211.5299782133524502, 88.86229166840097093 ) ) ;
#29579=CARTESIAN_POINT ( 'NONE',  ( -92.35000000000005116, 91.52997821335253548, 89.17979166840096639 ) ) ;
#29580=CARTESIAN_POINT ( 'NONE',  ( -95.00000000000002842, 92.66308142843932671, 80.75281250086716511 ) ) ;
#29581=CARTESIAN_POINT ( 'NONE',  ( 94.99999999999998579, 92.66308142843935514, 74.87906250086713555 ) ) ;
#29587=CARTESIAN_POINT ( 'NONE',  ( -96.32499999999996021, -207.7050326799711968, 86.16354166840096696 ) ) ;
#29602=CARTESIAN_POINT ( 'NONE',  ( -97.30629616937497417, -208.6684592857803011, 89.11364583420049712 ) ) ;
#29611=EDGE_CURVE ( 'NONE', #47064, #42482, #69045, .T. ) ;
#29612=CARTESIAN_POINT ( 'NONE',  ( 92.69370383062498320, 91.33154071421968467, 80.69989583420046131 ) ) ;
#29626=CARTESIAN_POINT ( 'NONE',  ( -95.00000000000002842, 92.66308142843932671, 85.67406250086715147 ) ) ;
#29635=CARTESIAN_POINT ( 'NONE',  ( 92.35001469846380928, -208.4700133004854194, 76.05645774805350356 ) ) ;
#29640=CARTESIAN_POINT ( 'NONE',  ( 97.30629616937498838, -208.6684592857803011, 80.64697916753382856 ) ) ;
#29642=VERTEX_POINT ( 'NONE', #23543 ) ;
#29648=CARTESIAN_POINT ( 'NONE',  ( 96.15314808468750130, -211.9973110713294489, 75.24947916753380639 ) ) ;
#29650=CARTESIAN_POINT ( 'NONE',  ( 92.69370383062501162, -208.6684592857803011, 78.31864583420050963 ) ) ;
#29652=CARTESIAN_POINT ( 'NONE',  ( -92.34999999999999432, -209.9999999999999716, 88.41249999999999432 ) ) ;
#29659=CARTESIAN_POINT ( 'NONE',  ( 97.64999999999999147, -209.9999999999999716, 87.22187500173430408 ) ) ;
#29660=CARTESIAN_POINT ( 'NONE',  ( 94.99999999999998579, 93.05995642670504253, 88.57124999999999204 ) ) ;
#29664=ORIENTED_EDGE ( 'NONE', *, *, #42022, .T. ) ;
#29665=( BOUNDED_CURVE ( )  B_SPLINE_CURVE ( 2, ( #28002, #44576, #73493, #20883, #16741, #61862, #10347 ),
 .UNSPECIFIED., .F., .F. ) 
 B_SPLINE_CURVE_WITH_KNOTS ( ( 3, 2, 2, 3 ),
 ( 0.3958333333333330373, 0.4027777777777774570, 0.4097222222222218768, 0.4166666666666662966 ),
 .UNSPECIFIED. ) 
 CURVE ( )  GEOMETRIC_REPRESENTATION_ITEM ( )  RATIONAL_B_SPLINE_CURVE ( ( 1.000000000000005329, 0.8660254037844333785, 1.000000000000000000, 0.8660254037844387076, 1.000000000000000000, 0.8660254037844462571, 0.9999999999999924505 ) ) 
 REPRESENTATION_ITEM ( '' )  );
#29670=CARTESIAN_POINT ( 'NONE',  ( 94.99999999999998579, 86.94004357329500010, 87.06312500173430635 ) ) ;
#29685=CARTESIAN_POINT ( 'NONE',  ( -97.65000000000001990, 91.52997821335253548, 87.40708333333333258 ) ) ;
#29687=CARTESIAN_POINT ( 'NONE',  ( 97.65000000000000568, 88.47002178664753558, 82.00958333333333883 ) ) ;
#29690=CARTESIAN_POINT ( 'NONE',  ( 92.34999999999999432, 90.00000000000002842, 75.39499999999999602 ) ) ;
#29691=CARTESIAN_POINT ( 'NONE',  ( -96.15314808468745866, -211.9973110713294489, 81.49364583420047836 ) ) ;
#29695=CARTESIAN_POINT ( 'NONE',  ( 95.04693102382874770, -212.6495843973424940, 75.00000002508419072 ) ) ;
#29697=CARTESIAN_POINT ( 'NONE',  ( -93.84685191531248449, -208.0026889286704943, 77.36614583420046642 ) ) ;
#29707=CARTESIAN_POINT ( 'NONE',  ( -92.69370383062502583, 88.66845928578038638, 77.20739583420046870 ) ) ;
#29710=ORIENTED_EDGE ( 'NONE', *, *, #23177, .T. ) ;
#29711=LINE ( 'NONE', #7543, #48426 ) ;
#29715=EDGE_CURVE ( 'NONE', #66290, #27169, #70129, .T. ) ;
#29716=CYLINDRICAL_SURFACE ( 'NONE', #1131, 2.649999999999985700 ) ;
#29719=CARTESIAN_POINT ( 'NONE',  ( -93.84685191531248449, -208.0026889286704943, 75.61989583420049144 ) ) ;
#29724=CARTESIAN_POINT ( 'NONE',  ( 92.35000000000000853, -209.9999999999999716, 88.09499999999999886 ) ) ;
#29727=CARTESIAN_POINT ( 'NONE',  ( 92.34999999999999432, 90.00000000000002842, 79.20499999999999829 ) ) ;
#29730=ORIENTED_EDGE ( 'NONE', *, *, #60700, .T. ) ;
#29734=CARTESIAN_POINT ( 'NONE',  ( 92.69370383062501162, -209.9999999999999716, 86.46781250086714010 ) ) ;
#29735=CARTESIAN_POINT ( 'NONE',  ( -97.64999999999994884, -210.0000359395364171, 83.72937624475883922 ) ) ;
#29737=CARTESIAN_POINT ( 'NONE',  ( 97.30629616937498838, -209.9999999999999716, 89.48406250086715374 ) ) ;
#29741=CARTESIAN_POINT ( 'NONE',  ( -97.30629616937501680, 90.00000000000004263, 79.64156250086715261 ) ) ;
#29751=CARTESIAN_POINT ( 'NONE',  ( 97.65000000000000568, -211.5299782133524218, 79.46958333333331836 ) ) ;
#29759=CARTESIAN_POINT ( 'NONE',  ( 93.32700159667687956, 88.01659165168841525, 74.96344747200082281 ) ) ;
#29761=EDGE_CURVE ( 'NONE', #42455, #34388, #12257, .T. ) ;
#29764=CARTESIAN_POINT ( 'NONE',  ( 96.15314808468748708, -208.0026889286704943, 82.44614583420046472 ) ) ;
#29773=CARTESIAN_POINT ( 'NONE',  ( -96.15314808468747287, -208.0026889286704943, 85.72697916753379843 ) ) ;
#29774=CARTESIAN_POINT ( 'NONE',  ( -92.69370383062502583, 91.33154071421968467, 81.28197916753381946 ) ) ;
#29776=CARTESIAN_POINT ( 'NONE',  ( 97.30629616937498838, 90.00000000000002842, 81.07031250086714635 ) ) ;
#29784=CARTESIAN_POINT ( 'NONE',  ( -92.34999999999999432, -209.9999999999999716, 90.00000000000000000 ) ) ;
#29785=CARTESIAN_POINT ( 'NONE',  ( -93.84685191531248449, -208.0026889286704943, 86.25614583420048120 ) ) ;
#29791=CARTESIAN_POINT ( 'NONE',  ( 97.65000000000000568, 91.52997821335250705, 80.21041666666666003 ) ) ;
#29795=AXIS2_PLACEMENT_3D ( 'NONE', #61930, #36851, #8282 ) ;
#29796=CARTESIAN_POINT ( 'NONE',  ( -97.65000000000001990, 91.52997821335253548, 77.88208333333332689 ) ) ;
#29797=EDGE_CURVE ( 'NONE', #4344, #11208, #69769, .T. ) ;
#29798=CARTESIAN_POINT ( 'NONE',  ( -92.34999999999999432, -209.9999999999999716, 78.88750000000000284 ) ) ;
#29800=CARTESIAN_POINT ( 'NONE',  ( -92.69370383062504004, 90.00000000000004263, 89.32531250086714181 ) ) ;
#29804=CARTESIAN_POINT ( 'NONE',  ( -96.32499999999996021, -207.7050326799711968, 78.46416666666667084 ) ) ;
#29806=CARTESIAN_POINT ( 'NONE',  ( -92.69370383062502583, 91.33154071421968467, 76.04322916753380923 ) ) ;
#29815=CARTESIAN_POINT ( 'NONE',  ( -96.15314808468747287, -208.0026889286704943, 84.61572916753381435 ) ) ;
#29816=AXIS2_PLACEMENT_3D ( 'NONE', #2445, #2064, #54997 ) ;
#29819=CARTESIAN_POINT ( 'NONE',  ( -92.69370383062498320, -208.6684592857803295, 77.47197916753381719 ) ) ;
#29820=DIRECTION ( 'NONE',  ( -0.000000000000000000, -0.000000000000000000, 1.000000000000000000 ) ) ;
#29824=DIRECTION ( 'NONE',  ( 1.000000000000000000, 0.000000000000000000, 0.000000000000000000 ) ) ;
#29825=CARTESIAN_POINT ( 'NONE',  ( -95.00000000000002842, 92.66308142843932671, 76.30781250086715772 ) ) ;
#29826=CARTESIAN_POINT ( 'NONE',  ( 92.69370383062501162, -211.3315407142195852, 76.99572916753380980 ) ) ;
#29827=ORIENTED_EDGE ( 'NONE', *, *, #11370, .F. ) ;
#29840=EDGE_CURVE ( 'NONE', #20056, #44202, #12620, .T. ) ;
#29846=CARTESIAN_POINT ( 'NONE',  ( 97.30629616937498838, 90.00000000000002842, 81.86406250086714920 ) ) ;
#29863=CARTESIAN_POINT ( 'NONE',  ( 95.00000000000000000, -213.0599564267049857, 87.06312500173429214 ) ) ;
#29868=CARTESIAN_POINT ( 'NONE',  ( -92.34999999999999432, -209.9999999999999716, 80.87187500173430976 ) ) ;
#29872=CARTESIAN_POINT ( 'NONE',  ( 94.99999999999998579, 93.05995642670504253, 79.12562500173429214 ) ) ;
#29873=CARTESIAN_POINT ( 'NONE',  ( -92.35000000000005116, 91.52997821335253548, 76.47979166840096354 ) ) ;
#29876=CARTESIAN_POINT ( 'NONE',  ( 92.69370383062498320, 90.00000000000002842, 79.64156250086715261 ) ) ;
#29877=EDGE_CURVE ( 'NONE', #37739, #7050, #64888, .T. ) ;
#29882=ORIENTED_EDGE ( 'NONE', *, *, #17232, .T. ) ;
#29891=( BOUNDED_CURVE ( )  B_SPLINE_CURVE ( 2, ( #1824, #64211, #70186, #58185, #19063, #42016, #64950 ),
 .UNSPECIFIED., .F., .F. ) 
 B_SPLINE_CURVE_WITH_KNOTS ( ( 3, 2, 2, 3 ),
 ( 0.5080151867253830389, 0.5150708844844118506, 0.5221266500252946807, 0.5291824299508929297 ),
 .UNSPECIFIED. ) 
 CURVE ( )  GEOMETRIC_REPRESENTATION_ITEM ( )  RATIONAL_B_SPLINE_CURVE ( ( 0.9999974259464162740, 0.8660266908235946248, 1.000000000000000000, 0.8660254037844387076, 1.000000000000000000, 0.8660254037844387076, 1.000000000000000000 ) ) 
 REPRESENTATION_ITEM ( '' )  );
#29892=CARTESIAN_POINT ( 'NONE',  ( -93.84685191531247028, -211.9973110713294489, 78.58322916753382970 ) ) ;
#29896=VECTOR ( 'NONE', #35729, 1000.000000000000000 ) ;
#29898=FACE_OUTER_BOUND ( 'NONE', #8817, .T. ) ;
#29909=CARTESIAN_POINT ( 'NONE',  ( 97.30629616937498838, 91.33154071421968467, 87.63197916753381378 ) ) ;
#29911=CARTESIAN_POINT ( 'NONE',  ( -93.84685191531247028, -211.9973110713294489, 87.47322916753381605 ) ) ;
#29915=CARTESIAN_POINT ( 'NONE',  ( 97.64999999999999147, -209.9999999999999716, 79.52249999999999375 ) ) ;
#29916=CARTESIAN_POINT ( 'NONE',  ( -97.64999999999994884, -208.4700217866474645, 81.05708333333333826 ) ) ;
#29917=CARTESIAN_POINT ( 'NONE',  ( -96.15314808468752972, 91.99731107132950569, 76.83697916753381207 ) ) ;
#29918=AXIS2_PLACEMENT_3D ( 'NONE', #26688, #49613, #66914 ) ;
#29921=CARTESIAN_POINT ( 'NONE',  ( 93.84685191531251292, -211.9973110713294489, 87.20864583420046756 ) ) ;
#29924=ORIENTED_EDGE ( 'NONE', *, *, #27975, .T. ) ;
#29928=LINE ( 'NONE', #1421, #31829 ) ;
#29929=ORIENTED_EDGE ( 'NONE', *, *, #9534, .T. ) ;
#29932=CARTESIAN_POINT ( 'NONE',  ( 92.69370383062501162, -208.6684592857803295, 80.22364583420048234 ) ) ;
#29934=FACE_OUTER_BOUND ( 'NONE', #55300, .T. ) ;
#29937=AXIS2_PLACEMENT_3D ( 'NONE', #20269, #43233, #14634 ) ;
#29940=CARTESIAN_POINT ( 'NONE',  ( 97.64999999999999147, -209.9999999999999716, 85.87249999999998806 ) ) ;
#29949=CARTESIAN_POINT ( 'NONE',  ( -95.00000000000002842, 92.66308142843932671, 88.37281250086715545 ) ) ;
#29953=CARTESIAN_POINT ( 'NONE',  ( 97.64999999999997726, -208.4700217866474645, 74.57479166840096241 ) ) ;
#29954=CARTESIAN_POINT ( 'NONE',  ( 94.99999999999998579, 93.05995642670504253, 77.77624999999999034 ) ) ;
#29958=CARTESIAN_POINT ( 'NONE',  ( 97.64999999999997726, -211.5299782133524218, 80.10458333333330927 ) ) ;
#29961=CARTESIAN_POINT ( 'NONE',  ( -96.32500000000001705, 92.29496732002878900, 87.43354166840096298 ) ) ;
#29962=CARTESIAN_POINT ( 'NONE',  ( 96.15314808468748708, 91.99731107132950569, 74.82614583420047438 ) ) ;
#29976=CARTESIAN_POINT ( 'NONE',  ( -92.69370383062498320, -211.3315407142195852, 75.30239583420048177 ) ) ;
#29985=ORIENTED_EDGE ( 'NONE', *, *, #67817, .T. ) ;
#29986=CARTESIAN_POINT ( 'NONE',  ( -94.99999999999997158, -212.6630814284392557, 87.42031250086715488 ) ) ;
#29989=VERTEX_POINT ( 'NONE', #8843 ) ;
#29990=CARTESIAN_POINT ( 'NONE',  ( -97.64999999950686060, 89.99996796133669363, 83.73041644179562581 ) ) ;
#29992=CARTESIAN_POINT ( 'NONE',  ( 94.99999999999998579, 92.66308142843932671, 82.49906250086715431 ) ) ;
#30003=CARTESIAN_POINT ( 'NONE',  ( -97.30629616937501680, 90.00000000000004263, 87.10281250086714522 ) ) ;
#30015=VECTOR ( 'NONE', #25112, 1000.000000000000000 ) ;
#30018=CARTESIAN_POINT ( 'NONE',  ( 96.15314808468750130, -211.9973110713294489, 83.66322916753382799 ) ) ;
#30029=CARTESIAN_POINT ( 'NONE',  ( 97.30629616937498838, -209.9999999999999716, 75.35531250086714294 ) ) ;
#30031=CARTESIAN_POINT ( 'NONE',  ( 93.84685191531249870, -208.0026889286704943, 78.90072916753382515 ) ) ;
#30040=CARTESIAN_POINT ( 'NONE',  ( -92.35000000000003695, 90.00000000000004263, 83.96750000000000114 ) ) ;
#30041=CARTESIAN_POINT ( 'NONE',  ( 92.35000000000002274, -208.4700217866474645, 83.67645833506762187 ) ) ;
#30042=CARTESIAN_POINT ( 'NONE',  ( 97.64999999999997726, 91.52997821335252127, 88.46541666666665549 ) ) ;
#30046=ORIENTED_EDGE ( 'NONE', *, *, #21888, .F. ) ;
#30050=CARTESIAN_POINT ( 'NONE',  ( 92.34999999999999432, 91.52997821335252127, 85.58145833506763722 ) ) ;
#30059=CARTESIAN_POINT ( 'NONE',  ( -97.64999999999986358, -208.4700217866474361, 75.34208333333333485 ) ) ;
#30060=ORIENTED_EDGE ( 'NONE', *, *, #4341, .F. ) ;
#30066=CARTESIAN_POINT ( 'NONE',  ( -95.00000000000002842, 86.94004357329504273, 88.88875000000000171 ) ) ;
#30067=VERTEX_POINT ( 'NONE', #68491 ) ;
#30073=CARTESIAN_POINT ( 'NONE',  ( -94.99999999999997158, -207.3369185715606307, 82.49906250086714010 ) ) ;
#30075=DIRECTION ( 'NONE',  ( -0.000000000000000000, -0.000000000000000000, 1.000000000000000000 ) ) ;
#30077=CARTESIAN_POINT ( 'NONE',  ( 94.99999999999998579, 93.05995642670504253, 89.28562500173430294 ) ) ;
#30089=CARTESIAN_POINT ( 'NONE',  ( -97.30629616937501680, 90.00000000000004263, 79.48281250086714067 ) ) ;
#30090=DIRECTION ( 'NONE',  ( -0.000000000000000000, -0.000000000000000000, 1.000000000000000000 ) ) ;
#30091=CARTESIAN_POINT ( 'NONE',  ( 97.65000000000004832, 88.47002178664756400, 76.29458333333333542 ) ) ;
#30097=FACE_OUTER_BOUND ( 'NONE', #22767, .T. ) ;
#30098=CARTESIAN_POINT ( 'NONE',  ( -97.30629616937497417, -208.6684592857803011, 76.41364583420049428 ) ) ;
#30111=LINE ( 'NONE', #53062, #53922 ) ;
#30114=( BOUNDED_CURVE ( )  B_SPLINE_CURVE ( 2, ( #74134, #29735, #62891, #11349, #492, #34284, #23024, #17732, #1238 ),
 .UNSPECIFIED., .F., .F. ) 
 B_SPLINE_CURVE_WITH_KNOTS ( ( 3, 2, 2, 2, 3 ),
 ( 0.3810111478283708664, 0.3810113392095190732, 0.3880671047504364868, 0.3951228702913539559, 0.4021785743347534581 ),
 .UNSPECIFIED. ) 
 CURVE ( )  GEOMETRIC_REPRESENTATION_ITEM ( )  RATIONAL_B_SPLINE_CURVE ( ( 0.9999927323218336106, 0.9999963660623495398, 1.000000000000000000, 0.8660254037844387076, 1.000000000000000000, 0.8660254037844387076, 1.000000000000000000, 0.8660265714968692352, 0.9999976645954944399 ) ) 
 REPRESENTATION_ITEM ( '' )  );
#30116=CARTESIAN_POINT ( 'NONE',  ( 96.15314808468748708, -208.0026889286704943, 84.98614583420047097 ) ) ;
#30117=CARTESIAN_POINT ( 'NONE',  ( 95.00000000000000000, -207.3369185715606307, 87.10281250086715943 ) ) ;
#30121=EDGE_LOOP ( 'NONE', ( #63827, #65854, #40532, #61137, #55371, #50030, #66847, #34007, #38159, #16953, #11820, #22360, #30318, #37575, #6055, #22840, #16562, #47614, #24345, #73061, #69295, #69612, #74129, #13432, #62897, #1, #9483, #62988, #13863, #8330, #64958, #11145, #18377, #4639, #8167, #7588, #44680, #47587, #10340, #18396, #57985, #7526, #44584, #10477, #33448, #37680, #62443, #62577, #16834, #48006, #38924, #7718 ) ) ;
#30123=VERTEX_POINT ( 'NONE', #41388 ) ;
#30125=CARTESIAN_POINT ( 'NONE',  ( -92.69370383062502583, 91.33154071421968467, 81.28197916753381946 ) ) ;
#30133=FACE_OUTER_BOUND ( 'NONE', #6848, .T. ) ;
#30141=ORIENTED_EDGE ( 'NONE', *, *, #40392, .T. ) ;
#30143=CARTESIAN_POINT ( 'NONE',  ( 97.30629616937498838, -211.3315407142195852, 81.65239583420049030 ) ) ;
#30148=CARTESIAN_POINT ( 'NONE',  ( -93.67499999999998295, -212.2949673200287179, 85.84604166840097150 ) ) ;
#30154=CARTESIAN_POINT ( 'NONE',  ( -94.99999999999997158, -207.3369185715606307, 83.76906250086713612 ) ) ;
#30155=CARTESIAN_POINT ( 'NONE',  ( -96.15314808468752972, 91.99731107132950569, 83.98072916753382344 ) ) ;
#30157=CARTESIAN_POINT ( 'NONE',  ( 93.84685191531248449, 88.00268892867053694, 82.12864583420046927 ) ) ;
#30164=CARTESIAN_POINT ( 'NONE',  ( -93.84685191531247028, -211.9973110713294489, 86.67947916753381321 ) ) ;
#30171=LINE ( 'NONE', #69663, #3660 ) ;
#30174=CARTESIAN_POINT ( 'NONE',  ( -93.67500000000003979, 92.29496732002878900, 75.18333333333332291 ) ) ;
#30177=CARTESIAN_POINT ( 'NONE',  ( -95.00000000000002842, 87.33691857156074434, 89.16656250086712987 ) ) ;
#30189=LINE ( 'NONE', #1307, #26100 ) ;
#30190=CARTESIAN_POINT ( 'NONE',  ( -92.35000000002592913, -210.0000117261698165, 82.77687459617060028 ) ) ;
#30191=CARTESIAN_POINT ( 'NONE',  ( -96.15314808468745866, -211.9973110713294489, 86.09739583420049769 ) ) ;
#30199=CARTESIAN_POINT ( 'NONE',  ( -92.69370383062498320, -211.3315407142195852, 75.46114583420049371 ) ) ;
#30200=CARTESIAN_POINT ( 'NONE',  ( 92.35000000000000853, -209.9999999999999716, 90.00000000000000000 ) ) ;
#30204=CARTESIAN_POINT ( 'NONE',  ( 97.65000000000000568, 91.52997821335252127, 85.36979166840096411 ) ) ;
#30207=CARTESIAN_POINT ( 'NONE',  ( 96.15314808468750130, -211.9973110713294489, 77.78947916753381264 ) ) ;
#30209=ADVANCED_FACE ( 'NONE', ( #41032 ), #29716, .F. ) ;
#30210=CYLINDRICAL_SURFACE ( 'NONE', #41995, 2.649999999999985700 ) ;
#30213=EDGE_CURVE ( 'NONE', #27925, #16429, #18447, .T. ) ;
#30222=CARTESIAN_POINT ( 'NONE',  ( -97.64999999999997726, -211.5299782133524502, 77.35291666666665833 ) ) ;
#30225=EDGE_CURVE ( 'NONE', #28278, #59392, #32478, .T. ) ;
#30229=CARTESIAN_POINT ( 'NONE',  ( 97.30629616937498838, 90.00000000000002842, 78.68906250086715204 ) ) ;
#30231=CARTESIAN_POINT ( 'NONE',  ( 92.35000000000002274, -211.5299782133524502, 76.08291666666666231 ) ) ;
#30240=CARTESIAN_POINT ( 'NONE',  ( -94.94576887096278028, 92.38875495131968307, 74.83591575723764322 ) ) ;
#30246=CARTESIAN_POINT ( 'NONE',  ( -94.99999999999997158, -213.0599564267049857, 79.44312500173428759 ) ) ;
#30249=CARTESIAN_POINT ( 'NONE',  ( 97.64999999999997726, 88.47002178664753558, 75.73895833506765030 ) ) ;
#30250=CARTESIAN_POINT ( 'NONE',  ( -92.35000000000005116, 88.47002178664754979, 77.00895833506763211 ) ) ;
#30252=CARTESIAN_POINT ( 'NONE',  ( 93.84685191531248449, 91.99731107132950569, 80.80572916753382628 ) ) ;
#30268=CARTESIAN_POINT ( 'NONE',  ( -96.15314808468745866, -211.9973110713294489, 77.20739583420048291 ) ) ;
#30282=EDGE_CURVE ( 'NONE', #16487, #24954, #58725, .T. ) ;
#30285=CARTESIAN_POINT ( 'NONE',  ( 92.69370383062498320, 88.66845928578035796, 83.50447916753383026 ) ) ;
#30287=CARTESIAN_POINT ( 'NONE',  ( -93.84685191531248449, -208.0026889286704943, 85.77989583420048803 ) ) ;
#30291=CARTESIAN_POINT ( 'NONE',  ( -93.67499999999998295, -207.7050326799711968, 80.89833333333332632 ) ) ;
#30292=CARTESIAN_POINT ( 'NONE',  ( -92.69370383062504004, 90.00000000000004263, 77.26031250086714408 ) ) ;
#30295=CARTESIAN_POINT ( 'NONE',  ( 95.00000000000000000, -212.6630814284392557, 87.26156250086714294 ) ) ;
#30296=ORIENTED_EDGE ( 'NONE', *, *, #70697, .T. ) ;
#30300=CARTESIAN_POINT ( 'NONE',  ( 97.65000000000009095, -211.5299782133523649, 75.65958333333333030 ) ) ;
#30305=CARTESIAN_POINT ( 'NONE',  ( 93.84685191531249870, -208.0026889286704943, 80.80572916753382628 ) ) ;
#30307=CARTESIAN_POINT ( 'NONE',  ( 92.35000000000000853, -209.9999999999999716, 76.03000000000000114 ) ) ;
#30308=EDGE_CURVE ( 'NONE', #36890, #32411, #51417, .T. ) ;
#30309=CARTESIAN_POINT ( 'NONE',  ( 90.00000000000000000, 85.00000000000002842, -80.00000000000000000 ) ) ;
#30314=CARTESIAN_POINT ( 'NONE',  ( 92.35000000000000853, -209.9999999999999716, 86.18999999999999773 ) ) ;
#30318=ORIENTED_EDGE ( 'NONE', *, *, #24969, .F. ) ;
#30319=ORIENTED_EDGE ( 'NONE', *, *, #4589, .T. ) ;
#30322=CARTESIAN_POINT ( 'NONE',  ( -93.84685191531254134, 91.99731107132950569, 87.04989583420048405 ) ) ;
#30325=CARTESIAN_POINT ( 'NONE',  ( 96.15314808468750130, -211.9973110713294489, 87.31447916753380412 ) ) ;
#30326=CARTESIAN_POINT ( 'NONE',  ( 97.64999999999997726, 91.52997821335252127, 77.03541666666666288 ) ) ;
#30328=CARTESIAN_POINT ( 'NONE',  ( -2.499999999999970690, 73.00000000000001421, -208.2999999999999261 ) ) ;
#30331=CARTESIAN_POINT ( 'NONE',  ( 97.64999999999999147, -209.9999999999999716, 80.15749999999999886 ) ) ;
#30333=CARTESIAN_POINT ( 'NONE',  ( -95.00000000000002842, 86.94004357329504273, 87.06312500173430635 ) ) ;
#30335=( BOUNDED_CURVE ( )  B_SPLINE_CURVE ( 2, ( #31318, #20033, #34842, #69783, #35202, #29182, #71532 ),
 .UNSPECIFIED., .F., .F. ) 
 B_SPLINE_CURVE_WITH_KNOTS ( ( 3, 2, 2, 3 ),
 ( 0.1666666666666666852, 0.1736111111111111049, 0.1805555555555554970, 0.1874999999999999167 ),
 .UNSPECIFIED. ) 
 CURVE ( )  GEOMETRIC_REPRESENTATION_ITEM ( )  RATIONAL_B_SPLINE_CURVE ( ( 0.9999999999999994449, 0.8660254037844392627, 1.000000000000000000, 0.8660254037844387076, 1.000000000000000000, 0.8660254037844402619, 0.9999999999999984457 ) ) 
 REPRESENTATION_ITEM ( '' )  );
#30336=CARTESIAN_POINT ( 'NONE',  ( 92.69370383062498320, 88.66845928578037217, 75.72572916753381378 ) ) ;
#30341=ORIENTED_EDGE ( 'NONE', *, *, #1137, .T. ) ;
#30348=CARTESIAN_POINT ( 'NONE',  ( 97.64999999999999147, -209.9999999999999716, 87.14249999999999829 ) ) ;
#30351=CARTESIAN_POINT ( 'NONE',  ( -96.15314808468747287, -208.0026889286704943, 88.42572916753381662 ) ) ;
#30360=CARTESIAN_POINT ( 'NONE',  ( 97.30629616937498838, 91.33154071421968467, 80.48822916753380241 ) ) ;
#30373=CARTESIAN_POINT ( 'NONE',  ( -97.30629616937501680, 88.66845928578038638, 85.88572916753381037 ) ) ;
#30383=EDGE_CURVE ( 'NONE', #63593, #5952, #55994, .T. ) ;
#30385=LINE ( 'NONE', #51853, #5574 ) ;
#30387=CARTESIAN_POINT ( 'NONE',  ( 95.00000000000000000, -212.6630814284392557, 83.61031250086716682 ) ) ;
#30389=EDGE_LOOP ( 'NONE', ( #48366, #50126, #5135, #45358 ) ) ;
#30394=CARTESIAN_POINT ( 'NONE',  ( 97.64999999999999147, -209.9999999999999716, 88.41249999999999432 ) ) ;
#30395=LINE ( 'NONE', #64262, #37588 ) ;
#30397=CARTESIAN_POINT ( 'NONE',  ( 97.30629616937498838, -208.6684592857803011, 81.28197916753381946 ) ) ;
#30398=ORIENTED_EDGE ( 'NONE', *, *, #13388, .T. ) ;
#30404=ORIENTED_EDGE ( 'NONE', *, *, #66780, .F. ) ;
#30406=CARTESIAN_POINT ( 'NONE',  ( 92.35000000000002274, -211.5299782133524502, 81.87729166840097150 ) ) ;
#30407=CARTESIAN_POINT ( 'NONE',  ( 93.67499999999998295, 92.29496732002878900, 87.98916666666666231 ) ) ;
#30414=CARTESIAN_POINT ( 'NONE',  ( -96.15314808468752972, 91.99731107132950569, 86.52072916753382970 ) ) ;
#30415=CARTESIAN_POINT ( 'NONE',  ( 93.84685191531248449, 88.00268892867053694, 86.57364583420047666 ) ) ;
#30417=CARTESIAN_POINT ( 'NONE',  ( 97.64999999999997726, 91.52997821335252127, 86.63979166840097434 ) ) ;
#30427=LINE ( 'NONE', #17684, #27722 ) ;
#30428=CARTESIAN_POINT ( 'NONE',  ( -92.35000000000003695, 90.00000000000004263, 85.23749999999999716 ) ) ;
#30429=ORIENTED_EDGE ( 'NONE', *, *, #45595, .F. ) ;
#30430=CARTESIAN_POINT ( 'NONE',  ( 96.32499999999998863, 87.70503267997126784, 81.95666666666666345 ) ) ;
#30435=CARTESIAN_POINT ( 'NONE',  ( -92.69370383062498320, -211.3315407142195852, 84.19239583420046813 ) ) ;
#30436=ORIENTED_EDGE ( 'NONE', *, *, #25029, .T. ) ;
#30437=DIRECTION ( 'NONE',  ( -1.000000000000000000, 3.061616997868382648E-16, 0.000000000000000000 ) ) ;
#30445=ADVANCED_FACE ( 'NONE', ( #49240 ), #72890, .F. ) ;
#30452=CARTESIAN_POINT ( 'NONE',  ( -95.00000000000002842, 87.33691857156074434, 76.46656250086712703 ) ) ;
#30453=CARTESIAN_POINT ( 'NONE',  ( 94.99999999999998579, 90.00000000000002842, 90.00000000000000000 ) ) ;
#30463=CARTESIAN_POINT ( 'NONE',  ( -94.99999999999997158, -207.3369185715606307, 77.57781250086715374 ) ) ;
#30464=FACE_OUTER_BOUND ( 'NONE', #32517, .T. ) ;
#30469=EDGE_CURVE ( 'NONE', #67440, #64530, #21396, .T. ) ;
#30470=CARTESIAN_POINT ( 'NONE',  ( 96.32499999999998863, -212.2949673200287179, 88.30666666666665776 ) ) ;
#30483=CARTESIAN_POINT ( 'NONE',  ( 97.30629616937498838, -208.6684592857803295, 84.93322916753379559 ) ) ;
#30484=CARTESIAN_POINT ( 'NONE',  ( 92.69370383062501162, -211.3315407142195852, 87.94947916753382344 ) ) ;
#30486=ORIENTED_EDGE ( 'NONE', *, *, #33606, .F. ) ;
#30487=CARTESIAN_POINT ( 'NONE',  ( -96.32500000000001705, 92.29496732002878900, 79.73416666666666686 ) ) ;
#30489=VERTEX_POINT ( 'NONE', #43983 ) ;
#30493=CARTESIAN_POINT ( 'NONE',  ( -92.69370383062502583, 88.66845928578038638, 79.27114583420048177 ) ) ;
#30494=ORIENTED_EDGE ( 'NONE', *, *, #23694, .F. ) ;
#30507=ORIENTED_EDGE ( 'NONE', *, *, #65022, .T. ) ;
#30508=CARTESIAN_POINT ( 'NONE',  ( 97.30629616937498838, -211.3315407142195852, 79.11239583420046984 ) ) ;
#30511=CARTESIAN_POINT ( 'NONE',  ( -92.34999999999999432, -211.5299782133524218, 85.89895833506763267 ) ) ;
#30517=CARTESIAN_POINT ( 'NONE',  ( -96.15314808468745866, -211.9973110713294489, 80.85864583420047325 ) ) ;
#30518=CARTESIAN_POINT ( 'NONE',  ( -93.84685191531254134, 91.99731107132950569, 82.60489583420049087 ) ) ;
#30521=CARTESIAN_POINT ( 'NONE',  ( 93.84685191531248449, 91.99731107132950569, 79.37697916753380412 ) ) ;
#30522=ORIENTED_EDGE ( 'NONE', *, *, #63115, .F. ) ;
#30525=CARTESIAN_POINT ( 'NONE',  ( -92.34999999999999432, -211.5299782133524218, 76.92958333333332632 ) ) ;
#30528=CARTESIAN_POINT ( 'NONE',  ( -92.69370383062498320, -211.3315407142195852, 82.92239583420045790 ) ) ;
#30532=CARTESIAN_POINT ( 'NONE',  ( 92.34999999999999432, 90.00000000000002842, 80.47499999999999432 ) ) ;
#30540=CARTESIAN_POINT ( 'NONE',  ( 92.35000000001612364, -210.0000060634596082, 88.17456390440206349 ) ) ;
#30541=CARTESIAN_POINT ( 'NONE',  ( -96.15314808468752972, 91.99731107132950569, 84.45697916753380241 ) ) ;
#30553=LINE ( 'NONE', #6893, #55069 ) ;
#30556=CARTESIAN_POINT ( 'NONE',  ( -94.99999999999997158, -212.6630814284392557, 86.15031250086714465 ) ) ;
#30561=( BOUNDED_CURVE ( )  B_SPLINE_CURVE ( 2, ( #34767, #64088, #589 ),
 .UNSPECIFIED., .F., .F. ) 
 B_SPLINE_CURVE_WITH_KNOTS ( ( 3, 3 ),
 ( 0.9791666666666669627, 0.9841647806526062636 ),
 .UNSPECIFIED. ) 
 CURVE ( )  GEOMETRIC_REPRESENTATION_ITEM ( )  RATIONAL_B_SPLINE_CURVE ( ( 0.9999999999999935607, 0.9035746763527958691, 0.9459494432169044398 ) ) 
 REPRESENTATION_ITEM ( '' )  );
#30562=CARTESIAN_POINT ( 'NONE',  ( 92.69370383062498320, 91.33154071421968467, 75.14364583420049826 ) ) ;
#30564=CARTESIAN_POINT ( 'NONE',  ( -93.84685191531247028, -211.9973110713294489, 77.94822916753382458 ) ) ;
#30567=CARTESIAN_POINT ( 'NONE',  ( -92.35000000000674447, -209.9999940177768565, 82.14187520865739600 ) ) ;
#30569=CARTESIAN_POINT ( 'NONE',  ( -92.35000000005469190, 89.99998298270445218, 88.49187441316097136 ) ) ;
#30573=CARTESIAN_POINT ( 'NONE',  ( 96.15314808468750130, -211.9973110713294489, 78.42447916753381776 ) ) ;
#30577=ORIENTED_EDGE ( 'NONE', *, *, #44605, .T. ) ;
#30588=CARTESIAN_POINT ( 'NONE',  ( 93.84685191531248449, 91.99731107132950569, 80.80572916753382628 ) ) ;
#30602=CARTESIAN_POINT ( 'NONE',  ( -97.64999999999996305, -209.9999999999999716, 84.36437500173430237 ) ) ;
#30606=CARTESIAN_POINT ( 'NONE',  ( -97.64999999999994884, -208.4700217866474645, 80.50145833506765314 ) ) ;
#30607=CARTESIAN_POINT ( 'NONE',  ( 97.64999999999999147, -209.9999999999999716, 90.00000000000000000 ) ) ;
#30608=CARTESIAN_POINT ( 'NONE',  ( 97.64999999999997726, 88.47002178664753558, 77.00895833506763211 ) ) ;
#30609=CARTESIAN_POINT ( 'NONE',  ( -92.35000000000003695, 90.00000000000004263, 74.52187500173430124 ) ) ;
#30611=CARTESIAN_POINT ( 'NONE',  ( 97.30629616937498838, 90.00000000000002842, 78.05406250086716113 ) ) ;
#30621=DIRECTION ( 'NONE',  ( -0.000000000000000000, -0.000000000000000000, 1.000000000000000000 ) ) ;
#30625=ORIENTED_EDGE ( 'NONE', *, *, #24608, .T. ) ;
#30631=CARTESIAN_POINT ( 'NONE',  ( -93.84685191531247028, -211.9973110713294489, 77.31322916753381946 ) ) ;
#30633=EDGE_LOOP ( 'NONE', ( #20766, #68736, #65722, #22113 ) ) ;
#30641=CARTESIAN_POINT ( 'NONE',  ( 97.64999999999999147, 90.00000000000002842, 89.68250000000000455 ) ) ;
#30644=EDGE_CURVE ( 'NONE', #41411, #2356, #11984, .T. ) ;
#30646=EDGE_CURVE ( 'NONE', #36423, #44854, #1123, .T. ) ;
#30648=CARTESIAN_POINT ( 'NONE',  ( 97.30629616937498838, 90.00000000000002842, 83.76906250086716454 ) ) ;
#30649=CARTESIAN_POINT ( 'NONE',  ( -93.84685191531247028, -211.9973110713294489, 84.93322916753382401 ) ) ;
#30653=CARTESIAN_POINT ( 'NONE',  ( -97.64999999999996305, -209.9999999999999716, 80.47499999999999432 ) ) ;
#30654=CARTESIAN_POINT ( 'NONE',  ( -97.30629616937501680, 91.33154071421968467, 76.25489583420049655 ) ) ;
#30655=VECTOR ( 'NONE', #49892, 1000.000000000000000 ) ;
#30659=CARTESIAN_POINT ( 'NONE',  ( 92.69370383062501162, -209.9999999999999716, 85.83281250086714920 ) ) ;
#30665=CARTESIAN_POINT ( 'NONE',  ( 95.00000000000000000, -213.0599564267049857, 75.55375000000000796 ) ) ;
#30671=CARTESIAN_POINT ( 'NONE',  ( 95.00000000000000000, -207.3369185715606307, 79.48281250086715488 ) ) ;
#30677=CARTESIAN_POINT ( 'NONE',  ( 92.35000000000002274, -211.5299782133524502, 85.60791666666665378 ) ) ;
#30685=CARTESIAN_POINT ( 'NONE',  ( -97.30629616937501680, 91.33154071421968467, 84.66864583420047552 ) ) ;
#30689=CARTESIAN_POINT ( 'NONE',  ( 93.67500000000001137, -212.2949673200287179, 74.94520833506761903 ) ) ;
#30690=CARTESIAN_POINT ( 'NONE',  ( 94.99999999999998579, 93.05995642670504253, 75.87125000000000341 ) ) ;
#30695=CARTESIAN_POINT ( 'NONE',  ( -92.34999999999999432, -209.9999999999999716, 85.23749999999999716 ) ) ;
#30698=CARTESIAN_POINT ( 'NONE',  ( -93.67500000000003979, 92.29496732002878900, 84.78770833506763438 ) ) ;
#30699=CARTESIAN_POINT ( 'NONE',  ( 93.84685191531248449, 91.99731107132950569, 85.88572916753381037 ) ) ;
#30704=CARTESIAN_POINT ( 'NONE',  ( -96.32499999999996021, -207.7050326799711968, 78.54354166840096241 ) ) ;
#30709=CARTESIAN_POINT ( 'NONE',  ( -93.84685191531248449, -208.0026889286704943, 75.46114583420047950 ) ) ;
#30712=AXIS2_PLACEMENT_3D ( 'NONE', #7721, #53579, #25005 ) ;
#30717=CARTESIAN_POINT ( 'NONE',  ( -94.99999999999997158, -212.6630814284392557, 89.32531250086715602 ) ) ;
#30720=DIRECTION ( 'NONE',  ( 1.000000000000000000, 0.000000000000000000, 0.000000000000000000 ) ) ;
#30724=CARTESIAN_POINT ( 'NONE',  ( 92.69370383062498320, 88.66845928578037217, 89.21947916753381946 ) ) ;
#30727=CARTESIAN_POINT ( 'NONE',  ( 96.15314808468748708, 91.99731107132950569, 81.17614583420048291 ) ) ;
#30732=EDGE_CURVE ( 'NONE', #9512, #9077, #70218, .T. ) ;
#30733=CARTESIAN_POINT ( 'NONE',  ( -92.35000000000003695, 90.00000000000004263, 87.77749999999998920 ) ) ;
#30734=FACE_OUTER_BOUND ( 'NONE', #5053, .T. ) ;
#30735=EDGE_CURVE ( 'NONE', #45993, #53141, #31125, .T. ) ;
#30740=CARTESIAN_POINT ( 'NONE',  ( -97.30629616937501680, 91.33154071421968467, 87.68489583420047495 ) ) ;
#30746=VECTOR ( 'NONE', #35442, 1000.000000000000000 ) ;
#30748=CARTESIAN_POINT ( 'NONE',  ( 93.84685191531249870, -208.0026889286704943, 81.44072916753381719 ) ) ;
#30758=( BOUNDED_CURVE ( )  B_SPLINE_CURVE ( 2, ( #71701, #61931, #66454, #4420, #32212, #15306, #32595, #9673, #72077 ),
 .UNSPECIFIED., .F., .F. ) 
 B_SPLINE_CURVE_WITH_KNOTS ( ( 3, 2, 2, 2, 3 ),
 ( 0.8255245790564498254, 0.8325803338241195561, 0.8396360993650018312, 0.8466918649058843283, 0.8466920362367555963 ),
 .UNSPECIFIED. ) 
 CURVE ( )  GEOMETRIC_REPRESENTATION_ITEM ( )  RATIONAL_B_SPLINE_CURVE ( ( 1.000000000000000000, 0.8660254037844387076, 1.000000000000000000, 0.8660254037844387076, 1.000000000000000000, 0.8660254037844387076, 1.000000000000000000, 0.9999967467762123086, 0.9999934937104166810 ) ) 
 REPRESENTATION_ITEM ( '' )  );
#30760=VERTEX_POINT ( 'NONE', #7459 ) ;
#30761=CARTESIAN_POINT ( 'NONE',  ( 92.69370383062501162, -211.3315407142195852, 79.69447916753381378 ) ) ;
#30764=VERTEX_POINT ( 'NONE', #58585 ) ;
#30768=CARTESIAN_POINT ( 'NONE',  ( 97.65000000000000568, -208.4700217866474645, 80.21041666666666003 ) ) ;
#30772=CARTESIAN_POINT ( 'NONE',  ( 97.64999999999999147, -209.9999999999999716, 83.41187500173430180 ) ) ;
#30773=CARTESIAN_POINT ( 'NONE',  ( 92.34999999999999432, 90.00000000000002842, 85.55499999999999261 ) ) ;
#30780=CARTESIAN_POINT ( 'NONE',  ( -96.15314808468751551, 88.00268892867056536, 88.63739583420048973 ) ) ;
#30781=CARTESIAN_POINT ( 'NONE',  ( 94.99999999999998579, 92.66308142843935514, 85.67406250086715147 ) ) ;
#30783=CARTESIAN_POINT ( 'NONE',  ( 94.99999999999998579, 86.94004357329500010, 86.42812500173430124 ) ) ;
#30790=VERTEX_POINT ( 'NONE', #8572 ) ;
#30791=VERTEX_POINT ( 'NONE', #7086 ) ;
#30794=CARTESIAN_POINT ( 'NONE',  ( -92.35000000000003695, 90.00000000000004263, 85.87249999999998806 ) ) ;
#30800=CARTESIAN_POINT ( 'NONE',  ( -92.69370383062498320, -209.9999999999999716, 82.34031250086714238 ) ) ;
#30806=DIRECTION ( 'NONE',  ( -0.000000000000000000, -0.000000000000000000, 1.000000000000000000 ) ) ;
#30814=CARTESIAN_POINT ( 'NONE',  ( 97.24889018994936407, -210.5903413996855704, 74.79348190356850523 ) ) ;
#30816=CARTESIAN_POINT ( 'NONE',  ( -92.35000000000003695, 89.99999999755290503, 75.15687493081163950 ) ) ;
#30818=ADVANCED_FACE ( 'NONE', ( #2604 ), #54429, .F. ) ;
#30819=CARTESIAN_POINT ( 'NONE',  ( -96.15314808468751551, 88.00268892867056536, 75.77864583420047495 ) ) ;
#30829=CARTESIAN_POINT ( 'NONE',  ( 92.34999999999999432, -211.5299782133524502, 77.35291666666665833 ) ) ;
#30831=LINE ( 'NONE', #2318, #65288 ) ;
#30832=CARTESIAN_POINT ( 'NONE',  ( -93.67499999999998295, -212.2949673200287179, 88.30666666666665776 ) ) ;
#30833=VECTOR ( 'NONE', #15156, 1000.000000000000000 ) ;
#30838=CARTESIAN_POINT ( 'NONE',  ( 96.32499999999998863, -207.7050326799711968, 81.61270833506763722 ) ) ;
#30842=VERTEX_POINT ( 'NONE', #13819 ) ;
#30844=CARTESIAN_POINT ( 'NONE',  ( 93.84685191531251292, -211.9973110713294489, 85.30364583420046642 ) ) ;
#30845=CARTESIAN_POINT ( 'NONE',  ( 96.15314808468748708, -208.0026889286704943, 88.31989583420048007 ) ) ;
#30849=CARTESIAN_POINT ( 'NONE',  ( 97.30629616937498838, -211.3315407142195852, 88.79614583420050167 ) ) ;
#30854=CARTESIAN_POINT ( 'NONE',  ( -93.84685191531254134, 91.99731107132950569, 76.25489583420049655 ) ) ;
#30868=AXIS2_PLACEMENT_3D ( 'NONE', #63970, #12077, #22627 ) ;
#30875=CARTESIAN_POINT ( 'NONE',  ( 97.30629616937498838, -208.6684592857803011, 77.94822916753381037 ) ) ;
#30880=CARTESIAN_POINT ( 'NONE',  ( -97.64999999999996305, -211.5299782133524218, 78.70229166840096013 ) ) ;
#30882=CARTESIAN_POINT ( 'NONE',  ( 94.99999999999998579, 90.00000000000002842, 90.00000000000000000 ) ) ;
#30885=CARTESIAN_POINT ( 'NONE',  ( -96.15314808468747287, -208.0026889286704943, 80.01197916753380923 ) ) ;
#30887=CARTESIAN_POINT ( 'NONE',  ( -92.69370383062502583, 91.33154071421968467, 80.64697916753382856 ) ) ;
#30890=CARTESIAN_POINT ( 'NONE',  ( 93.84685191531248449, 88.00268892867053694, 81.49364583420047836 ) ) ;
#30892=CARTESIAN_POINT ( 'NONE',  ( 92.35001943615621656, 91.52998943482253935, 78.59645755884380947 ) ) ;
#30898=CARTESIAN_POINT ( 'NONE',  ( -94.99999999999997158, -212.6630814284392557, 84.08656250086714579 ) ) ;
#30906=CARTESIAN_POINT ( 'NONE',  ( -97.65000000000001990, 88.47002178664754979, 76.08291666666666231 ) ) ;
#30907=CARTESIAN_POINT ( 'NONE',  ( -92.35000000000005116, 88.47002178664754979, 84.62895833506763665 ) ) ;
#30909=CARTESIAN_POINT ( 'NONE',  ( -93.84685191531252713, 88.00268892867056536, 86.67947916753381321 ) ) ;
#30916=CARTESIAN_POINT ( 'NONE',  ( -96.15314808468751551, 88.00268892867056536, 75.77864583420047495 ) ) ;
#30917=VECTOR ( 'NONE', #56273, 1000.000000000000000 ) ;
#30924=DIRECTION ( 'NONE',  ( 1.000000000000000000, 0.000000000000000000, 0.000000000000000000 ) ) ;
#30925=CARTESIAN_POINT ( 'NONE',  ( -94.99999999999997158, -207.3369185715606307, 83.92781250086716227 ) ) ;
#30926=AXIS2_PLACEMENT_3D ( 'NONE', #26759, #66988, #48599 ) ;
#30929=CARTESIAN_POINT ( 'NONE',  ( -97.30629616937497417, -208.6684592857803295, 77.04864583420048518 ) ) ;
#30938=AXIS2_PLACEMENT_3D ( 'NONE', #674, #47236, #17920 ) ;
#30939=CARTESIAN_POINT ( 'NONE',  ( 95.00000000000000000, -212.6630814284392557, 89.32531250086715602 ) ) ;
#30941=CARTESIAN_POINT ( 'NONE',  ( 97.64999999999999147, 90.00002467581458632, 87.22187585518555863 ) ) ;
#30946=CARTESIAN_POINT ( 'NONE',  ( 2.500000000000029754, 73.00000000000001421, -255.0000000000000000 ) ) ;
#30958=CARTESIAN_POINT ( 'NONE',  ( 93.84685191531248449, 88.00268892867053694, 81.65239583420049030 ) ) ;
#30961=CARTESIAN_POINT ( 'NONE',  ( -93.67500000000003979, 87.70503267997129626, 85.13166666666666060 ) ) ;
#30968=ORIENTED_EDGE ( 'NONE', *, *, #62213, .T. ) ;
#30972=CARTESIAN_POINT ( 'NONE',  ( -97.50991008589734577, 90.12150787501450111, 74.91582548749275361 ) ) ;
#30978=CARTESIAN_POINT ( 'NONE',  ( -94.99999999999997158, -206.9400435732949575, 74.68062500173429896 ) ) ;
#30980=CARTESIAN_POINT ( 'NONE',  ( 94.99999999999998579, 93.05995642670504253, 75.31562500173430408 ) ) ;
#30981=CARTESIAN_POINT ( 'NONE',  ( -92.35000000000005116, 88.47002178664754979, 75.10395833506764518 ) ) ;
#30984=CARTESIAN_POINT ( 'NONE',  ( 97.30629616937498838, 90.00000000000002842, 77.41906250086715602 ) ) ;
#30991=CARTESIAN_POINT ( 'NONE',  ( -92.34999999999999432, -209.9999999999999716, 80.15749999999999886 ) ) ;
#31002=CARTESIAN_POINT ( 'NONE',  ( 92.69370383062501162, -209.9999999999999716, 89.64281250086713726 ) ) ;
#31005=CARTESIAN_POINT ( 'NONE',  ( 92.34999999999999432, 90.00000000000002842, 84.28499999999999659 ) ) ;
#31007=ORIENTED_EDGE ( 'NONE', *, *, #32664, .T. ) ;
#31008=DIRECTION ( 'NONE',  ( 1.000000000000000000, 0.000000000000000000, 0.000000000000000000 ) ) ;
#31015=CARTESIAN_POINT ( 'NONE',  ( -92.34999999999999432, -209.9999999999999716, 90.00000000000000000 ) ) ;
#31019=CARTESIAN_POINT ( 'NONE',  ( 96.15314808468748708, 88.00268892867053694, 84.93322916753382401 ) ) ;
#31022=CARTESIAN_POINT ( 'NONE',  ( -96.15314808468747287, -208.0026889286704943, 87.79072916753381151 ) ) ;
#31026=CARTESIAN_POINT ( 'NONE',  ( -92.34999999999999432, -208.4700217866474645, 80.84541666666666515 ) ) ;
#31027=CARTESIAN_POINT ( 'NONE',  ( -97.30629616937501680, 91.33154071421968467, 76.88989583420047325 ) ) ;
#31030=CARTESIAN_POINT ( 'NONE',  ( 92.69370383062501162, -208.6684592857803011, 85.14489583420048291 ) ) ;
#31031=VERTEX_POINT ( 'NONE', #20466 ) ;
#31045=CARTESIAN_POINT ( 'NONE',  ( 92.69370383062501162, -208.6684592857803295, 78.31864583420050963 ) ) ;
#31052=CARTESIAN_POINT ( 'NONE',  ( 93.67500000000001137, -207.7050326799711968, 81.00416666666666288 ) ) ;
#31054=ORIENTED_EDGE ( 'NONE', *, *, #67931, .T. ) ;
#31058=CARTESIAN_POINT ( 'NONE',  ( -93.84685191531254134, 91.99731107132950569, 84.50989583420049200 ) ) ;
#31061=CARTESIAN_POINT ( 'NONE',  ( 92.34999999999999432, 90.00000000000002842, 76.66499999999999204 ) ) ;
#31065=CARTESIAN_POINT ( 'NONE',  ( -92.34999999999999432, -208.4700217866474645, 85.36979166840096411 ) ) ;
#31067=EDGE_CURVE ( 'NONE', #35173, #48383, #11034, .T. ) ;
#31070=CARTESIAN_POINT ( 'NONE',  ( -95.00000000000002842, 93.05995642670501411, 86.11062500173430578 ) ) ;
#31071=CARTESIAN_POINT ( 'NONE',  ( 97.30629616937498838, 90.00000000000002842, 87.57906250086715261 ) ) ;
#31079=CARTESIAN_POINT ( 'NONE',  ( -92.35000000000003695, 90.00000000000004263, 82.06250000000000000 ) ) ;
#31081=ADVANCED_FACE ( 'NONE', ( #26091 ), #13699, .F. ) ;
#31084=AXIS2_PLACEMENT_3D ( 'NONE', #21776, #44725, #27407 ) ;
#31090=CARTESIAN_POINT ( 'NONE',  ( -92.69370383062498320, -209.9999999999999716, 85.03906250086714635 ) ) ;
#31091=ORIENTED_EDGE ( 'NONE', *, *, #71115, .F. ) ;
#31101=CARTESIAN_POINT ( 'NONE',  ( 92.69370383062498320, 88.66845928578035796, 82.07572916753382231 ) ) ;
#31109=LINE ( 'NONE', #24010, #27489 ) ;
#31114=CARTESIAN_POINT ( 'NONE',  ( -95.00000000000002842, 92.66308142843932671, 86.30906250086714238 ) ) ;
#31118=ADVANCED_FACE ( 'NONE', ( #3567 ), #27579, .F. ) ;
#31119=LINE ( 'NONE', #53688, #65675 ) ;
#31122=CARTESIAN_POINT ( 'NONE',  ( 97.64999999999999147, -209.9999999999999716, 83.33250000000001023 ) ) ;
#31123=CARTESIAN_POINT ( 'NONE',  ( 97.64999999999999147, 90.00000000000002842, 85.23749999999999716 ) ) ;
#31124=CARTESIAN_POINT ( 'NONE',  ( -100.0000000000000142, 95.00000000000002842, 90.00000000000000000 ) ) ;
#31125=CIRCLE ( 'NONE', #64741, 3.299999999999969624 ) ;
#31128=CARTESIAN_POINT ( 'NONE',  ( 96.15314808468750130, -211.9973110713294489, 82.39322916753381776 ) ) ;
#31136=LINE ( 'NONE', #37903, #22011 ) ;
#31140=CARTESIAN_POINT ( 'NONE',  ( 97.30629616937498838, -208.6684592857803011, 76.20197916753382117 ) ) ;
#31142=ORIENTED_EDGE ( 'NONE', *, *, #4247, .F. ) ;
#31152=CARTESIAN_POINT ( 'NONE',  ( 97.64999999999997726, -208.4700217866474645, 84.09979166840095388 ) ) ;
#31153=CARTESIAN_POINT ( 'NONE',  ( 96.32499999999998863, 87.70503267997126784, 83.86166666666666458 ) ) ;
#31155=EDGE_CURVE ( 'NONE', #47765, #34388, #26395, .T. ) ;
#31162=CARTESIAN_POINT ( 'NONE',  ( -92.69370383062505425, 91.33154071421968467, 88.26697916753381890 ) ) ;
#31163=CARTESIAN_POINT ( 'NONE',  ( 92.69370383062498320, 90.00000000000002842, 81.38781250086714181 ) ) ;
#31164=ORIENTED_EDGE ( 'NONE', *, *, #578, .T. ) ;
#31165=CARTESIAN_POINT ( 'NONE',  ( 92.34999999999999432, 91.52997821335252127, 83.67645833506762187 ) ) ;
#31167=ORIENTED_EDGE ( 'NONE', *, *, #62949, .F. ) ;
#31171=ORIENTED_EDGE ( 'NONE', *, *, #31324, .T. ) ;
#31172=CARTESIAN_POINT ( 'NONE',  ( 97.64999999999999147, -209.9999999999999716, 90.00000000000000000 ) ) ;
#31174=CARTESIAN_POINT ( 'NONE',  ( -96.32500000000001705, 92.29496732002878900, 84.17916666666666003 ) ) ;
#31176=CARTESIAN_POINT ( 'NONE',  ( 92.34999999999999432, 90.00000000000002842, 90.00000000000000000 ) ) ;
#31180=CARTESIAN_POINT ( 'NONE',  ( -96.15314808468747287, -208.0026889286704943, 81.28197916753380525 ) ) ;
#31182=CIRCLE ( 'NONE', #29937, 26.50000000000000355 ) ;
#31197=CARTESIAN_POINT ( 'NONE',  ( -96.15314808468751551, 88.00268892867056536, 75.14364583420046984 ) ) ;
#31198=CYLINDRICAL_SURFACE ( 'NONE', #31084, 2.649999999999985700 ) ;
#31206=CARTESIAN_POINT ( 'NONE',  ( 93.84685191531248449, 88.00268892867053694, 89.27239583420049485 ) ) ;
#31209=CARTESIAN_POINT ( 'NONE',  ( 97.65000000000000568, -211.5299782133524502, 78.83458333333334167 ) ) ;
#31211=CARTESIAN_POINT ( 'NONE',  ( -93.67499999999998295, -212.2949673200287179, 89.57666666666666799 ) ) ;
#31216=CARTESIAN_POINT ( 'NONE',  ( -97.64999999999996305, -209.9999999999999716, 84.92000000000000171 ) ) ;
#31217=( BOUNDED_CURVE ( )  B_SPLINE_CURVE ( 2, ( #49881, #31853, #72801, #55908, #6273, #12262, #17171 ),
 .UNSPECIFIED., .F., .F. ) 
 B_SPLINE_CURVE_WITH_KNOTS ( ( 3, 2, 2, 3 ),
 ( 0.9101937466136234001, 0.9172495203192131408, 0.9243052858601306099, 0.9313609857438962525 ),
 .UNSPECIFIED. ) 
 CURVE ( )  GEOMETRIC_REPRESENTATION_ITEM ( )  RATIONAL_B_SPLINE_CURVE ( ( 1.000000000000000000, 0.8660254037844387076, 1.000000000000000000, 0.8660254037844387076, 1.000000000000000000, 0.8660266504798329601, 0.9999975066324136019 ) ) 
 REPRESENTATION_ITEM ( '' )  );
#31224=ORIENTED_EDGE ( 'NONE', *, *, #63437, .T. ) ;
#31228=CARTESIAN_POINT ( 'NONE',  ( 92.69370383062501162, -209.9999999999999716, 81.38781250086714181 ) ) ;
#31237=VECTOR ( 'NONE', #47214, 1000.000000000000000 ) ;
#31238=CARTESIAN_POINT ( 'NONE',  ( -95.00000000000002842, 92.66308142843932671, 75.67281250086716682 ) ) ;
#31240=EDGE_LOOP ( 'NONE', ( #5659, #27377, #24071, #49726 ) ) ;
#31250=CARTESIAN_POINT ( 'NONE',  ( 93.67500000000001137, -212.2949673200287179, 86.29583333333333428 ) ) ;
#31255=CARTESIAN_POINT ( 'NONE',  ( 93.84685191531249870, -208.0026889286704943, 79.37697916753380412 ) ) ;
#31258=CYLINDRICAL_SURFACE ( 'NONE', #63056, 2.649999999999985700 ) ;
#31267=CARTESIAN_POINT ( 'NONE',  ( -94.99999999999997158, -207.3369185715606307, 82.49906250086714010 ) ) ;
#31268=CARTESIAN_POINT ( 'NONE',  ( -97.30629616937501680, 88.66845928578038638, 77.78947916753381264 ) ) ;
#31270=CARTESIAN_POINT ( 'NONE',  ( 97.30629616937498838, 90.00000000000002842, 80.43531250086714124 ) ) ;
#31271=ORIENTED_EDGE ( 'NONE', *, *, #10291, .T. ) ;
#31277=CARTESIAN_POINT ( 'NONE',  ( -96.15314808468745866, -211.9973110713294489, 81.49364583420047836 ) ) ;
#31278=CARTESIAN_POINT ( 'NONE',  ( 94.99999999999998579, 86.94004357329502852, 86.98374999999998636 ) ) ;
#31281=EDGE_LOOP ( 'NONE', ( #15439, #47407, #74060, #35837, #5469, #28886 ) ) ;
#31284=CARTESIAN_POINT ( 'NONE',  ( -92.35000000000005116, 88.47002178664754979, 75.65958333333333030 ) ) ;
#31286=CARTESIAN_POINT ( 'NONE',  ( -93.84685191531254134, 91.99731107132950569, 85.62114583420046188 ) ) ;
#31291=CARTESIAN_POINT ( 'NONE',  ( -92.69370383062502583, 88.66845928578038638, 75.30239583420048177 ) ) ;
#31297=DIRECTION ( 'NONE',  ( 1.000000000000000000, 0.000000000000000000, 0.000000000000000000 ) ) ;
#31298=CARTESIAN_POINT ( 'NONE',  ( 92.35000000000000853, -209.9999999999999716, 84.92000000000000171 ) ) ;
#31299=CARTESIAN_POINT ( 'NONE',  ( -92.69370383062498320, -208.6684592857803011, 81.28197916753381946 ) ) ;
#31307=VERTEX_POINT ( 'NONE', #61753 ) ;
#31316=CARTESIAN_POINT ( 'NONE',  ( 92.69370383062501162, -208.6684592857803011, 87.84364583420048689 ) ) ;
#31318=CARTESIAN_POINT ( 'NONE',  ( 92.35000000000000853, -209.9999999999999716, 87.45999999999999375 ) ) ;
#31324=EDGE_CURVE ( 'NONE', #14688, #17922, #26418, .T. ) ;
#31325=ORIENTED_EDGE ( 'NONE', *, *, #29535, .T. ) ;
#31327=ORIENTED_EDGE ( 'NONE', *, *, #8646, .T. ) ;
#31328=ORIENTED_EDGE ( 'NONE', *, *, #23923, .T. ) ;
#31335=CARTESIAN_POINT ( 'NONE',  ( 97.30629616937498838, 91.33154071421968467, 80.01197916753380923 ) ) ;
#31338=ORIENTED_EDGE ( 'NONE', *, *, #17898, .T. ) ;
#31352=CARTESIAN_POINT ( 'NONE',  ( -92.34999999999999432, -211.5299782133524502, 75.73895833506765030 ) ) ;
#31353=CARTESIAN_POINT ( 'NONE',  ( -95.00000000000002842, 92.66308142843932671, 87.73781250086715033 ) ) ;
#31354=CARTESIAN_POINT ( 'NONE',  ( 97.64999999999997726, 88.47002178664753558, 76.37395833506761278 ) ) ;
#31355=CARTESIAN_POINT ( 'NONE',  ( -97.65000000000001990, 88.47002178664754979, 77.43229166840096411 ) ) ;
#31357=CARTESIAN_POINT ( 'NONE',  ( 92.69370383062498320, 88.66845928578037217, 77.15447916753382174 ) ) ;
#31384=ADVANCED_FACE ( 'NONE', ( #33156 ), #73001, .F. ) ;
#31386=CARTESIAN_POINT ( 'NONE',  ( 92.35000000009274856, -209.9999861897330788, 80.55392363656960697 ) ) ;
#31388=EDGE_CURVE ( 'NONE', #71815, #53141, #4992, .T. ) ;
#31392=CARTESIAN_POINT ( 'NONE',  ( 93.84685191531248449, 91.99731107132950569, 83.34572916753383254 ) ) ;
#31393=CARTESIAN_POINT ( 'NONE',  ( -97.30629616937497417, -211.3315407142195852, 84.77447916753381207 ) ) ;
#31400=CARTESIAN_POINT ( 'NONE',  ( -94.99999999999997158, -213.0599564267049857, 78.09374999999998579 ) ) ;
#31401=CARTESIAN_POINT ( 'NONE',  ( 92.35000000000000853, -209.9999999999999716, 78.57000000000000739 ) ) ;
#31404=CARTESIAN_POINT ( 'NONE',  ( 96.15314808468748708, -208.0026889286704943, 83.08114583420048405 ) ) ;
#31408=ORIENTED_EDGE ( 'NONE', *, *, #41607, .T. ) ;
#31411=ORIENTED_EDGE ( 'NONE', *, *, #58858, .F. ) ;
#31420=CARTESIAN_POINT ( 'NONE',  ( 93.84685191531251292, -211.9973110713294489, 78.47739583420049314 ) ) ;
#31424=( BOUNDED_CURVE ( )  B_SPLINE_CURVE ( 2, ( #34302, #36426, #71366, #35681, #65390 ),
 .UNSPECIFIED., .F., .F. ) 
 B_SPLINE_CURVE_WITH_KNOTS ( ( 3, 2, 3 ),
 ( 0.9525283480321510288, 0.9595841135600021721, 0.9629953541049918186 ),
 .UNSPECIFIED. ) 
 CURVE ( )  GEOMETRIC_REPRESENTATION_ITEM ( )  RATIONAL_B_SPLINE_CURVE ( ( 1.000000000000000000, 0.8660254037844387076, 1.000000000000000000, 0.9352274998423498742, 0.9330859296547722170 ) ) 
 REPRESENTATION_ITEM ( '' )  );
#31428=CARTESIAN_POINT ( 'NONE',  ( 96.32499999999998863, -212.2949673200287179, 81.32166666666667254 ) ) ;
#31429=EDGE_LOOP ( 'NONE', ( #59548, #14489, #68687, #6605 ) ) ;
#31432=ORIENTED_EDGE ( 'NONE', *, *, #23516, .T. ) ;
#31434=CARTESIAN_POINT ( 'NONE',  ( -92.69370383062504004, 90.00000000000004263, 83.13406250086715943 ) ) ;
#31437=CARTESIAN_POINT ( 'NONE',  ( 96.32499999999997442, 92.29496732002878900, 75.18333333333332291 ) ) ;
#31440=CARTESIAN_POINT ( 'NONE',  ( -97.64999999999996305, -209.9999999999999716, 84.36437500173430237 ) ) ;
#31444=CARTESIAN_POINT ( 'NONE',  ( -96.32500000000001705, 87.70503267997129626, 85.10520833506762983 ) ) ;
#31446=CARTESIAN_POINT ( 'NONE',  ( 92.69370383062498320, 91.33154071421968467, 85.93864583420048575 ) ) ;
#31462=CARTESIAN_POINT ( 'NONE',  ( -92.34999999999986642, -211.5299782133523649, 83.27958333333332064 ) ) ;
#31464=CARTESIAN_POINT ( 'NONE',  ( -92.69370383062498320, -211.3315407142195852, 84.98614583420047097 ) ) ;
#31472=CARTESIAN_POINT ( 'NONE',  ( 97.64999999999999147, 90.00000000000002842, 86.50750000000000739 ) ) ;
#31474=CARTESIAN_POINT ( 'NONE',  ( 97.64999999999999147, -209.9999999999999716, 82.77687500173431090 ) ) ;
#31475=CARTESIAN_POINT ( 'NONE',  ( 93.84685191531248449, 91.99731107132950569, 78.10697916753380809 ) ) ;
#31481=CARTESIAN_POINT ( 'NONE',  ( -97.65000000000001990, 90.00000000000004263, 76.74437500173429783 ) ) ;
#31487=CARTESIAN_POINT ( 'NONE',  ( -97.30629616937501680, 91.33154071421968467, 81.96989583420047154 ) ) ;
#31491=ORIENTED_EDGE ( 'NONE', *, *, #53048, .T. ) ;
#31497=CARTESIAN_POINT ( 'NONE',  ( 92.69370383062501162, -209.9999999999999716, 79.64156250086715261 ) ) ;
#31499=ORIENTED_EDGE ( 'NONE', *, *, #67253, .T. ) ;
#31503=DIRECTION ( 'NONE',  ( 0.000000000000000000, 0.000000000000000000, 1.000000000000000000 ) ) ;
#31508=CARTESIAN_POINT ( 'NONE',  ( 96.15314808468748708, -208.0026889286704943, 76.25489583420049655 ) ) ;
#31511=ORIENTED_EDGE ( 'NONE', *, *, #26702, .F. ) ;
#31514=CARTESIAN_POINT ( 'NONE',  ( -95.00000000000002842, 86.94004357329504273, 83.17374999999999829 ) ) ;
#31518=ORIENTED_EDGE ( 'NONE', *, *, #27903, .F. ) ;
#31520=CARTESIAN_POINT ( 'NONE',  ( 97.64999999999999147, -209.9999999999999716, 82.14187500173429157 ) ) ;
#31521=CARTESIAN_POINT ( 'NONE',  ( 97.64999999999997726, 91.52997821335252127, 85.29041666666665833 ) ) ;
#31524=CARTESIAN_POINT ( 'NONE',  ( -100.0000000000000142, 95.00000000000002842, 90.00000000000000000 ) ) ;
#31527=CARTESIAN_POINT ( 'NONE',  ( -96.15314808468751551, 88.00268892867056536, 87.36739583420049371 ) ) ;
#31528=CARTESIAN_POINT ( 'NONE',  ( 94.99999999999998579, 92.66308142843935514, 83.13406250086714522 ) ) ;
#31530=CARTESIAN_POINT ( 'NONE',  ( 94.99999999999998579, 86.94004357329500010, 81.34812500173430294 ) ) ;
#31533=CARTESIAN_POINT ( 'NONE',  ( 92.35000000000000853, -209.9999999999999716, 77.93499999999998806 ) ) ;
#31539=CARTESIAN_POINT ( 'NONE',  ( -96.32500000000001705, 87.70503267997129626, 83.12083333333332291 ) ) ;
#31545=CARTESIAN_POINT ( 'NONE',  ( -94.99999999999997158, -212.6630814284392557, 79.00656250086713328 ) ) ;
#31560=CARTESIAN_POINT ( 'NONE',  ( -93.67500000000003979, 92.29496732002878900, 88.59770833506763665 ) ) ;
#31563=CARTESIAN_POINT ( 'NONE',  ( -92.69370383062504004, 90.00000000000004263, 76.62531250086713897 ) ) ;
#31569=CARTESIAN_POINT ( 'NONE',  ( -2.499999999999973355, 65.00000000000000000, -290.0000000000000568 ) ) ;
#31576=CARTESIAN_POINT ( 'NONE',  ( -93.67499999999998295, -207.7050326799711968, 89.15333333333333599 ) ) ;
#31580=ORIENTED_EDGE ( 'NONE', *, *, #1333, .T. ) ;
#31585=ADVANCED_FACE ( 'NONE', ( #46308 ), #69235, .F. ) ;
#31592=CARTESIAN_POINT ( 'NONE',  ( 92.69370383062501162, -208.6684592857803295, 81.96989583420047154 ) ) ;
#31593=CARTESIAN_POINT ( 'NONE',  ( 97.30629616937498838, -211.3315407142195852, 87.52614583420049144 ) ) ;
#31595=CARTESIAN_POINT ( 'NONE',  ( 95.00000000000000000, -212.6630814284392557, 86.15031250086714465 ) ) ;
#31600=CARTESIAN_POINT ( 'NONE',  ( -92.69370383062504004, 90.00000000000004263, 78.68906250086715204 ) ) ;
#31605=ORIENTED_EDGE ( 'NONE', *, *, #64082, .F. ) ;
#31612=DIRECTION ( 'NONE',  ( -0.000000000000000000, -0.000000000000000000, 1.000000000000000000 ) ) ;
#31615=ADVANCED_FACE ( 'NONE', ( #3704 ), #21317, .F. ) ;
#31619=CARTESIAN_POINT ( 'NONE',  ( 92.69370383062501162, -211.3315407142195852, 78.90072916753381094 ) ) ;
#31622=CARTESIAN_POINT ( 'NONE',  ( -92.34999999999999432, -210.0000000198591295, 85.95187500101400246 ) ) ;
#31629=CARTESIAN_POINT ( 'NONE',  ( -97.64999999980591383, 89.99998015720542810, 86.27002759516649633 ) ) ;
#31631=CARTESIAN_POINT ( 'NONE',  ( -97.30629616937497417, -208.6684592857803011, 79.42989583420046529 ) ) ;
#31633=CARTESIAN_POINT ( 'NONE',  ( -92.69370383062502583, 88.66845928578038638, 77.36614583420048064 ) ) ;
#31635=CARTESIAN_POINT ( 'NONE',  ( 96.15314808468748708, 88.00268892867053694, 79.05947916753380866 ) ) ;
#31638=CARTESIAN_POINT ( 'NONE',  ( -94.99999999999997158, -212.6630814284392557, 88.53156250086713897 ) ) ;
#31639=CARTESIAN_POINT ( 'NONE',  ( -97.64999999999996305, -209.9999999999999716, 76.66499999999999204 ) ) ;
#31642=CARTESIAN_POINT ( 'NONE',  ( -94.99999999999997158, -207.3369185715606307, 83.13406250086714522 ) ) ;
#31652=CARTESIAN_POINT ( 'NONE',  ( -96.15314808468752972, 91.99731107132950569, 85.72697916753379843 ) ) ;
#31656=( BOUNDED_CURVE ( )  B_SPLINE_CURVE ( 2, ( #65985, #24999, #32482, #47933, #59593, #66712, #8462, #19356, #31742 ),
 .UNSPECIFIED., .F., .F. ) 
 B_SPLINE_CURVE_WITH_KNOTS ( ( 3, 2, 2, 2, 3 ),
 ( 0.08466915177892291033, 0.08466918649058885471, 0.09172495203147111587, 0.09878071757235337702, 0.1058364832022827828 ),
 .UNSPECIFIED. ) 
 CURVE ( )  GEOMETRIC_REPRESENTATION_ITEM ( )  RATIONAL_B_SPLINE_CURVE ( ( 0.9999986817990127452, 0.9999993408962638552, 1.000000000000000000, 0.8660254037844387076, 1.000000000000000000, 0.8660254037844387076, 1.000000000000000000, 0.8660254037844387076, 1.000000000000000000 ) ) 
 REPRESENTATION_ITEM ( '' )  );
#31667=CARTESIAN_POINT ( 'NONE',  ( -96.15314808468747287, -208.0026889286704943, 83.98072916753382344 ) ) ;
#31672=EDGE_CURVE ( 'NONE', #26258, #70972, #21112, .T. ) ;
#31676=DIRECTION ( 'NONE',  ( 0.000000000000000000, -0.000000000000000000, 1.000000000000000000 ) ) ;
#31678=CARTESIAN_POINT ( 'NONE',  ( 95.00000000000000000, -209.9999999999999716, 90.00000000000000000 ) ) ;
#31679=DIRECTION ( 'NONE',  ( -0.000000000000000000, -0.000000000000000000, 1.000000000000000000 ) ) ;
#31680=CARTESIAN_POINT ( 'NONE',  ( -12.75000000000000000, -120.0000000000000000, -80.00000000000001421 ) ) ;
#31683=DIRECTION ( 'NONE',  ( -0.000000000000000000, -0.000000000000000000, 1.000000000000000000 ) ) ;
#31685=CARTESIAN_POINT ( 'NONE',  ( 92.35000000003284981, 90.00000839192529156, 86.90410584365271518 ) ) ;
#31688=CARTESIAN_POINT ( 'NONE',  ( -97.64999999978461176, -209.9999789922612479, 79.91868729551984529 ) ) ;
#31696=DIRECTION ( 'NONE',  ( -0.000000000000000000, -0.000000000000000000, 1.000000000000000000 ) ) ;
#31700=CARTESIAN_POINT ( 'NONE',  ( 92.69370383062498320, 90.00000000000002842, 79.00656250086716170 ) ) ;
#31706=ORIENTED_EDGE ( 'NONE', *, *, #38596, .T. ) ;
#31708=VERTEX_POINT ( 'NONE', #47414 ) ;
#31718=CARTESIAN_POINT ( 'NONE',  ( -94.99999999999997158, -213.0599564267049857, 76.26812500173430465 ) ) ;
#31720=CARTESIAN_POINT ( 'NONE',  ( -97.30629616937501680, 91.33154071421968467, 89.74864583420048803 ) ) ;
#31722=CARTESIAN_POINT ( 'NONE',  ( 96.32499999999997442, 92.29496732002878900, 74.62770833506762358 ) ) ;
#31723=CARTESIAN_POINT ( 'NONE',  ( -97.30629616937501680, 91.33154071421968467, 87.68489583420047495 ) ) ;
#31726=CARTESIAN_POINT ( 'NONE',  ( 93.84685191531248449, 88.00268892867053694, 75.93739583420048689 ) ) ;
#31729=CARTESIAN_POINT ( 'NONE',  ( 97.64999999999997726, -211.5299782133524218, 87.72458333333332803 ) ) ;
#31731=CARTESIAN_POINT ( 'NONE',  ( -95.00000000000002842, 93.05995642670504253, 78.49062500173430124 ) ) ;
#31742=CARTESIAN_POINT ( 'NONE',  ( 97.64999999999999147, -210.0000000334413244, 87.85687500050293863 ) ) ;
#31746=CARTESIAN_POINT ( 'NONE',  ( -92.69370383062498320, -208.6684592857803011, 75.56697916753383026 ) ) ;
#31748=ORIENTED_EDGE ( 'NONE', *, *, #58478, .T. ) ;
#31749=CARTESIAN_POINT ( 'NONE',  ( -93.84685191531252713, 88.00268892867056536, 82.86947916753379673 ) ) ;
#31751=CYLINDRICAL_SURFACE ( 'NONE', #51083, 2.649999999999985700 ) ;
#31755=CARTESIAN_POINT ( 'NONE',  ( -94.99999999999997158, -206.9400435732949575, 87.30124999999999602 ) ) ;
#31761=CARTESIAN_POINT ( 'NONE',  ( 94.99999999999998579, 87.33691857156068750, 85.51531250086715374 ) ) ;
#31762=CARTESIAN_POINT ( 'NONE',  ( -92.69370383062498320, -208.6684592857803295, 83.18697916753382060 ) ) ;
#31763=CARTESIAN_POINT ( 'NONE',  ( 94.99999999999998579, 90.00000000000002842, 90.00000000000000000 ) ) ;
#31766=CARTESIAN_POINT ( 'NONE',  ( -92.34999999999999432, -211.5299782133524502, 78.19958333333332234 ) ) ;
#31769=CARTESIAN_POINT ( 'NONE',  ( 93.84685191531251292, -211.9973110713294489, 82.76364583420047438 ) ) ;
#31779=CARTESIAN_POINT ( 'NONE',  ( 95.00000000000000000, -207.3369185715606307, 76.94281250086714863 ) ) ;
#31783=EDGE_CURVE ( 'NONE', #44748, #25853, #43751, .T. ) ;
#31786=CARTESIAN_POINT ( 'NONE',  ( -92.35000000000005116, 88.47002178664754979, 83.35895833506764063 ) ) ;
#31787=CARTESIAN_POINT ( 'NONE',  ( 95.00000000000000000, -213.0599564267049857, 82.53874999999999318 ) ) ;
#31792=ORIENTED_EDGE ( 'NONE', *, *, #31067, .T. ) ;
#31794=CARTESIAN_POINT ( 'NONE',  ( -92.34999999999999432, -211.5299782133524218, 86.53395833506763779 ) ) ;
#31795=EDGE_CURVE ( 'NONE', #2080, #3079, #59120, .T. ) ;
#31797=CARTESIAN_POINT ( 'NONE',  ( -93.84685191531254134, 91.99731107132950569, 85.14489583420048291 ) ) ;
#31802=CARTESIAN_POINT ( 'NONE',  ( -93.67499999999998295, -212.2949673200287179, 83.94104166840097037 ) ) ;
#31804=CARTESIAN_POINT ( 'NONE',  ( -94.99999999999997158, -213.0599564267049857, 85.79312500173431033 ) ) ;
#31807=ORIENTED_EDGE ( 'NONE', *, *, #43066, .T. ) ;
#31808=CARTESIAN_POINT ( 'NONE',  ( -97.65000000000001990, 90.00000000000004263, 84.36437500173430237 ) ) ;
#31810=CARTESIAN_POINT ( 'NONE',  ( 92.69370383062498320, 88.66845928578037217, 87.94947916753382344 ) ) ;
#31813=DIRECTION ( 'NONE',  ( 1.000000000000000000, 0.000000000000000000, 0.000000000000000000 ) ) ;
#31814=LINE ( 'NONE', #65678, #49822 ) ;
#31818=CARTESIAN_POINT ( 'NONE',  ( -95.00000000000002842, 93.05995642670504253, 81.03062500173430749 ) ) ;
#31823=CARTESIAN_POINT ( 'NONE',  ( 2.500000000000034639, 90.00000000000000000, -310.0000000000000000 ) ) ;
#31827=CARTESIAN_POINT ( 'NONE',  ( -97.30629616937497417, -208.6684592857803011, 83.39864583420050792 ) ) ;
#31829=VECTOR ( 'NONE', #19020, 1000.000000000000000 ) ;
#31830=CARTESIAN_POINT ( 'NONE',  ( 97.65000000000004832, -211.5299782133523934, 81.37458333333333371 ) ) ;
#31835=CARTESIAN_POINT ( 'NONE',  ( 97.64999999964362587, 89.99995654222556141, 89.12687334326064104 ) ) ;
#31838=CARTESIAN_POINT ( 'NONE',  ( 94.99999999999998579, 92.66308142843935514, 89.64281250086715147 ) ) ;
#31840=CARTESIAN_POINT ( 'NONE',  ( 96.15314808468748708, 88.00268892867053694, 79.69447916753379957 ) ) ;
#31849=CARTESIAN_POINT ( 'NONE',  ( -92.69370383062494057, -209.7238243954290340, 74.79348190356849102 ) ) ;
#31853=CARTESIAN_POINT ( 'NONE',  ( -92.34999999999999432, -211.5299782133524218, 75.73895833506765030 ) ) ;
#31855=CARTESIAN_POINT ( 'NONE',  ( -93.84685191531254134, 91.99731107132950569, 83.08114583420048405 ) ) ;
#31861=( BOUNDED_CURVE ( )  B_SPLINE_CURVE ( 2, ( #71178, #48994, #60669, #24961, #59936, #8424, #70818, #66314, #8787 ),
 .UNSPECIFIED., .F., .F. ) 
 B_SPLINE_CURVE_WITH_KNOTS ( ( 3, 2, 2, 2, 3 ),
 ( 0.08466915177892317401, 0.08466918649058881308, 0.09172495203147107423, 0.09878071757235333539, 0.1058364832022826857 ),
 .UNSPECIFIED. ) 
 CURVE ( )  GEOMETRIC_REPRESENTATION_ITEM ( )  RATIONAL_B_SPLINE_CURVE ( ( 0.9999986817990245136, 0.9999993408962697394, 1.000000000000000000, 0.8660254037844387076, 1.000000000000000000, 0.8660254037844387076, 1.000000000000000000, 0.8660254037844387076, 1.000000000000000000 ) ) 
 REPRESENTATION_ITEM ( '' )  );
#31863=CARTESIAN_POINT ( 'NONE',  ( 92.35000000045006630, -210.0000310946952595, 88.81037122969986797 ) ) ;
#31864=CARTESIAN_POINT ( 'NONE',  ( 96.90829729882861443, 88.16127723153182671, 74.99954709728268654 ) ) ;
#31867=CARTESIAN_POINT ( 'NONE',  ( 95.00000000000000000, -207.3369185715606307, 78.21281250086717307 ) ) ;
#31871=DIRECTION ( 'NONE',  ( 0.000000000000000000, 0.000000000000000000, 1.000000000000000000 ) ) ;
#31876=CARTESIAN_POINT ( 'NONE',  ( 96.15314808468750130, -211.9973110713294489, 76.04322916753382344 ) ) ;
#31885=SHAPE_REPRESENTATION_RELATIONSHIP ( 'NONE' , 'NONE' ,  #65179, #59777 ) ;
#31889=VERTEX_POINT ( 'NONE', #61940 ) ;
#31890=CARTESIAN_POINT ( 'NONE',  ( 97.64999999999999147, 90.00000000000002842, 90.00000000000000000 ) ) ;
#31891=CARTESIAN_POINT ( 'NONE',  ( 96.32499999999998863, -207.7050326799711968, 81.61270833506763722 ) ) ;
#31892=EDGE_CURVE ( 'NONE', #54291, #56237, #33339, .T. ) ;
#31893=CARTESIAN_POINT ( 'NONE',  ( 97.64999999999997726, 91.52997821335252127, 84.02041666666667652 ) ) ;
#31902=CARTESIAN_POINT ( 'NONE',  ( -96.15314808468752972, 91.99731107132950569, 88.42572916753381662 ) ) ;
#31903=CARTESIAN_POINT ( 'NONE',  ( 93.84685191531248449, 88.00268892867053694, 80.22364583420046813 ) ) ;
#31905=CARTESIAN_POINT ( 'NONE',  ( 96.32499999999998863, 87.70503267997126784, 83.30604166840096525 ) ) ;
#31911=EDGE_CURVE ( 'NONE', #13389, #23740, #33180, .T. ) ;
#31916=CARTESIAN_POINT ( 'NONE',  ( -94.99999999999997158, -206.9400435732949575, 81.03062500173430749 ) ) ;
#31917=CARTESIAN_POINT ( 'NONE',  ( 97.64999999999997726, 91.52997821335252127, 87.90979166840095615 ) ) ;
#31920=CARTESIAN_POINT ( 'NONE',  ( -94.99999999999997158, -207.3369185715606307, 80.59406250086715318 ) ) ;
#31924=CYLINDRICAL_SURFACE ( 'NONE', #68188, 2.649999999999999467 ) ;
#31930=CARTESIAN_POINT ( 'NONE',  ( 92.69370383062498320, 91.33154071421968467, 88.31989583420048007 ) ) ;
#31931=CARTESIAN_POINT ( 'NONE',  ( -92.34999999999999432, -209.9999999999999716, 85.87249999999998806 ) ) ;
#31940=DIRECTION ( 'NONE',  ( 1.000000000000000000, 0.000000000000000000, 0.000000000000000000 ) ) ;
#31941=CARTESIAN_POINT ( 'NONE',  ( 96.15314808468748708, 91.99731107132950569, 89.58989583420049030 ) ) ;
#31942=DIRECTION ( 'NONE',  ( 1.000000000000000000, 0.000000000000000000, 0.000000000000000000 ) ) ;
#31945=CARTESIAN_POINT ( 'NONE',  ( -92.34999999999999432, -208.4700217866474645, 88.46541666666665549 ) ) ;
#31947=CARTESIAN_POINT ( 'NONE',  ( 97.64999999999601243, 89.99999541993086893, 76.42687486206342840 ) ) ;
#31948=PRODUCT ( 'housing', 'housing', '', ( #45623 ) ) ;
#31961=CARTESIAN_POINT ( 'NONE',  ( 93.84685191531251292, -211.9973110713294489, 80.85864583420047325 ) ) ;
#31962=CARTESIAN_POINT ( 'NONE',  ( 92.69370383062501162, -208.6684592857803295, 84.03364583420049883 ) ) ;
#31963=VERTEX_POINT ( 'NONE', #41972 ) ;
#31964=CARTESIAN_POINT ( 'NONE',  ( 96.15314808468750130, -211.9973110713294489, 86.20322916753382003 ) ) ;
#31966=ADVANCED_FACE ( 'NONE', ( #24309 ), #69417, .F. ) ;
#31969=CARTESIAN_POINT ( 'NONE',  ( -95.00000000000002842, 92.66308142843932671, 77.57781250086715374 ) ) ;
#31971=EDGE_CURVE ( 'NONE', #41695, #57350, #63388, .T. ) ;
#31974=ORIENTED_EDGE ( 'NONE', *, *, #673, .F. ) ;
#31975=CARTESIAN_POINT ( 'NONE',  ( 93.67499999999998295, 92.29496732002878900, 88.06854166840095388 ) ) ;
#31988=CARTESIAN_POINT ( 'NONE',  ( 97.30629616937498838, -208.6684592857803011, 78.58322916753381548 ) ) ;
#32000=CARTESIAN_POINT ( 'NONE',  ( -92.69370383062504004, 90.00000000000004263, 80.59406250086715318 ) ) ;
#32003=CARTESIAN_POINT ( 'NONE',  ( 97.30629616937498838, 88.66845928578037217, 77.84239583420045960 ) ) ;
#32006=CARTESIAN_POINT ( 'NONE',  ( -97.30629616937497417, -208.6684592857803011, 88.95489583420048518 ) ) ;
#32010=CARTESIAN_POINT ( 'NONE',  ( -96.15314808468747287, -208.0026889286704943, 83.18697916753382060 ) ) ;
#32011=CARTESIAN_POINT ( 'NONE',  ( 2.499999999999981348, -79.99999999999998579, -280.0000000000000000 ) ) ;
#32019=FACE_OUTER_BOUND ( 'NONE', #63396, .T. ) ;
#32022=CARTESIAN_POINT ( 'NONE',  ( -92.69370383062504004, 90.00000000000004263, 86.78531250086714977 ) ) ;
#32032=CARTESIAN_POINT ( 'NONE',  ( -96.15314808468747287, -208.0026889286704943, 81.44072916753381719 ) ) ;
#32039=ORIENTED_EDGE ( 'NONE', *, *, #35209, .T. ) ;
#32040=DIRECTION ( 'NONE',  ( 1.000000000000000000, 0.000000000000000000, 0.000000000000000000 ) ) ;
#32046=CYLINDRICAL_SURFACE ( 'NONE', #1326, 2.649999999999985700 ) ;
#32047=EDGE_LOOP ( 'NONE', ( #610, #413, #39056, #43593 ) ) ;
#32057=EDGE_CURVE ( 'NONE', #47514, #17108, #10574, .T. ) ;
#32063=EDGE_LOOP ( 'NONE', ( #7872, #53541, #7838, #32447, #55659 ) ) ;
#32070=CARTESIAN_POINT ( 'NONE',  ( 92.69370383062498320, 91.33154071421968467, 75.14364583420049826 ) ) ;
#32072=ADVANCED_FACE ( 'NONE', ( #55088 ), #38168, .F. ) ;
#32074=VERTEX_POINT ( 'NONE', #59629 ) ;
#32077=CARTESIAN_POINT ( 'NONE',  ( 92.69370383062498320, 91.33154071421968467, 88.31989583420046586 ) ) ;
#32079=CARTESIAN_POINT ( 'NONE',  ( 97.30629616937498838, -208.6684592857803011, 89.37822916753381719 ) ) ;
#32083=CARTESIAN_POINT ( 'NONE',  ( 96.32499999999997442, 92.29496732002878900, 77.80270833506763495 ) ) ;
#32087=CARTESIAN_POINT ( 'NONE',  ( -96.32499999999996021, -207.7050326799711968, 75.36854166840096525 ) ) ;
#32088=EDGE_CURVE ( 'NONE', #18817, #3169, #38468, .T. ) ;
#32092=CARTESIAN_POINT ( 'NONE',  ( 97.30629616937498838, 90.00000000000002842, 86.78531250086714977 ) ) ;
#32093=CARTESIAN_POINT ( 'NONE',  ( -96.15314808468752972, 91.99731107132950569, 87.63197916753379957 ) ) ;
#32094=( BOUNDED_CURVE ( )  B_SPLINE_CURVE ( 2, ( #22951, #61677, #23313, #10164, #67689, #56028, #4550 ),
 .UNSPECIFIED., .F., .F. ) 
 B_SPLINE_CURVE_WITH_KNOTS ( ( 3, 2, 2, 3 ),
 ( 0.8125000000000002220, 0.8194444444444446418, 0.8263888888888889506, 0.8333333333333334814 ),
 .UNSPECIFIED. ) 
 CURVE ( )  GEOMETRIC_REPRESENTATION_ITEM ( )  RATIONAL_B_SPLINE_CURVE ( ( 0.9999999999999956701, 0.8660254037844430375, 1.000000000000000000, 0.8660254037844387076, 1.000000000000000000, 0.8660254037844365982, 1.000000000000002220 ) ) 
 REPRESENTATION_ITEM ( '' )  );
#32096=CARTESIAN_POINT ( 'NONE',  ( 96.15314808468748708, 91.99731107132950569, 77.52489583420047836 ) ) ;
#32098=DIRECTION ( 'NONE',  ( -0.000000000000000000, -0.000000000000000000, 1.000000000000000000 ) ) ;
#32100=CARTESIAN_POINT ( 'NONE',  ( 95.00000000000000000, -213.0599564267049857, 77.53812500173428646 ) ) ;
#32101=CARTESIAN_POINT ( 'NONE',  ( -97.65000000000001990, 90.00000000000004263, 89.36499999999999488 ) ) ;
#32103=PLANE ( 'NONE',  #7230 ) ;
#32108=CARTESIAN_POINT ( 'NONE',  ( -95.00000000000002842, 93.05995642670501411, 80.31624999999998238 ) ) ;
#32110=CARTESIAN_POINT ( 'NONE',  ( 92.35000000000007958, -208.4700217866474361, 82.96208333333332519 ) ) ;
#32116=CARTESIAN_POINT ( 'NONE',  ( -93.84685191531252713, 88.00268892867056536, 80.96447916753380980 ) ) ;
#32118=DIRECTION ( 'NONE',  ( -0.000000000000000000, -0.000000000000000000, 1.000000000000000000 ) ) ;
#32126=CARTESIAN_POINT ( 'NONE',  ( 96.15314808468748708, 91.99731107132950569, 80.06489583420048461 ) ) ;
#32127=CARTESIAN_POINT ( 'NONE',  ( -94.99999999999997158, -212.6630814284392557, 84.24531250086717193 ) ) ;
#32130=CARTESIAN_POINT ( 'NONE',  ( -96.32499999999996021, -212.2949673200287179, 81.21583333333333599 ) ) ;
#32131=CARTESIAN_POINT ( 'NONE',  ( -93.67499999999998295, -207.7050326799711968, 77.72333333333332916 ) ) ;
#32134=CARTESIAN_POINT ( 'NONE',  ( 97.30629616937498838, -209.9999999999999716, 82.34031250086714238 ) ) ;
#32138=ORIENTED_EDGE ( 'NONE', *, *, #20865, .T. ) ;
#32145=CARTESIAN_POINT ( 'NONE',  ( -95.00000000000002842, 86.94004357329504273, 79.44312500173430180 ) ) ;
#32148=CARTESIAN_POINT ( 'NONE',  ( 92.69370383062501162, -211.3315407142195852, 77.78947916753381264 ) ) ;
#32149=CYLINDRICAL_SURFACE ( 'NONE', #14088, 2.649999999999985700 ) ;
#32150=LINE ( 'NONE', #61120, #50827 ) ;
#32151=CARTESIAN_POINT ( 'NONE',  ( -97.01659045497900991, 88.39448418669211094, 74.95309847082319266 ) ) ;
#32152=CARTESIAN_POINT ( 'NONE',  ( 96.15314808468748708, 88.00268892867053694, 85.56822916753381492 ) ) ;
#32155=CARTESIAN_POINT ( 'NONE',  ( 93.67500000000001137, -207.7050326799711968, 80.36916666666665776 ) ) ;
#32159=EDGE_LOOP ( 'NONE', ( #67225, #63741, #26384, #7768 ) ) ;
#32162=CARTESIAN_POINT ( 'NONE',  ( -92.69370383062502583, 91.33154071421968467, 84.45697916753383083 ) ) ;
#32171=CARTESIAN_POINT ( 'NONE',  ( -97.64999999999994884, -211.5299782133524502, 86.95729166840096980 ) ) ;
#32172=EDGE_CURVE ( 'NONE', #65748, #9715, #62609, .T. ) ;
#32176=CARTESIAN_POINT ( 'NONE',  ( -96.32500000000001705, 87.70503267997129626, 81.93020833506763267 ) ) ;
#32179=EDGE_CURVE ( 'NONE', #18340, #23470, #26879, .T. ) ;
#32180=CARTESIAN_POINT ( 'NONE',  ( 97.30629616937498838, 91.33154071421968467, 88.26697916753381890 ) ) ;
#32183=CARTESIAN_POINT ( 'NONE',  ( -97.64999999950686060, 89.99996796133669363, 83.73041644179562581 ) ) ;
#32186=VERTEX_POINT ( 'NONE', #56959 ) ;
#32189=ORIENTED_EDGE ( 'NONE', *, *, #24270, .F. ) ;
#32194=CARTESIAN_POINT ( 'NONE',  ( -93.84685191531247028, -211.9973110713294489, 84.29822916753381890 ) ) ;
#32195=VERTEX_POINT ( 'NONE', #28365 ) ;
#32198=ORIENTED_EDGE ( 'NONE', *, *, #68354, .T. ) ;
#32199=AXIS2_PLACEMENT_3D ( 'NONE', #64501, #12976, #35915 ) ;
#32204=CARTESIAN_POINT ( 'NONE',  ( 93.84685191531248449, 88.00268892867053694, 77.68364583420047609 ) ) ;
#32212=CARTESIAN_POINT ( 'NONE',  ( 93.67499999999999716, 87.70503267997126784, 76.85020833506763438 ) ) ;
#32214=CARTESIAN_POINT ( 'NONE',  ( -93.84685191531254134, 91.99731107132950569, 81.81114583420047381 ) ) ;
#32227=ADVANCED_FACE ( 'NONE', ( #10713 ), #62986, .F. ) ;
#32229=CARTESIAN_POINT ( 'NONE',  ( 92.69370383062501162, -208.6684592857803011, 77.68364583420047609 ) ) ;
#32234=FACE_OUTER_BOUND ( 'NONE', #1595, .T. ) ;
#32239=EDGE_CURVE ( 'NONE', #18753, #47168, #45690, .T. ) ;
#32240=CARTESIAN_POINT ( 'NONE',  ( 93.84685191531251292, -211.9973110713294489, 77.84239583420048803 ) ) ;
#32242=AXIS2_PLACEMENT_3D ( 'NONE', #60180, #37239, #71417 ) ;
#32244=FACE_OUTER_BOUND ( 'NONE', #54524, .T. ) ;
#32246=EDGE_CURVE ( 'NONE', #48302, #16851, #66799, .T. ) ;
#32247=EDGE_LOOP ( 'NONE', ( #49370, #74235, #60941, #53665 ) ) ;
#32250=( NAMED_UNIT ( * ) SI_UNIT ( $, .STERADIAN. ) SOLID_ANGLE_UNIT ( ) );
#32255=CARTESIAN_POINT ( 'NONE',  ( 96.32499999999998863, -212.2949673200287179, 80.76604166840097321 ) ) ;
#32256=CARTESIAN_POINT ( 'NONE',  ( 96.32499999999997442, 92.29496732002878900, 86.61333333333332973 ) ) ;
#32259=ADVANCED_FACE ( 'NONE', ( #4349 ), #27632, .F. ) ;
#32263=CARTESIAN_POINT ( 'NONE',  ( -93.84685191531252713, 88.00268892867056536, 84.93322916753382401 ) ) ;
#32264=CARTESIAN_POINT ( 'NONE',  ( 92.69370383062498320, 91.33154071421968467, 82.60489583420047666 ) ) ;
#32267=AXIS2_PLACEMENT_3D ( 'NONE', #64806, #59158, #7648 ) ;
#32284=CARTESIAN_POINT ( 'NONE',  ( -92.69370383062498320, -208.6684592857803011, 79.85322916753379729 ) ) ;
#32290=CARTESIAN_POINT ( 'NONE',  ( 96.32499999999998863, -207.7050326799711968, 83.51770833506763836 ) ) ;
#32292=CARTESIAN_POINT ( 'NONE',  ( 94.99999999999998579, 87.33691857156068750, 87.26156250086714294 ) ) ;
#32295=CARTESIAN_POINT ( 'NONE',  ( 92.35000000000000853, -209.9999999999999716, 88.09499999999999886 ) ) ;
#32299=CARTESIAN_POINT ( 'NONE',  ( -92.35000000000005116, 88.47002178664754979, 87.80395833506766223 ) ) ;
#32300=( BOUNDED_CURVE ( )  B_SPLINE_CURVE ( 2, ( #39713, #45735, #50600, #48834, #27676, #50979, #10759, #38965, #22410 ),
 .UNSPECIFIED., .F., .F. ) 
 B_SPLINE_CURVE_WITH_KNOTS ( ( 3, 2, 2, 2, 3 ),
 ( 0.4445132602971387792, 0.4515689946164713753, 0.4586247601573538724, 0.4656805256982363139, 0.4656806970056963091 ),
 .UNSPECIFIED. ) 
 CURVE ( )  GEOMETRIC_REPRESENTATION_ITEM ( )  RATIONAL_B_SPLINE_CURVE ( ( 0.9999988143381453032, 0.8660259966179892910, 1.000000000000000000, 0.8660254037844387076, 1.000000000000000000, 0.8660254037844387076, 1.000000000000000000, 0.9999967472207444974, 0.9999934945994379820 ) ) 
 REPRESENTATION_ITEM ( '' )  );
#32303=CARTESIAN_POINT ( 'NONE',  ( 92.35000000006144205, 90.00001182178868930, 76.10900611559256390 ) ) ;
#32309=DIRECTION ( 'NONE',  ( -1.000000000000000000, 3.061616997868383141E-16, -0.000000000000000000 ) ) ;
#32311=EDGE_CURVE ( 'NONE', #17108, #56237, #25502, .T. ) ;
#32312=DIRECTION ( 'NONE',  ( -0.000000000000000000, -0.000000000000000000, 1.000000000000000000 ) ) ;
#32313=CARTESIAN_POINT ( 'NONE',  ( -97.64999999999996305, -209.9999999999999716, 88.73000000000000398 ) ) ;
#32318=CARTESIAN_POINT ( 'NONE',  ( -97.30629616937495996, -209.9999999999999716, 89.64281250086713726 ) ) ;
#32325=ORIENTED_EDGE ( 'NONE', *, *, #53911, .T. ) ;
#32332=CARTESIAN_POINT ( 'NONE',  ( 93.84685191531251292, -211.9973110713294489, 82.76364583420047438 ) ) ;
#32333=CARTESIAN_POINT ( 'NONE',  ( 92.69370383062501162, -209.9999999999999716, 84.72156250086715090 ) ) ;
#32336=CARTESIAN_POINT ( 'NONE',  ( 92.69370383062501162, -209.9999999999999716, 87.26156250086715715 ) ) ;
#32342=CARTESIAN_POINT ( 'NONE',  ( -92.69370383062502583, 88.66845928578038638, 78.00114583420049996 ) ) ;
#32343=ORIENTED_EDGE ( 'NONE', *, *, #6809, .F. ) ;
#32344=VERTEX_POINT ( 'NONE', #70062 ) ;
#32360=CARTESIAN_POINT ( 'NONE',  ( 93.84685191531251292, -211.9973110713294489, 76.41364583420048007 ) ) ;
#32362=FACE_BOUND ( 'NONE', #71344, .T. ) ;
#32367=FACE_OUTER_BOUND ( 'NONE', #19498, .T. ) ;
#32369=CARTESIAN_POINT ( 'NONE',  ( -96.15314808468751551, 88.00268892867056536, 79.74739583420048916 ) ) ;
#32371=CARTESIAN_POINT ( 'NONE',  ( 93.84685191531248449, 88.00268892867053694, 77.04864583420047097 ) ) ;
#32374=CARTESIAN_POINT ( 'NONE',  ( -96.15314808468747287, -208.0026889286704943, 88.26697916753380468 ) ) ;
#32378=CARTESIAN_POINT ( 'NONE',  ( -94.99999999999997158, -207.3369185715606307, 79.95906250086713385 ) ) ;
#32383=VERTEX_POINT ( 'NONE', #63714 ) ;
#32391=CARTESIAN_POINT ( 'NONE',  ( 93.98225765065697601, -207.8046129959941197, 74.85985921673515975 ) ) ;
#32392=CARTESIAN_POINT ( 'NONE',  ( -96.15314808468751551, 88.00268892867056536, 83.39864583420047950 ) ) ;
#32402=CARTESIAN_POINT ( 'NONE',  ( -93.84685191531247028, -211.9973110713294489, 84.29822916753381890 ) ) ;
#32404=CARTESIAN_POINT ( 'NONE',  ( -97.64999999996709334, -209.9999916080759306, 86.90410584369134028 ) ) ;
#32411=VERTEX_POINT ( 'NONE', #28738 ) ;
#32412=CARTESIAN_POINT ( 'NONE',  ( 97.64999999999689351, 89.99999595380309358, 77.06187486178042434 ) ) ;
#32429=EDGE_LOOP ( 'NONE', ( #23397, #28848, #25084, #34706 ) ) ;
#32439=VERTEX_POINT ( 'NONE', #20040 ) ;
#32442=VERTEX_POINT ( 'NONE', #9133 ) ;
#32444=CARTESIAN_POINT ( 'NONE',  ( 93.84685191531248449, 91.99731107132950569, 75.72572916753382799 ) ) ;
#32447=ORIENTED_EDGE ( 'NONE', *, *, #43635, .F. ) ;
#32450=CARTESIAN_POINT ( 'NONE',  ( 96.15314808468748708, 88.00268892867053694, 87.31447916753380412 ) ) ;
#32452=CARTESIAN_POINT ( 'NONE',  ( 96.15314808468748708, -208.0026889286704943, 88.16114583420046813 ) ) ;
#32454=CARTESIAN_POINT ( 'NONE',  ( -92.35000000000005116, 91.52997821335253548, 77.11479166840095445 ) ) ;
#32457=CARTESIAN_POINT ( 'NONE',  ( -97.64999999999996305, -209.9999999999999716, 83.01499999999998636 ) ) ;
#32459=CARTESIAN_POINT ( 'NONE',  ( -93.67499999999998295, -207.7050326799711968, 75.26270833506764291 ) ) ;
#32460=CARTESIAN_POINT ( 'NONE',  ( -93.84685191531252713, 88.00268892867056536, 89.37822916753381719 ) ) ;
#32461=ORIENTED_EDGE ( 'NONE', *, *, #30383, .T. ) ;
#32463=CARTESIAN_POINT ( 'NONE',  ( 94.99999999999998579, 92.66308142843935514, 88.84906250086713442 ) ) ;
#32464=CARTESIAN_POINT ( 'NONE',  ( -96.15314808468751551, 88.00268892867056536, 86.57364583420047666 ) ) ;
#32469=DIRECTION ( 'NONE',  ( -0.000000000000000000, -0.000000000000000000, 1.000000000000000000 ) ) ;
#32478=B_SPLINE_CURVE_WITH_KNOTS ( 'NONE', 3,
 ( #36474, #14656, #7910, #47402, #48868, #71052 ),
 .UNSPECIFIED., .F., .F.,
 ( 4, 2, 4 ),
 ( 0.7528176110416423539, 0.8153862273022710605, 0.8779548435628997671 ),
 .UNSPECIFIED. ) ;
#32479=CARTESIAN_POINT ( 'NONE',  ( -97.65000000000001990, 90.00000000000004263, 82.37999999999999545 ) ) ;
#32482=CARTESIAN_POINT ( 'NONE',  ( 92.35000000000000853, -209.9999999999999716, 88.17437500173430465 ) ) ;
#32483=ADVANCED_FACE ( 'NONE', ( #54276, #20425, #8408 ), #53899, .F. ) ;
#32488=CARTESIAN_POINT ( 'NONE',  ( -95.00000000000002842, 87.33691857156074434, 81.54656250086715374 ) ) ;
#32491=CARTESIAN_POINT ( 'NONE',  ( 97.64999999997402824, 89.99998827382246702, 82.77687459617033028 ) ) ;
#32495=CARTESIAN_POINT ( 'NONE',  ( -95.00000000000002842, 93.05995642670504253, 79.04624999999997215 ) ) ;
#32498=CARTESIAN_POINT ( 'NONE',  ( -95.00000000000002842, 93.05995642670504253, 82.22124999999999773 ) ) ;
#32505=CARTESIAN_POINT ( 'NONE',  ( 96.15314808468748708, 91.99731107132950569, 81.96989583420048575 ) ) ;
#32506=CARTESIAN_POINT ( 'NONE',  ( -93.84685191531248449, -208.0026889286704943, 83.23989583420049598 ) ) ;
#32509=LINE ( 'NONE', #14482, #5305 ) ;
#32510=CARTESIAN_POINT ( 'NONE',  ( -96.32499999999996021, -212.2949673200287179, 77.40583333333331950 ) ) ;
#32512=CARTESIAN_POINT ( 'NONE',  ( -96.15314808468751551, 88.00268892867056536, 79.11239583420048405 ) ) ;
#32513=CARTESIAN_POINT ( 'NONE',  ( 95.00000000000000000, -212.6630814284392557, 82.18156250086714465 ) ) ;
#32517=EDGE_LOOP ( 'NONE', ( #65671, #17286, #68154, #42242 ) ) ;
#32526=CARTESIAN_POINT ( 'NONE',  ( 96.66079198124941740, -211.6002412367799934, 74.80065669543249385 ) ) ;
#32530=( BOUNDED_CURVE ( )  B_SPLINE_CURVE ( 2, ( #26833, #50879, #49759, #27580, #67435, #50120, #32836, #56911, #55787, #39615, #4306, #15930, #33210, #56155, #72681, #21182, #73804, #15184, #4673, #38119, #62557, #61057, #73436, #39243, #44886, #62173, #22317, #11040, #45260, #33963, #46733, #1287, #11399, #29060, #52738, #63666, #6154, #12507, #18151, #34332, #23431, #6512, #23070, #35444, #57273, #51627, #58373, #24173, #5780, #62940, #34700, #51987, #45998, #28686, #17776, #22697, #30164, #45643, #178, #64398, #535, #68926, #47107, #17415, #29785, #40348, #29412, #46362, #69290, #63293, #35798, #57652, #18514, #11753, #40722, #12135, #35078, #58008, #52360, #6872, #7252, #907, #70012, #23793, #69658, #41099, #17049, #41456, #64031, #12868, #58754, #53110, #68561, #39984, #59490, #7981, #1647, #18880, #43331, #8726, #37311, #54587, #66248, #59127, #9087, #30898, #14361, #36543, #26006, #25282, #13251, #42208, #60246, #70750, #71119, #37674, #2389, #24901, #48931, #53842, #48206, #7614, #32010, #31642, #24533, #47469, #36920, #30528, #13616, #54226, #3112, #14724, #19623, #48577, #65877, #2014, #59868, #60608, #70375, #71489, #8355, #53478, #71855, #20371, #41819, #19257, #42569, #64765, #47829, #25641, #65509, #65143, #36179, #13976, #31277, #2757, #19989, #42944, #43689, #61347, #10564, #67345, #38032, #56066, #44050, #10950, #44424, #38775, #55321, #67719, #66609, #9454, #16209, #33486, #15090, #20738, #66966, #38406, #3839, #60962, #50034, #62469, #54950, #32378, #22225, #9826, #49305, #61711, #39149, #16583, #21093, #56449, #26739, #4582, #72591, #3471, #15845, #10196, #33118, #73713, #62088, #32744, #49667, #15462, #4958, #39526, #55695, #27481, #4211, #50416, #45167, #27102, #72961, #21463, #21849, #73342, #26375, #44797, #27858, #50786, #68092, #72231, #51157, #1197, #41011, #69569, #52275, #45915, #40634, #11311, #35365, #6783, #29697, #28227, #34244, #41374, #34993, #450, #46641, #28975, #52646, #34610, #57188, #58289, #63209, #57560, #74091, #5693, #28595, #6431, #51907, #6069, #12051, #92, #24093, #62851, #5329, #23347, #68472, #18429, #63574, #17696, #69927, #64310, #29331, #57928, #63944, #18068, #47017, #68841, #33875, #51536, #17328, #40260, #11670, #39900, #22984, #12421, #56821, #46274, #819, #16963, #23705 ),
 .UNSPECIFIED., .F., .F. ) 
 B_SPLINE_CURVE_WITH_KNOTS ( ( 3, 2, 2, 2, 2, 2, 2, 2, 2, 2, 2, 2, 2, 2, 2, 2, 2, 2, 2, 2, 2, 2, 2, 2, 2, 2, 2, 2, 2, 2, 2, 2, 2, 2, 2, 2, 2, 2, 2, 2, 2, 2, 2, 2, 2, 2, 2, 2, 2, 2, 2, 2, 2, 2, 2, 2, 2, 2, 2, 2, 2, 2, 2, 2, 2, 2, 2, 2, 2, 2, 2, 2, 2, 2, 2, 2, 2, 2, 2, 2, 2, 2, 2, 2, 2, 2, 2, 2, 2, 2, 2, 2, 2, 2, 2, 2, 2, 2, 2, 2, 2, 2, 2, 2, 2, 2, 2, 2, 2, 2, 2, 2, 2, 2, 2, 2, 2, 2, 2, 2, 2, 2, 2, 2, 2, 2, 2, 2, 2, 2, 2, 2, 2, 2, 2, 2, 2, 2, 2, 2, 2, 3 ),
 ( 0.000000000000000000, 0.007055765384978172905, 0.01411153076995634581, 0.02116729615493451871, 0.02822306153991269162, 0.03527882692489087146, 0.04233459230986903743, 0.04939035769484721727, 0.05644612307982538324, 0.06350188846480356308, 0.07055765384978174293, 0.07761341923475992277, 0.08466918461973807486, 0.09172495000471626858, 0.09878071538969443455, 0.1058364807746726144, 0.1128922461596507665, 0.1199480115446289602, 0.1270037769296071262, 0.1340595423145853060, 0.1411153076995634859, 0.1481710730845416657, 0.1552268384695198455, 0.1622826038544979699, 0.1693383692394761497, 0.1763941346244543296, 0.1834499000094325372, 0.1905056653944106893, 0.1975614307793888691, 0.2046171961643670489, 0.2116729615493452288, 0.2187287269343233809, 0.2257844923193015330, 0.2328402577042797406, 0.2398960230892579204, 0.2469517884742360725, 0.2540075538592142523, 0.2610633192441924044, 0.2681190846291706120, 0.2751748500141487641, 0.2822306153991269717, 0.2892863807841050683, 0.2963421461690833314, 0.3033979115540614280, 0.3104536769390396911, 0.3175094423240178432, 0.3245652077089959398, 0.3316209730939742029, 0.3386767384789522994, 0.3457325038639305625, 0.3527882692489086591, 0.3598440346338868667, 0.3668998000188650743, 0.3739555654038432264, 0.3810113307888213785, 0.3880670961737995306, 0.3951228615587777382, 0.4021786269437558903, 0.4092343923287340979, 0.4162901577137122500, 0.4233459230986904576, 0.4304016884836686097, 0.4374574538686467617, 0.4445132192536249693, 0.4515689846386030659, 0.4586247500235813290, 0.4656805154085594811, 0.4727362807935376332, 0.4797920461785158408, 0.4868478115634939929, 0.4939035769484721450, 0.5009593423334502971, 0.5080151077184285047, 0.5150708731034067123, 0.5221266384883848088, 0.5291824038733630164, 0.5362381692583412240, 0.5432939346433194316, 0.5503497000282975282, 0.5574054654132757358, 0.5644612307982539434, 0.5715169961832320400, 0.5785727615682101366, 0.5856285269531884552, 0.5926842923381666628, 0.5997400577231447594, 0.6067958231081228559, 0.6138515884931010635, 0.6209073538780793822, 0.6279631192630574787, 0.6350188846480356863, 0.6420746500330137829, 0.6491304154179918795, 0.6561861808029701981, 0.6632419461879484057, 0.6702977115729265023, 0.6773534769579045989, 0.6844092423428829175, 0.6914650077278611251, 0.6985207731128392217, 0.7055765384978173183, 0.7126323038827955259, 0.7196880692677737335, 0.7267438346527518300, 0.7337996000377301486, 0.7408553654227082452, 0.7479111308076864528, 0.7549668961926645494, 0.7620226615776427570, 0.7690784269626209646, 0.7761341923475990612, 0.7831899577325773798, 0.7902457231175554764, 0.7973014885025335730, 0.8043572538875117806, 0.8114130192724900992, 0.8184687846574681958, 0.8255245500424462923, 0.8325803154274244999, 0.8396360808124025965, 0.8466918461973809151, 0.8537476115823590117, 0.8608033769673372193, 0.8678591423523153159, 0.8749149077372935235, 0.8819706731222718421, 0.8890264385072499387, 0.8960822038922280353, 0.9031379692772061318, 0.9101937346621844505, 0.9172495000471626581, 0.9243052654321407546, 0.9313610308171189622, 0.9384167962020971698, 0.9454725615870752664, 0.9525283269720534740, 0.9595840923570316816, 0.9666398577420097782, 0.9736956231269879858, 0.9807513885119661934, 0.9878071538969442900, 0.9900635123082156541 ),
 .UNSPECIFIED. ) 
 CURVE ( )  GEOMETRIC_REPRESENTATION_ITEM ( )  RATIONAL_B_SPLINE_CURVE ( ( 1.000000000000000000, 0.8660254037844387076, 1.000000000000000000, 0.8660254037844387076, 1.000000000000000000, 0.8660254037844387076, 1.000000000000000000, 0.8660254037844387076, 1.000000000000000000, 0.8660254037844387076, 1.000000000000000000, 0.8660254037844387076, 1.000000000000000000, 0.8660254037844387076, 1.000000000000000000, 0.8660254037844387076, 1.000000000000000000, 0.8660254037844387076, 1.000000000000000000, 0.8660254037844387076, 1.000000000000000000, 0.8660254037844387076, 1.000000000000000000, 0.8660254037844387076, 1.000000000000000000, 0.8660254037844387076, 1.000000000000000000, 0.8660254037844387076, 1.000000000000000000, 0.8660254037844387076, 1.000000000000000000, 0.8660254037844387076, 1.000000000000000000, 0.8660254037844387076, 1.000000000000000000, 0.8660254037844387076, 1.000000000000000000, 0.8660254037844387076, 1.000000000000000000, 0.8660254037844387076, 1.000000000000000000, 0.8660254037844387076, 1.000000000000000000, 0.8660254037844387076, 1.000000000000000000, 0.8660254037844387076, 1.000000000000000000, 0.8660254037844387076, 1.000000000000000000, 0.8660254037844387076, 1.000000000000000000, 0.8660254037844387076, 1.000000000000000000, 0.8660254037844387076, 1.000000000000000000, 0.8660254037844387076, 1.000000000000000000, 0.8660254037844387076, 1.000000000000000000, 0.8660254037844387076, 1.000000000000000000, 0.8660254037844387076, 1.000000000000000000, 0.8660254037844387076, 1.000000000000000000, 0.8660254037844387076, 1.000000000000000000, 0.8660254037844387076, 1.000000000000000000, 0.8660254037844387076, 1.000000000000000000, 0.8660254037844387076, 1.000000000000000000, 0.8660254037844387076, 1.000000000000000000, 0.8660254037844387076, 1.000000000000000000, 0.8660254037844387076, 1.000000000000000000, 0.8660254037844387076, 1.000000000000000000, 0.8660254037844387076, 1.000000000000000000, 0.8660254037844387076, 1.000000000000000000, 0.8660254037844387076, 1.000000000000000000, 0.8660254037844387076, 1.000000000000000000, 0.8660254037844387076, 1.000000000000000000, 0.8660254037844387076, 1.000000000000000000, 0.8660254037844387076, 1.000000000000000000, 0.8660254037844387076, 1.000000000000000000, 0.8660254037844387076, 1.000000000000000000, 0.8660254037844387076, 1.000000000000000000, 0.8660254037844387076, 1.000000000000000000, 0.8660254037844387076, 1.000000000000000000, 0.8660254037844387076, 1.000000000000000000, 0.8660254037844387076, 1.000000000000000000, 0.8660254037844387076, 1.000000000000000000, 0.8660254037844387076, 1.000000000000000000, 0.8660254037844387076, 1.000000000000000000, 0.8660254037844387076, 1.000000000000000000, 0.8660254037844387076, 1.000000000000000000, 0.8660254037844387076, 1.000000000000000000, 0.8660254037844387076, 1.000000000000000000, 0.8660254037844387076, 1.000000000000000000, 0.8660254037844387076, 1.000000000000000000, 0.8660254037844387076, 1.000000000000000000, 0.8660254037844387076, 1.000000000000000000, 0.8660254037844387076, 1.000000000000000000, 0.8660254037844387076, 1.000000000000000000, 0.8660254037844387076, 1.000000000000000000, 0.8660254037844387076, 1.000000000000000000, 0.8660254037844387076, 1.000000000000000000, 0.8660254037844387076, 1.000000000000000000, 0.8660254037844387076, 1.000000000000000000, 0.8660254037844387076, 1.000000000000000000, 0.8660254037844387076, 1.000000000000000000, 0.8660254037844387076, 1.000000000000000000, 0.8660254037844387076, 1.000000000000000000, 0.8660254037844387076, 1.000000000000000000, 0.8660254037844387076, 1.000000000000000000, 0.8660254037844387076, 1.000000000000000000, 0.8660254037844387076, 1.000000000000000000, 0.8660254037844387076, 1.000000000000000000, 0.8660254037844387076, 1.000000000000000000, 0.8660254037844387076, 1.000000000000000000, 0.8660254037844387076, 1.000000000000000000, 0.8660254037844387076, 1.000000000000000000, 0.8660254037844387076, 1.000000000000000000, 0.8660254037844387076, 1.000000000000000000, 0.8660254037844387076, 1.000000000000000000, 0.8660254037844387076, 1.000000000000000000, 0.8660254037844387076, 1.000000000000000000, 0.8660254037844387076, 1.000000000000000000, 0.8660254037844387076, 1.000000000000000000, 0.8660254037844387076, 1.000000000000000000, 0.8660254037844387076, 1.000000000000000000, 0.8660254037844387076, 1.000000000000000000, 0.8660254037844387076, 1.000000000000000000, 0.8660254037844387076, 1.000000000000000000, 0.8660254037844387076, 1.000000000000000000, 0.8660254037844387076, 1.000000000000000000, 0.8660254037844387076, 1.000000000000000000, 0.8660254037844387076, 1.000000000000000000, 0.8660254037844387076, 1.000000000000000000, 0.8660254037844387076, 1.000000000000000000, 0.8660254037844387076, 1.000000000000000000, 0.8660254037844387076, 1.000000000000000000, 0.8660254037844387076, 1.000000000000000000, 0.8660254037844387076, 1.000000000000000000, 0.8660254037844387076, 1.000000000000000000, 0.8660254037844387076, 1.000000000000000000, 0.8660254037844387076, 1.000000000000000000, 0.8660254037844387076, 1.000000000000000000, 0.8660254037844387076, 1.000000000000000000, 0.8660254037844387076, 1.000000000000000000, 0.8660254037844387076, 1.000000000000000000, 0.8660254037844387076, 1.000000000000000000, 0.8660254037844387076, 1.000000000000000000, 0.8660254037844387076, 1.000000000000000000, 0.8660254037844387076, 1.000000000000000000, 0.8660254037844387076, 1.000000000000000000, 0.8660254037844387076, 1.000000000000000000, 0.8660254037844387076, 1.000000000000000000, 0.8660254037844387076, 1.000000000000000000, 0.8660254037844387076, 1.000000000000000000, 0.8660254037844387076, 1.000000000000000000, 0.8660254037844387076, 1.000000000000000000, 0.8660254037844387076, 1.000000000000000000, 0.8660254037844387076, 1.000000000000000000, 0.8660254037844387076, 1.000000000000000000, 0.8660254037844387076, 1.000000000000000000, 0.8660254037844387076, 1.000000000000000000, 0.8660254037844387076, 1.000000000000000000, 0.8660254037844387076, 1.000000000000000000, 0.8660254037844387076, 1.000000000000000000, 0.8660254037844387076, 1.000000000000000000, 0.8660254037844387076, 1.000000000000000000, 0.8660254037844387076, 1.000000000000000000, 0.8660254037844387076, 1.000000000000000000, 0.8660254037844387076, 1.000000000000000000, 0.8660254037844387076, 1.000000000000000000, 0.8660254037844387076, 1.000000000000000000, 0.9571563550410487897, 0.9417145902178700734 ) ) 
 REPRESENTATION_ITEM ( '' )  );
#32531=CARTESIAN_POINT ( 'NONE',  ( 93.84685191531248449, 91.99731107132950569, 87.15572916753382060 ) ) ;
#32532=CARTESIAN_POINT ( 'NONE',  ( 96.32499999999998863, 87.70503267997126784, 75.05104166840095559 ) ) ;
#32533=CARTESIAN_POINT ( 'NONE',  ( 93.67500000000001137, -212.2949673200287179, 83.12083333333332291 ) ) ;
#32542=CARTESIAN_POINT ( 'NONE',  ( 92.35000000001610942, 89.99999393654047708, 88.17456390440148084 ) ) ;
#32547=CARTESIAN_POINT ( 'NONE',  ( -97.64999999999994884, -208.4700217866474645, 86.85145833506763324 ) ) ;
#32551=CARTESIAN_POINT ( 'NONE',  ( -92.35000000000003695, 90.00000000000004263, 84.04687500173430692 ) ) ;
#32554=CARTESIAN_POINT ( 'NONE',  ( 92.69370383062498320, 88.66845928578037217, 82.23447916753383424 ) ) ;
#32560=CARTESIAN_POINT ( 'NONE',  ( 92.35000000001610942, 89.99999393654047708, 88.17456390440148084 ) ) ;
#32571=CARTESIAN_POINT ( 'NONE',  ( -93.84685191531248449, -208.0026889286704943, 84.50989583420049200 ) ) ;
#32583=CARTESIAN_POINT ( 'NONE',  ( 94.99999999999998579, 87.33691857156068750, 78.37156250086714238 ) ) ;
#32587=DIRECTION ( 'NONE',  ( 1.000000000000000000, 0.000000000000000000, 0.000000000000000000 ) ) ;
#32593=LINE ( 'NONE', #20586, #36033 ) ;
#32595=CARTESIAN_POINT ( 'NONE',  ( 92.34999999999999432, 90.00000000000002842, 76.74437500173429783 ) ) ;
#32597=CARTESIAN_POINT ( 'NONE',  ( -95.00000000000002842, 87.33691857156074434, 83.45156250086714067 ) ) ;
#32609=CARTESIAN_POINT ( 'NONE',  ( 92.35004028547584198, 88.46999852781718232, 83.14729327728632313 ) ) ;
#32610=CARTESIAN_POINT ( 'NONE',  ( 92.69370383062501162, -211.3315407142195852, 77.78947916753381264 ) ) ;
#32617=CARTESIAN_POINT ( 'NONE',  ( 97.30629616937498838, -209.9999999999999716, 77.41906250086715602 ) ) ;
#32620=DIRECTION ( 'NONE',  ( 0.000000000000000000, -1.000000000000000000, 0.000000000000000000 ) ) ;
#32629=CARTESIAN_POINT ( 'NONE',  ( 95.00000000000000000, -213.0599564267049857, 81.34812500173430294 ) ) ;
#32630=CARTESIAN_POINT ( 'NONE',  ( 92.34999999999999432, 91.52997821335252127, 80.42208333333331893 ) ) ;
#32635=CARTESIAN_POINT ( 'NONE',  ( -92.69370383062498320, -210.0000000000000568, 74.79348190356851944 ) ) ;
#32638=CARTESIAN_POINT ( 'NONE',  ( -96.15314808468751551, 88.00268892867056536, 85.46239583420047836 ) ) ;
#32639=CARTESIAN_POINT ( 'NONE',  ( 93.84685191531248449, 91.99731107132950569, 81.91697916753381037 ) ) ;
#32644=ORIENTED_EDGE ( 'NONE', *, *, #24969, .T. ) ;
#32646=AXIS2_PLACEMENT_3D ( 'NONE', #57565, #51540, #11671 ) ;
#32651=CARTESIAN_POINT ( 'NONE',  ( 97.64999999999999147, 89.99999999755287661, 75.15687493081163950 ) ) ;
#32656=VERTEX_POINT ( 'NONE', #21518 ) ;
#32657=CARTESIAN_POINT ( 'NONE',  ( -94.26819495033781493, -212.6374485842881938, 75.02735117824597921 ) ) ;
#32658=CARTESIAN_POINT ( 'NONE',  ( -97.30629616937497417, -208.6684592857803011, 80.06489583420047040 ) ) ;
#32661=DIRECTION ( 'NONE',  ( -0.000000000000000000, -0.000000000000000000, -1.000000000000000000 ) ) ;
#32664=EDGE_CURVE ( 'NONE', #58390, #8233, #10136, .T. ) ;
#32667=CARTESIAN_POINT ( 'NONE',  ( 97.30629616937498838, 90.00000000000002842, 89.32531250086714181 ) ) ;
#32680=CARTESIAN_POINT ( 'NONE',  ( -97.64999999999996305, -209.9999999999999716, 83.65000000000000568 ) ) ;
#32682=CARTESIAN_POINT ( 'NONE',  ( 97.64999999999999147, -210.0000000334413244, 87.85687500050293863 ) ) ;
#32692=CARTESIAN_POINT ( 'NONE',  ( 96.15314808468750130, -211.9973110713294489, 88.10822916753382117 ) ) ;
#32698=CARTESIAN_POINT ( 'NONE',  ( 96.15314808468750130, -211.9973110713294489, 80.96447916753380980 ) ) ;
#32699=CARTESIAN_POINT ( 'NONE',  ( 95.00000000000000000, -207.3369185715606307, 84.56281250086716739 ) ) ;
#32701=CARTESIAN_POINT ( 'NONE',  ( 96.15314808468748708, -208.0026889286704943, 85.77989583420048803 ) ) ;
#32709=VERTEX_POINT ( 'NONE', #44477 ) ;
#32727=ORIENTED_EDGE ( 'NONE', *, *, #44819, .F. ) ;
#32728=VERTEX_POINT ( 'NONE', #38827 ) ;
#32732=CARTESIAN_POINT ( 'NONE',  ( -92.35000000000003695, 90.00000000000004263, 89.68250000000000455 ) ) ;
#32734=CARTESIAN_POINT ( 'NONE',  ( 92.69370383062498320, 91.33154071421968467, 76.88989583420047325 ) ) ;
#32736=( BOUNDED_CURVE ( )  B_SPLINE_CURVE ( 2, ( #48953, #71883, #54611, #3135, #65532, #42592, #20012 ),
 .UNSPECIFIED., .F., .F. ) 
 B_SPLINE_CURVE_WITH_KNOTS ( ( 3, 2, 2, 3 ),
 ( 0.2291666666666663521, 0.2361111111111107719, 0.2430555555555551639, 0.2499999999999995837 ),
 .UNSPECIFIED. ) 
 CURVE ( )  GEOMETRIC_REPRESENTATION_ITEM ( )  RATIONAL_B_SPLINE_CURVE ( ( 1.000000000000005995, 0.8660254037844328234, 1.000000000000000000, 0.8660254037844387076, 1.000000000000000000, 0.8660254037844467012, 0.9999999999999920064 ) ) 
 REPRESENTATION_ITEM ( '' )  );
#32739=CARTESIAN_POINT ( 'NONE',  ( -94.99999999999997158, -212.6630814284392557, 89.16656250086712987 ) ) ;
#32740=VERTEX_POINT ( 'NONE', #73392 ) ;
#32742=CARTESIAN_POINT ( 'NONE',  ( -92.34999999999999432, -209.9999999999999716, 90.00000000000000000 ) ) ;
#32744=CARTESIAN_POINT ( 'NONE',  ( -94.99999999999997158, -212.6630814284392557, 79.00656250086714749 ) ) ;
#32748=VECTOR ( 'NONE', #13165, 1000.000000000000000 ) ;
#32753=DIRECTION ( 'NONE',  ( -1.000000000000000000, 3.061616997868383141E-16, -0.000000000000000000 ) ) ;
#32755=CARTESIAN_POINT ( 'NONE',  ( 96.58546442478372285, -208.2943803060620667, 74.79912739178800507 ) ) ;
#32756=CARTESIAN_POINT ( 'NONE',  ( -93.84685191531254134, 91.99731107132950569, 80.54114583420046358 ) ) ;
#32767=CARTESIAN_POINT ( 'NONE',  ( -93.67500000000003979, 92.29496732002878900, 89.78833333333332689 ) ) ;
#32768=CARTESIAN_POINT ( 'NONE',  ( -94.99999999999997158, -209.9999999999999716, 90.00000000000000000 ) ) ;
#32769=CARTESIAN_POINT ( 'NONE',  ( -93.84685191531248449, -208.0026889286704943, 78.15989583420049769 ) ) ;
#32770=CARTESIAN_POINT ( 'NONE',  ( 92.35000000006144205, 90.00001182178868930, 76.10900611559256390 ) ) ;
#32771=EDGE_CURVE ( 'NONE', #74080, #55829, #28816, .T. ) ;
#32805=CARTESIAN_POINT ( 'NONE',  ( 96.15314808468748708, 91.99731107132950569, 74.98489583420048632 ) ) ;
#32809=ORIENTED_EDGE ( 'NONE', *, *, #57740, .T. ) ;
#32811=ORIENTED_EDGE ( 'NONE', *, *, #7066, .T. ) ;
#32812=CARTESIAN_POINT ( 'NONE',  ( 96.15314808468748708, 91.99731107132950569, 87.52614583420047722 ) ) ;
#32814=CARTESIAN_POINT ( 'NONE',  ( 93.84685191531251292, -211.9973110713294489, 84.03364583420047040 ) ) ;
#32816=CARTESIAN_POINT ( 'NONE',  ( -95.00000000000002842, 90.00000000000004263, 90.00000000000000000 ) ) ;
#32818=CARTESIAN_POINT ( 'NONE',  ( -92.35000000000312070, 89.99999595380251094, 77.06187486178039592 ) ) ;
#32823=CARTESIAN_POINT ( 'NONE',  ( 94.99999999999998579, 86.94004357329502852, 85.15812500173429100 ) ) ;
#32825=CARTESIAN_POINT ( 'NONE',  ( -92.69370383062498320, -211.3315407142195852, 87.36739583420047950 ) ) ;
#32826=CARTESIAN_POINT ( 'NONE',  ( -92.69370383062504004, 90.00000000000004263, 84.40406250086715545 ) ) ;
#32829=CARTESIAN_POINT ( 'NONE',  ( 94.99999999999998579, 92.66308142843935514, 86.94406250086714749 ) ) ;
#32830=CARTESIAN_POINT ( 'NONE',  ( -96.15314808468752972, 91.99731107132950569, 89.53697916753381492 ) ) ;
#32835=DIRECTION ( 'NONE',  ( 1.000000000000000000, 0.000000000000000000, 0.000000000000000000 ) ) ;
#32836=CARTESIAN_POINT ( 'NONE',  ( -92.69370383062498320, -209.9999999999999716, 89.32531250086714181 ) ) ;
#32844=EDGE_LOOP ( 'NONE', ( #21658, #73874, #73216, #49461 ) ) ;
#32846=CARTESIAN_POINT ( 'NONE',  ( -92.35000000000003695, 90.00000000000004263, 82.69749999999999091 ) ) ;
#32851=CARTESIAN_POINT ( 'NONE',  ( 92.35003236756685396, 91.52999690077596995, 87.48645704240065868 ) ) ;
#32852=CARTESIAN_POINT ( 'NONE',  ( -92.35000000000005116, 88.47002178664754979, 86.53395833506763779 ) ) ;
#32856=CARTESIAN_POINT ( 'NONE',  ( -97.30629616937501680, 90.00000000000004263, 83.29281250086714294 ) ) ;
#32861=FACE_OUTER_BOUND ( 'NONE', #47445, .T. ) ;
#32867=CARTESIAN_POINT ( 'NONE',  ( 92.69370383062498320, 90.00000000000002842, 79.00656250086716170 ) ) ;
#32869=CARTESIAN_POINT ( 'NONE',  ( -94.99999999999997158, -212.6630814284392557, 81.70531250086715147 ) ) ;
#32870=CYLINDRICAL_SURFACE ( 'NONE', #44591, 2.649999999999999467 ) ;
#32872=CARTESIAN_POINT ( 'NONE',  ( -97.65000000000001990, 89.99996511148930267, 83.09437620840749616 ) ) ;
#32873=CARTESIAN_POINT ( 'NONE',  ( -93.67499999999998295, -212.2949673200287179, 78.14666666666667538 ) ) ;
#32874=CARTESIAN_POINT ( 'NONE',  ( -92.69370383062504004, 90.00000000000004263, 79.32406250086715715 ) ) ;
#32875=CARTESIAN_POINT ( 'NONE',  ( 97.30629616937498838, -208.6684592857803011, 81.12322916753382174 ) ) ;
#32884=ORIENTED_EDGE ( 'NONE', *, *, #70802, .T. ) ;
#32885=ORIENTED_EDGE ( 'NONE', *, *, #46782, .F. ) ;
#32892=CARTESIAN_POINT ( 'NONE',  ( 94.99999999999998579, 92.66308142843935514, 87.10281250086715943 ) ) ;
#32895=CARTESIAN_POINT ( 'NONE',  ( 96.32499999999998863, -212.2949673200287179, 76.87666666666666515 ) ) ;
#32906=CARTESIAN_POINT ( 'NONE',  ( 96.32499999999998863, -212.2949673200287179, 82.67104166840096013 ) ) ;
#32911=CARTESIAN_POINT ( 'NONE',  ( -92.34999999999999432, -211.5299782133524502, 81.45395833506763950 ) ) ;
#32912=ORIENTED_EDGE ( 'NONE', *, *, #47115, .T. ) ;
#32916=CARTESIAN_POINT ( 'NONE',  ( -95.00000000000002842, 86.94004357329504273, 81.98312500173430806 ) ) ;
#32919=CARTESIAN_POINT ( 'NONE',  ( 97.30629616937498838, 88.66845928578037217, 83.71614583420050337 ) ) ;
#32921=CARTESIAN_POINT ( 'NONE',  ( -92.35000677009857384, -211.5299821220706917, 82.72395806468945523 ) ) ;
#32925=CARTESIAN_POINT ( 'NONE',  ( 97.65000000000000568, 91.52997821335250705, 87.83041666666669300 ) ) ;
#32929=DIRECTION ( 'NONE',  ( 1.000000000000000000, 0.000000000000000000, 0.000000000000000000 ) ) ;
#32937=CARTESIAN_POINT ( 'NONE',  ( -96.15314808468745866, -211.9973110713294489, 79.74739583420048916 ) ) ;
#32946=CARTESIAN_POINT ( 'NONE',  ( -92.34999999999999432, -211.5299782133524218, 76.37395833506761278 ) ) ;
#32947=CARTESIAN_POINT ( 'NONE',  ( 97.30629616937498838, 88.66845928578035796, 78.47739583420047893 ) ) ;
#32961=CARTESIAN_POINT ( 'NONE',  ( -97.30629616937501680, 88.66845928578038638, 83.34572916753381833 ) ) ;
#32968=( BOUNDED_CURVE ( )  B_SPLINE_CURVE ( 2, ( #44150, #32852, #11412, #68577, #5431, #62575, #56170 ),
 .UNSPECIFIED., .F., .F. ) 
 B_SPLINE_CURVE_WITH_KNOTS ( ( 3, 2, 2, 3 ),
 ( 0.1905056698837213069, 0.1975614351447063655, 0.2046172006855886960, 0.2116728463006670724 ),
 .UNSPECIFIED. ) 
 CURVE ( )  GEOMETRIC_REPRESENTATION_ITEM ( )  RATIONAL_B_SPLINE_CURVE ( ( 1.000000000000000000, 0.8660254037844387076, 1.000000000000000000, 0.8660254037844387076, 1.000000000000000000, 0.8660276809308478096, 0.9999954457845905420 ) ) 
 REPRESENTATION_ITEM ( '' )  );
#32974=CARTESIAN_POINT ( 'NONE',  ( 97.30629616937498838, -209.9999999999999716, 79.95906250086714806 ) ) ;
#32978=EDGE_CURVE ( 'NONE', #3617, #72633, #18272, .T. ) ;
#32984=B_SPLINE_CURVE_WITH_KNOTS ( 'NONE', 3,
 ( #11503, #34435, #5157, #45375, #64138, #50995, #58117, #6614, #11867, #46103, #68297, #5523, #34820, #62675, #11150, #34072, #57017, #28425 ),
 .UNSPECIFIED., .F., .F.,
 ( 4, 2, 2, 2, 2, 2, 2, 2, 4 ),
 ( -0.004093595876927202080, -0.003575961939746029588, -0.003058328002564857095, -0.002540694065383684603, -0.002023060128202512110, -0.001505426191021339618, -0.0009877922538401671254, -0.0004701583166589946329, 4.747562052217785961E-05 ),
 .UNSPECIFIED. ) ;
#32986=CARTESIAN_POINT ( 'NONE',  ( 95.00000000000000000, -213.0599564267049857, 87.61875000000000568 ) ) ;
#32988=ORIENTED_EDGE ( 'NONE', *, *, #58810, .F. ) ;
#32999=CARTESIAN_POINT ( 'NONE',  ( 97.64999999999997726, -211.5299782133524502, 78.91395833506763324 ) ) ;
#33000=CARTESIAN_POINT ( 'NONE',  ( 97.64999999999999147, 90.00000000000002842, 82.06250000000000000 ) ) ;
#33004=CARTESIAN_POINT ( 'NONE',  ( 90.00000000000001421, -204.9999999999999716, -80.00000000000000000 ) ) ;
#33007=CARTESIAN_POINT ( 'NONE',  ( -96.15314808468751551, 88.00268892867056536, 82.92239583420048632 ) ) ;
#33010=CARTESIAN_POINT ( 'NONE',  ( 94.99999999999998579, 92.66308142843935514, 78.68906250086713783 ) ) ;
#33018=CARTESIAN_POINT ( 'NONE',  ( -93.84685191531248449, -208.0026889286704943, 82.44614583420046472 ) ) ;
#33022=CARTESIAN_POINT ( 'NONE',  ( 97.64999999999999147, 90.00000000000002842, 78.88750000000000284 ) ) ;
#33028=CARTESIAN_POINT ( 'NONE',  ( 93.67499999999999716, 87.70503267997126784, 88.91520833506763211 ) ) ;
#33030=CARTESIAN_POINT ( 'NONE',  ( -94.99999999999997158, -207.3369185715606307, 78.68906250086713783 ) ) ;
#33038=CARTESIAN_POINT ( 'NONE',  ( -95.00000000000002842, 86.94004357329504273, 89.52374999999999261 ) ) ;
#33039=CARTESIAN_POINT ( 'NONE',  ( 92.69370383062498320, 90.00000000000002842, 89.64281250086713726 ) ) ;
#33040=DIRECTION ( 'NONE',  ( -0.000000000000000000, -0.000000000000000000, 1.000000000000000000 ) ) ;
#33041=CARTESIAN_POINT ( 'NONE',  ( 2.500000000000015987, 65.00000000000000000, -290.0000000000000568 ) ) ;
#33042=DIRECTION ( 'NONE',  ( -1.000000000000000000, -0.000000000000000000, -0.000000000000000000 ) ) ;
#33047=CARTESIAN_POINT ( 'NONE',  ( -96.32500000000001705, 92.29496732002878900, 75.92416666666666458 ) ) ;
#33052=CARTESIAN_POINT ( 'NONE',  ( -94.99999999999997158, -206.9400435732949575, 85.39624999999998067 ) ) ;
#33054=LINE ( 'NONE', #60545, #51775 ) ;
#33062=CARTESIAN_POINT ( 'NONE',  ( 97.30629616937498838, -211.3315407142195852, 88.16114583420048234 ) ) ;
#33067=CARTESIAN_POINT ( 'NONE',  ( 0.000000000000000000, -80.00000000000000000, -90.00000000000000000 ) ) ;
#33072=CARTESIAN_POINT ( 'NONE',  ( 92.69370383062501162, -209.9999999999999716, 78.21281250086714465 ) ) ;
#33073=CARTESIAN_POINT ( 'NONE',  ( 95.00000000000000000, -207.3369185715606307, 86.46781250086714010 ) ) ;
#33076=CARTESIAN_POINT ( 'NONE',  ( 96.15314808468750130, -211.9973110713294489, 85.56822916753381492 ) ) ;
#33088=CARTESIAN_POINT ( 'NONE',  ( 92.35000000000000853, -209.9999999999999716, 89.44437500173430067 ) ) ;
#33091=VERTEX_POINT ( 'NONE', #55651 ) ;
#33098=DIRECTION ( 'NONE',  ( 1.000000000000000000, 0.000000000000000000, 0.000000000000000000 ) ) ;
#33102=CARTESIAN_POINT ( 'NONE',  ( -92.35000000000003695, 90.00000000000004263, 87.14249999999999829 ) ) ;
#33104=CARTESIAN_POINT ( 'NONE',  ( -97.30629616937501680, 88.66845928578038638, 77.15447916753382174 ) ) ;
#33107=VERTEX_POINT ( 'NONE', #9412 ) ;
#33108=CARTESIAN_POINT ( 'NONE',  ( 97.30629616937498838, 91.33154071421968467, 77.31322916753380525 ) ) ;
#33111=CARTESIAN_POINT ( 'NONE',  ( -96.15314808468745866, -211.9973110713294489, 89.11364583420048291 ) ) ;
#33118=CARTESIAN_POINT ( 'NONE',  ( -92.69370383062498320, -209.9999999999999716, 79.16531250086714522 ) ) ;
#33127=VECTOR ( 'NONE', #35463, 1000.000000000000000 ) ;
#33129=DIRECTION ( 'NONE',  ( 0.000000000000000000, 0.000000000000000000, -1.000000000000000000 ) ) ;
#33130=CARTESIAN_POINT ( 'NONE',  ( -97.30629616937501680, 90.00000000000004263, 82.65781250086713783 ) ) ;
#33131=CARTESIAN_POINT ( 'NONE',  ( 97.64999999999999147, 90.00000000000002842, 76.98250000000000171 ) ) ;
#33138=CARTESIAN_POINT ( 'NONE',  ( -95.00000000000002842, 90.00000000000004263, 90.00000000000000000 ) ) ;
#33143=CARTESIAN_POINT ( 'NONE',  ( -92.69370383062498320, -209.9999999999999716, 78.68906250086715204 ) ) ;
#33152=DIRECTION ( 'NONE',  ( -0.000000000000000000, -0.000000000000000000, 1.000000000000000000 ) ) ;
#33153=EDGE_CURVE ( 'NONE', #8129, #12189, #8163, .T. ) ;
#33156=FACE_OUTER_BOUND ( 'NONE', #62800, .T. ) ;
#33158=CARTESIAN_POINT ( 'NONE',  ( 92.34999999999999432, 90.00000000000002842, 78.57000000000000739 ) ) ;
#33161=CARTESIAN_POINT ( 'NONE',  ( 97.30629616937498838, -208.6684592857803295, 88.74322916753382628 ) ) ;
#33162=CARTESIAN_POINT ( 'NONE',  ( 92.35000000000000853, -209.9999999999999716, 86.18999999999999773 ) ) ;
#33164=EDGE_LOOP ( 'NONE', ( #2880, #37270, #49357, #56055 ) ) ;
#33170=CARTESIAN_POINT ( 'NONE',  ( -90.00000000000000000, -116.0000000000000142, 39.99999999999996447 ) ) ;
#33171=ORIENTED_EDGE ( 'NONE', *, *, #3599, .T. ) ;
#33175=CARTESIAN_POINT ( 'NONE',  ( -95.00000000000002842, 90.00000000000004263, 73.40771935957695860 ) ) ;
#33180=( BOUNDED_CURVE ( )  B_SPLINE_CURVE ( 2, ( #7751, #30300, #47597, #30665, #53245, #41587, #29552 ),
 .UNSPECIFIED., .F., .F. ) 
 B_SPLINE_CURVE_WITH_KNOTS ( ( 3, 2, 2, 3 ),
 ( 0.9374999999999995559, 0.9444444444444441977, 0.9513888888888889506, 0.9583333333333337034 ),
 .UNSPECIFIED. ) 
 CURVE ( )  GEOMETRIC_REPRESENTATION_ITEM ( )  RATIONAL_B_SPLINE_CURVE ( ( 1.000000000000008660, 0.8660254037844301589, 1.000000000000000000, 0.8660254037844387076, 1.000000000000000000, 0.8660254037844322683, 1.000000000000006439 ) ) 
 REPRESENTATION_ITEM ( '' )  );
#33181=CARTESIAN_POINT ( 'NONE',  ( 96.15314808468748708, 88.00268892867053694, 77.31322916753381946 ) ) ;
#33188=CARTESIAN_POINT ( 'NONE',  ( 97.30629616937498838, 90.00000000000002842, 87.42031250086714067 ) ) ;
#33191=CARTESIAN_POINT ( 'NONE',  ( 92.69370383062501162, -209.9999999999999716, 83.92781250086714806 ) ) ;
#33199=CARTESIAN_POINT ( 'NONE',  ( -94.99999999999997158, -212.6630814284392557, 87.26156250086714294 ) ) ;
#33200=CARTESIAN_POINT ( 'NONE',  ( -95.00000000000002842, 92.66308142843932671, 86.46781250086716852 ) ) ;
#33203=CARTESIAN_POINT ( 'NONE',  ( 97.30629616937498838, 90.00000000000002842, 89.32531250086714181 ) ) ;
#33204=CARTESIAN_POINT ( 'NONE',  ( -92.69370383062502583, 91.33154071421968467, 88.10822916753380696 ) ) ;
#33208=DIRECTION ( 'NONE',  ( 1.000000000000000000, 0.000000000000000000, 0.000000000000000000 ) ) ;
#33210=CARTESIAN_POINT ( 'NONE',  ( -97.30629616937495996, -209.9999999999999716, 89.00781250086714635 ) ) ;
#33216=ORIENTED_EDGE ( 'NONE', *, *, #38442, .T. ) ;
#33217=CARTESIAN_POINT ( 'NONE',  ( -92.35000000000005116, 91.52997821335253548, 80.21041666666666003 ) ) ;
#33219=FACE_OUTER_BOUND ( 'NONE', #26152, .T. ) ;
#33222=CARTESIAN_POINT ( 'NONE',  ( 92.35000000003358878, -210.0000076551254153, 78.01464417100928017 ) ) ;
#33226=CARTESIAN_POINT ( 'NONE',  ( -92.69370383062502583, 88.66845928578038638, 81.01739583420048518 ) ) ;
#33227=AXIS2_PLACEMENT_3D ( 'NONE', #17018, #11724, #57620 ) ;
#33232=DIRECTION ( 'NONE',  ( -0.000000000000000000, -0.000000000000000000, 1.000000000000000000 ) ) ;
#33233=CARTESIAN_POINT ( 'NONE',  ( -96.32500000000001705, 92.29496732002878900, 82.27416666666665890 ) ) ;
#33234=VECTOR ( 'NONE', #35916, 1000.000000000000000 ) ;
#33236=CARTESIAN_POINT ( 'NONE',  ( 94.99999999999998579, 92.66308142843932671, 82.02281250086714692 ) ) ;
#33237=CARTESIAN_POINT ( 'NONE',  ( -94.99999999999997158, -212.6630814284392557, 79.80031250086715033 ) ) ;
#33241=CARTESIAN_POINT ( 'NONE',  ( -97.64999999999994884, -211.5299782133524502, 75.44791666666667140 ) ) ;
#33244=AXIS2_PLACEMENT_3D ( 'NONE', #62711, #16076, #15707 ) ;
#33246=CARTESIAN_POINT ( 'NONE',  ( -92.69370383062505425, 91.33154071421968467, 78.10697916753383652 ) ) ;
#33247=CARTESIAN_POINT ( 'NONE',  ( 93.84685191531249870, -208.0026889286704943, 81.28197916753380525 ) ) ;
#33257=ORIENTED_EDGE ( 'NONE', *, *, #59430, .F. ) ;
#33263=CARTESIAN_POINT ( 'NONE',  ( 93.84685191531248449, 91.99731107132950569, 85.88572916753381037 ) ) ;
#33264=CARTESIAN_POINT ( 'NONE',  ( -26.50044424985255276, 0.001194404164626844313, -80.00000000000000000 ) ) ;
#33265=CARTESIAN_POINT ( 'NONE',  ( 93.67500000000001137, -207.7050326799711968, 79.09916666666666174 ) ) ;
#33267=ORIENTED_EDGE ( 'NONE', *, *, #31155, .F. ) ;
#33273=EDGE_CURVE ( 'NONE', #21836, #19615, #53835, .T. ) ;
#33280=CYLINDRICAL_SURFACE ( 'NONE', #70756, 2.649999999999999467 ) ;
#33281=DIRECTION ( 'NONE',  ( 1.000000000000000000, 0.000000000000000000, 0.000000000000000000 ) ) ;
#33283=CARTESIAN_POINT ( 'NONE',  ( -96.32499999999996021, -207.7050326799711968, 84.25854166840096582 ) ) ;
#33285=DIRECTION ( 'NONE',  ( 1.000000000000000000, 0.000000000000000000, 0.000000000000000000 ) ) ;
#33288=CARTESIAN_POINT ( 'NONE',  ( 93.67499999999998295, 92.29496732002878900, 82.98854166840096980 ) ) ;
#33289=CARTESIAN_POINT ( 'NONE',  ( -97.65000000000001990, 88.47002178664754979, 82.51229166840094820 ) ) ;
#33291=CARTESIAN_POINT ( 'NONE',  ( 96.15314808468748708, 88.00268892867053694, 84.93322916753382401 ) ) ;
#33306=CARTESIAN_POINT ( 'NONE',  ( -93.84685191531248449, -208.0026889286704943, 82.60489583420049087 ) ) ;
#33317=DIRECTION ( 'NONE',  ( 1.343011723336883198E-16, -1.000000000000000000, 0.000000000000000000 ) ) ;
#33319=DIRECTION ( 'NONE',  ( -0.000000000000000000, -0.000000000000000000, -1.000000000000000000 ) ) ;
#33322=CARTESIAN_POINT ( 'NONE',  ( 96.15314808468748708, 88.00268892867053694, 89.37822916753381719 ) ) ;
#33327=EDGE_CURVE ( 'NONE', #30842, #52479, #15397, .T. ) ;
#33328=CARTESIAN_POINT ( 'NONE',  ( -97.30629616937501680, 91.33154071421968467, 80.69989583420046131 ) ) ;
#33332=DIRECTION ( 'NONE',  ( -0.000000000000000000, -0.000000000000000000, 1.000000000000000000 ) ) ;
#33339=LINE ( 'NONE', #56300, #34722 ) ;
#33340=CARTESIAN_POINT ( 'NONE',  ( 95.00000000000000000, -212.6630814284392557, 76.62531250086715318 ) ) ;
#33343=ORIENTED_EDGE ( 'NONE', *, *, #29268, .T. ) ;
#33351=AXIS2_PLACEMENT_3D ( 'NONE', #14391, #21128, #31676 ) ;
#33355=CARTESIAN_POINT ( 'NONE',  ( 93.67500000000001137, -207.7050326799711968, 88.62416666666665321 ) ) ;
#33357=CARTESIAN_POINT ( 'NONE',  ( -97.64999999999990621, -208.4700217866474077, 88.04208333333330927 ) ) ;
#33359=ORIENTED_EDGE ( 'NONE', *, *, #31783, .T. ) ;
#33365=CARTESIAN_POINT ( 'NONE',  ( 97.64999999999997726, -208.4700217866474645, 79.65479166840096070 ) ) ;
#33366=CARTESIAN_POINT ( 'NONE',  ( 97.64999999999997726, 88.47002178664753558, 81.37458333333333371 ) ) ;
#33368=CARTESIAN_POINT ( 'NONE',  ( 92.35000000000000853, -209.9999999999999716, 75.47437500173430180 ) ) ;
#33373=CARTESIAN_POINT ( 'NONE',  ( -97.30629616937501680, 90.00000000000004263, 84.72156250086715090 ) ) ;
#33375=CARTESIAN_POINT ( 'NONE',  ( 96.15314808468748708, 88.00268892867053694, 78.42447916753381776 ) ) ;
#33385=CARTESIAN_POINT ( 'NONE',  ( -96.15314808468745866, -211.9973110713294489, 78.95364583420047211 ) ) ;
#33387=ORIENTED_EDGE ( 'NONE', *, *, #44665, .T. ) ;
#33389=CARTESIAN_POINT ( 'NONE',  ( 96.32499999999997442, 92.29496732002878900, 78.99333333333332519 ) ) ;
#33394=CARTESIAN_POINT ( 'NONE',  ( -92.69370383062498320, -208.6684592857803011, 75.40822916753381833 ) ) ;
#33395=ORIENTED_EDGE ( 'NONE', *, *, #25572, .F. ) ;
#33399=CARTESIAN_POINT ( 'NONE',  ( -97.64999999999996305, -209.9999999999999716, 89.44437500173430067 ) ) ;
#33403=CARTESIAN_POINT ( 'NONE',  ( 93.84685191531248449, 91.99731107132950569, 87.63197916753379957 ) ) ;
#33405=CARTESIAN_POINT ( 'NONE',  ( -92.35000000000005116, -211.0554082285339916, 75.04099707143593889 ) ) ;
#33409=DIRECTION ( 'NONE',  ( 0.000000000000000000, 0.000000000000000000, 1.000000000000000000 ) ) ;
#33416=( BOUNDED_CURVE ( )  B_SPLINE_CURVE ( 2, ( #64406, #68937, #57660, #64040, #6166, #29069, #23443 ),
 .UNSPECIFIED., .F., .F. ) 
 B_SPLINE_CURVE_WITH_KNOTS ( ( 3, 2, 2, 3 ),
 ( 0.06249999999999966693, 0.06944444444444407283, 0.07638888888888849260, 0.08333333333333288462 ),
 .UNSPECIFIED. ) 
 CURVE ( )  GEOMETRIC_REPRESENTATION_ITEM ( )  RATIONAL_B_SPLINE_CURVE ( ( 1.000000000000006439, 0.8660254037844322683, 1.000000000000000000, 0.8660254037844387076, 1.000000000000000000, 0.8660254037844472563, 0.9999999999999914513 ) ) 
 REPRESENTATION_ITEM ( '' )  );
#33417=CARTESIAN_POINT ( 'NONE',  ( -97.65000000000009095, 91.52997821335249284, 75.97708333333333997 ) ) ;
#33422=CARTESIAN_POINT ( 'NONE',  ( -92.35000000000003695, 90.00000000000004263, 90.00000000000000000 ) ) ;
#33425=CARTESIAN_POINT ( 'NONE',  ( -97.64999999999994884, -208.4700217866474645, 83.59708333333334451 ) ) ;
#33427=EDGE_CURVE ( 'NONE', #66194, #16558, #52979, .T. ) ;
#33430=FACE_OUTER_BOUND ( 'NONE', #41617, .T. ) ;
#33435=CARTESIAN_POINT ( 'NONE',  ( 97.30629616937498838, -209.9999999999999716, 87.57906250086715261 ) ) ;
#33441=LINE ( 'NONE', #39478, #59624 ) ;
#33444=CARTESIAN_POINT ( 'NONE',  ( 93.84685191531249870, -208.0026889286704943, 76.83697916753381207 ) ) ;
#33445=ORIENTED_EDGE ( 'NONE', *, *, #11598, .T. ) ;
#33446=CARTESIAN_POINT ( 'NONE',  ( 95.00000000000000000, -207.3369185715606307, 81.38781250086715602 ) ) ;
#33448=ORIENTED_EDGE ( 'NONE', *, *, #58795, .F. ) ;
#33451=CARTESIAN_POINT ( 'NONE',  ( -96.15314808468751551, 88.00268892867056536, 75.30239583420048177 ) ) ;
#33453=CARTESIAN_POINT ( 'NONE',  ( -92.35000000000395914, -210.0000045800647115, 76.42687486209126746 ) ) ;
#33459=ORIENTED_EDGE ( 'NONE', *, *, #38002, .F. ) ;
#33461=APPLICATION_CONTEXT ( 'automotive_design' ) ;
#33476=CARTESIAN_POINT ( 'NONE',  ( -97.65000000000001990, 88.47002178664754979, 89.41791666666667027 ) ) ;
#33481=CARTESIAN_POINT ( 'NONE',  ( -96.15314808468745866, -211.9973110713294489, 85.30364583420046642 ) ) ;
#33482=EDGE_LOOP ( 'NONE', ( #38936, #34522, #11666, #52927 ) ) ;
#33486=CARTESIAN_POINT ( 'NONE',  ( -92.69370383062498320, -208.6684592857803295, 80.48822916753380241 ) ) ;
#33491=CARTESIAN_POINT ( 'NONE',  ( -97.64999999999990621, -211.5299782133524786, 79.25791666666667368 ) ) ;
#33493=ORIENTED_EDGE ( 'NONE', *, *, #31324, .F. ) ;
#33498=CARTESIAN_POINT ( 'NONE',  ( 92.34999999999999432, 90.00000000000002842, 90.00000000000000000 ) ) ;
#33499=CARTESIAN_POINT ( 'NONE',  ( -97.30629616937501680, 91.33154071421968467, 81.33489583420048064 ) ) ;
#33503=FACE_OUTER_BOUND ( 'NONE', #7881, .T. ) ;
#33514=CARTESIAN_POINT ( 'NONE',  ( -92.69370383062498320, -208.6684592857803011, 80.01197916753380923 ) ) ;
#33518=ADVANCED_FACE ( 'NONE', ( #32244 ), #55564, .T. ) ;
#33520=CARTESIAN_POINT ( 'NONE',  ( -96.32500000000001705, 92.29496732002878900, 88.62416666666665321 ) ) ;
#33531=CARTESIAN_POINT ( 'NONE',  ( -99.99999999999997158, -204.9999999999999716, -79.99999999999998579 ) ) ;
#33534=CARTESIAN_POINT ( 'NONE',  ( 95.00000000000000000, -212.6630814284392557, 88.53156250086716739 ) ) ;
#33535=DIRECTION ( 'NONE',  ( 0.000000000000000000, 1.000000000000000000, 0.000000000000000000 ) ) ;
#33547=ORIENTED_EDGE ( 'NONE', *, *, #33959, .F. ) ;
#33553=CARTESIAN_POINT ( 'NONE',  ( 96.15314808468748708, 88.00268892867053694, 76.04322916753382344 ) ) ;
#33560=CARTESIAN_POINT ( 'NONE',  ( 92.69370383062498320, 88.66845928578037217, 88.42572916753380241 ) ) ;
#33562=CARTESIAN_POINT ( 'NONE',  ( 92.69370383062501162, -209.9999999999999716, 85.19781250086714408 ) ) ;
#33567=CARTESIAN_POINT ( 'NONE',  ( -97.64999999953592180, 89.99996903277666149, 77.38038495128051864 ) ) ;
#33574=CARTESIAN_POINT ( 'NONE',  ( -96.15314808468745866, -211.9973110713294489, 88.47864583420047779 ) ) ;
#33575=CARTESIAN_POINT ( 'NONE',  ( -97.30629616937501680, 90.00000000000004263, 84.72156250086715090 ) ) ;
#33576=ORIENTED_EDGE ( 'NONE', *, *, #69522, .T. ) ;
#33577=CARTESIAN_POINT ( 'NONE',  ( 97.30629616937498838, 90.00000000000002842, 88.05531250086713158 ) ) ;
#33578=CARTESIAN_POINT ( 'NONE',  ( -92.69370383062502583, 91.33154071421968467, 85.56822916753380071 ) ) ;
#33582=CARTESIAN_POINT ( 'NONE',  ( 92.35000000000000853, -209.9999999999999716, 87.45999999999999375 ) ) ;
#33585=CARTESIAN_POINT ( 'NONE',  ( 92.35000000000000853, -209.9999999999999716, 82.37999999999999545 ) ) ;
#33593=CARTESIAN_POINT ( 'NONE',  ( -93.67500000000003979, 92.29496732002878900, 81.53333333333333144 ) ) ;
#33594=EDGE_CURVE ( 'NONE', #19615, #55850, #49446, .T. ) ;
#33598=CARTESIAN_POINT ( 'NONE',  ( -97.64997259622870729, 91.52999403492728447, 79.86645724064027263 ) ) ;
#33602=AXIS2_PLACEMENT_3D ( 'NONE', #73906, #26650, #50983 ) ;
#33604=CARTESIAN_POINT ( 'NONE',  ( -92.69370383062502583, 88.66845928578038638, 79.74739583420047495 ) ) ;
#33606=EDGE_CURVE ( 'NONE', #5670, #59848, #38274, .T. ) ;
#33609=CARTESIAN_POINT ( 'NONE',  ( 95.00000000000000000, -209.9999999999999716, 90.00000000000000000 ) ) ;
#33613=CARTESIAN_POINT ( 'NONE',  ( -92.35000000000005116, 91.52997821335254969, 82.11541666666664696 ) ) ;
#33619=CARTESIAN_POINT ( 'NONE',  ( 97.30629616937498838, 91.33154071421968467, 80.01197916753382344 ) ) ;
#33620=CARTESIAN_POINT ( 'NONE',  ( -93.84685191531247028, -211.9973110713294489, 79.21822916753382060 ) ) ;
#33622=VERTEX_POINT ( 'NONE', #22099 ) ;
#33623=CARTESIAN_POINT ( 'NONE',  ( -96.32500000000001705, 87.70503267997129626, 87.01020833506763097 ) ) ;
#33629=AXIS2_PLACEMENT_3D ( 'NONE', #37280, #26351, #37646 ) ;
#33631=CARTESIAN_POINT ( 'NONE',  ( -95.00000000000002842, 87.33691857156074434, 78.53031250086715431 ) ) ;
#33632=CARTESIAN_POINT ( 'NONE',  ( 93.84685191531249870, -208.0026889286704943, 79.37697916753380412 ) ) ;
#33638=( BOUNDED_CURVE ( )  B_SPLINE_CURVE ( 2, ( #31298, #21781, #54252, #48600, #71513, #8750, #37331 ),
 .UNSPECIFIED., .F., .F. ) 
 B_SPLINE_CURVE_WITH_KNOTS ( ( 3, 2, 2, 3 ),
 ( 0.3333333333333333703, 0.3402777777777777901, 0.3472222222222221544, 0.3541666666666665741 ),
 .UNSPECIFIED. ) 
 CURVE ( )  GEOMETRIC_REPRESENTATION_ITEM ( )  RATIONAL_B_SPLINE_CURVE ( ( 0.9999999999999988898, 0.8660254037844398178, 1.000000000000000000, 0.8660254037844387076, 1.000000000000000000, 0.8660254037844408170, 0.9999999999999978906 ) ) 
 REPRESENTATION_ITEM ( '' )  );
#33639=CARTESIAN_POINT ( 'NONE',  ( -97.64999999998384794, -210.0000060634594661, 88.17456390440159453 ) ) ;
#33640=ORIENTED_EDGE ( 'NONE', *, *, #33768, .F. ) ;
#33642=ORIENTED_EDGE ( 'NONE', *, *, #47066, .T. ) ;
#33645=CARTESIAN_POINT ( 'NONE',  ( 92.69370383062501162, -209.9999999999999716, 75.19656250086714522 ) ) ;
#33649=CARTESIAN_POINT ( 'NONE',  ( 93.84685191531248449, 91.99731107132950569, 85.25072916753381946 ) ) ;
#33651=CARTESIAN_POINT ( 'NONE',  ( 97.64999999999997726, -208.4700217866474645, 76.40041666666667197 ) ) ;
#33664=CARTESIAN_POINT ( 'NONE',  ( 92.35004149907317128, 88.46999782714644311, 83.78229332575389776 ) ) ;
#33666=CARTESIAN_POINT ( 'NONE',  ( -97.64999999999994884, -211.5299782133524502, 83.14729166840096752 ) ) ;
#33667=EDGE_LOOP ( 'NONE', ( #52698, #7030, #47339, #70148 ) ) ;
#33670=CARTESIAN_POINT ( 'NONE',  ( 92.34999999999999432, 90.00000000000002842, 83.72937500173429726 ) ) ;
#33671=CARTESIAN_POINT ( 'NONE',  ( -92.35000000000005116, 88.47002178664754979, 80.18395833506764347 ) ) ;
#33673=CARTESIAN_POINT ( 'NONE',  ( 92.69370383062498320, 88.66845928578037217, 82.86947916753382515 ) ) ;
#33674=CARTESIAN_POINT ( 'NONE',  ( 94.99999999999998579, 93.05995642670504253, 83.49125000000000796 ) ) ;
#33689=EDGE_CURVE ( 'NONE', #44189, #13090, #47530, .T. ) ;
#33692=FACE_OUTER_BOUND ( 'NONE', #20903, .T. ) ;
#33694=CARTESIAN_POINT ( 'NONE',  ( -2.500000000000012879, -65.00000000000000000, -290.0000000000000568 ) ) ;
#33695=CARTESIAN_POINT ( 'NONE',  ( -94.99999999999997158, -207.3369185715606307, 80.75281250086715090 ) ) ;
#33696=ORIENTED_EDGE ( 'NONE', *, *, #64843, .T. ) ;
#33697=CARTESIAN_POINT ( 'NONE',  ( -97.30629616937501680, 91.33154071421968467, 88.95489583420048518 ) ) ;
#33700=CARTESIAN_POINT ( 'NONE',  ( -97.64995975555112295, -211.5300014484957956, 77.43229327564779396 ) ) ;
#33701=CARTESIAN_POINT ( 'NONE',  ( 96.32499999999998863, 87.70503267997126784, 82.03604166840096923 ) ) ;
#33712=EDGE_CURVE ( 'NONE', #41677, #24219, #18702, .T. ) ;
#33720=CARTESIAN_POINT ( 'NONE',  ( -95.00000000000002842, 92.66308142843932671, 80.59406250086715318 ) ) ;
#33724=CARTESIAN_POINT ( 'NONE',  ( 93.84685191531249870, -208.0026889286704943, 88.90197916753380980 ) ) ;
#33726=VERTEX_POINT ( 'NONE', #47164 ) ;
#33728=CARTESIAN_POINT ( 'NONE',  ( -94.99999999999997158, -209.9999999999999716, 90.00000000000000000 ) ) ;
#33734=CARTESIAN_POINT ( 'NONE',  ( 95.00000000000000000, -207.3369185715606307, 76.30781250086715772 ) ) ;
#33739=CARTESIAN_POINT ( 'NONE',  ( 97.06449789201064959, -208.9360650323630182, 74.79348190356853365 ) ) ;
#33744=CARTESIAN_POINT ( 'NONE',  ( 92.35000000000000853, -209.9999999999999716, 87.45999999999999375 ) ) ;
#33745=EDGE_LOOP ( 'NONE', ( #27680, #597, #38171, #72552 ) ) ;
#33753=CARTESIAN_POINT ( 'NONE',  ( 97.64999999999999147, -209.9999999999999716, 75.15687500173430635 ) ) ;
#33754=CARTESIAN_POINT ( 'NONE',  ( 97.64999999999997726, 88.47002178664753558, 80.73958333333332860 ) ) ;
#33761=CARTESIAN_POINT ( 'NONE',  ( -92.69370383062504004, 90.00000000000004263, 83.13406250086715943 ) ) ;
#33762=CARTESIAN_POINT ( 'NONE',  ( 92.69370383062498320, 88.66845928578037217, 77.63072916753380071 ) ) ;
#33768=EDGE_CURVE ( 'NONE', #62654, #57250, #64455, .T. ) ;
#33773=CARTESIAN_POINT ( 'NONE',  ( -94.99999999999997158, -212.6630814284392557, 79.00656250086713328 ) ) ;
#33775=EDGE_CURVE ( 'NONE', #67569, #44773, #5773, .T. ) ;
#33778=CARTESIAN_POINT ( 'NONE',  ( 100.0010000000000190, -123.9999999999999858, -40.00000000000002132 ) ) ;
#33779=ADVANCED_FACE ( 'NONE', ( #55008 ), #36608, .F. ) ;
#33780=ADVANCED_FACE ( 'NONE', ( #54287, #9148, #53910, #71177, #36981, #25341 ), #59556, .T. ) ;
#33782=ORIENTED_EDGE ( 'NONE', *, *, #69130, .T. ) ;
#33785=CARTESIAN_POINT ( 'NONE',  ( -93.84685191531247028, -211.9973110713294489, 75.88447916753381151 ) ) ;
#33787=CARTESIAN_POINT ( 'NONE',  ( -97.64999999996709334, -209.9999916080759306, 86.90410584369134028 ) ) ;
#33795=CARTESIAN_POINT ( 'NONE',  ( 92.69370383062498320, 91.33154071421968467, 86.41489583420047893 ) ) ;
#33812=CARTESIAN_POINT ( 'NONE',  ( -97.64999999999996305, -209.9999999999999716, 86.18999999999999773 ) ) ;
#33813=CARTESIAN_POINT ( 'NONE',  ( -92.35000000000003695, 90.00000000000004263, 80.15749999999999886 ) ) ;
#33820=CARTESIAN_POINT ( 'NONE',  ( 97.30629616937498838, -208.6684592857803011, 85.72697916753381264 ) ) ;
#33825=DIRECTION ( 'NONE',  ( -0.000000000000000000, -0.000000000000000000, 1.000000000000000000 ) ) ;
#33828=AXIS2_PLACEMENT_3D ( 'NONE', #71651, #61133, #14134 ) ;
#33829=CARTESIAN_POINT ( 'NONE',  ( 92.69370383062501162, -209.9999999999999716, 76.94281250086713442 ) ) ;
#33831=CARTESIAN_POINT ( 'NONE',  ( 95.00000000000000000, -212.6630814284392557, 82.97531250086716170 ) ) ;
#33842=CARTESIAN_POINT ( 'NONE',  ( 92.35000000000000853, -209.9999999999999716, 76.74437500173429783 ) ) ;
#33843=CARTESIAN_POINT ( 'NONE',  ( 95.00000000000000000, -213.0599564267049857, 88.33312500173428816 ) ) ;
#33847=( BOUNDED_CURVE ( )  B_SPLINE_CURVE ( 2, ( #8193, #36391, #60097, #12720, #42786, #1497, #31122 ),
 .UNSPECIFIED., .F., .F. ) 
 B_SPLINE_CURVE_WITH_KNOTS ( ( 3, 2, 2, 3 ),
 ( 0.4166666666666662966, 0.4236111111111106609, 0.4305555555555550806, 0.4374999999999994449 ),
 .UNSPECIFIED. ) 
 CURVE ( )  GEOMETRIC_REPRESENTATION_ITEM ( )  RATIONAL_B_SPLINE_CURVE ( ( 1.000000000000007550, 0.8660254037844311581, 1.000000000000000000, 0.8660254037844387076, 1.000000000000000000, 0.8660254037844493658, 0.9999999999999893419 ) ) 
 REPRESENTATION_ITEM ( '' )  );
#33853=CARTESIAN_POINT ( 'NONE',  ( 96.15314808468750130, -211.9973110713294489, 75.24947916753380639 ) ) ;
#33859=CARTESIAN_POINT ( 'NONE',  ( 96.32499999999997442, 92.29496732002878900, 79.70770833506762187 ) ) ;
#33862=CARTESIAN_POINT ( 'NONE',  ( -97.30629616937501680, 90.00000000000004263, 76.46656250086715545 ) ) ;
#33864=CARTESIAN_POINT ( 'NONE',  ( 93.84685191531248449, 91.99731107132950569, 74.93197916753379673 ) ) ;
#33867=( BOUNDED_SURFACE ( )  B_SPLINE_SURFACE ( 1, 2, ( 
 ( #34497, #344, #51052, #57440, #16856, #29579, #28865, #46907, #18318, #46526, #11204, #5216, #63832, #69095, #40896, #17583, #45432, #12305, #40515, #63459, #11934, #1077, #69452, #68361, #703, #23973, #23596, #71662, #43121, #48738, #54385, #36715, #66052, #58539, #70541, #20160, #7420, #35605, #29961, #7034, #54025, #1451, #2563, #19052, #14149, #30333, #52912, #24337, #25443, #47273, #2184, #42736, #59663, #18679, #53277, #42371, #47634, #8145, #65672, #1814, #53645, #70176, #24700, #31070, #36347, #42004, #48371, #13037, #13779, #64941, #41621, #71284, #37098, #48009, #13416, #64559, #19422, #19789, #60049, #25069, #2917, #8532, #31444, #35976, #25808, #59289, #58928, #7782, #30698, #70922, #65310, #44221, #27664, #21261, #26547, #54753, #31808, #4012, #55498, #15648, #38581, #14900, #32551, #60410, #66419, #49107, #38953, #66774, #4758, #50589, #4380, #72034, #73516, #21648, #55119, #73142, #72404, #22023, #44602, #20909, #67144, #43859, #67519, #27278, #37479, #61513, #56243, #16007, #44968, #14526, #8891, #33289, #9996, #3282, #26171, #49479, #20546, #60774, #43500, #37843, #9256, #32916, #32176, #55868, #15269, #61889, #3646, #38201, #61144, #50208, #9633, #26914, #10369, #49844, #72760, #62642, #261, #5498, #17496, #618, #11118, #11481, #23884, #39703, #40425, #68647, #34042, #11839, #45345, #46075, #28394, #73889, #10747, #51330, #28773, #33671, #34409, #39326, #35158, #6237, #63373, #46440, #52436, #17129, #34790, #69010, #16765, #74266, #57731, #23152, #29137, #22398, #52073, #23509, #56626, #68269, #5125, #56993, #22783, #58094, #29500, #69368, #28026, #990, #17864, #45725, #40810, #40061, #6596, #63745, #63022, #12221, #57352, #67894, #16384, #62262, #50968, #5864, #51713, #8444, #54307, #59959, #65589, #47916, #2832, #69735, #7334, #31355, #18597, #46820, #41176, #18235, #65221, #12593, #13692, #30250, #25362, #41537, #64112, #35524, #36629, #58451, #13329, #53937, #70835, #29873, #64474, #53557, #58834, #19336, #2475, #12949, #64850, #6949, #35886, #42292, #47550, #53189, #59574, #24258, #24981, #1725, #52825, #1367, #24613, #7692, #47182, #36263, #70094, #14056, #8060, #30981, #48289, #70454, #18961, #71197, #19703, #41910, #59201, #42651, #2094, #37006, #30609, #55406, #26825 ),
 ( #61430, #67429, #32830, #49751, #73048, #9909, #43415, #66337, #43027, #14810, #25721, #21176, #8806, #38858, #3196, #37757, #26086, #71575, #20072, #60691, #10282, #60328, #37394, #9170, #38491, #61801, #50113, #65968, #61051, #33204, #56148, #48660, #3562, #14440, #49016, #54668, #55779, #31723, #32093, #3929, #72674, #26460, #71947, #20461, #67051, #38112, #55033, #9548, #44127, #15558, #49396, #4297, #72322, #27185, #20821, #43773, #66692, #15178, #32464, #21554, #44512, #15925, #56535, #5772, #63287, #51620, #17042, #68920, #28679, #27943, #50873, #73430, #73796, #4667, #34325, #39236, #34693, #33578, #45254, #5038, #50502, #21937, #22310, #29053, #62166, #16296, #68171, #172, #57647, #17406, #44880, #74174, #27574, #67802, #10652, #23063, #62551, #45992, #45637, #16671, #39609, #51242, #11032, #33956, #68555, #40341, #56905, #6147, #5411, #28306, #22689, #39978, #62933, #11746, #11391, #57267, #39262, #55433, #44534, #50529, #32856, #62191, #54693, #66717, #16322, #3586, #67828, #26108, #31749, #50141, #71970, #73076, #15203, #10310, #26487, #3219, #49043, #21581, #20484, #72696, #38887, #55806, #14832, #49419, #38513, #43799, #4322, #61825, #72346, #49778, #43440, #20845, #27208, #32488, #38139, #67454, #9196, #9935, #61075, #37784, #66357, #21200, #15946, #33226, #32116, #44154, #60716, #55056, #9568, #56173, #3951, #21959, #26853, #4694, #67080, #15580, #27600, #61453, #73454, #44907, #23812, #69305, #17070, #17435, #40002, #63685, #555, #33604, #11770, #52377, #33981, #18172, #34348, #23450, #29432, #34724, #41115, #56563, #45658, #69674, #56930, #46754, #5066, #10678, #29075, #50899, #52003, #68581, #12152, #5434, #27964, #73823, #46379, #22337, #51647, #17792, #57668, #68201, #28329, #40364, #22719, #6173, #40742, #51267, #28708, #45280, #74202, #35098, #11415, #62961, #58025, #62578, #63310, #57288, #16698, #39633, #5802, #46016, #11060, #194, #23088, #925, #6531, #68947, #42586, #48596, #13268, #59512, #65161, #12887, #24552, #7998, #70772, #13632, #70029, #19274, #36562, #29806, #64414, #6889, #53127, #1667, #30916, #71137, #2032, #41840, #52761, #47847, #48227, #42230, #7629, #31291, #25298, #19639, #71507, #53860, #70391, #65524, #35818, #64788, #53496, #54245, #2408, #2773, #13995 ) ),
 .UNSPECIFIED., .F., .F., .F. ) 
 B_SPLINE_SURFACE_WITH_KNOTS ( ( 2, 2 ),
 ( 3, 2, 2, 2, 2, 2, 2, 2, 2, 2, 2, 2, 2, 2, 2, 2, 2, 2, 2, 2, 2, 2, 2, 2, 2, 2, 2, 2, 2, 2, 2, 2, 2, 2, 2, 2, 2, 2, 2, 2, 2, 2, 2, 2, 2, 2, 2, 2, 2, 2, 2, 2, 2, 2, 2, 2, 2, 2, 2, 2, 2, 2, 2, 2, 2, 2, 2, 2, 2, 2, 2, 2, 2, 2, 2, 2, 2, 2, 2, 2, 2, 2, 2, 2, 2, 2, 2, 2, 2, 2, 2, 2, 2, 2, 2, 2, 2, 2, 2, 2, 2, 2, 2, 2, 2, 2, 2, 2, 2, 2, 2, 2, 2, 2, 2, 2, 2, 2, 2, 2, 2, 2, 2, 2, 2, 2, 2, 2, 2, 2, 2, 2, 2, 2, 2, 2, 2, 2, 2, 2, 2, 2, 3 ),
 ( 0.000000000000000000, 1.000000000000000000 ),
 ( 0.000000000000000000, 0.006944444444444444059, 0.01388888888888888812, 0.02083333333333333218, 0.02777777777777777624, 0.03472222222222222376, 0.04166666666666666435, 0.04861111111111111188, 0.05555555555555555247, 0.06250000000000000000, 0.06944444444444444753, 0.07638888888888889506, 0.08333333333333332871, 0.09027777777777777624, 0.09722222222222222376, 0.1041666666666666713, 0.1111111111111111049, 0.1180555555555555525, 0.1250000000000000000, 0.1319444444444444475, 0.1388888888888888951, 0.1458333333333333426, 0.1527777777777777901, 0.1597222222222222099, 0.1666666666666666574, 0.1736111111111111049, 0.1805555555555555525, 0.1875000000000000000, 0.1944444444444444475, 0.2013888888888888951, 0.2083333333333333426, 0.2152777777777777901, 0.2222222222222222099, 0.2291666666666666574, 0.2361111111111111049, 0.2430555555555555525, 0.2500000000000000000, 0.2569444444444444198, 0.2638888888888888951, 0.2708333333333333148, 0.2777777777777777901, 0.2847222222222222099, 0.2916666666666666852, 0.2986111111111111049, 0.3055555555555555802, 0.3125000000000000000, 0.3194444444444444198, 0.3263888888888888951, 0.3333333333333333148, 0.3402777777777777901, 0.3472222222222222099, 0.3541666666666666852, 0.3611111111111111049, 0.3680555555555555802, 0.3750000000000000000, 0.3819444444444444198, 0.3888888888888888951, 0.3958333333333333148, 0.4027777777777777901, 0.4097222222222222099, 0.4166666666666666852, 0.4236111111111111049, 0.4305555555555555802, 0.4375000000000000000, 0.4444444444444444198, 0.4513888888888888951, 0.4583333333333333148, 0.4652777777777777901, 0.4722222222222222099, 0.4791666666666666852, 0.4861111111111111049, 0.4930555555555555802, 0.5000000000000000000, 0.5069444444444444198, 0.5138888888888888395, 0.5208333333333333703, 0.5277777777777777901, 0.5347222222222222099, 0.5416666666666666297, 0.5486111111111111605, 0.5555555555555555802, 0.5625000000000000000, 0.5694444444444444198, 0.5763888888888888395, 0.5833333333333333703, 0.5902777777777777901, 0.5972222222222222099, 0.6041666666666666297, 0.6111111111111111605, 0.6180555555555555802, 0.6250000000000000000, 0.6319444444444444198, 0.6388888888888888395, 0.6458333333333333703, 0.6527777777777777901, 0.6597222222222222099, 0.6666666666666666297, 0.6736111111111111605, 0.6805555555555555802, 0.6875000000000000000, 0.6944444444444444198, 0.7013888888888888395, 0.7083333333333333703, 0.7152777777777777901, 0.7222222222222222099, 0.7291666666666666297, 0.7361111111111111605, 0.7430555555555555802, 0.7500000000000000000, 0.7569444444444444198, 0.7638888888888888395, 0.7708333333333333703, 0.7777777777777777901, 0.7847222222222222099, 0.7916666666666666297, 0.7986111111111111605, 0.8055555555555555802, 0.8125000000000000000, 0.8194444444444444198, 0.8263888888888888395, 0.8333333333333333703, 0.8402777777777777901, 0.8472222222222222099, 0.8541666666666666297, 0.8611111111111111605, 0.8680555555555555802, 0.8750000000000000000, 0.8819444444444444198, 0.8888888888888888395, 0.8958333333333333703, 0.9027777777777777901, 0.9097222222222222099, 0.9166666666666666297, 0.9236111111111111605, 0.9305555555555555802, 0.9375000000000000000, 0.9444444444444444198, 0.9513888888888888395, 0.9583333333333333703, 0.9652777777777777901, 0.9722222222222222099, 0.9791666666666666297, 0.9842226981114289286 ),
 .UNSPECIFIED. ) 
 GEOMETRIC_REPRESENTATION_ITEM ( )  RATIONAL_B_SPLINE_SURFACE ( (
 ( 1.000000000000000000, 0.8660254037844387076, 1.000000000000000000, 0.8660254037844387076, 1.000000000000000000, 0.8660254037844387076, 1.000000000000000000, 0.8660254037844387076, 1.000000000000000000, 0.8660254037844387076, 1.000000000000000000, 0.8660254037844387076, 1.000000000000000000, 0.8660254037844387076, 1.000000000000000000, 0.8660254037844387076, 1.000000000000000000, 0.8660254037844387076, 1.000000000000000000, 0.8660254037844387076, 1.000000000000000000, 0.8660254037844387076, 1.000000000000000000, 0.8660254037844387076, 1.000000000000000000, 0.8660254037844387076, 1.000000000000000000, 0.8660254037844387076, 1.000000000000000000, 0.8660254037844387076, 1.000000000000000000, 0.8660254037844387076, 1.000000000000000000, 0.8660254037844387076, 1.000000000000000000, 0.8660254037844387076, 1.000000000000000000, 0.8660254037844387076, 1.000000000000000000, 0.8660254037844387076, 1.000000000000000000, 0.8660254037844387076, 1.000000000000000000, 0.8660254037844387076, 1.000000000000000000, 0.8660254037844387076, 1.000000000000000000, 0.8660254037844387076, 1.000000000000000000, 0.8660254037844387076, 1.000000000000000000, 0.8660254037844387076, 1.000000000000000000, 0.8660254037844387076, 1.000000000000000000, 0.8660254037844387076, 1.000000000000000000, 0.8660254037844387076, 1.000000000000000000, 0.8660254037844387076, 1.000000000000000000, 0.8660254037844387076, 1.000000000000000000, 0.8660254037844387076, 1.000000000000000000, 0.8660254037844387076, 1.000000000000000000, 0.8660254037844387076, 1.000000000000000000, 0.8660254037844387076, 1.000000000000000000, 0.8660254037844387076, 1.000000000000000000, 0.8660254037844387076, 1.000000000000000000, 0.8660254037844387076, 1.000000000000000000, 0.8660254037844387076, 1.000000000000000000, 0.8660254037844387076, 1.000000000000000000, 0.8660254037844387076, 1.000000000000000000, 0.8660254037844387076, 1.000000000000000000, 0.8660254037844387076, 1.000000000000000000, 0.8660254037844387076, 1.000000000000000000, 0.8660254037844387076, 1.000000000000000000, 0.8660254037844387076, 1.000000000000000000, 0.8660254037844387076, 1.000000000000000000, 0.8660254037844387076, 1.000000000000000000, 0.8660254037844387076, 1.000000000000000000, 0.8660254037844387076, 1.000000000000000000, 0.8660254037844387076, 1.000000000000000000, 0.8660254037844387076, 1.000000000000000000, 0.8660254037844387076, 1.000000000000000000, 0.8660254037844387076, 1.000000000000000000, 0.8660254037844387076, 1.000000000000000000, 0.8660254037844387076, 1.000000000000000000, 0.8660254037844387076, 1.000000000000000000, 0.8660254037844387076, 1.000000000000000000, 0.8660254037844387076, 1.000000000000000000, 0.8660254037844387076, 1.000000000000000000, 0.8660254037844387076, 1.000000000000000000, 0.8660254037844387076, 1.000000000000000000, 0.8660254037844387076, 1.000000000000000000, 0.8660254037844387076, 1.000000000000000000, 0.8660254037844387076, 1.000000000000000000, 0.8660254037844387076, 1.000000000000000000, 0.8660254037844387076, 1.000000000000000000, 0.8660254037844387076, 1.000000000000000000, 0.8660254037844387076, 1.000000000000000000, 0.8660254037844387076, 1.000000000000000000, 0.8660254037844387076, 1.000000000000000000, 0.8660254037844387076, 1.000000000000000000, 0.8660254037844387076, 1.000000000000000000, 0.8660254037844387076, 1.000000000000000000, 0.8660254037844387076, 1.000000000000000000, 0.8660254037844387076, 1.000000000000000000, 0.8660254037844387076, 1.000000000000000000, 0.8660254037844387076, 1.000000000000000000, 0.8660254037844387076, 1.000000000000000000, 0.8660254037844387076, 1.000000000000000000, 0.8660254037844387076, 1.000000000000000000, 0.8660254037844387076, 1.000000000000000000, 0.8660254037844387076, 1.000000000000000000, 0.8660254037844387076, 1.000000000000000000, 0.8660254037844387076, 1.000000000000000000, 0.8660254037844387076, 1.000000000000000000, 0.8660254037844387076, 1.000000000000000000, 0.8660254037844387076, 1.000000000000000000, 0.8660254037844387076, 1.000000000000000000, 0.8660254037844387076, 1.000000000000000000, 0.8660254037844387076, 1.000000000000000000, 0.8660254037844387076, 1.000000000000000000, 0.8660254037844387076, 1.000000000000000000, 0.8660254037844387076, 1.000000000000000000, 0.8660254037844387076, 1.000000000000000000, 0.8660254037844387076, 1.000000000000000000, 0.8660254037844387076, 1.000000000000000000, 0.8660254037844387076, 1.000000000000000000, 0.8660254037844387076, 1.000000000000000000, 0.8660254037844387076, 1.000000000000000000, 0.8660254037844387076, 1.000000000000000000, 0.8660254037844387076, 1.000000000000000000, 0.8660254037844387076, 1.000000000000000000, 0.8660254037844387076, 1.000000000000000000, 0.8660254037844387076, 1.000000000000000000, 0.8660254037844387076, 1.000000000000000000, 0.8660254037844387076, 1.000000000000000000, 0.8660254037844387076, 1.000000000000000000, 0.8660254037844387076, 1.000000000000000000, 0.8660254037844387076, 1.000000000000000000, 0.8660254037844387076, 1.000000000000000000, 0.8660254037844387076, 1.000000000000000000, 0.8660254037844387076, 1.000000000000000000, 0.8660254037844387076, 1.000000000000000000, 0.8660254037844387076, 1.000000000000000000, 0.8660254037844387076, 1.000000000000000000, 0.8660254037844387076, 1.000000000000000000, 0.8660254037844387076, 1.000000000000000000, 0.8660254037844387076, 1.000000000000000000, 0.8660254037844387076, 1.000000000000000000, 0.8660254037844387076, 1.000000000000000000, 0.8660254037844387076, 1.000000000000000000, 0.8660254037844387076, 1.000000000000000000, 0.8660254037844387076, 1.000000000000000000, 0.8660254037844387076, 1.000000000000000000, 0.8660254037844387076, 1.000000000000000000, 0.8660254037844387076, 1.000000000000000000, 0.8660254037844387076, 1.000000000000000000, 0.8660254037844387076, 1.000000000000000000, 0.8660254037844387076, 1.000000000000000000, 0.8660254037844387076, 1.000000000000000000, 0.8660254037844387076, 1.000000000000000000, 0.8660254037844387076, 1.000000000000000000, 0.8660254037844387076, 1.000000000000000000, 0.8660254037844387076, 1.000000000000000000, 0.8660254037844387076, 1.000000000000000000, 0.8660254037844387076, 1.000000000000000000, 0.8660254037844387076, 1.000000000000000000, 0.8660254037844387076, 1.000000000000000000, 0.8660254037844387076, 1.000000000000000000, 0.8660254037844387076, 1.000000000000000000, 0.9024573129378109515, 0.9469501470576147106),
 ( 1.000000000000000000, 0.8660254037844387076, 1.000000000000000000, 0.8660254037844387076, 1.000000000000000000, 0.8660254037844387076, 1.000000000000000000, 0.8660254037844387076, 1.000000000000000000, 0.8660254037844387076, 1.000000000000000000, 0.8660254037844387076, 1.000000000000000000, 0.8660254037844387076, 1.000000000000000000, 0.8660254037844387076, 1.000000000000000000, 0.8660254037844387076, 1.000000000000000000, 0.8660254037844387076, 1.000000000000000000, 0.8660254037844387076, 1.000000000000000000, 0.8660254037844387076, 1.000000000000000000, 0.8660254037844387076, 1.000000000000000000, 0.8660254037844387076, 1.000000000000000000, 0.8660254037844387076, 1.000000000000000000, 0.8660254037844387076, 1.000000000000000000, 0.8660254037844387076, 1.000000000000000000, 0.8660254037844387076, 1.000000000000000000, 0.8660254037844387076, 1.000000000000000000, 0.8660254037844387076, 1.000000000000000000, 0.8660254037844387076, 1.000000000000000000, 0.8660254037844387076, 1.000000000000000000, 0.8660254037844387076, 1.000000000000000000, 0.8660254037844387076, 1.000000000000000000, 0.8660254037844387076, 1.000000000000000000, 0.8660254037844387076, 1.000000000000000000, 0.8660254037844387076, 1.000000000000000000, 0.8660254037844387076, 1.000000000000000000, 0.8660254037844387076, 1.000000000000000000, 0.8660254037844387076, 1.000000000000000000, 0.8660254037844387076, 1.000000000000000000, 0.8660254037844387076, 1.000000000000000000, 0.8660254037844387076, 1.000000000000000000, 0.8660254037844387076, 1.000000000000000000, 0.8660254037844387076, 1.000000000000000000, 0.8660254037844387076, 1.000000000000000000, 0.8660254037844387076, 1.000000000000000000, 0.8660254037844387076, 1.000000000000000000, 0.8660254037844387076, 1.000000000000000000, 0.8660254037844387076, 1.000000000000000000, 0.8660254037844387076, 1.000000000000000000, 0.8660254037844387076, 1.000000000000000000, 0.8660254037844387076, 1.000000000000000000, 0.8660254037844387076, 1.000000000000000000, 0.8660254037844387076, 1.000000000000000000, 0.8660254037844387076, 1.000000000000000000, 0.8660254037844387076, 1.000000000000000000, 0.8660254037844387076, 1.000000000000000000, 0.8660254037844387076, 1.000000000000000000, 0.8660254037844387076, 1.000000000000000000, 0.8660254037844387076, 1.000000000000000000, 0.8660254037844387076, 1.000000000000000000, 0.8660254037844387076, 1.000000000000000000, 0.8660254037844387076, 1.000000000000000000, 0.8660254037844387076, 1.000000000000000000, 0.8660254037844387076, 1.000000000000000000, 0.8660254037844387076, 1.000000000000000000, 0.8660254037844387076, 1.000000000000000000, 0.8660254037844387076, 1.000000000000000000, 0.8660254037844387076, 1.000000000000000000, 0.8660254037844387076, 1.000000000000000000, 0.8660254037844387076, 1.000000000000000000, 0.8660254037844387076, 1.000000000000000000, 0.8660254037844387076, 1.000000000000000000, 0.8660254037844387076, 1.000000000000000000, 0.8660254037844387076, 1.000000000000000000, 0.8660254037844387076, 1.000000000000000000, 0.8660254037844387076, 1.000000000000000000, 0.8660254037844387076, 1.000000000000000000, 0.8660254037844387076, 1.000000000000000000, 0.8660254037844387076, 1.000000000000000000, 0.8660254037844387076, 1.000000000000000000, 0.8660254037844387076, 1.000000000000000000, 0.8660254037844387076, 1.000000000000000000, 0.8660254037844387076, 1.000000000000000000, 0.8660254037844387076, 1.000000000000000000, 0.8660254037844387076, 1.000000000000000000, 0.8660254037844387076, 1.000000000000000000, 0.8660254037844387076, 1.000000000000000000, 0.8660254037844387076, 1.000000000000000000, 0.8660254037844387076, 1.000000000000000000, 0.8660254037844387076, 1.000000000000000000, 0.8660254037844387076, 1.000000000000000000, 0.8660254037844387076, 1.000000000000000000, 0.8660254037844387076, 1.000000000000000000, 0.8660254037844387076, 1.000000000000000000, 0.8660254037844387076, 1.000000000000000000, 0.8660254037844387076, 1.000000000000000000, 0.8660254037844387076, 1.000000000000000000, 0.8660254037844387076, 1.000000000000000000, 0.8660254037844387076, 1.000000000000000000, 0.8660254037844387076, 1.000000000000000000, 0.8660254037844387076, 1.000000000000000000, 0.8660254037844387076, 1.000000000000000000, 0.8660254037844387076, 1.000000000000000000, 0.8660254037844387076, 1.000000000000000000, 0.8660254037844387076, 1.000000000000000000, 0.8660254037844387076, 1.000000000000000000, 0.8660254037844387076, 1.000000000000000000, 0.8660254037844387076, 1.000000000000000000, 0.8660254037844387076, 1.000000000000000000, 0.8660254037844387076, 1.000000000000000000, 0.8660254037844387076, 1.000000000000000000, 0.8660254037844387076, 1.000000000000000000, 0.8660254037844387076, 1.000000000000000000, 0.8660254037844387076, 1.000000000000000000, 0.8660254037844387076, 1.000000000000000000, 0.8660254037844387076, 1.000000000000000000, 0.8660254037844387076, 1.000000000000000000, 0.8660254037844387076, 1.000000000000000000, 0.8660254037844387076, 1.000000000000000000, 0.8660254037844387076, 1.000000000000000000, 0.8660254037844387076, 1.000000000000000000, 0.8660254037844387076, 1.000000000000000000, 0.8660254037844387076, 1.000000000000000000, 0.8660254037844387076, 1.000000000000000000, 0.8660254037844387076, 1.000000000000000000, 0.8660254037844387076, 1.000000000000000000, 0.8660254037844387076, 1.000000000000000000, 0.8660254037844387076, 1.000000000000000000, 0.8660254037844387076, 1.000000000000000000, 0.8660254037844387076, 1.000000000000000000, 0.8660254037844387076, 1.000000000000000000, 0.8660254037844387076, 1.000000000000000000, 0.8660254037844387076, 1.000000000000000000, 0.8660254037844387076, 1.000000000000000000, 0.8660254037844387076, 1.000000000000000000, 0.8660254037844387076, 1.000000000000000000, 0.8660254037844387076, 1.000000000000000000, 0.8660254037844387076, 1.000000000000000000, 0.8660254037844387076, 1.000000000000000000, 0.8660254037844387076, 1.000000000000000000, 0.8660254037844387076, 1.000000000000000000, 0.8660254037844387076, 1.000000000000000000, 0.8660254037844387076, 1.000000000000000000, 0.8660254037844387076, 1.000000000000000000, 0.8660254037844387076, 1.000000000000000000, 0.8660254037844387076, 1.000000000000000000, 0.8660254037844387076, 1.000000000000000000, 0.8660254037844387076, 1.000000000000000000, 0.8660254037844387076, 1.000000000000000000, 0.9024573129378109515, 0.9469501470576147106) ) ) 
 REPRESENTATION_ITEM ( '' )  SURFACE ( )  );
#33869=CARTESIAN_POINT ( 'NONE',  ( -92.69370383062498320, -209.9999999999999716, 87.42031250086714067 ) ) ;
#33875=CARTESIAN_POINT ( 'NONE',  ( -92.69370383062498320, -209.9999999999999716, 75.35531250086714294 ) ) ;
#33886=CARTESIAN_POINT ( 'NONE',  ( -97.30629616937501680, 88.66845928578038638, 83.34572916753380412 ) ) ;
#33891=CARTESIAN_POINT ( 'NONE',  ( -92.34999999999999432, -210.0000000983656605, 80.23687499810813506 ) ) ;
#33900=CARTESIAN_POINT ( 'NONE',  ( -97.30629616937497417, -211.3315407142195852, 79.69447916753381378 ) ) ;
#33904=CARTESIAN_POINT ( 'NONE',  ( 97.64999999999996305, -209.9999996502043018, 77.69687501385438111 ) ) ;
#33907=DIRECTION ( 'NONE',  ( -0.000000000000000000, -0.000000000000000000, 1.000000000000000000 ) ) ;
#33934=CARTESIAN_POINT ( 'NONE',  ( 96.32499999999998863, 87.70503267997126784, 87.67166666666666686 ) ) ;
#33935=FACE_OUTER_BOUND ( 'NONE', #26566, .T. ) ;
#33941=CARTESIAN_POINT ( 'NONE',  ( 97.30629616937498838, 90.00000000000002842, 84.88031250086713442 ) ) ;
#33944=CARTESIAN_POINT ( 'NONE',  ( 92.69370383062501162, -211.3315407142195852, 85.88572916753382458 ) ) ;
#33950=CARTESIAN_POINT ( 'NONE',  ( -96.32500000000001705, 87.70503267997129626, 79.31083333333333485 ) ) ;
#33952=CARTESIAN_POINT ( 'NONE',  ( -93.84685191531248449, -208.0026889286704943, 86.25614583420048120 ) ) ;
#33953=CARTESIAN_POINT ( 'NONE',  ( -97.30629616937501680, 90.00000000000004263, 85.99156250086716113 ) ) ;
#33955=CARTESIAN_POINT ( 'NONE',  ( 97.30629616937498838, 88.66845928578037217, 82.92239583420045790 ) ) ;
#33956=CARTESIAN_POINT ( 'NONE',  ( -92.69370383062502583, 88.66845928578038638, 84.19239583420046813 ) ) ;
#33959=EDGE_CURVE ( 'NONE', #11821, #47514, #67404, .T. ) ;
#33960=CARTESIAN_POINT ( 'NONE',  ( -94.99999999999997158, -213.0599564267049857, 80.71312500173429783 ) ) ;
#33963=CARTESIAN_POINT ( 'NONE',  ( -92.69370383062498320, -208.6684592857803295, 88.10822916753380696 ) ) ;
#33964=CARTESIAN_POINT ( 'NONE',  ( -92.34999999999996589, -211.5299782133524502, 82.00958333333333883 ) ) ;
#33969=VERTEX_POINT ( 'NONE', #74151 ) ;
#33970=CARTESIAN_POINT ( 'NONE',  ( -96.32500000000001705, 92.29496732002878900, 78.46416666666667084 ) ) ;
#33973=ADVANCED_FACE ( 'NONE', ( #33935 ), #28283, .F. ) ;
#33975=CARTESIAN_POINT ( 'NONE',  ( -92.35000000000306386, -210.0000040461925437, 77.06187486178056645 ) ) ;
#33981=CARTESIAN_POINT ( 'NONE',  ( -96.15314808468751551, 88.00268892867056536, 79.58864583420047722 ) ) ;
#33990=( BOUNDED_CURVE ( )  B_SPLINE_CURVE ( 2, ( #26317, #66188, #54890, #9391, #53778, #2701, #65813 ),
 .UNSPECIFIED., .F., .F. ) 
 B_SPLINE_CURVE_WITH_KNOTS ( ( 3, 2, 2, 3 ),
 ( 0.7408554641864679713, 0.7479111473335298133, 0.7549669128744131985, 0.7620226289464459013 ),
 .UNSPECIFIED. ) 
 CURVE ( )  GEOMETRIC_REPRESENTATION_ITEM ( )  RATIONAL_B_SPLINE_CURVE ( ( 0.9999968710553057694, 0.8660269682750552089, 1.000000000000000000, 0.8660254037844387076, 1.000000000000000000, 0.8660263430970122078, 0.9999981213880242414 ) ) 
 REPRESENTATION_ITEM ( '' )  );
#33993=CARTESIAN_POINT ( 'NONE',  ( 93.84685191531248449, 88.00268892867053694, 78.47739583420049314 ) ) ;
#33994=CARTESIAN_POINT ( 'NONE',  ( -92.69370383062498320, -211.3315407142195852, 80.54114583420049200 ) ) ;
#33996=EDGE_LOOP ( 'NONE', ( #14665, #17291, #40321, #13108, #56651, #29111 ) ) ;
#34001=CARTESIAN_POINT ( 'NONE',  ( -97.30629616937501680, 91.33154071421968467, 77.04864583420048518 ) ) ;
#34002=CARTESIAN_POINT ( 'NONE',  ( 95.00000000000000000, -212.6630814284392557, 79.64156250086713840 ) ) ;
#34006=FACE_OUTER_BOUND ( 'NONE', #61942, .T. ) ;
#34007=ORIENTED_EDGE ( 'NONE', *, *, #68354, .F. ) ;
#34008=CARTESIAN_POINT ( 'NONE',  ( 92.34999999999999432, 90.00000000000002842, 90.00000000000000000 ) ) ;
#34013=CARTESIAN_POINT ( 'NONE',  ( 97.30629616937498838, -208.6684592857803295, 76.20197916753382117 ) ) ;
#34018=AXIS2_PLACEMENT_3D ( 'NONE', #71608, #12982, #65256 ) ;
#34020=CARTESIAN_POINT ( 'NONE',  ( 93.84685191531248449, 88.00268892867053694, 84.19239583420049655 ) ) ;
#34021=CARTESIAN_POINT ( 'NONE',  ( 97.64999999999999147, -209.9999999999999716, 78.88750000000000284 ) ) ;
#34024=LINE ( 'NONE', #45439, #24463 ) ;
#34031=CARTESIAN_POINT ( 'NONE',  ( 92.34999999999999432, 90.00000000000002842, 83.65000000000000568 ) ) ;
#34035=CYLINDRICAL_SURFACE ( 'NONE', #60829, 2.649999999999999467 ) ;
#34037=CARTESIAN_POINT ( 'NONE',  ( -97.64999999999996305, -209.9999999999999716, 83.72937500173429726 ) ) ;
#34040=ORIENTED_EDGE ( 'NONE', *, *, #22748, .F. ) ;
#34041=CARTESIAN_POINT ( 'NONE',  ( 97.64999999999997726, 91.52997821335252127, 78.38479166840096468 ) ) ;
#34042=CARTESIAN_POINT ( 'NONE',  ( -96.32500000000001705, 87.70503267997129626, 80.66020833506763665 ) ) ;
#34045=CARTESIAN_POINT ( 'NONE',  ( 93.84685191531248449, 88.00268892867053694, 83.55739583420049144 ) ) ;
#34049=CARTESIAN_POINT ( 'NONE',  ( 97.64999999999999147, 90.00000000000002842, 90.00000000000000000 ) ) ;
#34054=CARTESIAN_POINT ( 'NONE',  ( -95.00000000000002842, 90.00000000000004263, 90.00000000000000000 ) ) ;
#34067=CARTESIAN_POINT ( 'NONE',  ( -93.84685191531247028, -211.9973110713294489, 81.75822916753382685 ) ) ;
#34072=CARTESIAN_POINT ( 'NONE',  ( -95.29566955672730444, -212.6272429001226953, 74.99300273738367650 ) ) ;
#34074=CARTESIAN_POINT ( 'NONE',  ( 93.84685191531248449, 88.00268892867053694, 75.14364583420046984 ) ) ;
#34081=( BOUNDED_CURVE ( )  B_SPLINE_CURVE ( 2, ( #21715, #45412, #5567, #28842, #22095, #45034, #67958, #28096, #16453 ),
 .UNSPECIFIED., .F., .F. ) 
 B_SPLINE_CURVE_WITH_KNOTS ( ( 3, 2, 2, 2, 3 ),
 ( 0.4868478063929145838, 0.4939035878617654696, 0.5009593534026473005, 0.5080151189435291315, 0.5080151867253829279 ),
 .UNSPECIFIED. ) 
 CURVE ( )  GEOMETRIC_REPRESENTATION_ITEM ( )  RATIONAL_B_SPLINE_CURVE ( ( 1.000000000000000000, 0.8660254037844387076, 1.000000000000000000, 0.8660254037844387076, 1.000000000000000000, 0.8660254037844387076, 1.000000000000000000, 0.9999987129608483016, 0.9999974259464248227 ) ) 
 REPRESENTATION_ITEM ( '' )  );
#34082=CARTESIAN_POINT ( 'NONE',  ( 96.15314808468748708, 88.00268892867053694, 86.83822916753382515 ) ) ;
#34084=CARTESIAN_POINT ( 'NONE',  ( -96.15314808468745866, -211.9973110713294489, 89.27239583420049485 ) ) ;
#34088=CARTESIAN_POINT ( 'NONE',  ( -97.30629616937501680, 91.33154071421968467, 78.79489583420047438 ) ) ;
#34089=CIRCLE ( 'NONE', #54529, 3.299999999999997158 ) ;
#34093=ORIENTED_EDGE ( 'NONE', *, *, #69046, .F. ) ;
#34099=ADVANCED_FACE ( 'NONE', ( #16643 ), #73776, .F. ) ;
#34112=CARTESIAN_POINT ( 'NONE',  ( 92.35000000000002274, -211.5299782133524502, 88.78291666666667936 ) ) ;
#34116=ORIENTED_EDGE ( 'NONE', *, *, #2237, .T. ) ;
#34123=CARTESIAN_POINT ( 'NONE',  ( 97.64999999999997726, -208.4700217866474645, 77.74979166840097378 ) ) ;
#34124=CARTESIAN_POINT ( 'NONE',  ( 94.99999999999998579, 93.05995642670504253, 82.22124999999999773 ) ) ;
#34126=DIRECTION ( 'NONE',  ( 1.000000000000000000, 0.000000000000000000, 0.000000000000000000 ) ) ;
#34128=DIRECTION ( 'NONE',  ( -0.000000000000000000, -0.000000000000000000, 1.000000000000000000 ) ) ;
#34132=CARTESIAN_POINT ( 'NONE',  ( 92.35002600533567829, 88.47000677245996769, 84.41729270697884147 ) ) ;
#34133=CARTESIAN_POINT ( 'NONE',  ( -92.69370383062505425, 91.33154071421968467, 80.64697916753382856 ) ) ;
#34134=CARTESIAN_POINT ( 'NONE',  ( 93.84685191531248449, 91.99731107132950569, 76.83697916753381207 ) ) ;
#34135=EDGE_CURVE ( 'NONE', #18610, #28278, #64321, .T. ) ;
#34140=CARTESIAN_POINT ( 'NONE',  ( -94.99999999999997158, -206.9400435732949575, 77.77624999999999034 ) ) ;
#34143=EDGE_CURVE ( 'NONE', #51953, #47366, #59554, .T. ) ;
#34144=CARTESIAN_POINT ( 'NONE',  ( -97.30629616937497417, -208.6684592857803011, 78.79489583420047438 ) ) ;
#34155=CARTESIAN_POINT ( 'NONE',  ( -97.30629616937495996, -209.9999999999999716, 76.94281250086713442 ) ) ;
#34160=CARTESIAN_POINT ( 'NONE',  ( 92.35000000003358878, -210.0000076551254153, 78.01464417100928017 ) ) ;
#34161=CARTESIAN_POINT ( 'NONE',  ( 100.0010000000000190, -115.9999999999999716, -40.00000000000002132 ) ) ;
#34167=CARTESIAN_POINT ( 'NONE',  ( 97.30629616937498838, 88.66845928578035796, 85.46239583420044994 ) ) ;
#34174=CARTESIAN_POINT ( 'NONE',  ( -97.64999999980591383, 89.99998015682162134, 84.36502760998403971 ) ) ;
#34180=LINE ( 'NONE', #16897, #14515 ) ;
#34183=CARTESIAN_POINT ( 'NONE',  ( -93.67499999999998295, -212.2949673200287179, 83.22666666666665947 ) ) ;
#34191=CARTESIAN_POINT ( 'NONE',  ( 97.30629616937498838, -211.3315407142195852, 84.35114583420049428 ) ) ;
#34193=ORIENTED_EDGE ( 'NONE', *, *, #68089, .F. ) ;
#34200=CARTESIAN_POINT ( 'NONE',  ( 95.00000000000000000, -212.6630814284392557, 77.73656250086713726 ) ) ;
#34203=CARTESIAN_POINT ( 'NONE',  ( 97.30629616937498838, -209.9999999999999716, 83.76906250086716454 ) ) ;
#34212=CARTESIAN_POINT ( 'NONE',  ( 97.65000000000009095, 91.52997821335247863, 85.92541666666664923 ) ) ;
#34213=CARTESIAN_POINT ( 'NONE',  ( 97.64999999999997726, -211.5299782133524502, 85.26395833506762756 ) ) ;
#34214=ADVANCED_FACE ( 'NONE', ( #3450 ), #3086, .F. ) ;
#34217=VERTEX_POINT ( 'NONE', #42541 ) ;
#34222=ORIENTED_EDGE ( 'NONE', *, *, #63245, .F. ) ;
#34233=CARTESIAN_POINT ( 'NONE',  ( -96.32500000000001705, 87.70503267997129626, 88.20083333333332121 ) ) ;
#34235=EDGE_CURVE ( 'NONE', #44854, #29642, #529, .T. ) ;
#34236=CARTESIAN_POINT ( 'NONE',  ( 97.30629616937498838, 90.00000000000002842, 74.72031250086713783 ) ) ;
#34239=CARTESIAN_POINT ( 'NONE',  ( -97.30629616937497417, -211.3315407142195852, 84.61572916753380014 ) ) ;
#34244=CARTESIAN_POINT ( 'NONE',  ( -92.69370383062498320, -209.9999999999999716, 77.26031250086714408 ) ) ;
#34245=CARTESIAN_POINT ( 'NONE',  ( -92.35000000000003695, 89.99999989488615881, 86.58687499784845443 ) ) ;
#34246=DIRECTION ( 'NONE',  ( -0.000000000000000000, -0.000000000000000000, 1.000000000000000000 ) ) ;
#34251=CARTESIAN_POINT ( 'NONE',  ( -97.30629616937501680, 91.33154071421968467, 78.79489583420047438 ) ) ;
#34262=FACE_OUTER_BOUND ( 'NONE', #1180, .T. ) ;
#34263=CARTESIAN_POINT ( 'NONE',  ( -94.99999999999997158, -212.6630814284392557, 80.43531250086715545 ) ) ;
#34269=CARTESIAN_POINT ( 'NONE',  ( 93.67499999999998295, 92.29496732002878900, 76.63854166840096127 ) ) ;
#34281=( BOUNDED_SURFACE ( )  B_SPLINE_SURFACE ( 1, 2, ( 
 ( #41413, #35404, #47065, #48163, #64720, #6825, #29737, #7933, #36134, #52693, #59083, #24134, #64354, #12827, #19212, #69967, #42162, #65466, #35753, #30849, #7202, #25237, #70329, #65096, #71073, #13930, #47785, #19575, #58704, #42523, #7571, #36871, #59820, #49263, #65827, #21418, #20695, #61666, #61300, #66921, #4167, #9409, #66570, #48888, #54906, #42900, #72188, #43647, #32336, #27437, #71444, #54539, #10153, #19943, #9044, #60201, #3068, #25963, #9788, #15050, #15415, #26694, #15803, #27064, #14314, #37261, #4539, #8684, #31964, #31595, #71812, #44377, #44007, #43283, #14682, #60919, #32701, #20325, #37988, #66206, #33076, #55279, #55647, #3428, #26336, #56019, #67304, #37630, #60566, #49995, #38363, #3799, #49621, #21057, #72551, #38738, #72914, #68434, #34566, #10908, #51122, #51867, #63169, #6387, #56778, #49, #16537, #22941, #22186, #45881, #410, #45127, #68802, #57885, #34203, #62807, #4916, #50374, #74046, #46231, #73295, #50745, #68046, #17283, #63532, #62431, #40217, #21808, #45503, #33831, #5287, #44756, #56409, #57514, #28188, #11626, #62044, #6027, #39484, #69165, #67679, #12009, #22557, #28929, #16922, #11269, #23303, #57150, #17655, #40587, #39860, #5656, #16168, #73670, #34945, #39107, #10521, #28549, #51488, #33446, #27816, #30397, #59729, #65004, #48075, #70985, #24046, #47698, #59357, #775, #35667, #1147, #69524, #13486, #7484, #53708, #1517, #12372, #36046, #46969, #12739, #58606, #7107, #13841, #41686, #36410, #24767, #70608, #13109, #1880, #7846, #30761, #2249, #19125, #19487, #25144, #58992, #52230, #53341, #18025, #24400, #42073, #42438, #40965, #65375, #52592, #30031, #36783, #29289, #23660, #35317, #46596, #18749, #63901, #58245, #6744, #52975, #29650, #69882, #18378, #41325, #64266, #64624, #47335, #70240, #72469, #32240, #60478, #43924, #43192, #54449, #4081, #66844, #2625, #32617, #55562, #38269, #61212, #72102, #49175, #26609, #8593, #26236, #72828, #71723, #20224, #20610, #60836, #48436, #44284, #21330, #19856, #49543, #8958, #43565, #55190, #31508, #31140, #37170, #9701, #31876, #15715, #8209, #20972, #54820, #67213, #3346, #38650, #2979, #25872, #9318, #54094, #3715, #26978, #48804, #15327, #66118, #49908, #14591, #25505, #71351, #42806, #14967, #66481, #37543, #65736, #37906 ),
 ( #14216, #60115, #67959, #51779, #34479, #50280, #73210, #22850, #5568, #73583, #68338, #11182, #39769, #11543, #68713, #5195, #45791, #22096, #62334, #63085, #74337, #17561, #16454, #34112, #27731, #57059, #33355, #28464, #57422, #56313, #51397, #69074, #45413, #73956, #16082, #61581, #10818, #5934, #10065, #61953, #4830, #17199, #324, #45035, #40129, #32986, #56689, #39394, #33744, #55933, #67588, #28843, #28097, #23218, #21716, #46145, #50655, #4450, #27348, #44671, #51035, #39018, #22470, #16831, #10436, #62716, #19034, #7401, #69798, #47250, #70903, #63813, #30314, #53258, #63444, #1058, #24319, #46887, #29940, #18296, #34856, #64916, #64181, #30677, #1795, #35955, #47612, #52890, #35585, #17933, #23950, #11913, #41237, #12653, #1435, #40495, #57796, #23572, #53620, #6299, #52501, #29198, #46505, #69434, #24680, #58520, #58906, #70157, #59271, #70520, #52141, #685, #47991, #40877, #7015, #12284, #35222, #13398, #13021, #58156, #6655, #36327, #29562, #64541, #18661, #41600, #25051, #41985, #7765, #2164, #32533, #8873, #15247, #3627, #25429, #2896, #49459, #42719, #2545, #72383, #3989, #31787, #8123, #60391, #9233, #43482, #71642, #55101, #54368, #65652, #38180, #26526, #13763, #43841, #66758, #20887, #61126, #54734, #3260, #37825, #19770, #37461, #9616, #8508, #31428, #26151, #72013, #59640, #55478, #26893, #31052, #60755, #20138, #49089, #66399, #14125, #42352, #48351, #49821, #43102, #19404, #65291, #32155, #66030, #36699, #14503, #54005, #37076, #60026, #20523, #71265, #14881, #25790, #48720, #68248, #61865, #16745, #10350, #73869, #11099, #68626, #5108, #56604, #73123, #39681, #44580, #33265, #15988, #22378, #28751, #34021, #17110, #40040, #67501, #62622, #28377, #44198, #4741, #38931, #38561, #56971, #50946, #22764, #44950, #55848, #28006, #56222, #27643, #50568, #73497, #57331, #10729, #5479, #51308, #74241, #45323, #45700, #62999, #11458, #34390, #5842, #72743, #21243, #67124, #15629, #61497, #9975, #67872, #32895, #4359, #27257, #50187, #21627, #22004, #16363, #39306, #62238, #33651, #40403, #1347, #596, #58069, #36242, #30231, #18941, #34771, #64831, #41154, #47531, #35862, #57707, #35136, #7312, #23487, #6215, #53172, #59185, #64094, #63352, #18213, #41517, #24239, #29477, #12928, #12195, #46419, #70435 ) ),
 .UNSPECIFIED., .F., .F., .F. ) 
 B_SPLINE_SURFACE_WITH_KNOTS ( ( 2, 2 ),
 ( 3, 2, 2, 2, 2, 2, 2, 2, 2, 2, 2, 2, 2, 2, 2, 2, 2, 2, 2, 2, 2, 2, 2, 2, 2, 2, 2, 2, 2, 2, 2, 2, 2, 2, 2, 2, 2, 2, 2, 2, 2, 2, 2, 2, 2, 2, 2, 2, 2, 2, 2, 2, 2, 2, 2, 2, 2, 2, 2, 2, 2, 2, 2, 2, 2, 2, 2, 2, 2, 2, 2, 2, 2, 2, 2, 2, 2, 2, 2, 2, 2, 2, 2, 2, 2, 2, 2, 2, 2, 2, 2, 2, 2, 2, 2, 2, 2, 2, 2, 2, 2, 2, 2, 2, 2, 2, 2, 2, 2, 2, 2, 2, 2, 2, 2, 2, 2, 2, 2, 2, 2, 2, 2, 2, 2, 2, 2, 2, 2, 2, 2, 2, 2, 2, 2, 2, 2, 2, 2, 2, 2, 2, 2, 3 ),
 ( 0.000000000000000000, 1.000000000000000000 ),
 ( 0.000000000000000000, 0.006944444444444444059, 0.01388888888888888812, 0.02083333333333333218, 0.02777777777777777624, 0.03472222222222222376, 0.04166666666666666435, 0.04861111111111111188, 0.05555555555555555247, 0.06250000000000000000, 0.06944444444444444753, 0.07638888888888889506, 0.08333333333333332871, 0.09027777777777777624, 0.09722222222222222376, 0.1041666666666666713, 0.1111111111111111049, 0.1180555555555555525, 0.1250000000000000000, 0.1319444444444444475, 0.1388888888888888951, 0.1458333333333333426, 0.1527777777777777901, 0.1597222222222222099, 0.1666666666666666574, 0.1736111111111111049, 0.1805555555555555525, 0.1875000000000000000, 0.1944444444444444475, 0.2013888888888888951, 0.2083333333333333426, 0.2152777777777777901, 0.2222222222222222099, 0.2291666666666666574, 0.2361111111111111049, 0.2430555555555555525, 0.2500000000000000000, 0.2569444444444444198, 0.2638888888888888951, 0.2708333333333333148, 0.2777777777777777901, 0.2847222222222222099, 0.2916666666666666852, 0.2986111111111111049, 0.3055555555555555802, 0.3125000000000000000, 0.3194444444444444198, 0.3263888888888888951, 0.3333333333333333148, 0.3402777777777777901, 0.3472222222222222099, 0.3541666666666666852, 0.3611111111111111049, 0.3680555555555555802, 0.3750000000000000000, 0.3819444444444444198, 0.3888888888888888951, 0.3958333333333333148, 0.4027777777777777901, 0.4097222222222222099, 0.4166666666666666852, 0.4236111111111111049, 0.4305555555555555802, 0.4375000000000000000, 0.4444444444444444198, 0.4513888888888888951, 0.4583333333333333148, 0.4652777777777777901, 0.4722222222222222099, 0.4791666666666666852, 0.4861111111111111049, 0.4930555555555555802, 0.5000000000000000000, 0.5069444444444444198, 0.5138888888888888395, 0.5208333333333333703, 0.5277777777777777901, 0.5347222222222222099, 0.5416666666666666297, 0.5486111111111111605, 0.5555555555555555802, 0.5625000000000000000, 0.5694444444444444198, 0.5763888888888888395, 0.5833333333333333703, 0.5902777777777777901, 0.5972222222222222099, 0.6041666666666666297, 0.6111111111111111605, 0.6180555555555555802, 0.6250000000000000000, 0.6319444444444444198, 0.6388888888888888395, 0.6458333333333333703, 0.6527777777777777901, 0.6597222222222222099, 0.6666666666666666297, 0.6736111111111111605, 0.6805555555555555802, 0.6875000000000000000, 0.6944444444444444198, 0.7013888888888888395, 0.7083333333333333703, 0.7152777777777777901, 0.7222222222222222099, 0.7291666666666666297, 0.7361111111111111605, 0.7430555555555555802, 0.7500000000000000000, 0.7569444444444444198, 0.7638888888888888395, 0.7708333333333333703, 0.7777777777777777901, 0.7847222222222222099, 0.7916666666666666297, 0.7986111111111111605, 0.8055555555555555802, 0.8125000000000000000, 0.8194444444444444198, 0.8263888888888888395, 0.8333333333333333703, 0.8402777777777777901, 0.8472222222222222099, 0.8541666666666666297, 0.8611111111111111605, 0.8680555555555555802, 0.8750000000000000000, 0.8819444444444444198, 0.8888888888888888395, 0.8958333333333333703, 0.9027777777777777901, 0.9097222222222222099, 0.9166666666666666297, 0.9236111111111111605, 0.9305555555555555802, 0.9375000000000000000, 0.9444444444444444198, 0.9513888888888888395, 0.9583333333333333703, 0.9652777777777777901, 0.9722222222222222099, 0.9791666666666666297, 0.9842226772312638872, 0.9940649040035764994 ),
 .UNSPECIFIED. ) 
 GEOMETRIC_REPRESENTATION_ITEM ( )  RATIONAL_B_SPLINE_SURFACE ( (
 ( 1.000000000000000000, 0.8660254037844387076, 1.000000000000000000, 0.8660254037844387076, 1.000000000000000000, 0.8660254037844387076, 1.000000000000000000, 0.8660254037844387076, 1.000000000000000000, 0.8660254037844387076, 1.000000000000000000, 0.8660254037844387076, 1.000000000000000000, 0.8660254037844387076, 1.000000000000000000, 0.8660254037844387076, 1.000000000000000000, 0.8660254037844387076, 1.000000000000000000, 0.8660254037844387076, 1.000000000000000000, 0.8660254037844387076, 1.000000000000000000, 0.8660254037844387076, 1.000000000000000000, 0.8660254037844387076, 1.000000000000000000, 0.8660254037844387076, 1.000000000000000000, 0.8660254037844387076, 1.000000000000000000, 0.8660254037844387076, 1.000000000000000000, 0.8660254037844387076, 1.000000000000000000, 0.8660254037844387076, 1.000000000000000000, 0.8660254037844387076, 1.000000000000000000, 0.8660254037844387076, 1.000000000000000000, 0.8660254037844387076, 1.000000000000000000, 0.8660254037844387076, 1.000000000000000000, 0.8660254037844387076, 1.000000000000000000, 0.8660254037844387076, 1.000000000000000000, 0.8660254037844387076, 1.000000000000000000, 0.8660254037844387076, 1.000000000000000000, 0.8660254037844387076, 1.000000000000000000, 0.8660254037844387076, 1.000000000000000000, 0.8660254037844387076, 1.000000000000000000, 0.8660254037844387076, 1.000000000000000000, 0.8660254037844387076, 1.000000000000000000, 0.8660254037844387076, 1.000000000000000000, 0.8660254037844387076, 1.000000000000000000, 0.8660254037844387076, 1.000000000000000000, 0.8660254037844387076, 1.000000000000000000, 0.8660254037844387076, 1.000000000000000000, 0.8660254037844387076, 1.000000000000000000, 0.8660254037844387076, 1.000000000000000000, 0.8660254037844387076, 1.000000000000000000, 0.8660254037844387076, 1.000000000000000000, 0.8660254037844387076, 1.000000000000000000, 0.8660254037844387076, 1.000000000000000000, 0.8660254037844387076, 1.000000000000000000, 0.8660254037844387076, 1.000000000000000000, 0.8660254037844387076, 1.000000000000000000, 0.8660254037844387076, 1.000000000000000000, 0.8660254037844387076, 1.000000000000000000, 0.8660254037844387076, 1.000000000000000000, 0.8660254037844387076, 1.000000000000000000, 0.8660254037844387076, 1.000000000000000000, 0.8660254037844387076, 1.000000000000000000, 0.8660254037844387076, 1.000000000000000000, 0.8660254037844387076, 1.000000000000000000, 0.8660254037844387076, 1.000000000000000000, 0.8660254037844387076, 1.000000000000000000, 0.8660254037844387076, 1.000000000000000000, 0.8660254037844387076, 1.000000000000000000, 0.8660254037844387076, 1.000000000000000000, 0.8660254037844387076, 1.000000000000000000, 0.8660254037844387076, 1.000000000000000000, 0.8660254037844387076, 1.000000000000000000, 0.8660254037844387076, 1.000000000000000000, 0.8660254037844387076, 1.000000000000000000, 0.8660254037844387076, 1.000000000000000000, 0.8660254037844387076, 1.000000000000000000, 0.8660254037844387076, 1.000000000000000000, 0.8660254037844387076, 1.000000000000000000, 0.8660254037844387076, 1.000000000000000000, 0.8660254037844387076, 1.000000000000000000, 0.8660254037844387076, 1.000000000000000000, 0.8660254037844387076, 1.000000000000000000, 0.8660254037844387076, 1.000000000000000000, 0.8660254037844387076, 1.000000000000000000, 0.8660254037844387076, 1.000000000000000000, 0.8660254037844387076, 1.000000000000000000, 0.8660254037844387076, 1.000000000000000000, 0.8660254037844387076, 1.000000000000000000, 0.8660254037844387076, 1.000000000000000000, 0.8660254037844387076, 1.000000000000000000, 0.8660254037844387076, 1.000000000000000000, 0.8660254037844387076, 1.000000000000000000, 0.8660254037844387076, 1.000000000000000000, 0.8660254037844387076, 1.000000000000000000, 0.8660254037844387076, 1.000000000000000000, 0.8660254037844387076, 1.000000000000000000, 0.8660254037844387076, 1.000000000000000000, 0.8660254037844387076, 1.000000000000000000, 0.8660254037844387076, 1.000000000000000000, 0.8660254037844387076, 1.000000000000000000, 0.8660254037844387076, 1.000000000000000000, 0.8660254037844387076, 1.000000000000000000, 0.8660254037844387076, 1.000000000000000000, 0.8660254037844387076, 1.000000000000000000, 0.8660254037844387076, 1.000000000000000000, 0.8660254037844387076, 1.000000000000000000, 0.8660254037844387076, 1.000000000000000000, 0.8660254037844387076, 1.000000000000000000, 0.8660254037844387076, 1.000000000000000000, 0.8660254037844387076, 1.000000000000000000, 0.8660254037844387076, 1.000000000000000000, 0.8660254037844387076, 1.000000000000000000, 0.8660254037844387076, 1.000000000000000000, 0.8660254037844387076, 1.000000000000000000, 0.8660254037844387076, 1.000000000000000000, 0.8660254037844387076, 1.000000000000000000, 0.8660254037844387076, 1.000000000000000000, 0.8660254037844387076, 1.000000000000000000, 0.8660254037844387076, 1.000000000000000000, 0.8660254037844387076, 1.000000000000000000, 0.8660254037844387076, 1.000000000000000000, 0.8660254037844387076, 1.000000000000000000, 0.8660254037844387076, 1.000000000000000000, 0.8660254037844387076, 1.000000000000000000, 0.8660254037844387076, 1.000000000000000000, 0.8660254037844387076, 1.000000000000000000, 0.8660254037844387076, 1.000000000000000000, 0.8660254037844387076, 1.000000000000000000, 0.8660254037844387076, 1.000000000000000000, 0.8660254037844387076, 1.000000000000000000, 0.8660254037844387076, 1.000000000000000000, 0.8660254037844387076, 1.000000000000000000, 0.8660254037844387076, 1.000000000000000000, 0.8660254037844387076, 1.000000000000000000, 0.8660254037844387076, 1.000000000000000000, 0.8660254037844387076, 1.000000000000000000, 0.8660254037844387076, 1.000000000000000000, 0.8660254037844387076, 1.000000000000000000, 0.8660254037844387076, 1.000000000000000000, 0.8660254037844387076, 1.000000000000000000, 0.8660254037844387076, 1.000000000000000000, 0.8660254037844387076, 1.000000000000000000, 0.8660254037844387076, 1.000000000000000000, 0.8660254037844387076, 1.000000000000000000, 0.8660254037844387076, 1.000000000000000000, 0.8660254037844387076, 1.000000000000000000, 0.8660254037844387076, 1.000000000000000000, 0.8660254037844387076, 1.000000000000000000, 0.8660254037844387076, 1.000000000000000000, 0.8660254037844387076, 1.000000000000000000, 0.8660254037844387076, 1.000000000000000000, 0.8660254037844387076, 1.000000000000000000, 0.9024577157650929271, 0.9469497795711361299, 0.9469497795711361299, 0.9469497795711361299),
 ( 1.000000000000000000, 0.8660254037844387076, 1.000000000000000000, 0.8660254037844387076, 1.000000000000000000, 0.8660254037844387076, 1.000000000000000000, 0.8660254037844387076, 1.000000000000000000, 0.8660254037844387076, 1.000000000000000000, 0.8660254037844387076, 1.000000000000000000, 0.8660254037844387076, 1.000000000000000000, 0.8660254037844387076, 1.000000000000000000, 0.8660254037844387076, 1.000000000000000000, 0.8660254037844387076, 1.000000000000000000, 0.8660254037844387076, 1.000000000000000000, 0.8660254037844387076, 1.000000000000000000, 0.8660254037844387076, 1.000000000000000000, 0.8660254037844387076, 1.000000000000000000, 0.8660254037844387076, 1.000000000000000000, 0.8660254037844387076, 1.000000000000000000, 0.8660254037844387076, 1.000000000000000000, 0.8660254037844387076, 1.000000000000000000, 0.8660254037844387076, 1.000000000000000000, 0.8660254037844387076, 1.000000000000000000, 0.8660254037844387076, 1.000000000000000000, 0.8660254037844387076, 1.000000000000000000, 0.8660254037844387076, 1.000000000000000000, 0.8660254037844387076, 1.000000000000000000, 0.8660254037844387076, 1.000000000000000000, 0.8660254037844387076, 1.000000000000000000, 0.8660254037844387076, 1.000000000000000000, 0.8660254037844387076, 1.000000000000000000, 0.8660254037844387076, 1.000000000000000000, 0.8660254037844387076, 1.000000000000000000, 0.8660254037844387076, 1.000000000000000000, 0.8660254037844387076, 1.000000000000000000, 0.8660254037844387076, 1.000000000000000000, 0.8660254037844387076, 1.000000000000000000, 0.8660254037844387076, 1.000000000000000000, 0.8660254037844387076, 1.000000000000000000, 0.8660254037844387076, 1.000000000000000000, 0.8660254037844387076, 1.000000000000000000, 0.8660254037844387076, 1.000000000000000000, 0.8660254037844387076, 1.000000000000000000, 0.8660254037844387076, 1.000000000000000000, 0.8660254037844387076, 1.000000000000000000, 0.8660254037844387076, 1.000000000000000000, 0.8660254037844387076, 1.000000000000000000, 0.8660254037844387076, 1.000000000000000000, 0.8660254037844387076, 1.000000000000000000, 0.8660254037844387076, 1.000000000000000000, 0.8660254037844387076, 1.000000000000000000, 0.8660254037844387076, 1.000000000000000000, 0.8660254037844387076, 1.000000000000000000, 0.8660254037844387076, 1.000000000000000000, 0.8660254037844387076, 1.000000000000000000, 0.8660254037844387076, 1.000000000000000000, 0.8660254037844387076, 1.000000000000000000, 0.8660254037844387076, 1.000000000000000000, 0.8660254037844387076, 1.000000000000000000, 0.8660254037844387076, 1.000000000000000000, 0.8660254037844387076, 1.000000000000000000, 0.8660254037844387076, 1.000000000000000000, 0.8660254037844387076, 1.000000000000000000, 0.8660254037844387076, 1.000000000000000000, 0.8660254037844387076, 1.000000000000000000, 0.8660254037844387076, 1.000000000000000000, 0.8660254037844387076, 1.000000000000000000, 0.8660254037844387076, 1.000000000000000000, 0.8660254037844387076, 1.000000000000000000, 0.8660254037844387076, 1.000000000000000000, 0.8660254037844387076, 1.000000000000000000, 0.8660254037844387076, 1.000000000000000000, 0.8660254037844387076, 1.000000000000000000, 0.8660254037844387076, 1.000000000000000000, 0.8660254037844387076, 1.000000000000000000, 0.8660254037844387076, 1.000000000000000000, 0.8660254037844387076, 1.000000000000000000, 0.8660254037844387076, 1.000000000000000000, 0.8660254037844387076, 1.000000000000000000, 0.8660254037844387076, 1.000000000000000000, 0.8660254037844387076, 1.000000000000000000, 0.8660254037844387076, 1.000000000000000000, 0.8660254037844387076, 1.000000000000000000, 0.8660254037844387076, 1.000000000000000000, 0.8660254037844387076, 1.000000000000000000, 0.8660254037844387076, 1.000000000000000000, 0.8660254037844387076, 1.000000000000000000, 0.8660254037844387076, 1.000000000000000000, 0.8660254037844387076, 1.000000000000000000, 0.8660254037844387076, 1.000000000000000000, 0.8660254037844387076, 1.000000000000000000, 0.8660254037844387076, 1.000000000000000000, 0.8660254037844387076, 1.000000000000000000, 0.8660254037844387076, 1.000000000000000000, 0.8660254037844387076, 1.000000000000000000, 0.8660254037844387076, 1.000000000000000000, 0.8660254037844387076, 1.000000000000000000, 0.8660254037844387076, 1.000000000000000000, 0.8660254037844387076, 1.000000000000000000, 0.8660254037844387076, 1.000000000000000000, 0.8660254037844387076, 1.000000000000000000, 0.8660254037844387076, 1.000000000000000000, 0.8660254037844387076, 1.000000000000000000, 0.8660254037844387076, 1.000000000000000000, 0.8660254037844387076, 1.000000000000000000, 0.8660254037844387076, 1.000000000000000000, 0.8660254037844387076, 1.000000000000000000, 0.8660254037844387076, 1.000000000000000000, 0.8660254037844387076, 1.000000000000000000, 0.8660254037844387076, 1.000000000000000000, 0.8660254037844387076, 1.000000000000000000, 0.8660254037844387076, 1.000000000000000000, 0.8660254037844387076, 1.000000000000000000, 0.8660254037844387076, 1.000000000000000000, 0.8660254037844387076, 1.000000000000000000, 0.8660254037844387076, 1.000000000000000000, 0.8660254037844387076, 1.000000000000000000, 0.8660254037844387076, 1.000000000000000000, 0.8660254037844387076, 1.000000000000000000, 0.8660254037844387076, 1.000000000000000000, 0.8660254037844387076, 1.000000000000000000, 0.8660254037844387076, 1.000000000000000000, 0.8660254037844387076, 1.000000000000000000, 0.8660254037844387076, 1.000000000000000000, 0.8660254037844387076, 1.000000000000000000, 0.8660254037844387076, 1.000000000000000000, 0.8660254037844387076, 1.000000000000000000, 0.8660254037844387076, 1.000000000000000000, 0.8660254037844387076, 1.000000000000000000, 0.8660254037844387076, 1.000000000000000000, 0.8660254037844387076, 1.000000000000000000, 0.8660254037844387076, 1.000000000000000000, 0.8660254037844387076, 1.000000000000000000, 0.8660254037844387076, 1.000000000000000000, 0.8660254037844387076, 1.000000000000000000, 0.8660254037844387076, 1.000000000000000000, 0.8660254037844387076, 1.000000000000000000, 0.8660254037844387076, 1.000000000000000000, 0.8660254037844387076, 1.000000000000000000, 0.8660254037844387076, 1.000000000000000000, 0.8660254037844387076, 1.000000000000000000, 0.8660254037844387076, 1.000000000000000000, 0.8660254037844387076, 1.000000000000000000, 0.8660254037844387076, 1.000000000000000000, 0.9024577157650929271, 0.9469497795711361299, 0.9469497795711361299, 0.9469497795711361299) ) ) 
 REPRESENTATION_ITEM ( '' )  SURFACE ( )  );
#34283=CARTESIAN_POINT ( 'NONE',  ( 92.69370383062501162, -209.9999999999999716, 89.00781250086714635 ) ) ;
#34284=CARTESIAN_POINT ( 'NONE',  ( -94.99999999999997158, -206.9400435732949575, 83.57062500173429953 ) ) ;
#34296=EDGE_CURVE ( 'NONE', #7474, #1262, #59465, .T. ) ;
#34300=DIRECTION ( 'NONE',  ( 1.000000000000000000, 0.000000000000000000, 0.000000000000000000 ) ) ;
#34302=CARTESIAN_POINT ( 'NONE',  ( -92.35000000000003695, 89.99999999755290503, 75.15687493081163950 ) ) ;
#34305=CARTESIAN_POINT ( 'NONE',  ( 94.99999999999998579, 92.66308142843935514, 86.30906250086715659 ) ) ;
#34308=CARTESIAN_POINT ( 'NONE',  ( 92.69370383062501162, -209.9999999999999716, 82.65781250086713783 ) ) ;
#34310=EDGE_CURVE ( 'NONE', #35350, #42474, #104, .T. ) ;
#34312=CARTESIAN_POINT ( 'NONE',  ( -96.32499999999996021, -212.2949673200287179, 81.29520833506762756 ) ) ;
#34313=CARTESIAN_POINT ( 'NONE',  ( -92.35000000000000853, 88.47002178664756400, 84.54958333333334508 ) ) ;
#34320=CARTESIAN_POINT ( 'NONE',  ( -92.69370383062498320, -211.3315407142195852, 88.00239583420047040 ) ) ;
#34321=CARTESIAN_POINT ( 'NONE',  ( -93.84685191531252713, 88.00268892867056536, 85.56822916753381492 ) ) ;
#34324=CARTESIAN_POINT ( 'NONE',  ( 92.69370383062498320, 90.00000000000002842, 85.83281250086714920 ) ) ;
#34325=CARTESIAN_POINT ( 'NONE',  ( -96.15314808468752972, 91.99731107132950569, 85.72697916753379843 ) ) ;
#34331=CARTESIAN_POINT ( 'NONE',  ( 92.35000000000000853, 91.52997821335253548, 87.40708333333333258 ) ) ;
#34332=CARTESIAN_POINT ( 'NONE',  ( -94.99999999999997158, -207.3369185715606307, 87.57906250086713840 ) ) ;
#34340=CARTESIAN_POINT ( 'NONE',  ( -95.00000000000002842, 93.05995642670501411, 76.50624999999999432 ) ) ;
#34341=DIRECTION ( 'NONE',  ( -0.000000000000000000, -0.000000000000000000, 1.000000000000000000 ) ) ;
#34342=CARTESIAN_POINT ( 'NONE',  ( 93.67500000000001137, -207.7050326799711968, 81.00416666666666288 ) ) ;
#34348=CARTESIAN_POINT ( 'NONE',  ( -97.30629616937501680, 90.00000000000004263, 79.48281250086714067 ) ) ;
#34354=CARTESIAN_POINT ( 'NONE',  ( -94.99999999999997158, -209.9999999999999716, 90.00000000000000000 ) ) ;
#34359=CARTESIAN_POINT ( 'NONE',  ( 94.99999999999998579, 87.33691857156068750, 77.89531250086714920 ) ) ;
#34361=CARTESIAN_POINT ( 'NONE',  ( -93.84685191531247028, -211.9973110713294489, 80.48822916753381662 ) ) ;
#34366=DIRECTION ( 'NONE',  ( 1.000000000000000000, 0.000000000000000000, 0.000000000000000000 ) ) ;
#34370=CARTESIAN_POINT ( 'NONE',  ( -92.69370383062505425, 91.33154071421968467, 74.93197916753381094 ) ) ;
#34371=CARTESIAN_POINT ( 'NONE',  ( 92.69370383062501162, -211.3315407142195852, 78.90072916753381094 ) ) ;
#34379=CARTESIAN_POINT ( 'NONE',  ( -93.67499999999998295, -207.7050326799711968, 83.43833333333333258 ) ) ;
#34387=ORIENTED_EDGE ( 'NONE', *, *, #67293, .F. ) ;
#34388=VERTEX_POINT ( 'NONE', #9430 ) ;
#34389=CARTESIAN_POINT ( 'NONE',  ( 96.15314808468748708, 91.99731107132950569, 81.96989583420048575 ) ) ;
#34390=CARTESIAN_POINT ( 'NONE',  ( 92.35000000000002274, -211.5299782133524502, 77.35291666666665833 ) ) ;
#34391=ORIENTED_EDGE ( 'NONE', *, *, #29797, .T. ) ;
#34404=CARTESIAN_POINT ( 'NONE',  ( -97.64999999999994884, -208.4700217866474645, 83.04145833506763097 ) ) ;
#34408=CARTESIAN_POINT ( 'NONE',  ( 96.32499999999997442, 92.29496732002878900, 77.80270833506763495 ) ) ;
#34409=CARTESIAN_POINT ( 'NONE',  ( -93.67500000000003979, 87.70503267997129626, 80.13104166840095388 ) ) ;
#34411=CARTESIAN_POINT ( 'NONE',  ( 92.69370383062498320, 88.66845928578037217, 79.05947916753382287 ) ) ;
#34430=LINE ( 'NONE', #33694, #13730 ) ;
#34431=CARTESIAN_POINT ( 'NONE',  ( -92.69370383062498320, -209.9999999999999716, 81.22906250086715829 ) ) ;
#34434=CARTESIAN_POINT ( 'NONE',  ( 97.64999999964365429, -210.0000434577794408, 89.12687334326047051 ) ) ;
#34435=CARTESIAN_POINT ( 'NONE',  ( -97.51895106303136629, -210.1706338775387621, 74.92125785461011844 ) ) ;
#34442=CARTESIAN_POINT ( 'NONE',  ( 92.34999999999999432, 90.00000000000002842, 76.66499999999999204 ) ) ;
#34443=CARTESIAN_POINT ( 'NONE',  ( -94.99999999999997158, -206.9400435732949575, 76.58562500173430010 ) ) ;
#34444=CARTESIAN_POINT ( 'NONE',  ( 99.99999999999998579, 95.00000000000002842, 90.00000000000000000 ) ) ;
#34448=CARTESIAN_POINT ( 'NONE',  ( 93.84685191531248449, 91.99731107132950569, 87.79072916753381151 ) ) ;
#34450=CARTESIAN_POINT ( 'NONE',  ( -93.84685191531248449, -208.0026889286704943, 88.31989583420048007 ) ) ;
#34451=CARTESIAN_POINT ( 'NONE',  ( -92.35000000000003695, 90.00000000000004263, 80.79249999999998977 ) ) ;
#34455=CARTESIAN_POINT ( 'NONE',  ( -95.00000000000002842, 87.33691857156074434, 79.64156250086713840 ) ) ;
#34459=LINE ( 'NONE', #52123, #24660 ) ;
#34466=CARTESIAN_POINT ( 'NONE',  ( 96.15314808468750130, -211.9973110713294489, 76.67822916753381435 ) ) ;
#34471=CARTESIAN_POINT ( 'NONE',  ( 92.69370383062501162, -208.6684592857803295, 84.66864583420047552 ) ) ;
#34475=CARTESIAN_POINT ( 'NONE',  ( -93.67499999999998295, -207.7050326799711968, 77.16770833506762983 ) ) ;
#34479=CARTESIAN_POINT ( 'NONE',  ( 96.32499999999998863, -207.7050326799711968, 89.78833333333332689 ) ) ;
#34482=ORIENTED_EDGE ( 'NONE', *, *, #54013, .F. ) ;
#34486=CARTESIAN_POINT ( 'NONE',  ( -93.84685191531254134, 91.99731107132950569, 88.95489583420049939 ) ) ;
#34489=CARTESIAN_POINT ( 'NONE',  ( 95.00000000000000000, -213.0599564267049857, 76.26812500173430465 ) ) ;
#34490=CARTESIAN_POINT ( 'NONE',  ( 97.64999999999997726, 88.47002178664753558, 78.83458333333334167 ) ) ;
#34493=CARTESIAN_POINT ( 'NONE',  ( 97.65000000000000568, -208.4700217866474645, 75.20979166840096752 ) ) ;
#34497=CARTESIAN_POINT ( 'NONE',  ( -97.65000000000001990, 90.00000000000004263, 89.44437500173430067 ) ) ;
#34498=CARTESIAN_POINT ( 'NONE',  ( -97.30629616937501680, 90.00000000000004263, 80.91156250086716284 ) ) ;
#34499=CARTESIAN_POINT ( 'NONE',  ( 96.15314808468748708, 88.00268892867053694, 88.74322916753382628 ) ) ;
#34507=CARTESIAN_POINT ( 'NONE',  ( -97.30629616937497417, -208.6684592857803011, 77.52489583420046415 ) ) ;
#34509=VERTEX_POINT ( 'NONE', #57534 ) ;
#34515=( BOUNDED_CURVE ( )  B_SPLINE_CURVE ( 2, ( #54016, #43850, #55486, #49833, #2554, #72751, #25435 ),
 .UNSPECIFIED., .F., .F. ) 
 B_SPLINE_CURVE_WITH_KNOTS ( ( 3, 2, 2, 3 ),
 ( 0.8333333333333334814, 0.8402777777777779011, 0.8472222222222222099, 0.8541666666666666297 ),
 .UNSPECIFIED. ) 
 CURVE ( )  GEOMETRIC_REPRESENTATION_ITEM ( )  RATIONAL_B_SPLINE_CURVE ( ( 0.9999999999999978906, 0.8660254037844408170, 1.000000000000000000, 0.8660254037844387076, 1.000000000000000000, 0.8660254037844387076, 1.000000000000000000 ) ) 
 REPRESENTATION_ITEM ( '' )  );
#34516=CARTESIAN_POINT ( 'NONE',  ( -97.30629616937497417, -211.3315407142195852, 76.99572916753380980 ) ) ;
#34522=ORIENTED_EDGE ( 'NONE', *, *, #15216, .F. ) ;
#34526=CARTESIAN_POINT ( 'NONE',  ( 92.34999999999999432, -210.0000225208804068, 86.26937578065383150 ) ) ;
#34527=CARTESIAN_POINT ( 'NONE',  ( 92.69370383062498320, 90.00000000000002842, 83.92781250086714806 ) ) ;
#34529=CARTESIAN_POINT ( 'NONE',  ( -92.34999999999990905, -211.5299782133524218, 83.91458333333333997 ) ) ;
#34530=CARTESIAN_POINT ( 'NONE',  ( -95.00000000000002842, 86.94004357329504273, 88.25374999999999659 ) ) ;
#34541=B_SPLINE_CURVE_WITH_KNOTS ( 'NONE', 3,
 ( #45177, #32755, #44440, #67353, #38788, #66975, #15476, #68100, #45559, #61721, #55705, #32391, #73352, #5335, #50046, #38419, #72971, #50795, #4592, #60972, #27113, #73721, #15855, #10205 ),
 .UNSPECIFIED., .F., .F.,
 ( 4, 2, 2, 2, 2, 2, 2, 2, 2, 2, 2, 4 ),
 ( -0.009991285186810519234, -0.009254074022779607347, -0.008516862858748697196, -0.007779651694717785310, -0.007411046112702331101, -0.007042440530686875158, -0.006673834948671420950, -0.006305229366655965006, -0.005568018202625055722, -0.004830807038594145571, -0.004462201456578723455, -0.004093595874563301339 ),
 .UNSPECIFIED. ) ;
#34546=CARTESIAN_POINT ( 'NONE',  ( -97.65000000000001990, 90.00000000000004263, 79.83999999999998920 ) ) ;
#34556=CARTESIAN_POINT ( 'NONE',  ( 97.30629616937498838, -208.6684592857803011, 86.36197916753383197 ) ) ;
#34560=DIRECTION ( 'NONE',  ( -0.000000000000000000, -0.000000000000000000, 1.000000000000000000 ) ) ;
#34562=CARTESIAN_POINT ( 'NONE',  ( -96.32499999999996021, -207.7050326799711968, 79.81354166840095843 ) ) ;
#34566=CARTESIAN_POINT ( 'NONE',  ( 93.84685191531249870, -208.0026889286704943, 84.61572916753381435 ) ) ;
#34576=DIRECTION ( 'NONE',  ( 1.000000000000000000, 0.000000000000000000, 0.000000000000000000 ) ) ;
#34578=EDGE_LOOP ( 'NONE', ( #30494, #40033, #19309, #19576 ) ) ;
#34580=CARTESIAN_POINT ( 'NONE',  ( 95.00000000000000000, -213.0599564267049857, 87.69812500173429726 ) ) ;
#34596=CARTESIAN_POINT ( 'NONE',  ( 93.67500000000001137, -212.2949673200287179, 76.13583333333333769 ) ) ;
#34600=CARTESIAN_POINT ( 'NONE',  ( -92.35000000000005116, 88.47002178664754979, 86.45458333333333201 ) ) ;
#34602=CARTESIAN_POINT ( 'NONE',  ( 97.30629616937498838, 91.33154071421968467, 74.77322916753379900 ) ) ;
#34603=ORIENTED_EDGE ( 'NONE', *, *, #24270, .T. ) ;
#34605=CARTESIAN_POINT ( 'NONE',  ( -93.84685191531248449, -208.0026889286704943, 86.25614583420048120 ) ) ;
#34610=CARTESIAN_POINT ( 'NONE',  ( -97.30629616937497417, -208.6684592857803295, 76.88989583420047325 ) ) ;
#34615=CARTESIAN_POINT ( 'NONE',  ( -92.35000000000012221, 90.00000071509187194, 85.31687502647973531 ) ) ;
#34620=CARTESIAN_POINT ( 'NONE',  ( -95.00000000000002842, 87.33691857156074434, 79.00656250086713328 ) ) ;
#34621=DIRECTION ( 'NONE',  ( -2.628368902995175337E-16, -1.000000000000000000, 0.000000000000000000 ) ) ;
#34629=EDGE_CURVE ( 'NONE', #14315, #17407, #23116, .T. ) ;
#34635=CARTESIAN_POINT ( 'NONE',  ( -94.99999999999997158, -212.6630814284392557, 75.35531250086715715 ) ) ;
#34637=FACE_OUTER_BOUND ( 'NONE', #49186, .T. ) ;
#34642=LINE ( 'NONE', #15877, #72953 ) ;
#34649=ORIENTED_EDGE ( 'NONE', *, *, #22560, .T. ) ;
#34656=CARTESIAN_POINT ( 'NONE',  ( 97.30629616937498838, -211.3315407142195852, 89.27239583420048064 ) ) ;
#34660=ORIENTED_EDGE ( 'NONE', *, *, #59788, .T. ) ;
#34667=ORIENTED_EDGE ( 'NONE', *, *, #17232, .F. ) ;
#34669=AXIS2_PLACEMENT_3D ( 'NONE', #10998, #44852, #66687 ) ;
#34670=ORIENTED_EDGE ( 'NONE', *, *, #19612, .F. ) ;
#34672=CARTESIAN_POINT ( 'NONE',  ( 92.49271422325853109, 89.65937732759924472, 74.92458348457969919 ) ) ;
#34677=CARTESIAN_POINT ( 'NONE',  ( 93.84685191531248449, 88.00268892867053694, 84.03364583420047040 ) ) ;
#34679=CARTESIAN_POINT ( 'NONE',  ( 93.84685191531249870, -208.0026889286704943, 80.64697916753381435 ) ) ;
#34689=CARTESIAN_POINT ( 'NONE',  ( -96.15314808468747287, -208.0026889286704943, 85.09197916753380753 ) ) ;
#34690=CARTESIAN_POINT ( 'NONE',  ( -92.69370383062504004, 90.00000000000004263, 82.49906250086715431 ) ) ;
#34692=CARTESIAN_POINT ( 'NONE',  ( 97.30629616937498838, 90.00000000000002842, 83.61031250086713840 ) ) ;
#34693=CARTESIAN_POINT ( 'NONE',  ( -93.84685191531254134, 91.99731107132950569, 85.62114583420046188 ) ) ;
#34697=CYLINDRICAL_SURFACE ( 'NONE', #45164, 2.649999999999985700 ) ;
#34700=CARTESIAN_POINT ( 'NONE',  ( -96.15314808468747287, -208.0026889286704943, 86.99697916753380866 ) ) ;
#34706=ORIENTED_EDGE ( 'NONE', *, *, #61002, .F. ) ;
#34715=CARTESIAN_POINT ( 'NONE',  ( -93.67500000000003979, 92.29496732002878900, 77.72333333333332916 ) ) ;
#34716=DIRECTION ( 'NONE',  ( -0.000000000000000000, -0.000000000000000000, 1.000000000000000000 ) ) ;
#34722=VECTOR ( 'NONE', #58508, 1000.000000000000000 ) ;
#34724=CARTESIAN_POINT ( 'NONE',  ( -95.00000000000002842, 92.66308142843932671, 79.32406250086714294 ) ) ;
#34728=CARTESIAN_POINT ( 'NONE',  ( 92.34999999999999432, 90.00000000000002842, 86.82500000000000284 ) ) ;
#34730=CARTESIAN_POINT ( 'NONE',  ( -93.84685191531247028, -211.9973110713294489, 88.10822916753382117 ) ) ;
#34735=( BOUNDED_CURVE ( )  B_SPLINE_CURVE ( 2, ( #18835, #41776, #30487, #48526, #18114, #1240, #8308 ),
 .UNSPECIFIED., .F., .F. ) 
 B_SPLINE_CURVE_WITH_KNOTS ( ( 3, 2, 2, 3 ),
 ( 0.6666666666666667407, 0.6736111111111112715, 0.6805555555555555802, 0.6875000000000000000 ),
 .UNSPECIFIED. ) 
 CURVE ( )  GEOMETRIC_REPRESENTATION_ITEM ( )  RATIONAL_B_SPLINE_CURVE ( ( 0.9999999999999978906, 0.8660254037844408170, 1.000000000000000000, 0.8660254037844387076, 1.000000000000000000, 0.8660254037844387076, 1.000000000000000000 ) ) 
 REPRESENTATION_ITEM ( '' )  );
#34737=CARTESIAN_POINT ( 'NONE',  ( 93.84685191531248449, 91.99731107132950569, 77.63072916753381492 ) ) ;
#34738=VECTOR ( 'NONE', #13302, 1000.000000000000000 ) ;
#34740=CARTESIAN_POINT ( 'NONE',  ( -93.84685191531247028, -211.9973110713294489, 81.12322916753382174 ) ) ;
#34742=ORIENTED_EDGE ( 'NONE', *, *, #65258, .F. ) ;
#34744=CARTESIAN_POINT ( 'NONE',  ( -94.99999999999997158, -213.0599564267049857, 76.18874999999999886 ) ) ;
#34747=ADVANCED_FACE ( 'NONE', ( #25680 ), #32046, .F. ) ;
#34751=CARTESIAN_POINT ( 'NONE',  ( -92.69370383062505425, 91.33154071421968467, 75.56697916753383026 ) ) ;
#34752=CARTESIAN_POINT ( 'NONE',  ( 92.69370383062501162, -209.9999999999999716, 76.94281250086713442 ) ) ;
#34759=CARTESIAN_POINT ( 'NONE',  ( -95.00000000000002842, 93.05995642670504253, 79.12562500173429214 ) ) ;
#34767=CARTESIAN_POINT ( 'NONE',  ( 97.64999999999999147, -209.9999999999999716, 75.07749999999998636 ) ) ;
#34770=CARTESIAN_POINT ( 'NONE',  ( 92.69370383062498320, 90.00000000000002842, 82.81656250086714977 ) ) ;
#34771=CARTESIAN_POINT ( 'NONE',  ( 92.35000000000002274, -208.4700217866474645, 75.97708333333333997 ) ) ;
#34783=CARTESIAN_POINT ( 'NONE',  ( -97.64999999999996305, -209.9999999999999716, 89.90078125043358170 ) ) ;
#34785=CARTESIAN_POINT ( 'NONE',  ( -92.34999999999999432, -211.5299782133524502, 78.91395833506763324 ) ) ;
#34789=CARTESIAN_POINT ( 'NONE',  ( 97.64999999999997726, 91.52997821335252127, 79.01979166840095559 ) ) ;
#34790=CARTESIAN_POINT ( 'NONE',  ( -93.67500000000003979, 92.29496732002878900, 79.70770833506762187 ) ) ;
#34793=CARTESIAN_POINT ( 'NONE',  ( 96.15314808468748708, 88.00268892867053694, 79.85322916753381151 ) ) ;
#34798=DIRECTION ( 'NONE',  ( 1.000000000000000000, 0.000000000000000000, 0.000000000000000000 ) ) ;
#34804=CARTESIAN_POINT ( 'NONE',  ( -97.64999999999996305, -209.9999999999999716, 90.00000000000000000 ) ) ;
#34813=CARTESIAN_POINT ( 'NONE',  ( -94.99999999999997158, -212.6630814284392557, 76.62531250086715318 ) ) ;
#34820=CARTESIAN_POINT ( 'NONE',  ( -96.10855813657714464, -212.3693961633073855, 74.97612907457856579 ) ) ;
#34822=CARTESIAN_POINT ( 'NONE',  ( 94.99999999999998579, 92.66308142843932671, 76.14906250086716000 ) ) ;
#34825=LINE ( 'NONE', #62295, #27708 ) ;
#34827=FACE_OUTER_BOUND ( 'NONE', #55224, .T. ) ;
#34833=CARTESIAN_POINT ( 'NONE',  ( 92.69370383062498320, 90.00000000000002842, 87.26156250086715715 ) ) ;
#34837=CARTESIAN_POINT ( 'NONE',  ( 92.35004028547589883, -211.5300014721827608, 83.14729327728633734 ) ) ;
#34838=CARTESIAN_POINT ( 'NONE',  ( -96.15314808468751551, 88.00268892867056536, 80.22364583420046813 ) ) ;
#34842=CARTESIAN_POINT ( 'NONE',  ( 93.67500000000001137, -207.7050326799711968, 87.35416666666665719 ) ) ;
#34843=FACE_OUTER_BOUND ( 'NONE', #3722, .T. ) ;
#34845=DIRECTION ( 'NONE',  ( -1.000000000000000000, 0.000000000000000000, 0.000000000000000000 ) ) ;
#34850=CARTESIAN_POINT ( 'NONE',  ( 95.00000000000000000, -212.6630814284392557, 80.43531250086715545 ) ) ;
#34851=CARTESIAN_POINT ( 'NONE',  ( -94.99999999999997158, -209.9999999999999716, 90.00000000000000000 ) ) ;
#34852=CARTESIAN_POINT ( 'NONE',  ( 94.99999999999998579, 90.00000000000002842, 90.00000000000000000 ) ) ;
#34853=CARTESIAN_POINT ( 'NONE',  ( -97.64999999999996305, -210.0000348529796668, 77.37937620717859488 ) ) ;
#34854=CARTESIAN_POINT ( 'NONE',  ( 93.67499999999998295, 92.29496732002878900, 83.62354166840097491 ) ) ;
#34856=CARTESIAN_POINT ( 'NONE',  ( 96.32499999999998863, -212.2949673200287179, 85.76666666666665151 ) ) ;
#34859=EDGE_LOOP ( 'NONE', ( #6763, #329 ) ) ;
#34867=CARTESIAN_POINT ( 'NONE',  ( -96.15314808468752972, 91.99731107132950569, 85.88572916753381037 ) ) ;
#34869=ADVANCED_FACE ( 'NONE', ( #47506 ), #8764, .F. ) ;
#34871=DIRECTION ( 'NONE',  ( -0.000000000000000000, -0.000000000000000000, 1.000000000000000000 ) ) ;
#34872=CARTESIAN_POINT ( 'NONE',  ( 97.64999999999997726, -208.4700217866474645, 76.47979166840096354 ) ) ;
#34873=CARTESIAN_POINT ( 'NONE',  ( 92.34999999999999432, 90.00000000000002842, 77.93499999999998806 ) ) ;
#34877=CARTESIAN_POINT ( 'NONE',  ( 92.35000000005783249, -210.0000112241611703, 75.47473230081648410 ) ) ;
#34878=ORIENTED_EDGE ( 'NONE', *, *, #13717, .T. ) ;
#34882=CARTESIAN_POINT ( 'NONE',  ( -96.15314808468752972, 91.99731107132950569, 80.17072916753382117 ) ) ;
#34883=CARTESIAN_POINT ( 'NONE',  ( 92.69370383062498320, 88.66845928578037217, 88.58447916753382856 ) ) ;
#34889=CARTESIAN_POINT ( 'NONE',  ( -93.26027265873601380, 91.51405112163766375, 74.79348190356853365 ) ) ;
#34892=CARTESIAN_POINT ( 'NONE',  ( -93.84685191531247028, -211.9973110713294489, 78.42447916753381776 ) ) ;
#34900=CARTESIAN_POINT ( 'NONE',  ( -96.15314808468747287, -208.0026889286704943, 87.79072916753381151 ) ) ;
#34912=CARTESIAN_POINT ( 'NONE',  ( 94.99999999999998579, 87.33691857156068750, 85.35656250086714181 ) ) ;
#34914=CARTESIAN_POINT ( 'NONE',  ( -92.35000000000003695, 90.00000000000004263, 75.71250000000000568 ) ) ;
#34928=CARTESIAN_POINT ( 'NONE',  ( 92.35000000000000853, -209.9999999999999716, 90.00000000000000000 ) ) ;
#34931=ORIENTED_EDGE ( 'NONE', *, *, #7164, .T. ) ;
#34937=CARTESIAN_POINT ( 'NONE',  ( 93.84685191531251292, -211.9973110713294489, 86.73239583420048859 ) ) ;
#34938=ORIENTED_EDGE ( 'NONE', *, *, #32246, .F. ) ;
#34942=CARTESIAN_POINT ( 'NONE',  ( 93.67500000000001137, -207.7050326799711968, 88.62416666666665321 ) ) ;
#34945=CARTESIAN_POINT ( 'NONE',  ( 93.84685191531251292, -211.9973110713294489, 81.65239583420049030 ) ) ;
#34960=CARTESIAN_POINT ( 'NONE',  ( 97.64999999999997726, -211.5299782133524502, 88.43895833506762472 ) ) ;
#34965=( BOUNDED_CURVE ( )  B_SPLINE_CURVE ( 2, ( #22519, #23258, #45835, #68757, #62766, #53573, #63131 ),
 .UNSPECIFIED., .F., .F. ) 
 B_SPLINE_CURVE_WITH_KNOTS ( ( 3, 2, 2, 3 ),
 ( 0.5416666666666665186, 0.5486111111111110494, 0.5555555555555553582, 0.5624999999999997780 ),
 .UNSPECIFIED. ) 
 CURVE ( )  GEOMETRIC_REPRESENTATION_ITEM ( )  RATIONAL_B_SPLINE_CURVE ( ( 1.000000000000002220, 0.8660254037844365982, 1.000000000000000000, 0.8660254037844387076, 1.000000000000000000, 0.8660254037844430375, 0.9999999999999956701 ) ) 
 REPRESENTATION_ITEM ( '' )  );
#34975=CIRCLE ( 'NONE', #69787, 23.50000000000000355 ) ;
#34981=CARTESIAN_POINT ( 'NONE',  ( -92.35000000000005116, 88.47002178664754979, 87.72458333333332803 ) ) ;
#34983=CARTESIAN_POINT ( 'NONE',  ( 93.67500000000001137, -207.7050326799711968, 89.89416666666666345 ) ) ;
#34987=CARTESIAN_POINT ( 'NONE',  ( -96.15314808468745866, -211.9973110713294489, 85.93864583420048575 ) ) ;
#34988=ORIENTED_EDGE ( 'NONE', *, *, #59612, .F. ) ;
#34993=CARTESIAN_POINT ( 'NONE',  ( -93.84685191531247028, -211.9973110713294489, 77.15447916753380753 ) ) ;
#34999=CARTESIAN_POINT ( 'NONE',  ( 93.67499999999999716, 87.70503267997126784, 80.02520833506763154 ) ) ;
#35001=CARTESIAN_POINT ( 'NONE',  ( -96.15314808468752972, 91.99731107132950569, 80.01197916753380923 ) ) ;
#35015=CARTESIAN_POINT ( 'NONE',  ( 92.35000000000000853, -209.9999999999999716, 78.57000000000000739 ) ) ;
#35016=CARTESIAN_POINT ( 'NONE',  ( -96.15314808468747287, -208.0026889286704943, 75.72572916753382799 ) ) ;
#35031=CARTESIAN_POINT ( 'NONE',  ( 97.30629616937498838, -208.6684592857803295, 86.20322916753380582 ) ) ;
#35038=VERTEX_POINT ( 'NONE', #36946 ) ;
#35039=CARTESIAN_POINT ( 'NONE',  ( -95.00000000000002842, 92.66308142843932671, 79.48281250086715488 ) ) ;
#35051=EDGE_CURVE ( 'NONE', #58070, #41704, #33638, .T. ) ;
#35055=CARTESIAN_POINT ( 'NONE',  ( 92.69370383062498320, 91.33154071421968467, 85.77989583420048803 ) ) ;
#35057=CARTESIAN_POINT ( 'NONE',  ( 95.00000000000000000, -207.3369185715606307, 81.86406250086714920 ) ) ;
#35059=DIRECTION ( 'NONE',  ( 1.000000000000000000, 0.000000000000000000, 0.000000000000000000 ) ) ;
#35062=CARTESIAN_POINT ( 'NONE',  ( 95.00000000000000000, -206.9400435732949575, 79.04624999999997215 ) ) ;
#35063=FACE_OUTER_BOUND ( 'NONE', #51323, .T. ) ;
#35064=CARTESIAN_POINT ( 'NONE',  ( -93.67500000000003979, 87.70503267997129626, 79.41666666666665719 ) ) ;
#35065=DIRECTION ( 'NONE',  ( 0.000000000000000000, 0.000000000000000000, -1.000000000000000000 ) ) ;
#35066=CARTESIAN_POINT ( 'NONE',  ( -92.69370383062498320, -211.3315407142195852, 85.46239583420047836 ) ) ;
#35067=CARTESIAN_POINT ( 'NONE',  ( -93.84685191531254134, 91.99731107132950569, 81.33489583420049485 ) ) ;
#35071=CARTESIAN_POINT ( 'NONE',  ( 93.84685191531248449, 88.00268892867053694, 85.30364583420046642 ) ) ;
#35077=CARTESIAN_POINT ( 'NONE',  ( 96.32499999999998863, -207.7050326799711968, 85.34333333333333371 ) ) ;
#35078=CARTESIAN_POINT ( 'NONE',  ( -93.84685191531248449, -208.0026889286704943, 85.62114583420046188 ) ) ;
#35080=CARTESIAN_POINT ( 'NONE',  ( -92.35000000035638834, 89.99995654222792041, 89.12687334326074051 ) ) ;
#35089=CARTESIAN_POINT ( 'NONE',  ( -96.32500000000001705, 92.29496732002878900, 76.55916666666666970 ) ) ;
#35092=CARTESIAN_POINT ( 'NONE',  ( -93.84685191531254134, 91.99731107132950569, 88.16114583420046813 ) ) ;
#35098=CARTESIAN_POINT ( 'NONE',  ( -97.30629616937501680, 88.66845928578038638, 77.63072916753380071 ) ) ;
#35103=CARTESIAN_POINT ( 'NONE',  ( 97.64999999999999147, -210.0000000255706709, 84.04687500080852658 ) ) ;
#35105=CARTESIAN_POINT ( 'NONE',  ( -97.30629616937495996, -209.9999999999999716, 85.35656250086715602 ) ) ;
#35107=CARTESIAN_POINT ( 'NONE',  ( 92.69370383062498320, 88.66845928578035796, 77.15447916753382174 ) ) ;
#35108=CARTESIAN_POINT ( 'NONE',  ( -94.99999999999997158, -207.3369185715606307, 75.67281250086715261 ) ) ;
#35111=CARTESIAN_POINT ( 'NONE',  ( -92.35000000002600018, 89.99998827382285072, 82.77687459617033028 ) ) ;
#35112=CARTESIAN_POINT ( 'NONE',  ( -97.65000000000001990, 90.00000000000004263, 82.37999999999999545 ) ) ;
#35114=CARTESIAN_POINT ( 'NONE',  ( -96.15314808468752972, 91.99731107132950569, 75.72572916753382799 ) ) ;
#35115=CARTESIAN_POINT ( 'NONE',  ( 97.30629616937498838, -211.3315407142195852, 77.84239583420045960 ) ) ;
#35133=ORIENTED_EDGE ( 'NONE', *, *, #31971, .F. ) ;
#35135=CARTESIAN_POINT ( 'NONE',  ( 92.69370383062498320, 91.33154071421968467, 82.12864583420048348 ) ) ;
#35136=CARTESIAN_POINT ( 'NONE',  ( 97.64999999999997726, -211.5299782133524502, 75.65958333333333030 ) ) ;
#35153=CARTESIAN_POINT ( 'NONE',  ( -97.64999999999994884, -208.4700217866474645, 78.59645833506763779 ) ) ;
#35157=CARTESIAN_POINT ( 'NONE',  ( 93.67499999999999716, 87.70503267997126784, 80.02520833506763154 ) ) ;
#35158=CARTESIAN_POINT ( 'NONE',  ( -96.32500000000001705, 87.70503267997129626, 80.02520833506763154 ) ) ;
#35159=ORIENTED_EDGE ( 'NONE', *, *, #71085, .F. ) ;
#35160=CARTESIAN_POINT ( 'NONE',  ( 97.30629616937498838, 90.00000000000002842, 78.68906250086715204 ) ) ;
#35161=CARTESIAN_POINT ( 'NONE',  ( 94.99999999999998579, 86.94004357329502852, 75.55375000000000796 ) ) ;
#35167=CARTESIAN_POINT ( 'NONE',  ( 93.67500000000001137, -207.7050326799711968, 77.19416666666666060 ) ) ;
#35173=VERTEX_POINT ( 'NONE', #51097 ) ;
#35178=( BOUNDED_CURVE ( )  B_SPLINE_CURVE ( 2, ( #39174, #50057, #73734, #49331, #68112, #72985, #10586 ),
 .UNSPECIFIED., .F., .F. ) 
 B_SPLINE_CURVE_WITH_KNOTS ( ( 3, 2, 2, 3 ),
 ( 0.1666666666666666852, 0.1736111111111111049, 0.1805555555555554970, 0.1874999999999999167 ),
 .UNSPECIFIED. ) 
 CURVE ( )  GEOMETRIC_REPRESENTATION_ITEM ( )  RATIONAL_B_SPLINE_CURVE ( ( 0.9999999999999994449, 0.8660254037844392627, 1.000000000000000000, 0.8660254037844387076, 1.000000000000000000, 0.8660254037844402619, 0.9999999999999984457 ) ) 
 REPRESENTATION_ITEM ( '' )  );
#35179=CARTESIAN_POINT ( 'NONE',  ( -94.99999999999997158, -212.6630814284392557, 79.16531250086715943 ) ) ;
#35186=CYLINDRICAL_SURFACE ( 'NONE', #65661, 2.649999999999985700 ) ;
#35189=DIRECTION ( 'NONE',  ( 1.000000000000000000, 0.000000000000000000, 0.000000000000000000 ) ) ;
#35193=CARTESIAN_POINT ( 'NONE',  ( 92.69370383062498320, 91.33154071421968467, 87.20864583420048177 ) ) ;
#35194=CARTESIAN_POINT ( 'NONE',  ( -96.15314808468747287, -208.0026889286704943, 89.69572916753382685 ) ) ;
#35198=CARTESIAN_POINT ( 'NONE',  ( -93.84685191531252713, 88.00268892867056536, 77.15447916753380753 ) ) ;
#35199=CARTESIAN_POINT ( 'NONE',  ( 95.00000000000000000, -207.3369185715606307, 86.94406250086714749 ) ) ;
#35202=CARTESIAN_POINT ( 'NONE',  ( 96.32499999999998863, -207.7050326799711968, 87.24833333333333485 ) ) ;
#35209=EDGE_CURVE ( 'NONE', #3737, #14250, #34180, .T. ) ;
#35211=ORIENTED_EDGE ( 'NONE', *, *, #157, .T. ) ;
#35213=CARTESIAN_POINT ( 'NONE',  ( 95.00000000000000000, -212.6630814284392557, 82.34031250086714238 ) ) ;
#35222=CARTESIAN_POINT ( 'NONE',  ( 96.32499999999998863, -212.2949673200287179, 83.86166666666666458 ) ) ;
#35228=CARTESIAN_POINT ( 'NONE',  ( 96.90829729882862864, -211.8387227684681591, 74.99954709728268654 ) ) ;
#35232=CARTESIAN_POINT ( 'NONE',  ( -92.69370383062504004, 90.00000000000004263, 87.57906250086715261 ) ) ;
#35235=CARTESIAN_POINT ( 'NONE',  ( 95.00000000000000000, -206.9400435732949575, 75.31562500173430408 ) ) ;
#35236=CARTESIAN_POINT ( 'NONE',  ( 97.64999999999997726, 88.47002178664753558, 76.92958333333332632 ) ) ;
#35239=CARTESIAN_POINT ( 'NONE',  ( 97.65000000000000568, 91.52997821335252127, 79.57541666666666913 ) ) ;
#35245=CARTESIAN_POINT ( 'NONE',  ( -97.30629616937501680, 88.66845928578038638, 81.59947916753382913 ) ) ;
#35246=CARTESIAN_POINT ( 'NONE',  ( 92.69370383062498320, 88.66845928578037217, 76.36072916753381890 ) ) ;
#35257=CARTESIAN_POINT ( 'NONE',  ( -92.69370383062498320, -209.9999999999999716, 74.72031250086713783 ) ) ;
#35266=CARTESIAN_POINT ( 'NONE',  ( -94.99999999999997158, -207.3369185715606307, 88.37281250086715545 ) ) ;
#35267=ORIENTED_EDGE ( 'NONE', *, *, #1744, .T. ) ;
#35273=ORIENTED_EDGE ( 'NONE', *, *, #51777, .F. ) ;
#35277=CARTESIAN_POINT ( 'NONE',  ( 93.84685191531248449, 91.99731107132950569, 83.18697916753382060 ) ) ;
#35280=CARTESIAN_POINT ( 'NONE',  ( -97.65000000000010516, 91.52997821335249284, 81.05708333333332405 ) ) ;
#35283=CARTESIAN_POINT ( 'NONE',  ( -95.00000000000002842, 93.05995642670504253, 84.20562500173429044 ) ) ;
#35286=AXIS2_PLACEMENT_3D ( 'NONE', #49435, #55075, #8102 ) ;
#35290=CARTESIAN_POINT ( 'NONE',  ( -95.00000000000002842, 92.66308142843932671, 88.84906250086713442 ) ) ;
#35300=CARTESIAN_POINT ( 'NONE',  ( 97.64999999999999147, 90.00000000000002842, 76.98250000000000171 ) ) ;
#35306=CARTESIAN_POINT ( 'NONE',  ( 96.15314808468750130, -211.9973110713294489, 85.56822916753381492 ) ) ;
#35313=CARTESIAN_POINT ( 'NONE',  ( -97.65000000000001990, 90.00000000000004263, 90.00000000000000000 ) ) ;
#35315=EDGE_CURVE ( 'NONE', #3278, #25333, #19828, .T. ) ;
#35317=CARTESIAN_POINT ( 'NONE',  ( 97.30629616937498838, -209.9999999999999716, 78.68906250086715204 ) ) ;
#35327=CARTESIAN_POINT ( 'NONE',  ( 12.74955575014744547, 0.001194404164628405998, -80.00000000000001421 ) ) ;
#35328=CARTESIAN_POINT ( 'NONE',  ( 93.67500000000001137, -207.7050326799711968, 85.52854166840096184 ) ) ;
#35329=CARTESIAN_POINT ( 'NONE',  ( 97.64999999999997726, 88.47002178664753558, 88.35958333333333314 ) ) ;
#35333=EDGE_CURVE ( 'NONE', #9811, #48440, #42779, .T. ) ;
#35336=ORIENTED_EDGE ( 'NONE', *, *, #1649, .T. ) ;
#35340=CARTESIAN_POINT ( 'NONE',  ( 93.67499999999999716, 87.70503267997126784, 87.01020833506763097 ) ) ;
#35348=VERTEX_POINT ( 'NONE', #37145 ) ;
#35350=VERTEX_POINT ( 'NONE', #53318 ) ;
#35353=CARTESIAN_POINT ( 'NONE',  ( -95.00000000000002842, 86.94004357329504273, 86.34874999999999545 ) ) ;
#35359=LINE ( 'NONE', #58283, #46822 ) ;
#35360=CARTESIAN_POINT ( 'NONE',  ( -97.30629616937495996, -209.9999999999999716, 83.29281250086714294 ) ) ;
#35365=CARTESIAN_POINT ( 'NONE',  ( -96.15314808468747287, -208.0026889286704943, 77.47197916753380298 ) ) ;
#35368=CARTESIAN_POINT ( 'NONE',  ( -92.35000000000005116, 88.47002178664754979, 85.26395833506762756 ) ) ;
#35371=CARTESIAN_POINT ( 'NONE',  ( 97.64999999999999147, 90.00000000000002842, 88.41249999999999432 ) ) ;
#35373=CARTESIAN_POINT ( 'NONE',  ( -92.69370383062502583, 91.33154071421968467, 78.58322916753381548 ) ) ;
#35383=CARTESIAN_POINT ( 'NONE',  ( -92.69370383062498320, -208.6684592857803011, 77.47197916753381719 ) ) ;
#35387=VERTEX_POINT ( 'NONE', #2600 ) ;
#35391=EDGE_CURVE ( 'NONE', #66421, #71848, #41322, .T. ) ;
#35393=EDGE_CURVE ( 'NONE', #34509, #69471, #30758, .T. ) ;
#35399=( BOUNDED_CURVE ( )  B_SPLINE_CURVE ( 2, ( #22514, #17977, #57842, #40919, #57103, #45458, #39809 ),
 .UNSPECIFIED., .F., .T. ) 
 B_SPLINE_CURVE_WITH_KNOTS ( ( 3, 2, 2, 3 ),
 ( 0.5416666666666665186, 0.5486111111111110494, 0.5555555555555553582, 0.5624999999999997780 ),
 .UNSPECIFIED. ) 
 CURVE ( )  GEOMETRIC_REPRESENTATION_ITEM ( )  RATIONAL_B_SPLINE_CURVE ( ( 1.000000000000002220, 0.8660254037844365982, 1.000000000000000000, 0.8660254037844387076, 1.000000000000000000, 0.8660254037844430375, 0.9999999999999956701 ) ) 
 REPRESENTATION_ITEM ( '' )  );
#35400=CARTESIAN_POINT ( 'NONE',  ( 92.69370383062501162, -208.6684592857803295, 83.87489583420047268 ) ) ;
#35404=CARTESIAN_POINT ( 'NONE',  ( 92.69370383062501162, -208.6684592857803011, 89.74864583420048803 ) ) ;
#35408=CARTESIAN_POINT ( 'NONE',  ( -96.15314808468751551, 88.00268892867056536, 81.01739583420049939 ) ) ;
#35410=VERTEX_POINT ( 'NONE', #50252 ) ;
#35412=ORIENTED_EDGE ( 'NONE', *, *, #3587, .T. ) ;
#35414=EDGE_CURVE ( 'NONE', #30764, #37620, #54285, .T. ) ;
#35416=CARTESIAN_POINT ( 'NONE',  ( 92.34999999999999432, 88.47002178664752137, 80.60729166840097548 ) ) ;
#35418=CARTESIAN_POINT ( 'NONE',  ( 93.89144186338212705, 87.63060383671354714, 74.97612907457775577 ) ) ;
#35423=CARTESIAN_POINT ( 'NONE',  ( 95.00000000000000000, -207.3369185715606307, 83.13406250086714522 ) ) ;
#35428=CARTESIAN_POINT ( 'NONE',  ( 96.32499999999998863, 87.70503267997126784, 85.13166666666666060 ) ) ;
#35430=DIRECTION ( 'NONE',  ( -0.000000000000000000, -0.000000000000000000, 1.000000000000000000 ) ) ;
#35432=CARTESIAN_POINT ( 'NONE',  ( -92.69370383062498320, -208.6684592857803011, 83.66322916753379957 ) ) ;
#35433=CARTESIAN_POINT ( 'NONE',  ( -92.69370383062502583, 91.33154071421968467, 82.55197916753382970 ) ) ;
#35435=CARTESIAN_POINT ( 'NONE',  ( 94.99999999999998579, 87.33691857156068750, 85.35656250086714181 ) ) ;
#35442=DIRECTION ( 'NONE',  ( -1.000000000000000000, 3.061616997868383141E-16, -0.000000000000000000 ) ) ;
#35444=CARTESIAN_POINT ( 'NONE',  ( -92.69370383062498320, -211.3315407142195852, 87.36739583420047950 ) ) ;
#35451=CARTESIAN_POINT ( 'NONE',  ( -92.35000000000005116, 91.52997821335253548, 77.67041666666665378 ) ) ;
#35453=CARTESIAN_POINT ( 'NONE',  ( -96.15314808468752972, 91.99731107132950569, 88.26697916753380468 ) ) ;
#35463=DIRECTION ( 'NONE',  ( -0.000000000000000000, -0.000000000000000000, 1.000000000000000000 ) ) ;
#35469=CARTESIAN_POINT ( 'NONE',  ( -94.99999999999997158, -207.3369185715606307, 85.83281250086714920 ) ) ;
#35472=CARTESIAN_POINT ( 'NONE',  ( 96.15314808468748708, 91.99731107132950569, 77.52489583420047836 ) ) ;
#35473=CARTESIAN_POINT ( 'NONE',  ( -96.15314808468747287, -208.0026889286704943, 76.99572916753382401 ) ) ;
#35478=CARTESIAN_POINT ( 'NONE',  ( 23.50000000000000355, -120.0000000000000000, -64.00000000000000000 ) ) ;
#35479=CARTESIAN_POINT ( 'NONE',  ( 92.35000000006144205, 90.00001182123735077, 81.82400613091868991 ) ) ;
#35481=CARTESIAN_POINT ( 'NONE',  ( -92.69370383062504004, 90.00000000000004263, 76.14906250086716000 ) ) ;
#35482=CARTESIAN_POINT ( 'NONE',  ( 95.00000000000000000, -207.3369185715606307, 76.14906250086716000 ) ) ;
#35483=ORIENTED_EDGE ( 'NONE', *, *, #20955, .F. ) ;
#35485=ADVANCED_FACE ( 'NONE', ( #55541 ), #38240, .F. ) ;
#35487=CARTESIAN_POINT ( 'NONE',  ( 94.99999999999998579, 90.00000000000002842, 90.00000000000000000 ) ) ;
#35488=EDGE_CURVE ( 'NONE', #11208, #21866, #31217, .T. ) ;
#35494=ORIENTED_EDGE ( 'NONE', *, *, #33327, .T. ) ;
#35498=CARTESIAN_POINT ( 'NONE',  ( 97.65000000000000568, -208.4700217866474645, 79.65479166840096070 ) ) ;
#35500=ORIENTED_EDGE ( 'NONE', *, *, #32311, .F. ) ;
#35504=CARTESIAN_POINT ( 'NONE',  ( 94.99999999999998579, 92.66308142843935514, 82.02281250086714692 ) ) ;
#35519=CARTESIAN_POINT ( 'NONE',  ( -96.32499999999996021, -207.7050326799711968, 79.81354166840095843 ) ) ;
#35523=CARTESIAN_POINT ( 'NONE',  ( 96.32499999999997442, 92.29496732002878900, 80.97770833506763211 ) ) ;
#35524=CARTESIAN_POINT ( 'NONE',  ( -97.65000000000001990, 88.47002178664754979, 76.79729166840095900 ) ) ;
#35526=CARTESIAN_POINT ( 'NONE',  ( 96.15314808468748708, 88.00268892867053694, 81.12322916753382174 ) ) ;
#35527=CARTESIAN_POINT ( 'NONE',  ( 93.67499999999999716, 87.70503267997126784, 75.50083333333331836 ) ) ;
#35536=CARTESIAN_POINT ( 'NONE',  ( -93.09170270117142820, -211.8387227684682159, 74.99954709728268654 ) ) ;
#35539=CARTESIAN_POINT ( 'NONE',  ( -93.84685191531247028, -211.9973110713294489, 76.04322916753382344 ) ) ;
#35542=EDGE_CURVE ( 'NONE', #31963, #36799, #45388, .T. ) ;
#35547=CARTESIAN_POINT ( 'NONE',  ( 96.32499999999998863, 87.70503267997126784, 85.84604166840097150 ) ) ;
#35549=CARTESIAN_POINT ( 'NONE',  ( -95.00000000000002842, 90.00000000000004263, 90.00000000000000000 ) ) ;
#35556=LINE ( 'NONE', #52860, #6453 ) ;
#35557=CARTESIAN_POINT ( 'NONE',  ( 92.34999999999999432, 90.00000000000002842, 90.00000000000000000 ) ) ;
#35560=EDGE_CURVE ( 'NONE', #35348, #71136, #72490, .T. ) ;
#35561=CARTESIAN_POINT ( 'NONE',  ( 92.69370383062498320, 91.33154071421968467, 88.47864583420047779 ) ) ;
#35562=CARTESIAN_POINT ( 'NONE',  ( -96.15314808468745866, -211.9973110713294489, 88.00239583420048461 ) ) ;
#35566=CARTESIAN_POINT ( 'NONE',  ( -97.64999999999994884, -208.4700217866474645, 82.96208333333333940 ) ) ;
#35567=CARTESIAN_POINT ( 'NONE',  ( -97.30629616937501680, 88.66845928578038638, 77.63072916753380071 ) ) ;
#35568=CARTESIAN_POINT ( 'NONE',  ( 97.30629616937498838, -211.3315407142195852, 88.00239583420047040 ) ) ;
#35571=ORIENTED_EDGE ( 'NONE', *, *, #24955, .F. ) ;
#35578=CARTESIAN_POINT ( 'NONE',  ( 97.30629616937498838, -211.3315407142195852, 81.81114583420048803 ) ) ;
#35585=CARTESIAN_POINT ( 'NONE',  ( 96.32499999999998863, -207.7050326799711968, 85.34333333333333371 ) ) ;
#35592=CARTESIAN_POINT ( 'NONE',  ( -93.84685191531254134, 91.99731107132950569, 87.68489583420048916 ) ) ;
#35597=CARTESIAN_POINT ( 'NONE',  ( 96.32499999999998863, -212.2949673200287179, 75.05104166840095559 ) ) ;
#35598=CARTESIAN_POINT ( 'NONE',  ( 92.34999999999999432, 91.52997821335252127, 77.88208333333332689 ) ) ;
#35600=CARTESIAN_POINT ( 'NONE',  ( -92.34999999999999432, -208.4700217866474645, 87.90979166840095615 ) ) ;
#35601=ORIENTED_EDGE ( 'NONE', *, *, #6785, .F. ) ;
#35605=CARTESIAN_POINT ( 'NONE',  ( -97.65000000000001990, 91.52997821335253548, 87.48645833506763836 ) ) ;
#35606=( BOUNDED_CURVE ( )  B_SPLINE_CURVE ( 2, ( #63229, #18449, #51182, #11689, #39924, #62872, #28992, #6090, #51926 ),
 .UNSPECIFIED., .F., .F. ) 
 B_SPLINE_CURVE_WITH_KNOTS ( ( 3, 2, 2, 2, 3 ),
 ( 0.2540073681283128160, 0.2540075594717651764, 0.2610633250126475624, 0.2681190905535300040, 0.2751748541904413536 ),
 .UNSPECIFIED. ) 
 CURVE ( )  GEOMETRIC_REPRESENTATION_ITEM ( )  RATIONAL_B_SPLINE_CURVE ( ( 0.9999927337532890093, 0.9999963667781160970, 1.000000000000000000, 0.8660254037844387076, 1.000000000000000000, 0.8660254037844387076, 1.000000000000000000, 0.8660254037844387076, 1.000000000000000000 ) ) 
 REPRESENTATION_ITEM ( '' )  );
#35607=CARTESIAN_POINT ( 'NONE',  ( 96.15314808468748708, 88.00268892867053694, 75.24947916753380639 ) ) ;
#35608=VERTEX_POINT ( 'NONE', #34451 ) ;
#35609=CARTESIAN_POINT ( 'NONE',  ( 97.64999999999999147, -209.9999999999999716, 83.96750000000000114 ) ) ;
#35613=DIRECTION ( 'NONE',  ( 1.000000000000000000, 0.000000000000000000, 0.000000000000000000 ) ) ;
#35622=CARTESIAN_POINT ( 'NONE',  ( -94.99999999999997158, -207.3369185715606307, 87.73781250086715033 ) ) ;
#35628=DIRECTION ( 'NONE',  ( 1.000000000000000000, 0.000000000000000000, 0.000000000000000000 ) ) ;
#35629=CARTESIAN_POINT ( 'NONE',  ( 97.30629616937498838, 91.33154071421968467, 83.02822916753379445 ) ) ;
#35640=LINE ( 'NONE', #48046, #30015 ) ;
#35643=CARTESIAN_POINT ( 'NONE',  ( -97.30629616937501680, 91.33154071421968467, 85.14489583420045449 ) ) ;
#35646=EDGE_CURVE ( 'NONE', #43675, #45993, #63787, .T. ) ;
#35652=CARTESIAN_POINT ( 'NONE',  ( 97.64999999999999147, 90.00000000000002842, 90.00000000000000000 ) ) ;
#35658=CARTESIAN_POINT ( 'NONE',  ( 93.84685191531251292, -211.9973110713294489, 81.65239583420049030 ) ) ;
#35665=CARTESIAN_POINT ( 'NONE',  ( 95.00000000000000000, -212.6630814284392557, 75.83156250086715033 ) ) ;
#35667=CARTESIAN_POINT ( 'NONE',  ( 93.84685191531249870, -208.0026889286704943, 80.80572916753382628 ) ) ;
#35668=ORIENTED_EDGE ( 'NONE', *, *, #68576, .F. ) ;
#35672=LINE ( 'NONE', #23666, #4596 ) ;
#35673=( LENGTH_UNIT ( ) NAMED_UNIT ( * ) SI_UNIT ( .MILLI., .METRE. ) );
#35674=CARTESIAN_POINT ( 'NONE',  ( -15.70044424985254850, 0.001194404164626844313, -85.59999999999999432 ) ) ;
#35677=CARTESIAN_POINT ( 'NONE',  ( 96.32499999999998863, -207.7050326799711968, 84.15270833506762926 ) ) ;
#35678=CARTESIAN_POINT ( 'NONE',  ( 92.34999999999999432, 91.52997821335252127, 88.67708333333332860 ) ) ;
#35680=CARTESIAN_POINT ( 'NONE',  ( 97.65000000000000568, 91.52997821335252127, 84.73479166840094479 ) ) ;
#35681=CARTESIAN_POINT ( 'NONE',  ( -94.26819495033768703, 87.36255141571193406, 75.02735117824596500 ) ) ;
#35685=ORIENTED_EDGE ( 'NONE', *, *, #39550, .F. ) ;
#35687=CARTESIAN_POINT ( 'NONE',  ( 92.34999999999999432, 91.52997821335252127, 86.21645833506764234 ) ) ;
#35690=CARTESIAN_POINT ( 'NONE',  ( -94.99999999999997158, -213.0599564267049857, 78.17312500173430578 ) ) ;
#35691=CARTESIAN_POINT ( 'NONE',  ( -92.34999999999990905, -208.4700217866474929, 75.13041666666666174 ) ) ;
#35698=CARTESIAN_POINT ( 'NONE',  ( 97.64999999999993463, 91.52997821335253548, 81.48041666666665606 ) ) ;
#35699=CARTESIAN_POINT ( 'NONE',  ( -92.35000000000003695, 90.00000000000004263, 88.41249999999999432 ) ) ;
#35701=DIRECTION ( 'NONE',  ( -0.000000000000000000, -0.000000000000000000, 1.000000000000000000 ) ) ;
#35702=EDGE_CURVE ( 'NONE', #65117, #14143, #29540, .T. ) ;
#35704=VERTEX_POINT ( 'NONE', #70133 ) ;
#35706=CARTESIAN_POINT ( 'NONE',  ( -97.30629616937497417, -211.3315407142195852, 83.34572916753380412 ) ) ;
#35715=EDGE_CURVE ( 'NONE', #35704, #16558, #15861, .T. ) ;
#35722=CARTESIAN_POINT ( 'NONE',  ( -95.00000000000002842, 92.66308142843932671, 79.95906250086713385 ) ) ;
#35727=DIRECTION ( 'NONE',  ( 4.476705744456277943E-17, -1.000000000000000000, 0.000000000000000000 ) ) ;
#35729=DIRECTION ( 'NONE',  ( -0.000000000000000000, -0.000000000000000000, 1.000000000000000000 ) ) ;
#35732=CARTESIAN_POINT ( 'NONE',  ( -97.30629616937497417, -211.3315407142195852, 75.88447916753382572 ) ) ;
#35734=CARTESIAN_POINT ( 'NONE',  ( 94.99999999999998579, 90.00000000000002842, 90.00000000000000000 ) ) ;
#35746=ORIENTED_EDGE ( 'NONE', *, *, #20951, .F. ) ;
#35749=ORIENTED_EDGE ( 'NONE', *, *, #53135, .T. ) ;
#35750=CARTESIAN_POINT ( 'NONE',  ( 97.30629616937498838, -208.6684592857803295, 84.29822916753380468 ) ) ;
#35751=CARTESIAN_POINT ( 'NONE',  ( 95.00000000000000000, -207.3369185715606307, 89.00781250086716057 ) ) ;
#35753=CARTESIAN_POINT ( 'NONE',  ( 97.30629616937498838, -209.9999999999999716, 88.84906250086716284 ) ) ;
#35757=CARTESIAN_POINT ( 'NONE',  ( -92.69370383062504004, 90.00000000000004263, 79.95906250086714806 ) ) ;
#35760=ORIENTED_EDGE ( 'NONE', *, *, #68143, .T. ) ;
#35764=EDGE_LOOP ( 'NONE', ( #10530, #65306, #40001, #61226 ) ) ;
#35766=CYLINDRICAL_SURFACE ( 'NONE', #60883, 15.70000000000000284 ) ;
#35769=FACE_OUTER_BOUND ( 'NONE', #29384, .T. ) ;
#35772=CARTESIAN_POINT ( 'NONE',  ( 92.35000000000000853, -209.9999844236436672, 80.55437446300187787 ) ) ;
#35777=CARTESIAN_POINT ( 'NONE',  ( 95.00000000000000000, -212.6630814284392557, 81.54656250086715374 ) ) ;
#35782=CARTESIAN_POINT ( 'NONE',  ( -96.32499999999996021, -207.7050326799711968, 89.25916666666667254 ) ) ;
#35786=CARTESIAN_POINT ( 'NONE',  ( -97.30629616937495996, -209.9999999999999716, 83.29281250086714294 ) ) ;
#35787=EDGE_CURVE ( 'NONE', #65641, #64543, #57146, .T. ) ;
#35788=CARTESIAN_POINT ( 'NONE',  ( -97.30629616937501680, 88.66845928578038638, 80.96447916753382401 ) ) ;
#35790=CARTESIAN_POINT ( 'NONE',  ( 96.15314808468748708, 91.99731107132950569, 79.90614583420047268 ) ) ;
#35791=EDGE_LOOP ( 'NONE', ( #47286, #40251 ) ) ;
#35792=CYLINDRICAL_SURFACE ( 'NONE', #52711, 2.649999999999985700 ) ;
#35798=CARTESIAN_POINT ( 'NONE',  ( -96.15314808468745866, -211.9973110713294489, 85.93864583420048575 ) ) ;
#35809=CARTESIAN_POINT ( 'NONE',  ( -92.35000000000005116, 91.52997821335253548, 75.13041666666666174 ) ) ;
#35818=CARTESIAN_POINT ( 'NONE',  ( -96.15314808468752972, 91.99731107132950569, 74.93197916753379673 ) ) ;
#35822=CARTESIAN_POINT ( 'NONE',  ( 92.35000000000002274, -210.0000225213918554, 84.36437578067152288 ) ) ;
#35825=CARTESIAN_POINT ( 'NONE',  ( -97.30629616937497417, -208.6684592857803011, 86.57364583420047666 ) ) ;
#35832=( BOUNDED_CURVE ( )  B_SPLINE_CURVE ( 2, ( #72414, #43868, #14536, #3292, #56253, #21659, #73156 ),
 .UNSPECIFIED., .F., .F. ) 
 B_SPLINE_CURVE_WITH_KNOTS ( ( 3, 2, 2, 3 ),
 ( 0.7916666666666669627, 0.7986111111111114935, 0.8055555555555558023, 0.8125000000000002220 ),
 .UNSPECIFIED. ) 
 CURVE ( )  GEOMETRIC_REPRESENTATION_ITEM ( )  RATIONAL_B_SPLINE_CURVE ( ( 0.9999999999999935607, 0.8660254037844451469, 1.000000000000000000, 0.8660254037844387076, 1.000000000000000000, 0.8660254037844343777, 1.000000000000004219 ) ) 
 REPRESENTATION_ITEM ( '' )  );
#35834=CARTESIAN_POINT ( 'NONE',  ( 92.35000000006144205, 90.00001182178868930, 76.10900611559256390 ) ) ;
#35835=CARTESIAN_POINT ( 'NONE',  ( -92.69370383062498320, -208.6684592857803295, 74.93197916753381094 ) ) ;
#35837=ORIENTED_EDGE ( 'NONE', *, *, #2151, .T. ) ;
#35840=DIRECTION ( 'NONE',  ( -0.000000000000000000, -0.000000000000000000, 1.000000000000000000 ) ) ;
#35841=CARTESIAN_POINT ( 'NONE',  ( -92.69370383062505425, 88.66845928578038638, 75.46114583420049371 ) ) ;
#35842=CARTESIAN_POINT ( 'NONE',  ( 97.30629616937498838, -208.6684592857803011, 76.67822916753378593 ) ) ;
#35847=DIRECTION ( 'NONE',  ( -0.000000000000000000, -0.000000000000000000, 1.000000000000000000 ) ) ;
#35848=ORIENTED_EDGE ( 'NONE', *, *, #5879, .F. ) ;
#35851=CARTESIAN_POINT ( 'NONE',  ( -97.64999999992180335, 90.00001303125199570, 79.28395951162846700 ) ) ;
#35857=CARTESIAN_POINT ( 'NONE',  ( -97.64999999999996305, -209.9999999999999716, 77.29999999999999716 ) ) ;
#35860=CARTESIAN_POINT ( 'NONE',  ( 97.30629616937498838, 88.66845928578037217, 78.63614583420049087 ) ) ;
#35861=DIRECTION ( 'NONE',  ( -3.061616997868382648E-16, -1.000000000000000000, -5.966227995846078450E-16 ) ) ;
#35862=CARTESIAN_POINT ( 'NONE',  ( 97.64999999999997726, -208.4700217866474645, 75.76541666666666686 ) ) ;
#35868=ORIENTED_EDGE ( 'NONE', *, *, #49340, .T. ) ;
#35874=CARTESIAN_POINT ( 'NONE',  ( 93.67499999999999716, 87.70503267997126784, 83.75583333333332803 ) ) ;
#35877=ADVANCED_FACE ( 'NONE', ( #59996 ), #32870, .F. ) ;
#35878=DIRECTION ( 'NONE',  ( 0.000000000000000000, -0.000000000000000000, -1.000000000000000000 ) ) ;
#35881=CARTESIAN_POINT ( 'NONE',  ( -97.64999999999996305, -209.9999999999999716, 79.28437500173430408 ) ) ;
#35885=CARTESIAN_POINT ( 'NONE',  ( 94.99999999999998579, 86.94004357329500010, 76.90312500173429555 ) ) ;
#35886=CARTESIAN_POINT ( 'NONE',  ( -96.32500000000001705, 92.29496732002878900, 76.00354166840097037 ) ) ;
#35887=AXIS2_PLACEMENT_3D ( 'NONE', #67104, #72370, #61481 ) ;
#35889=CARTESIAN_POINT ( 'NONE',  ( 93.84685191531248449, 91.99731107132950569, 80.17072916753382117 ) ) ;
#35898=LINE ( 'NONE', #12602, #42015 ) ;
#35902=CARTESIAN_POINT ( 'NONE',  ( 97.64999999999999147, -209.9999999999999716, 90.00000000000000000 ) ) ;
#35907=CARTESIAN_POINT ( 'NONE',  ( -96.15314808468745866, -211.9973110713294489, 77.84239583420048803 ) ) ;
#35914=DIRECTION ( 'NONE',  ( -0.000000000000000000, -0.000000000000000000, 1.000000000000000000 ) ) ;
#35915=DIRECTION ( 'NONE',  ( -1.000000000000000000, 0.000000000000000000, 0.000000000000000000 ) ) ;
#35916=DIRECTION ( 'NONE',  ( -0.000000000000000000, -0.000000000000000000, -1.000000000000000000 ) ) ;
#35920=CARTESIAN_POINT ( 'NONE',  ( -94.99999999999997158, -209.9999999999999716, 90.00000000000000000 ) ) ;
#35926=CARTESIAN_POINT ( 'NONE',  ( 97.30629616937498838, 91.33154071421968467, 82.55197916753380127 ) ) ;
#35928=CARTESIAN_POINT ( 'NONE',  ( -97.30629616937497417, -208.6684592857803295, 86.57364583420047666 ) ) ;
#35933=CARTESIAN_POINT ( 'NONE',  ( -92.34999999999999432, -208.4700217866474645, 81.48041666666665606 ) ) ;
#35934=CARTESIAN_POINT ( 'NONE',  ( -95.00000000000002842, 92.66308142843932671, 74.87906250086713555 ) ) ;
#35939=CARTESIAN_POINT ( 'NONE',  ( 97.30629616937498838, -211.3315407142195852, 88.63739583420047552 ) ) ;
#35941=VERTEX_POINT ( 'NONE', #67094 ) ;
#35948=CARTESIAN_POINT ( 'NONE',  ( 97.30629616937498838, -211.3315407142195852, 81.17614583420049712 ) ) ;
#35950=CARTESIAN_POINT ( 'NONE',  ( 96.32499999999997442, 92.29496732002878900, 80.89833333333332632 ) ) ;
#35955=CARTESIAN_POINT ( 'NONE',  ( 92.35000000000002274, -208.4700217866474645, 85.50208333333331723 ) ) ;
#35957=EDGE_CURVE ( 'NONE', #73349, #42384, #9209, .T. ) ;
#35961=ORIENTED_EDGE ( 'NONE', *, *, #22081, .F. ) ;
#35964=CARTESIAN_POINT ( 'NONE',  ( -92.69370383062502583, 91.33154071421968467, 86.99697916753382287 ) ) ;
#35968=CARTESIAN_POINT ( 'NONE',  ( 92.69370383062501162, -208.6684592857803011, 87.68489583420047495 ) ) ;
#35970=CARTESIAN_POINT ( 'NONE',  ( 97.64999999999999147, 90.00000000000002842, 77.61749999999999261 ) ) ;
#35974=CARTESIAN_POINT ( 'NONE',  ( 92.35000000000000853, -209.9999999999999716, 79.83999999999998920 ) ) ;
#35975=ORIENTED_EDGE ( 'NONE', *, *, #12366, .F. ) ;
#35976=CARTESIAN_POINT ( 'NONE',  ( -97.65000000000001990, 88.47002178664754979, 85.05229166840096866 ) ) ;
#35977=CARTESIAN_POINT ( 'NONE',  ( 92.69370383062498320, 90.00000000000002842, 75.67281250086713840 ) ) ;
#35984=CARTESIAN_POINT ( 'NONE',  ( -97.64999999980587120, -210.0000198427943587, 86.27002759516035724 ) ) ;
#35989=CARTESIAN_POINT ( 'NONE',  ( -94.99999999999997158, -212.6630814284392557, 75.19656250086714522 ) ) ;
#35994=AXIS2_PLACEMENT_3D ( 'NONE', #67198, #19839, #15697 ) ;
#35998=CARTESIAN_POINT ( 'NONE',  ( -97.30629616937497417, -208.6684592857803011, 87.20864583420049598 ) ) ;
#36002=ORIENTED_EDGE ( 'NONE', *, *, #37623, .T. ) ;
#36004=CARTESIAN_POINT ( 'NONE',  ( -92.35001333515640454, 91.52998591240866233, 83.46479220096853169 ) ) ;
#36007=CARTESIAN_POINT ( 'NONE',  ( 97.30629616937498838, 91.33154071421968467, 89.53697916753382913 ) ) ;
#36009=CARTESIAN_POINT ( 'NONE',  ( 97.30629616937498838, 90.00000000000002842, 80.43531250086714124 ) ) ;
#36019=CARTESIAN_POINT ( 'NONE',  ( 97.64999999999990621, -209.9999992849081139, 85.31687502647973531 ) ) ;
#36023=CARTESIAN_POINT ( 'NONE',  ( -92.69370383062505425, 88.66845928578038638, 85.46239583420044994 ) ) ;
#36033=VECTOR ( 'NONE', #9292, 1000.000000000000000 ) ;
#36035=CARTESIAN_POINT ( 'NONE',  ( 97.30629616937498838, -209.9999999999999716, 82.49906250086715431 ) ) ;
#36038=ORIENTED_EDGE ( 'NONE', *, *, #12546, .F. ) ;
#36043=( BOUNDED_CURVE ( )  B_SPLINE_CURVE ( 2, ( #26583, #49516, #72438, #20941, #15301, #43897, #38238 ),
 .UNSPECIFIED., .F., .F. ) 
 B_SPLINE_CURVE_WITH_KNOTS ( ( 3, 2, 2, 3 ),
 ( 0.1874999999999999167, 0.1944444444444443365, 0.2013888888888887285, 0.2083333333333331483 ),
 .UNSPECIFIED. ) 
 CURVE ( )  GEOMETRIC_REPRESENTATION_ITEM ( )  RATIONAL_B_SPLINE_CURVE ( ( 1.000000000000001554, 0.8660254037844371533, 1.000000000000000000, 0.8660254037844387076, 1.000000000000000000, 0.8660254037844424824, 0.9999999999999962252 ) ) 
 REPRESENTATION_ITEM ( '' )  );
#36044=CARTESIAN_POINT ( 'NONE',  ( 97.30629616937498838, -208.6684592857803295, 75.40822916753381833 ) ) ;
#36046=CARTESIAN_POINT ( 'NONE',  ( 93.84685191531251292, -211.9973110713294489, 80.38239583420048007 ) ) ;
#36058=CARTESIAN_POINT ( 'NONE',  ( 96.32499999999998863, -212.2949673200287179, 82.67104166840096013 ) ) ;
#36060=CARTESIAN_POINT ( 'NONE',  ( 96.66079198124940319, 88.39975876321993553, 74.80065669543250806 ) ) ;
#36064=DIRECTION ( 'NONE',  ( -0.000000000000000000, -0.000000000000000000, 1.000000000000000000 ) ) ;
#36067=CARTESIAN_POINT ( 'NONE',  ( -92.69370383062505425, 88.66845928578038638, 86.89114583420048632 ) ) ;
#36069=CARTESIAN_POINT ( 'NONE',  ( 93.67499999999999716, 87.70503267997126784, 84.47020833506762472 ) ) ;
#36074=VECTOR ( 'NONE', #52855, 1000.000000000000000 ) ;
#36082=CARTESIAN_POINT ( 'NONE',  ( 97.64999999999999147, 90.00000000000002842, 81.42749999999999488 ) ) ;
#36084=CARTESIAN_POINT ( 'NONE',  ( -92.35000000000005116, 91.52997821335253548, 85.92541666666664923 ) ) ;
#36086=CARTESIAN_POINT ( 'NONE',  ( 7.103376864691351012E-17, -120.0000000000000000, -90.00000000000000000 ) ) ;
#36088=EDGE_LOOP ( 'NONE', ( #10157, #29102, #51065, #33547 ) ) ;
#36089=DIRECTION ( 'NONE',  ( -0.000000000000000000, -0.000000000000000000, 1.000000000000000000 ) ) ;
#36090=CARTESIAN_POINT ( 'NONE',  ( -92.69370383062498320, -209.9999999999999716, 84.24531250086714351 ) ) ;
#36098=EDGE_CURVE ( 'NONE', #13520, #23087, #61976, .T. ) ;
#36105=CARTESIAN_POINT ( 'NONE',  ( 94.99999999999998579, 93.05995642670504253, 82.93562500173430863 ) ) ;
#36107=CARTESIAN_POINT ( 'NONE',  ( -92.69370383062504004, 90.00000000000004263, 74.72031250086713783 ) ) ;
#36116=CARTESIAN_POINT ( 'NONE',  ( -92.69370383062498320, -211.3315407142195852, 76.09614583420048461 ) ) ;
#36117=FACE_OUTER_BOUND ( 'NONE', #26695, .T. ) ;
#36125=DIRECTION ( 'NONE',  ( -0.000000000000000000, -0.000000000000000000, 1.000000000000000000 ) ) ;
#36130=CARTESIAN_POINT ( 'NONE',  ( 95.00000000000000000, -212.6630814284392557, 85.99156250086714692 ) ) ;
#36131=CARTESIAN_POINT ( 'NONE',  ( 95.00000000000000000, -212.6630814284392557, 88.05531250086714579 ) ) ;
#36134=CARTESIAN_POINT ( 'NONE',  ( 96.15314808468750130, -211.9973110713294489, 89.37822916753381719 ) ) ;
#36136=ORIENTED_EDGE ( 'NONE', *, *, #73582, .F. ) ;
#36138=ORIENTED_EDGE ( 'NONE', *, *, #15200, .F. ) ;
#36140=CARTESIAN_POINT ( 'NONE',  ( -95.00000000000002842, 87.33691857156074434, 81.07031250086716057 ) ) ;
#36143=EDGE_CURVE ( 'NONE', #36383, #8621, #38914, .T. ) ;
#36155=EDGE_CURVE ( 'NONE', #43311, #49534, #17810, .T. ) ;
#36159=CARTESIAN_POINT ( 'NONE',  ( 92.69370383062501162, -211.3315407142195852, 77.63072916753380071 ) ) ;
#36167=CARTESIAN_POINT ( 'NONE',  ( -93.84685191531247028, -211.9973110713294489, 82.86947916753379673 ) ) ;
#36169=CARTESIAN_POINT ( 'NONE',  ( -92.69370383062504004, 90.00000000000004263, 83.13406250086715943 ) ) ;
#36172=CARTESIAN_POINT ( 'NONE',  ( 92.69370383062498320, 91.33154071421968467, 80.06489583420047040 ) ) ;
#36176=CARTESIAN_POINT ( 'NONE',  ( -96.32499999999996021, -212.2949673200287179, 83.20020833506764291 ) ) ;
#36179=CARTESIAN_POINT ( 'NONE',  ( -93.84685191531247028, -211.9973110713294489, 81.59947916753381492 ) ) ;
#36191=CARTESIAN_POINT ( 'NONE',  ( -92.35000000000005116, 88.93104485797731229, 75.04052853044679239 ) ) ;
#36194=CARTESIAN_POINT ( 'NONE',  ( -97.30629616937501680, 90.00000000000004263, 87.73781250086713612 ) ) ;
#36206=CARTESIAN_POINT ( 'NONE',  ( -92.69370383062498320, -211.3315407142195852, 86.25614583420048120 ) ) ;
#36211=CARTESIAN_POINT ( 'NONE',  ( -97.30629616937497417, -211.3315407142195852, 77.78947916753381264 ) ) ;
#36212=CARTESIAN_POINT ( 'NONE',  ( 92.34999999999988063, 91.52997821335246442, 88.67708333333332860 ) ) ;
#36215=CARTESIAN_POINT ( 'NONE',  ( 93.67499999999998295, 92.29496732002878900, 75.92416666666666458 ) ) ;
#36219=CARTESIAN_POINT ( 'NONE',  ( 96.15314808468748708, -208.0026889286704943, 76.09614583420047040 ) ) ;
#36223=ORIENTED_EDGE ( 'NONE', *, *, #50937, .T. ) ;
#36234=CARTESIAN_POINT ( 'NONE',  ( 93.67500000000001137, -207.7050326799711968, 76.63854166840096127 ) ) ;
#36238=ORIENTED_EDGE ( 'NONE', *, *, #55174, .F. ) ;
#36239=CARTESIAN_POINT ( 'NONE',  ( 92.69370383062498320, 90.00000000000002842, 79.64156250086715261 ) ) ;
#36242=CARTESIAN_POINT ( 'NONE',  ( 93.67500000000001137, -212.2949673200287179, 76.13583333333333769 ) ) ;
#36258=CARTESIAN_POINT ( 'NONE',  ( -96.32499999999996021, -212.2949673200287179, 78.12020833506763040 ) ) ;
#36260=CARTESIAN_POINT ( 'NONE',  ( -92.34999999999999432, -209.9999999999999716, 90.00000000000000000 ) ) ;
#36262=CARTESIAN_POINT ( 'NONE',  ( 96.32499999999998863, 87.70503267997126784, 77.59104166840097605 ) ) ;
#36263=CARTESIAN_POINT ( 'NONE',  ( -95.00000000000002842, 93.05995642670501411, 75.31562500173430408 ) ) ;
#36264=( BOUNDED_CURVE ( )  B_SPLINE_CURVE ( 2, ( #42836, #37573, #26268, #1915, #19155, #42106, #2282, #22506, #32651 ),
 .UNSPECIFIED., .F., .F. ) 
 B_SPLINE_CURVE_WITH_KNOTS ( ( 3, 2, 2, 2, 3 ),
 ( 0.9313609857393204683, 0.9313610513964742932, 0.9384168169373562352, 0.9454725824782379551, 0.9525283480321510288 ),
 .UNSPECIFIED. ) 
 CURVE ( )  GEOMETRIC_REPRESENTATION_ITEM ( )  RATIONAL_B_SPLINE_CURVE ( ( 0.9999975066323365525, 0.9999987533045672228, 1.000000000000000000, 0.8660254037844387076, 1.000000000000000000, 0.8660254037844387076, 1.000000000000000000, 0.8660254037844387076, 1.000000000000000000 ) ) 
 REPRESENTATION_ITEM ( '' )  );
#36267=CARTESIAN_POINT ( 'NONE',  ( 92.69370383062498320, 91.33154071421968467, 76.41364583420049428 ) ) ;
#36268=CARTESIAN_POINT ( 'NONE',  ( 94.99999999999998579, 93.05995642670504253, 82.22124999999999773 ) ) ;
#36279=CARTESIAN_POINT ( 'NONE',  ( -97.65000000000001990, 91.52997821335253548, 86.21645833506764234 ) ) ;
#36282=CARTESIAN_POINT ( 'NONE',  ( -96.15314808468745866, -211.9973110713294489, 79.11239583420048405 ) ) ;
#36291=CARTESIAN_POINT ( 'NONE',  ( 94.99999999999998579, 90.00000000000002842, 90.00000000000000000 ) ) ;
#36298=CARTESIAN_POINT ( 'NONE',  ( 92.69370383062498320, 88.66845928578035796, 82.23447916753383424 ) ) ;
#36299=CARTESIAN_POINT ( 'NONE',  ( -92.69370383062498320, -208.6684592857803295, 85.09197916753380753 ) ) ;
#36303=CARTESIAN_POINT ( 'NONE',  ( -97.64999999999994884, -211.5299782133524502, 79.89291666666666458 ) ) ;
#36304=CARTESIAN_POINT ( 'NONE',  ( -95.00000000000002842, 87.33691857156074434, 77.73656250086713726 ) ) ;
#36308=CARTESIAN_POINT ( 'NONE',  ( 96.15314808468750130, -211.9973110713294489, 86.04447916753380809 ) ) ;
#36313=EDGE_CURVE ( 'NONE', #14968, #42545, #61537, .T. ) ;
#36320=CARTESIAN_POINT ( 'NONE',  ( 96.15314808468750130, -211.9973110713294489, 82.39322916753381776 ) ) ;
#36327=CARTESIAN_POINT ( 'NONE',  ( 92.35000000000002274, -208.4700217866474645, 83.59708333333334451 ) ) ;
#36332=CARTESIAN_POINT ( 'NONE',  ( 95.00000000000000000, -213.0599564267049857, 86.98374999999998636 ) ) ;
#36333=CIRCLE ( 'NONE', #50722, 3.299999999999983391 ) ;
#36334=CARTESIAN_POINT ( 'NONE',  ( -97.30629616937501680, 91.33154071421968467, 85.30364583420048064 ) ) ;
#36336=FACE_OUTER_BOUND ( 'NONE', #56956, .T. ) ;
#36337=CARTESIAN_POINT ( 'NONE',  ( 92.69370383062501162, -209.9999999999999716, 87.10281250086714522 ) ) ;
#36341=ADVANCED_FACE ( 'NONE', ( #3505 ), #26409, .F. ) ;
#36347=CARTESIAN_POINT ( 'NONE',  ( -93.67500000000003979, 92.29496732002878900, 86.05770833506763040 ) ) ;
#36349=CARTESIAN_POINT ( 'NONE',  ( 92.69370383062498320, 91.33154071421968467, 87.84364583420048689 ) ) ;
#36353=CARTESIAN_POINT ( 'NONE',  ( -92.74366017909925120, 90.55049048501740572, 74.79348190356847681 ) ) ;
#36358=CARTESIAN_POINT ( 'NONE',  ( -96.15314808468745866, -211.9973110713294489, 75.77864583420047495 ) ) ;
#36359=ORIENTED_EDGE ( 'NONE', *, *, #11640, .T. ) ;
#36364=CARTESIAN_POINT ( 'NONE',  ( -93.84685191531247028, -211.9973110713294489, 86.20322916753382003 ) ) ;
#36365=ORIENTED_EDGE ( 'NONE', *, *, #58164, .F. ) ;
#36368=CARTESIAN_POINT ( 'NONE',  ( 92.35000000000000853, -209.9999999999999716, 90.00000000000000000 ) ) ;
#36369=CARTESIAN_POINT ( 'NONE',  ( 93.84685191531248449, 91.99731107132950569, 89.06072916753382174 ) ) ;
#36371=CARTESIAN_POINT ( 'NONE',  ( 96.15314808468748708, 88.00268892867053694, 80.96447916753380980 ) ) ;
#36383=VERTEX_POINT ( 'NONE', #43359 ) ;
#36384=CARTESIAN_POINT ( 'NONE',  ( -93.84685191531254134, 91.99731107132950569, 87.52614583420047722 ) ) ;
#36391=CARTESIAN_POINT ( 'NONE',  ( 92.34999999999993747, -208.4700217866475214, 83.59708333333334451 ) ) ;
#36392=AXIS2_PLACEMENT_3D ( 'NONE', #46661, #56840, #68863 ) ;
#36400=CARTESIAN_POINT ( 'NONE',  ( 96.15314808468748708, -208.0026889286704943, 82.60489583420049087 ) ) ;
#36410=CARTESIAN_POINT ( 'NONE',  ( 97.30629616937498838, -208.6684592857803011, 80.01197916753380923 ) ) ;
#36419=ORIENTED_EDGE ( 'NONE', *, *, #8646, .F. ) ;
#36420=DIRECTION ( 'NONE',  ( -0.000000000000000000, -0.000000000000000000, 1.000000000000000000 ) ) ;
#36421=CARTESIAN_POINT ( 'NONE',  ( 92.35000000000002274, -211.5299782133524502, 85.05229166840096866 ) ) ;
#36422=CARTESIAN_POINT ( 'NONE',  ( 93.67499999999999716, 87.70503267997126784, 85.02583333333332405 ) ) ;
#36423=VERTEX_POINT ( 'NONE', #51568 ) ;
#36426=CARTESIAN_POINT ( 'NONE',  ( -92.35000000000005116, 88.47002178664754979, 75.10395833506764518 ) ) ;
#36431=CARTESIAN_POINT ( 'NONE',  ( -97.30629616937501680, 90.00000000000004263, 88.53156250086716739 ) ) ;
#36432=CARTESIAN_POINT ( 'NONE',  ( 92.69370383062498320, 91.33154071421968467, 83.87489583420047268 ) ) ;
#36434=CARTESIAN_POINT ( 'NONE',  ( 97.64999999999997726, 91.52997821335252127, 86.00479166840096923 ) ) ;
#36445=CARTESIAN_POINT ( 'NONE',  ( -97.65000000000001990, 90.00000000000004263, 85.55499999999999261 ) ) ;
#36447=DIRECTION ( 'NONE',  ( -0.000000000000000000, -0.000000000000000000, 1.000000000000000000 ) ) ;
#36452=CARTESIAN_POINT ( 'NONE',  ( -92.69370383062498320, -211.3315407142195852, 82.28739583420048120 ) ) ;
#36466=CARTESIAN_POINT ( 'NONE',  ( -92.69370383062502583, 88.66845928578038638, 89.43114583420049257 ) ) ;
#36474=CARTESIAN_POINT ( 'NONE',  ( 95.04693102382854875, 87.35041560265749183, 75.00000002508419072 ) ) ;
#36478=CARTESIAN_POINT ( 'NONE',  ( -96.32499999999996021, -207.7050326799711968, 87.35416666666665719 ) ) ;
#36480=DIRECTION ( 'NONE',  ( 0.000000000000000000, 0.000000000000000000, 1.000000000000000000 ) ) ;
#36482=( BOUNDED_CURVE ( )  B_SPLINE_CURVE ( 2, ( #405, #57879, #64999, #23297, #12367, #63527, #6381 ),
 .UNSPECIFIED., .F., .F. ) 
 B_SPLINE_CURVE_WITH_KNOTS ( ( 3, 2, 2, 3 ),
 ( 0.2499999999999995837, 0.2569444444444442532, 0.2638888888888890061, 0.2708333333333337034 ),
 .UNSPECIFIED. ) 
 CURVE ( )  GEOMETRIC_REPRESENTATION_ITEM ( )  RATIONAL_B_SPLINE_CURVE ( ( 1.000000000000007994, 0.8660254037844307140, 1.000000000000000000, 0.8660254037844387076, 1.000000000000000000, 0.8660254037844311581, 1.000000000000007550 ) ) 
 REPRESENTATION_ITEM ( '' )  );
#36486=CARTESIAN_POINT ( 'NONE',  ( -97.65000000000001990, 90.00000000000004263, 84.92000000000000171 ) ) ;
#36494=CARTESIAN_POINT ( 'NONE',  ( 95.00000000000000000, -207.3369185715606307, 83.76906250086715033 ) ) ;
#36495=CARTESIAN_POINT ( 'NONE',  ( 97.30629616937498838, -211.3315407142195852, 88.79614583420048746 ) ) ;
#36506=CARTESIAN_POINT ( 'NONE',  ( -93.84685191531254134, 91.99731107132950569, 81.96989583420048575 ) ) ;
#36507=ORIENTED_EDGE ( 'NONE', *, *, #10535, .F. ) ;
#36521=ORIENTED_EDGE ( 'NONE', *, *, #54498, .T. ) ;
#36523=CARTESIAN_POINT ( 'NONE',  ( 93.84685191531251292, -211.9973110713294489, 77.04864583420047097 ) ) ;
#36525=CARTESIAN_POINT ( 'NONE',  ( -96.32499999999996021, -212.2949673200287179, 85.74020833506763495 ) ) ;
#36526=EDGE_LOOP ( 'NONE', ( #9817, #62566, #39022, #45418 ) ) ;
#36530=CARTESIAN_POINT ( 'NONE',  ( -92.35000000005462084, -210.0000170173125014, 88.49187441316038871 ) ) ;
#36532=CARTESIAN_POINT ( 'NONE',  ( -93.84685191531248449, -208.0026889286704943, 81.17614583420048291 ) ) ;
#36533=CARTESIAN_POINT ( 'NONE',  ( -97.30629616937501680, 91.33154071421968467, 77.68364583420047609 ) ) ;
#36536=CARTESIAN_POINT ( 'NONE',  ( 97.30629616937498838, 91.33154071421968467, 81.75822916753381264 ) ) ;
#36543=CARTESIAN_POINT ( 'NONE',  ( -97.30629616937497417, -211.3315407142195852, 83.98072916753380923 ) ) ;
#36549=ORIENTED_EDGE ( 'NONE', *, *, #64082, .T. ) ;
#36551=CARTESIAN_POINT ( 'NONE',  ( -97.65000000000001990, 91.52997821335253548, 75.34208333333333485 ) ) ;
#36553=CARTESIAN_POINT ( 'NONE',  ( -92.69370383062504004, 90.00000000000004263, 84.24531250086714351 ) ) ;
#36562=CARTESIAN_POINT ( 'NONE',  ( -93.84685191531254134, 91.99731107132950569, 76.09614583420047040 ) ) ;
#36567=EDGE_CURVE ( 'NONE', #31031, #4841, #34642, .T. ) ;
#36570=CARTESIAN_POINT ( 'NONE',  ( -93.84685191531248449, -208.0026889286704943, 84.50989583420049200 ) ) ;
#36571=VECTOR ( 'NONE', #66266, 1000.000000000000114 ) ;
#36578=CARTESIAN_POINT ( 'NONE',  ( -96.15314808468745866, -211.9973110713294489, 77.84239583420048803 ) ) ;
#36579=CARTESIAN_POINT ( 'NONE',  ( 97.65000000000004832, 91.52997821335247863, 88.46541666666664128 ) ) ;
#36581=CARTESIAN_POINT ( 'NONE',  ( 99.99999999999998579, 95.00000000000002842, 90.00000000000000000 ) ) ;
#36586=CARTESIAN_POINT ( 'NONE',  ( 97.30629616937498838, -208.6684592857803011, 89.53697916753382913 ) ) ;
#36603=CARTESIAN_POINT ( 'NONE',  ( 96.32499999999998863, -207.7050326799711968, 76.53270833506762472 ) ) ;
#36606=CARTESIAN_POINT ( 'NONE',  ( 96.15314808468748708, 91.99731107132950569, 80.06489583420048461 ) ) ;
#36608=CYLINDRICAL_SURFACE ( 'NONE', #58806, 2.649999999999985700 ) ;
#36609=B_SPLINE_CURVE_WITH_KNOTS ( 'NONE', 3,
 ( #9765, #38717, #44739, #20302, #37613, #15028 ),
 .UNSPECIFIED., .F., .F.,
 ( 4, 2, 4 ),
 ( 0.7528176110416704425, 0.8153862273022827178, 0.8779548435628951042 ),
 .UNSPECIFIED. ) ;
#36621=FACE_OUTER_BOUND ( 'NONE', #54387, .T. ) ;
#36624=CARTESIAN_POINT ( 'NONE',  ( -95.00000000000002842, 86.94004357329504273, 78.09374999999998579 ) ) ;
#36626=CARTESIAN_POINT ( 'NONE',  ( -96.32499999999996021, -207.7050326799711968, 74.73354166840096013 ) ) ;
#36627=CARTESIAN_POINT ( 'NONE',  ( -96.15314808468751551, 88.00268892867056536, 88.00239583420048461 ) ) ;
#36628=CARTESIAN_POINT ( 'NONE',  ( 97.64999999999997726, 91.52997821335252127, 75.84479166840098685 ) ) ;
#36629=CARTESIAN_POINT ( 'NONE',  ( -97.65000000000001990, 90.00000000000004263, 76.74437500173429783 ) ) ;
#36631=CARTESIAN_POINT ( 'NONE',  ( 96.15314808468748708, 91.99731107132950569, 78.15989583420049769 ) ) ;
#36632=CARTESIAN_POINT ( 'NONE',  ( 97.64999999999997726, 91.52997821335253548, 82.11541666666664696 ) ) ;
#36634=DIRECTION ( 'NONE',  ( -0.000000000000000000, -0.000000000000000000, 1.000000000000000000 ) ) ;
#36652=CARTESIAN_POINT ( 'NONE',  ( -96.15314808468747287, -208.0026889286704943, 75.72572916753382799 ) ) ;
#36655=EDGE_CURVE ( 'NONE', #32728, #10456, #6813, .T. ) ;
#36665=DIRECTION ( 'NONE',  ( -0.000000000000000000, -0.000000000000000000, 1.000000000000000000 ) ) ;
#36669=CARTESIAN_POINT ( 'NONE',  ( 96.15314808468748708, 88.00268892867053694, 83.66322916753382799 ) ) ;
#36670=CARTESIAN_POINT ( 'NONE',  ( -94.99999999999997158, -212.6630814284392557, 86.78531250086713555 ) ) ;
#36674=CARTESIAN_POINT ( 'NONE',  ( -96.32499999999996021, -212.2949673200287179, 79.94583333333332575 ) ) ;
#36675=CARTESIAN_POINT ( 'NONE',  ( -95.00000000000002842, 87.33691857156074434, 75.19656250086714522 ) ) ;
#36678=CARTESIAN_POINT ( 'NONE',  ( 95.00000000000000000, -207.3369185715606307, 84.40406250086712703 ) ) ;
#36686=ORIENTED_EDGE ( 'NONE', *, *, #60291, .F. ) ;
#36687=CARTESIAN_POINT ( 'NONE',  ( -93.67500000000003979, 87.70503267997129626, 79.49604166840096298 ) ) ;
#36689=VECTOR ( 'NONE', #51199, 1000.000000000000000 ) ;
#36692=CARTESIAN_POINT ( 'NONE',  ( 92.69370383062501162, -211.3315407142195852, 79.05947916753382287 ) ) ;
#36695=( BOUNDED_CURVE ( )  B_SPLINE_CURVE ( 2, ( #30331, #29958, #24698, #70174, #52909, #13035, #35974 ),
 .UNSPECIFIED., .F., .F. ) 
 B_SPLINE_CURVE_WITH_KNOTS ( ( 3, 2, 2, 3 ),
 ( 0.6458333333333334814, 0.6527777777777779011, 0.6597222222222223209, 0.6666666666666667407 ),
 .UNSPECIFIED. ) 
 CURVE ( )  GEOMETRIC_REPRESENTATION_ITEM ( )  RATIONAL_B_SPLINE_CURVE ( ( 0.9999999999999978906, 0.8660254037844408170, 1.000000000000000000, 0.8660254037844387076, 1.000000000000000000, 0.8660254037844365982, 1.000000000000002220 ) ) 
 REPRESENTATION_ITEM ( '' )  );
#36697=DIRECTION ( 'NONE',  ( -0.000000000000000000, -0.000000000000000000, 1.000000000000000000 ) ) ;
#36699=CARTESIAN_POINT ( 'NONE',  ( 96.32499999999998863, -207.7050326799711968, 80.26333333333332121 ) ) ;
#36705=CARTESIAN_POINT ( 'NONE',  ( -97.30629616937501680, 90.00000000000004263, 82.81656250086714977 ) ) ;
#36708=CARTESIAN_POINT ( 'NONE',  ( 96.32499999999998863, 87.70503267997126784, 76.24166666666666003 ) ) ;
#36714=VERTEX_POINT ( 'NONE', #2327 ) ;
#36715=CARTESIAN_POINT ( 'NONE',  ( -92.35000000000005116, 88.47002178664754979, 87.80395833506763381 ) ) ;
#36716=( BOUNDED_CURVE ( )  B_SPLINE_CURVE ( 2, ( #73642, #51837, #16513, #11597, #56379, #40555, #56755 ),
 .UNSPECIFIED., .F., .F. ) 
 B_SPLINE_CURVE_WITH_KNOTS ( ( 3, 2, 2, 3 ),
 ( 0.7291666666666665186, 0.7361111111111109384, 0.7430555555555553582, 0.7499999999999996669 ),
 .UNSPECIFIED. ) 
 CURVE ( )  GEOMETRIC_REPRESENTATION_ITEM ( )  RATIONAL_B_SPLINE_CURVE ( ( 1.000000000000002220, 0.8660254037844365982, 1.000000000000000000, 0.8660254037844387076, 1.000000000000000000, 0.8660254037844451469, 0.9999999999999935607 ) ) 
 REPRESENTATION_ITEM ( '' )  );
#36717=CARTESIAN_POINT ( 'NONE',  ( 96.15314808468748708, 91.99731107132950569, 85.14489583420048291 ) ) ;
#36729=EDGE_CURVE ( 'NONE', #49534, #44854, #69219, .T. ) ;
#36737=CARTESIAN_POINT ( 'NONE',  ( -95.00000000000002842, 93.05995642670504253, 75.31562500173430408 ) ) ;
#36738=CARTESIAN_POINT ( 'NONE',  ( -97.30629616937497417, -208.6684592857803011, 84.66864583420047552 ) ) ;
#36739=ORIENTED_EDGE ( 'NONE', *, *, #31892, .T. ) ;
#36748=CARTESIAN_POINT ( 'NONE',  ( 93.84685191531248449, 88.00268892867053694, 80.22364583420046813 ) ) ;
#36750=CARTESIAN_POINT ( 'NONE',  ( -97.64998201403408018, 91.52998859755483352, 80.50145761676020584 ) ) ;
#36759=CARTESIAN_POINT ( 'NONE',  ( -92.69370383062505425, 88.66845928578038638, 87.36739583420047950 ) ) ;
#36766=MANIFOLD_SOLID_BREP ( 'Thread5', #64417 ) ;
#36767=CARTESIAN_POINT ( 'NONE',  ( -99.99999999999998579, -124.0000000000000142, -40.00000000000002132 ) ) ;
#36770=CARTESIAN_POINT ( 'NONE',  ( 92.69370383062501162, -209.9999999999999716, 82.18156250086715886 ) ) ;
#36772=EDGE_LOOP ( 'NONE', ( #69635, #57529, #24064, #12330 ) ) ;
#36783=CARTESIAN_POINT ( 'NONE',  ( 95.00000000000000000, -207.3369185715606307, 78.84781250086714977 ) ) ;
#36786=EDGE_LOOP ( 'NONE', ( #58001, #2223, #13209, #19965 ) ) ;
#36790=CARTESIAN_POINT ( 'NONE',  ( 95.00000000000000000, -206.9400435732949575, 80.31624999999999659 ) ) ;
#36793=CARTESIAN_POINT ( 'NONE',  ( 93.67500000000001137, -212.2949673200287179, 85.10520833506762983 ) ) ;
#36794=CARTESIAN_POINT ( 'NONE',  ( 92.34999999999999432, 90.00000000000002842, 83.65000000000000568 ) ) ;
#36799=VERTEX_POINT ( 'NONE', #19563 ) ;
#36800=CARTESIAN_POINT ( 'NONE',  ( -97.30629616937501680, 91.33154071421968467, 88.47864583420047779 ) ) ;
#36801=CARTESIAN_POINT ( 'NONE',  ( 97.30629616937498838, 91.33154071421968467, 81.12322916753382174 ) ) ;
#36803=CARTESIAN_POINT ( 'NONE',  ( 94.99999999999998579, 93.05995642670504253, 86.74562500173429669 ) ) ;
#36810=ORIENTED_EDGE ( 'NONE', *, *, #13312, .F. ) ;
#36814=CARTESIAN_POINT ( 'NONE',  ( -97.65000000000001990, 91.52997821335253548, 85.50208333333331723 ) ) ;
#36817=CARTESIAN_POINT ( 'NONE',  ( 97.06449789201045064, 91.06393496763742235, 74.79348190356853365 ) ) ;
#36821=CARTESIAN_POINT ( 'NONE',  ( -93.84685191531247028, -211.9973110713294489, 81.59947916753381492 ) ) ;
#36827=DIRECTION ( 'NONE',  ( 0.000000000000000000, 0.000000000000000000, -1.000000000000000000 ) ) ;
#36830=CARTESIAN_POINT ( 'NONE',  ( 97.64999999989935020, -209.9999769027737671, 83.41187580057901130 ) ) ;
#36838=CARTESIAN_POINT ( 'NONE',  ( -92.69370383062502583, 91.33154071421968467, 74.77322916753379900 ) ) ;
#36851=DIRECTION ( 'NONE',  ( -0.000000000000000000, -0.000000000000000000, -1.000000000000000000 ) ) ;
#36852=DIRECTION ( 'NONE',  ( -0.000000000000000000, -0.000000000000000000, 1.000000000000000000 ) ) ;
#36853=CARTESIAN_POINT ( 'NONE',  ( -92.34999999999999432, -211.5299782133524502, 86.45458333333333201 ) ) ;
#36855=CARTESIAN_POINT ( 'NONE',  ( -2.500000000000015543, -73.00000000000001421, -204.9999999999999716 ) ) ;
#36862=ORIENTED_EDGE ( 'NONE', *, *, #8500, .T. ) ;
#36867=CARTESIAN_POINT ( 'NONE',  ( 97.30629616937498838, -211.3315407142195852, 81.65239583420047609 ) ) ;
#36868=CARTESIAN_POINT ( 'NONE',  ( 92.69370383062501162, -208.6684592857803295, 88.47864583420047779 ) ) ;
#36871=CARTESIAN_POINT ( 'NONE',  ( 97.30629616937498838, -211.3315407142195852, 88.16114583420048234 ) ) ;
#36875=ORIENTED_EDGE ( 'NONE', *, *, #33594, .F. ) ;
#36876=CARTESIAN_POINT ( 'NONE',  ( -97.30629616937501680, 91.33154071421968467, 75.77864583420048916 ) ) ;
#36878=AXIS2_PLACEMENT_3D ( 'NONE', #15089, #3470, #38031 ) ;
#36882=CARTESIAN_POINT ( 'NONE',  ( 94.99999999999998579, 93.05995642670504253, 88.01562500173432113 ) ) ;
#36887=ORIENTED_EDGE ( 'NONE', *, *, #10723, .T. ) ;
#36888=CARTESIAN_POINT ( 'NONE',  ( 97.64999999999999147, -209.9999999999999716, 86.50750000000000739 ) ) ;
#36890=VERTEX_POINT ( 'NONE', #67289 ) ;
#36894=CARTESIAN_POINT ( 'NONE',  ( 95.00000000000000000, -207.3369185715606307, 77.41906250086714181 ) ) ;
#36896=CARTESIAN_POINT ( 'NONE',  ( -97.64999999950698850, -210.0000320324311076, 85.63541623677365067 ) ) ;
#36900=CARTESIAN_POINT ( 'NONE',  ( -92.35000000053402403, -209.9999467984910382, 78.96687695417375608 ) ) ;
#36908=CARTESIAN_POINT ( 'NONE',  ( -92.69370383062498320, -211.3315407142195852, 82.28739583420048120 ) ) ;
#36910=CARTESIAN_POINT ( 'NONE',  ( -97.30629616937501680, 90.00000000000004263, 78.37156250086715659 ) ) ;
#36912=CARTESIAN_POINT ( 'NONE',  ( 97.30629616937498838, 91.33154071421968467, 81.12322916753382174 ) ) ;
#36917=CARTESIAN_POINT ( 'NONE',  ( -92.34999999999999432, -209.9999999999999716, 76.98250000000000171 ) ) ;
#36920=CARTESIAN_POINT ( 'NONE',  ( -92.69370383062498320, -209.9999999999999716, 82.97531250086714749 ) ) ;
#36922=CARTESIAN_POINT ( 'NONE',  ( -97.64999999999996305, -209.9999999999999716, 89.36499999999999488 ) ) ;
#36929=CYLINDRICAL_SURFACE ( 'NONE', #58364, 2.649999999999985700 ) ;
#36930=CARTESIAN_POINT ( 'NONE',  ( -96.15314808468751551, 88.00268892867056536, 85.93864583420048575 ) ) ;
#36934=( BOUNDED_CURVE ( )  B_SPLINE_CURVE ( 2, ( #32101, #49023, #55040, #21183, #20081, #71582, #71954 ),
 .UNSPECIFIED., .F., .F. ) 
 B_SPLINE_CURVE_WITH_KNOTS ( ( 3, 2, 2, 3 ),
 ( 0.04166666666666644231, 0.04861111111111085514, 0.05555555555555525410, 0.06249999999999966693 ),
 .UNSPECIFIED. ) 
 CURVE ( )  GEOMETRIC_REPRESENTATION_ITEM ( )  RATIONAL_B_SPLINE_CURVE ( ( 1.000000000000004219, 0.8660254037844343777, 1.000000000000000000, 0.8660254037844387076, 1.000000000000000000, 0.8660254037844451469, 0.9999999999999935607 ) ) 
 REPRESENTATION_ITEM ( '' )  );
#36940=ADVANCED_FACE ( 'NONE', ( #48703 ), #58229, .F. ) ;
#36946=CARTESIAN_POINT ( 'NONE',  ( -97.64999999999996305, -209.9999999999999716, 82.37999999999999545 ) ) ;
#36948=CARTESIAN_POINT ( 'NONE',  ( -94.99999999999997158, -212.6630814284392557, 82.97531250086716170 ) ) ;
#36964=CARTESIAN_POINT ( 'NONE',  ( 96.15314808468748708, -208.0026889286704943, 88.31989583420048007 ) ) ;
#36972=VERTEX_POINT ( 'NONE', #12358 ) ;
#36976=ORIENTED_EDGE ( 'NONE', *, *, #51886, .T. ) ;
#36980=CARTESIAN_POINT ( 'NONE',  ( 94.99999999999998579, 92.66308142843935514, 79.48281250086715488 ) ) ;
#36981=FACE_BOUND ( 'NONE', #35791, .T. ) ;
#36983=CARTESIAN_POINT ( 'NONE',  ( -97.65000000000001990, 90.00000000000004263, 84.92000000000000171 ) ) ;
#36991=ORIENTED_EDGE ( 'NONE', *, *, #5650, .T. ) ;
#36996=CARTESIAN_POINT ( 'NONE',  ( -96.34407192492912486, 92.02656496471897185, 74.86703477254886252 ) ) ;
#37003=CARTESIAN_POINT ( 'NONE',  ( -94.99999999999997158, -213.0599564267049857, 77.53812500173428646 ) ) ;
#37005=CARTESIAN_POINT ( 'NONE',  ( 94.99999999999998579, 86.94004357329500010, 75.63312500173429953 ) ) ;
#37006=CARTESIAN_POINT ( 'NONE',  ( -92.35000000000005116, 91.52997821335253548, 74.57479166840096241 ) ) ;
#37008=CARTESIAN_POINT ( 'NONE',  ( 96.15314808468748708, 91.99731107132950569, 75.61989583420049144 ) ) ;
#37010=DIRECTION ( 'NONE',  ( -0.000000000000000000, -0.000000000000000000, 1.000000000000000000 ) ) ;
#37015=CARTESIAN_POINT ( 'NONE',  ( -97.64999999999996305, -209.9999999999999716, 79.83999999999998920 ) ) ;
#37016=CARTESIAN_POINT ( 'NONE',  ( 97.64999999999999147, 90.00000000000002842, 85.23749999999999716 ) ) ;
#37026=CARTESIAN_POINT ( 'NONE',  ( 92.69370383062501162, -209.9999999999999716, 89.80156250086714920 ) ) ;
#37029=CARTESIAN_POINT ( 'NONE',  ( -94.99999999999997158, -212.6630814284392557, 75.99031250086716227 ) ) ;
#37038=LINE ( 'NONE', #65998, #22524 ) ;
#37043=CARTESIAN_POINT ( 'NONE',  ( -96.32499999999996021, -212.2949673200287179, 76.13583333333333769 ) ) ;
#37046=CARTESIAN_POINT ( 'NONE',  ( 92.69370383062498320, 88.66845928578035796, 84.13947916753383538 ) ) ;
#37049=CARTESIAN_POINT ( 'NONE',  ( -94.99999999999997158, -212.6630814284392557, 86.15031250086717307 ) ) ;
#37053=CARTESIAN_POINT ( 'NONE',  ( -93.67499999999998295, -207.7050326799711968, 81.53333333333333144 ) ) ;
#37057=CARTESIAN_POINT ( 'NONE',  ( 97.30629616937498838, -211.3315407142195852, 84.19239583420046813 ) ) ;
#37060=ORIENTED_EDGE ( 'NONE', *, *, #52327, .T. ) ;
#37069=CARTESIAN_POINT ( 'NONE',  ( 96.15314808468748708, -208.0026889286704943, 78.79489583420048859 ) ) ;
#37070=CARTESIAN_POINT ( 'NONE',  ( -93.67499999999998295, -207.7050326799711968, 80.89833333333332632 ) ) ;
#37074=CARTESIAN_POINT ( 'NONE',  ( 93.67499999999999716, 87.70503267997126784, 76.77083333333332860 ) ) ;
#37076=CARTESIAN_POINT ( 'NONE',  ( 97.64999999999997726, -211.5299782133524502, 80.10458333333332348 ) ) ;
#37083=CARTESIAN_POINT ( 'NONE',  ( -93.67499999999998295, -212.2949673200287179, 86.48104166840096241 ) ) ;
#37085=CARTESIAN_POINT ( 'NONE',  ( -92.69370383062504004, 90.00000000000004263, 85.67406250086715147 ) ) ;
#37089=CARTESIAN_POINT ( 'NONE',  ( 97.64999999999999147, 90.00000000000002842, 75.07749999999998636 ) ) ;
#37094=CARTESIAN_POINT ( 'NONE',  ( -94.99999999999997158, -213.0599564267049857, 84.52312500173428589 ) ) ;
#37098=CARTESIAN_POINT ( 'NONE',  ( -97.65000000000001990, 90.00000000000004263, 85.63437500173431260 ) ) ;
#37102=CARTESIAN_POINT ( 'NONE',  ( 94.99999999999998579, 87.33691857156068750, 87.42031250086715488 ) ) ;
#37114=ORIENTED_EDGE ( 'NONE', *, *, #27410, .T. ) ;
#37121=CARTESIAN_POINT ( 'NONE',  ( -97.30629616937497417, -211.3315407142195852, 82.86947916753382515 ) ) ;
#37123=CARTESIAN_POINT ( 'NONE',  ( 92.34999999999999432, 90.00000000000002842, 90.00000000000000000 ) ) ;
#37125=AXIS2_PLACEMENT_3D ( 'NONE', #51357, #17158, #63046 ) ;
#37126=VECTOR ( 'NONE', #31679, 1000.000000000000000 ) ;
#37132=CARTESIAN_POINT ( 'NONE',  ( 97.30629616937498838, 88.66845928578037217, 89.43114583420049257 ) ) ;
#37134=CARTESIAN_POINT ( 'NONE',  ( 97.30629616937498838, 90.00000000000002842, 78.53031250086714010 ) ) ;
#37138=VECTOR ( 'NONE', #53343, 1000.000000000000000 ) ;
#37139=CARTESIAN_POINT ( 'NONE',  ( 94.68886060456908638, 92.37342585364821446, 74.84415580543370083 ) ) ;
#37142=DIRECTION ( 'NONE',  ( 1.000000000000000000, 0.000000000000000000, 0.000000000000000000 ) ) ;
#37145=CARTESIAN_POINT ( 'NONE',  ( 97.64999999999999147, 90.00000000000002842, 82.69749999999999091 ) ) ;
#37147=CARTESIAN_POINT ( 'NONE',  ( -93.84685191531252713, 88.00268892867056536, 86.04447916753380809 ) ) ;
#37151=( BOUNDED_CURVE ( )  B_SPLINE_CURVE ( 2, ( #41162, #1356, #69725, #63733, #11466, #52812, #24247, #977, #68634 ),
 .UNSPECIFIED., .F., .F. ) 
 B_SPLINE_CURVE_WITH_KNOTS ( ( 3, 2, 2, 2, 3 ),
 ( 0.9313609857438962525, 0.9313610514010480790, 0.9384168169419646599, 0.9454725824828811298, 0.9525283480368235134 ),
 .UNSPECIFIED. ) 
 CURVE ( )  GEOMETRIC_REPRESENTATION_ITEM ( )  RATIONAL_B_SPLINE_CURVE ( ( 0.9999975066324136019, 0.9999987533046057475, 1.000000000000000000, 0.8660254037844387076, 1.000000000000000000, 0.8660254037844387076, 1.000000000000000000, 0.8660254037844387076, 1.000000000000000000 ) ) 
 REPRESENTATION_ITEM ( '' )  );
#37160=CARTESIAN_POINT ( 'NONE',  ( 95.00000000000000000, -212.6630814284392557, 80.43531250086715545 ) ) ;
#37167=CARTESIAN_POINT ( 'NONE',  ( 7.103376864691351012E-17, -120.0000000000000000, -64.00000000000000000 ) ) ;
#37168=CARTESIAN_POINT ( 'NONE',  ( -94.99999999999997158, -209.9999999999999716, 90.00000000000000000 ) ) ;
#37170=CARTESIAN_POINT ( 'NONE',  ( 97.30629616937498838, -209.9999999999999716, 76.14906250086716000 ) ) ;
#37171=EDGE_CURVE ( 'NONE', #5952, #24150, #64130, .T. ) ;
#37177=CARTESIAN_POINT ( 'NONE',  ( -92.34999999999992326, 88.47002178664760663, 83.27958333333332064 ) ) ;
#37179=CIRCLE ( 'NONE', #6016, 2.649999999999985700 ) ;
#37184=CARTESIAN_POINT ( 'NONE',  ( 92.35000000000002274, -211.5299782133524502, 83.78229166840095843 ) ) ;
#37185=CARTESIAN_POINT ( 'NONE',  ( 96.32499999999998863, 87.70503267997126784, 85.13166666666666060 ) ) ;
#37191=CARTESIAN_POINT ( 'NONE',  ( -95.00000000000002842, 92.66308142843932671, 86.46781250086714010 ) ) ;
#37192=EDGE_CURVE ( 'NONE', #50665, #53082, #55096, .T. ) ;
#37193=CARTESIAN_POINT ( 'NONE',  ( 96.15314808468748708, 88.00268892867053694, 82.23447916753380582 ) ) ;
#37195=CARTESIAN_POINT ( 'NONE',  ( 93.67499999999999716, 87.70503267997126784, 83.20020833506764291 ) ) ;
#37198=CARTESIAN_POINT ( 'NONE',  ( 96.32499999999998863, -212.2949673200287179, 78.14666666666667538 ) ) ;
#37199=EDGE_LOOP ( 'NONE', ( #22569, #67496, #49998, #1470 ) ) ;
#37202=CARTESIAN_POINT ( 'NONE',  ( -93.67500000000003979, 92.29496732002878900, 85.97833333333332462 ) ) ;
#37204=CARTESIAN_POINT ( 'NONE',  ( -96.32500000000001705, 92.29496732002878900, 85.44916666666665606 ) ) ;
#37208=FACE_OUTER_BOUND ( 'NONE', #62217, .T. ) ;
#37212=CARTESIAN_POINT ( 'NONE',  ( -97.30629616937497417, -208.6684592857803011, 79.42989583420046529 ) ) ;
#37215=EDGE_CURVE ( 'NONE', #31963, #62638, #2516, .T. ) ;
#37225=CARTESIAN_POINT ( 'NONE',  ( -92.35000000000007958, -211.5299782133525071, 85.81958333333332689 ) ) ;
#37227=CARTESIAN_POINT ( 'NONE',  ( 96.32499999999998863, 87.70503267997126784, 86.48104166840096241 ) ) ;
#37228=CARTESIAN_POINT ( 'NONE',  ( -93.84685191531252713, 88.00268892867056536, 76.51947916753380241 ) ) ;
#37232=DIRECTION ( 'NONE',  ( -0.000000000000000000, -0.000000000000000000, 1.000000000000000000 ) ) ;
#37235=AXIS2_PLACEMENT_3D ( 'NONE', #37513, #72076, #60450 ) ;
#37237=LINE ( 'NONE', #61929, #51456 ) ;
#37238=AXIS2_PLACEMENT_3D ( 'NONE', #47475, #53483, #24904 ) ;
#37239=DIRECTION ( 'NONE',  ( 0.000000000000000000, 0.000000000000000000, -1.000000000000000000 ) ) ;
#37242=CARTESIAN_POINT ( 'NONE',  ( -96.32499999999996021, -207.7050326799711968, 88.62416666666665321 ) ) ;
#37249=SURFACE_SIDE_STYLE ('',( #38344 ) ) ;
#37258=CARTESIAN_POINT ( 'NONE',  ( 95.00000000000000000, -212.6630814284392557, 80.27656250086714351 ) ) ;
#37259=CARTESIAN_POINT ( 'NONE',  ( 95.00000000000000000, -212.6630814284392557, 88.69031250086716511 ) ) ;
#37261=CARTESIAN_POINT ( 'NONE',  ( 97.30629616937498838, -208.6684592857803011, 86.36197916753383197 ) ) ;
#37269=CARTESIAN_POINT ( 'NONE',  ( -97.30629616937501680, 90.00000000000004263, 77.73656250086715147 ) ) ;
#37270=ORIENTED_EDGE ( 'NONE', *, *, #21629, .F. ) ;
#37280=CARTESIAN_POINT ( 'NONE',  ( 95.00000000000000000, -209.9999999999999716, 90.00000000000000000 ) ) ;
#37287=CARTESIAN_POINT ( 'NONE',  ( 92.69370383062501162, -211.3315407142195852, 76.99572916753380980 ) ) ;
#37288=VECTOR ( 'NONE', #13517, 1000.000000000000000 ) ;
#37290=CARTESIAN_POINT ( 'NONE',  ( -97.65000000000001990, 90.00000000000004263, 81.74500000000000455 ) ) ;
#37299=CARTESIAN_POINT ( 'NONE',  ( -92.69370383062498320, -211.3315407142195852, 79.74739583420047495 ) ) ;
#37300=CARTESIAN_POINT ( 'NONE',  ( -95.00000000000002842, 92.66308142843932671, 80.11781250086714579 ) ) ;
#37304=CARTESIAN_POINT ( 'NONE',  ( 97.30629616937498838, 90.00000000000002842, 79.80031250086713612 ) ) ;
#37307=CARTESIAN_POINT ( 'NONE',  ( -92.69370383062498320, -208.6684592857803011, 89.37822916753381719 ) ) ;
#37311=CARTESIAN_POINT ( 'NONE',  ( -93.84685191531248449, -208.0026889286704943, 84.35114583420048007 ) ) ;
#37318=CARTESIAN_POINT ( 'NONE',  ( -92.35000000000003695, 90.00000000000004263, 75.07749999999998636 ) ) ;
#37320=CARTESIAN_POINT ( 'NONE',  ( -93.84685191531254134, 91.99731107132950569, 84.98614583420047097 ) ) ;
#37321=CARTESIAN_POINT ( 'NONE',  ( -97.42291288542703853, -209.3980460039468596, 74.90604073465185309 ) ) ;
#37331=CARTESIAN_POINT ( 'NONE',  ( 97.64999999999999147, -209.9999999999999716, 84.60249999999999204 ) ) ;
#37333=CARTESIAN_POINT ( 'NONE',  ( -94.99999999999997158, -207.3369185715606307, 82.65781250086715204 ) ) ;
#37336=CARTESIAN_POINT ( 'NONE',  ( 97.30629616937498838, 91.33154071421968467, 74.93197916753381094 ) ) ;
#37343=CARTESIAN_POINT ( 'NONE',  ( -95.00000000000002842, 93.05995642670504253, 78.41125000000000966 ) ) ;
#37351=CARTESIAN_POINT ( 'NONE',  ( 95.00000000000000000, -212.6630814284392557, 75.19656250086714522 ) ) ;
#37353=CARTESIAN_POINT ( 'NONE',  ( 94.99999999999998579, 86.94004357329502852, 87.06312500173429214 ) ) ;
#37356=LINE ( 'NONE', #72277, #67636 ) ;
#37364=CARTESIAN_POINT ( 'NONE',  ( 97.64999999999602665, -210.0000045800691737, 76.42687486206342840 ) ) ;
#37369=CARTESIAN_POINT ( 'NONE',  ( 92.69370383062498320, 88.66845928578037217, 79.05947916753382287 ) ) ;
#37389=CARTESIAN_POINT ( 'NONE',  ( -94.99999999999997158, -213.0599564267049857, 75.63312500173429953 ) ) ;
#37393=CARTESIAN_POINT ( 'NONE',  ( 96.32499999999998863, 87.70503267997126784, 75.68604166840097491 ) ) ;
#37394=CARTESIAN_POINT ( 'NONE',  ( -96.15314808468751551, 88.00268892867056536, 88.47864583420047779 ) ) ;
#37395=( BOUNDED_CURVE ( )  B_SPLINE_CURVE ( 2, ( #3269, #8134, #25798, #48362, #54743, #55109, #32542 ),
 .UNSPECIFIED., .F., .F. ) 
 B_SPLINE_CURVE_WITH_KNOTS ( ( 3, 2, 2, 3 ),
 ( 0.06350193517735322479, 0.07055765540882333320, 0.07761342094970606620, 0.08466915177892317401 ),
 .UNSPECIFIED. ) 
 CURVE ( )  GEOMETRIC_REPRESENTATION_ITEM ( )  RATIONAL_B_SPLINE_CURVE ( ( 0.9999982793443895623, 0.8660262641177686183, 1.000000000000000000, 0.8660254037844387076, 1.000000000000000000, 0.8660260628881687461, 0.9999986817990250687 ) ) 
 REPRESENTATION_ITEM ( '' )  );
#37396=ORIENTED_EDGE ( 'NONE', *, *, #7386, .F. ) ;
#37397=CARTESIAN_POINT ( 'NONE',  ( 94.99999999999998579, 87.33691857156068750, 75.35531250086715715 ) ) ;
#37400=CARTESIAN_POINT ( 'NONE',  ( 92.35000000000000853, -209.9999999999999716, 77.37937500173428873 ) ) ;
#37404=ORIENTED_EDGE ( 'NONE', *, *, #24556, .F. ) ;
#37420=ORIENTED_EDGE ( 'NONE', *, *, #47066, .F. ) ;
#37423=CARTESIAN_POINT ( 'NONE',  ( -97.65000000000001990, 90.00000000000004263, 79.20499999999999829 ) ) ;
#37426=CARTESIAN_POINT ( 'NONE',  ( 96.32499999999998863, -207.7050326799711968, 80.34270833506762699 ) ) ;
#37430=CARTESIAN_POINT ( 'NONE',  ( 94.99999999999998579, 92.66308142843932671, 83.92781250086716227 ) ) ;
#37431=CARTESIAN_POINT ( 'NONE',  ( -96.15314808468745866, -211.9973110713294489, 81.65239583420049030 ) ) ;
#37437=CARTESIAN_POINT ( 'NONE',  ( -93.67499999999998295, -207.7050326799711968, 78.35833333333333428 ) ) ;
#37443=CARTESIAN_POINT ( 'NONE',  ( 97.30629616937498838, -211.3315407142195852, 83.55739583420047722 ) ) ;
#37455=CARTESIAN_POINT ( 'NONE',  ( 92.69370383062501162, -208.6684592857803295, 77.68364583420047609 ) ) ;
#37460=FACE_OUTER_BOUND ( 'NONE', #36772, .T. ) ;
#37461=CARTESIAN_POINT ( 'NONE',  ( 97.64999999999997726, -208.4700217866474645, 81.48041666666665606 ) ) ;
#37469=CARTESIAN_POINT ( 'NONE',  ( -93.84685191531254134, 91.99731107132950569, 83.23989583420049598 ) ) ;
#37472=CARTESIAN_POINT ( 'NONE',  ( 97.64999999999997726, 91.52997821335252127, 75.76541666666666686 ) ) ;
#37475=CARTESIAN_POINT ( 'NONE',  ( -92.34999999999999432, -209.9999999999999716, 87.22187500173430408 ) ) ;
#37479=CARTESIAN_POINT ( 'NONE',  ( -93.67500000000003979, 92.29496732002878900, 82.88270833506763324 ) ) ;
#37481=CARTESIAN_POINT ( 'NONE',  ( 94.99999999999998579, 92.66308142843935514, 85.19781250086714408 ) ) ;
#37483=CARTESIAN_POINT ( 'NONE',  ( -96.32500000000001705, 87.70503267997129626, 85.74020833506763495 ) ) ;
#37489=CARTESIAN_POINT ( 'NONE',  ( 2.499999999999979572, 80.00000000000000000, -280.0000000000000000 ) ) ;
#37490=ORIENTED_EDGE ( 'NONE', *, *, #73825, .T. ) ;
#37493=CARTESIAN_POINT ( 'NONE',  ( 92.34999999999999432, 90.00001683226676619, 78.64937441956428188 ) ) ;
#37498=CARTESIAN_POINT ( 'NONE',  ( -92.69370383062498320, -209.9999999999999716, 85.67406250086715147 ) ) ;
#37506=CARTESIAN_POINT ( 'NONE',  ( 97.30629616937498838, 88.66845928578035796, 76.57239583420046358 ) ) ;
#37512=CARTESIAN_POINT ( 'NONE',  ( 97.65000000000000568, -211.5299782133524502, 84.54958333333334508 ) ) ;
#37513=CARTESIAN_POINT ( 'NONE',  ( -94.99999999999997158, -209.9999999999999716, 75.00000000000000000 ) ) ;
#37515=ORIENTED_EDGE ( 'NONE', *, *, #34296, .T. ) ;
#37517=CARTESIAN_POINT ( 'NONE',  ( -95.00000000000002842, 92.66308142843932671, 81.86406250086713499 ) ) ;
#37522=ORIENTED_EDGE ( 'NONE', *, *, #17143, .F. ) ;
#37526=FACE_OUTER_BOUND ( 'NONE', #31281, .T. ) ;
#37530=CARTESIAN_POINT ( 'NONE',  ( 97.30629616937498838, -209.9999999999999716, 79.32406250086715715 ) ) ;
#37533=ORIENTED_EDGE ( 'NONE', *, *, #26636, .T. ) ;
#37540=FACE_OUTER_BOUND ( 'NONE', #3281, .T. ) ;
#37542=CARTESIAN_POINT ( 'NONE',  ( 92.35000000000000853, -209.9999999999999716, 90.00000000000000000 ) ) ;
#37543=CARTESIAN_POINT ( 'NONE',  ( 96.66079198124938898, -211.6002412367799934, 74.80065669543249385 ) ) ;
#37545=DIRECTION ( 'NONE',  ( -0.000000000000000000, -0.000000000000000000, 1.000000000000000000 ) ) ;
#37549=CARTESIAN_POINT ( 'NONE',  ( -93.67499999999998295, -207.7050326799711968, 82.24770833506762813 ) ) ;
#37556=CARTESIAN_POINT ( 'NONE',  ( 92.35000000000002274, -208.4700217866474645, 79.23145833506762870 ) ) ;
#37557=CARTESIAN_POINT ( 'NONE',  ( 93.67499999999998295, 92.29496732002878900, 83.54416666666666913 ) ) ;
#37563=CARTESIAN_POINT ( 'NONE',  ( -92.69370383062505425, 91.33154071421968467, 89.53697916753382913 ) ) ;
#37564=CARTESIAN_POINT ( 'NONE',  ( 96.15314808468748708, 91.99731107132950569, 80.54114583420046358 ) ) ;
#37565=ORIENTED_EDGE ( 'NONE', *, *, #25450, .F. ) ;
#37566=CARTESIAN_POINT ( 'NONE',  ( 94.99999999999998579, 93.05995642670504253, 81.66562500173431260 ) ) ;
#37573=CARTESIAN_POINT ( 'NONE',  ( 92.34999999999999432, 89.99998767024830215, 75.47437542817786493 ) ) ;
#37574=CARTESIAN_POINT ( 'NONE',  ( -96.32500000000001705, 87.70503267997129626, 85.02583333333332405 ) ) ;
#37575=ORIENTED_EDGE ( 'NONE', *, *, #15261, .F. ) ;
#37580=CARTESIAN_POINT ( 'NONE',  ( -93.84685191531248449, -208.0026889286704943, 79.27114583420046756 ) ) ;
#37588=VECTOR ( 'NONE', #64622, 1000.000000000000000 ) ;
#37590=CARTESIAN_POINT ( 'NONE',  ( 93.84685191531248449, 91.99731107132950569, 86.99697916753380866 ) ) ;
#37600=( BOUNDED_CURVE ( )  B_SPLINE_CURVE ( 2, ( #38780, #61716, #10199, #16586, #27487, #33491, #10567 ),
 .UNSPECIFIED., .F., .F. ) 
 B_SPLINE_CURVE_WITH_KNOTS ( ( 3, 2, 2, 3 ),
 ( 0.6875000000000000000, 0.6944444444444443088, 0.7013888888888887285, 0.7083333333333331483 ),
 .UNSPECIFIED. ) 
 CURVE ( )  GEOMETRIC_REPRESENTATION_ITEM ( )  RATIONAL_B_SPLINE_CURVE ( ( 1.000000000000000000, 0.8660254037844387076, 1.000000000000000000, 0.8660254037844387076, 1.000000000000000000, 0.8660254037844430375, 0.9999999999999956701 ) ) 
 REPRESENTATION_ITEM ( '' )  );
#37608=CIRCLE ( 'NONE', #5203, 3.299999999999969624 ) ;
#37612=CARTESIAN_POINT ( 'NONE',  ( -97.64999999999994884, -211.5299782133524502, 88.14791666666666003 ) ) ;
#37613=CARTESIAN_POINT ( 'NONE',  ( -93.33265519076742578, 87.91120745868269637, 75.00000000000000000 ) ) ;
#37620=VERTEX_POINT ( 'NONE', #51941 ) ;
#37623=EDGE_CURVE ( 'NONE', #54593, #69330, #63243, .T. ) ;
#37627=CARTESIAN_POINT ( 'NONE',  ( 92.69370383062501162, -208.6684592857803295, 80.06489583420047040 ) ) ;
#37628=CARTESIAN_POINT ( 'NONE',  ( 92.69370383062501162, -208.6684592857803295, 86.57364583420047666 ) ) ;
#37629=VERTEX_POINT ( 'NONE', #68128 ) ;
#37630=CARTESIAN_POINT ( 'NONE',  ( 95.00000000000000000, -207.3369185715606307, 85.19781250086714408 ) ) ;
#37634=CARTESIAN_POINT ( 'NONE',  ( -96.15314808468751551, 88.00268892867056536, 78.47739583420049314 ) ) ;
#37646=DIRECTION ( 'NONE',  ( 1.000000000000000000, 0.000000000000000000, 0.000000000000000000 ) ) ;
#37652=CARTESIAN_POINT ( 'NONE',  ( 96.15314808468748708, -208.0026889286704943, 79.90614583420047268 ) ) ;
#37660=CARTESIAN_POINT ( 'NONE',  ( -93.67500000000003979, 87.70503267997129626, 80.68666666666665321 ) ) ;
#37662=DIRECTION ( 'NONE',  ( 1.000000000000000000, 0.000000000000000000, 0.000000000000000000 ) ) ;
#37664=CARTESIAN_POINT ( 'NONE',  ( -92.69370383062502583, 91.33154071421968467, 78.74197916753382742 ) ) ;
#37667=CARTESIAN_POINT ( 'NONE',  ( 92.69370383062498320, 91.33154071421968467, 76.25489583420049655 ) ) ;
#37671=CARTESIAN_POINT ( 'NONE',  ( 97.65000000000000568, 88.47002178664752137, 77.64395833506762301 ) ) ;
#37672=CARTESIAN_POINT ( 'NONE',  ( 92.35000000039376289, -209.9999706925934504, 76.74344264317686282 ) ) ;
#37674=CARTESIAN_POINT ( 'NONE',  ( -92.69370383062498320, -211.3315407142195852, 83.55739583420047722 ) ) ;
#37675=VECTOR ( 'NONE', #58735, 1000.000000000000000 ) ;
#37679=EDGE_LOOP ( 'NONE', ( #30046, #72119, #53078, #47672 ) ) ;
#37680=ORIENTED_EDGE ( 'NONE', *, *, #63437, .F. ) ;
#37684=EDGE_CURVE ( 'NONE', #20714, #54372, #4627, .T. ) ;
#37686=CARTESIAN_POINT ( 'NONE',  ( -97.30629616937501680, 91.33154071421968467, 85.77989583420048803 ) ) ;
#37687=CARTESIAN_POINT ( 'NONE',  ( -96.90895014231831794, -208.4386293813703901, 74.88237134757153513 ) ) ;
#37695=CARTESIAN_POINT ( 'NONE',  ( 97.64999999999999147, 89.99999998014077107, 85.95187500101400246 ) ) ;
#37700=CARTESIAN_POINT ( 'NONE',  ( 93.67500000000001137, -212.2949673200287179, 82.48583333333333201 ) ) ;
#37701=CARTESIAN_POINT ( 'NONE',  ( -97.30629616937497417, -208.6684592857803011, 81.49364583420047836 ) ) ;
#37706=ADVANCED_FACE ( 'NONE', ( #10234 ), #62511, .F. ) ;
#37718=EDGE_CURVE ( 'NONE', #13389, #40893, #5367, .T. ) ;
#37731=LINE ( 'NONE', #20048, #34738 ) ;
#37735=CARTESIAN_POINT ( 'NONE',  ( 96.15314808468748708, 88.00268892867053694, 75.40822916753381833 ) ) ;
#37739=VERTEX_POINT ( 'NONE', #5735 ) ;
#37740=ORIENTED_EDGE ( 'NONE', *, *, #134, .T. ) ;
#37741=CARTESIAN_POINT ( 'NONE',  ( 94.99999999999998579, 92.66308142843935514, 88.84906250086713442 ) ) ;
#37743=CARTESIAN_POINT ( 'NONE',  ( 92.69370383062501162, -209.9999999999999716, 89.64281250086713726 ) ) ;
#37751=CARTESIAN_POINT ( 'NONE',  ( -93.67499999999998295, -207.7050326799711968, 77.16770833506762983 ) ) ;
#37752=CARTESIAN_POINT ( 'NONE',  ( -93.84685191531252713, 88.00268892867056536, 88.10822916753382117 ) ) ;
#37756=CARTESIAN_POINT ( 'NONE',  ( 92.69370383062498320, 90.00000000000002842, 86.46781250086714010 ) ) ;
#37757=CARTESIAN_POINT ( 'NONE',  ( -95.00000000000002842, 92.66308142843932671, 88.84906250086713442 ) ) ;
#37759=CARTESIAN_POINT ( 'NONE',  ( 92.69370383062498320, 88.66845928578037217, 76.51947916753381662 ) ) ;
#37761=CARTESIAN_POINT ( 'NONE',  ( 92.35000000000000853, -211.5299782133524218, 87.51291666666666913 ) ) ;
#37774=CARTESIAN_POINT ( 'NONE',  ( -92.35000000000005116, 91.52997821335253548, 80.84541666666666515 ) ) ;
#37780=CARTESIAN_POINT ( 'NONE',  ( -92.35000000000400178, 89.99999541993113894, 76.42687486206344261 ) ) ;
#37784=CARTESIAN_POINT ( 'NONE',  ( -95.00000000000002842, 92.66308142843932671, 81.22906250086715829 ) ) ;
#37788=CARTESIAN_POINT ( 'NONE',  ( -92.35000000000006537, 90.00000034979574082, 77.69687501385438111 ) ) ;
#37790=DIRECTION ( 'NONE',  ( 1.000000000000000000, 0.000000000000000000, 0.000000000000000000 ) ) ;
#37796=CARTESIAN_POINT ( 'NONE',  ( 94.99999999999998579, 87.33691857156068750, 79.16531250086715943 ) ) ;
#37797=EDGE_CURVE ( 'NONE', #57437, #13520, #70698, .T. ) ;
#37798=CARTESIAN_POINT ( 'NONE',  ( -97.30629616937497417, -211.3315407142195852, 82.86947916753379673 ) ) ;
#37802=CARTESIAN_POINT ( 'NONE',  ( -94.99999999999997158, -213.0599564267049857, 76.82374999999998977 ) ) ;
#37806=CARTESIAN_POINT ( 'NONE',  ( 95.00000000000000000, -212.6630814284392557, 82.81656250086713555 ) ) ;
#37818=CARTESIAN_POINT ( 'NONE',  ( 97.30629616937498838, -208.6684592857803295, 79.37697916753381833 ) ) ;
#37821=CARTESIAN_POINT ( 'NONE',  ( -97.40333747838809586, 89.15460556225126254, 74.93511027845775629 ) ) ;
#37822=( BOUNDED_CURVE ( )  B_SPLINE_CURVE ( 2, ( #2708, #1965, #59081, #14312, #47782, #71441, #25589, #13201, #13565, #54536, #70702, #42897, #7569, #3065, #19210, #35751, #18831, #70327, #65463, #36495, #42160, #37259, #7199, #65093, #59445, #36868, #7931, #19941, #30845, #60198, #71071, #65825, #53793, #36131, #53066, #30484, #1601, #18468, #8682, #41410, #64351, #19572, #2342, #31593, #47421, #12823, #48161, #24487, #58702, #42521, #13928, #30117, #41773, #64718, #59818, #8306, #26334, #61664, #5558, #15047, #15413, #37628, #55645, #33073, #26692, #17191, #54903, #21415, #57051, #10149, #45784, #44375, #57415, #28458, #60917, #51390, #74329, #22843, #9786, #67302, #15800, #28836, #68706, #49993, #40123, #43281, #38735, #21054, #63078, #44005, #66204, #61297, #11535, #72186, #14679, #9407, #32333, #34471, #38361, #32699, #60563, #49619, #55277, #72548, #37986, #5927, #9041, #72911, #20693, #31962, #71810, #3426, #27060, #20323, #49260, #43644, #66567, #3797, #66918, #4163, #18654, #52883, #63807, #1425, #70514, #40871, #29190, #12277, #41594, #69792, #51772, #17924, #40487, #23942, #47241, #24673, #58149, #41228, #17554, #19026, #36320, #35213, #58514, #52134, #53251, #1790, #64910, #6647, #24313, #64534, #679, #35578, #13391, #7758, #70150, #7008, #7394, #13014, #29556, #59260, #47604, #316, #23565, #35948, #52494, #46498, #69425, #41977, #58899, #46878, #30305, #23209, #63436, #1051, #46138, #69068, #11907, #34850, #12646, #57788, #18291, #29932, #64172, #6292, #19398, #59633, #66393, #60748, #42345, #70897, #42710, #14118, #53999, #65282, #25782, #30671, #38174, #37818, #48343, #13753, #15238, #66023, #54727, #36692, #53612, #8117, #14496, #60018, #37069, #66752, #8502, #20517, #14872, #2538, #31420, #54362, #2887, #31045, #25423, #9225, #61118, #71256, #55091, #19763, #3253, #48713, #25044, #32148, #65645, #37455, #71632, #20132, #43095, #43475, #60383, #8866, #2157, #47983, #72377, #3621, #26520, #49453, #20878, #31779, #26141, #49082, #43834, #72007, #50181, #5472, #67493, #62615, #22372, #4353, #4734, #45694, #38923, #34013, #73115, #68618, #10344, #67117, #40036, #68242, #9606, #17106, #44943, #38552, #21619, #62232, #49815, #67866, #45316, #61859, #28372, #15620, #33645, #16738, #73862, #56964, #56598, #15981, #39674, #11092, #32526, #5101, #16357 ),
 .UNSPECIFIED., .F., .F. ) 
 B_SPLINE_CURVE_WITH_KNOTS ( ( 3, 2, 2, 2, 2, 2, 2, 2, 2, 2, 2, 2, 2, 2, 2, 2, 2, 2, 2, 2, 2, 2, 2, 2, 2, 2, 2, 2, 2, 2, 2, 2, 2, 2, 2, 2, 2, 2, 2, 2, 2, 2, 2, 2, 2, 2, 2, 2, 2, 2, 2, 2, 2, 2, 2, 2, 2, 2, 2, 2, 2, 2, 2, 2, 2, 2, 2, 2, 2, 2, 2, 2, 2, 2, 2, 2, 2, 2, 2, 2, 2, 2, 2, 2, 2, 2, 2, 2, 2, 2, 2, 2, 2, 2, 2, 2, 2, 2, 2, 2, 2, 2, 2, 2, 2, 2, 2, 2, 2, 2, 2, 2, 2, 2, 2, 2, 2, 2, 2, 2, 2, 2, 2, 2, 2, 2, 2, 2, 2, 2, 2, 2, 2, 2, 2, 2, 2, 2, 2, 2, 2, 2, 2, 3 ),
 ( 0.000000000000000000, 0.007055764916269565389, 0.01411152983253913078, 0.02116729474880869530, 0.02822305966507826155, 0.03527882458134783128, 0.04233458949761739060, 0.04939035441388696379, 0.05644611933015652311, 0.06350188424642609630, 0.07055764916269566256, 0.07761341407896522882, 0.08466917899523478119, 0.09172494391150436133, 0.09878070882777392758, 0.1058364737440434938, 0.1128922386603130462, 0.1199480035765826125, 0.1270037684928521926, 0.1340595334091217450, 0.1411152983253913251, 0.1481710632416609053, 0.1552268281579304576, 0.1622825930742000100, 0.1693383579904695624, 0.1763941229067391425, 0.1834498878230087227, 0.1905056527392782750, 0.1975614176555478552, 0.2046171825718174075, 0.2116729474880869877, 0.2187287124043565678, 0.2257844773206260924, 0.2328402422368956726, 0.2398960071531652249, 0.2469517720694348051, 0.2540075369857043852, 0.2610633019019739098, 0.2681190668182434900, 0.2751748317345130701, 0.2822305966507826502, 0.2892863615670521749, 0.2963421264833218105, 0.3033978913995913351, 0.3104536563158609153, 0.3175094212321304399, 0.3245651861484000200, 0.3316209510646696002, 0.3386767159809391248, 0.3457324808972087604, 0.3527882458134782850, 0.3598440107297478652, 0.3668997756460174453, 0.3739555405622870254, 0.3810113054785565501, 0.3880670703948260747, 0.3951228353110957103, 0.4021786002273652350, 0.4092343651436348151, 0.4162901300599043952, 0.4233458949761739754, 0.4304016598924435000, 0.4374574248087131356, 0.4445131897249826602, 0.4515689546412521849, 0.4586247195575217650, 0.4656804844737913451, 0.4727362493900609253, 0.4797920143063304499, 0.4868477792226000855, 0.4939035441388696102, 0.5009593090551391903, 0.5080150739714087704, 0.5150708388876782395, 0.5221266038039478197, 0.5291823687202175108, 0.5362381336364869799, 0.5432938985527565601, 0.5503496634690261402, 0.5574054283852957203, 0.5644611933015653005, 0.5715169582178348806, 0.5785727231341043497, 0.5856284880503739299, 0.5926842529666436210, 0.5997400178829130901, 0.6067957827991826703, 0.6138515477154522504, 0.6209073126317218305, 0.6279630775479914107, 0.6350188424642608798, 0.6420746073805304599, 0.6491303722968000400, 0.6561861372130696202, 0.6632419021293392003, 0.6702976670456087804, 0.6773534319618782495, 0.6844091968781479407, 0.6914649617944175208, 0.6985207267106869899, 0.7055764916269565701, 0.7126322565432261502, 0.7196880214594957303, 0.7267437863757653105, 0.7337995512920348906, 0.7408553162083043597, 0.7479110811245740509, 0.7549668460408436310, 0.7620226109571131001, 0.7690783758733826803, 0.7761341407896521494, 0.7831899057059218405, 0.7902456706221914207, 0.7973014355384608898, 0.8043572004547304699, 0.8114129653710001611, 0.8184687302872696302, 0.8255244952035392103, 0.8325802601198087904, 0.8396360250360782596, 0.8466917899523479507, 0.8537475548686175308, 0.8608033197848870000, 0.8678590847011565801, 0.8749148496174262712, 0.8819706145336957404, 0.8890263794499653205, 0.8960821443662349006, 0.9031379092825043697, 0.9101936741987740609, 0.9172494391150435300, 0.9243052040313131101, 0.9313609689475826903, 0.9384167338638522704, 0.9454724987801218505, 0.9525282636963914307, 0.9595840286126608998, 0.9666397935289304799, 0.9736955584452001711, 0.9807513233614696402, 0.9878070882777392203, 0.9948628531940088005, 0.9999999123559569769, 1.000000000000000000 ),
 .UNSPECIFIED. ) 
 CURVE ( )  GEOMETRIC_REPRESENTATION_ITEM ( )  RATIONAL_B_SPLINE_CURVE ( ( 1.000000000000000000, 0.8660254037844387076, 1.000000000000000000, 0.8660254037844387076, 1.000000000000000000, 0.8660254037844387076, 1.000000000000000000, 0.8660254037844387076, 1.000000000000000000, 0.8660254037844387076, 1.000000000000000000, 0.8660254037844387076, 1.000000000000000000, 0.8660254037844387076, 1.000000000000000000, 0.8660254037844387076, 1.000000000000000000, 0.8660254037844387076, 1.000000000000000000, 0.8660254037844387076, 1.000000000000000000, 0.8660254037844387076, 1.000000000000000000, 0.8660254037844387076, 1.000000000000000000, 0.8660254037844387076, 1.000000000000000000, 0.8660254037844387076, 1.000000000000000000, 0.8660254037844387076, 1.000000000000000000, 0.8660254037844387076, 1.000000000000000000, 0.8660254037844387076, 1.000000000000000000, 0.8660254037844387076, 1.000000000000000000, 0.8660254037844387076, 1.000000000000000000, 0.8660254037844387076, 1.000000000000000000, 0.8660254037844387076, 1.000000000000000000, 0.8660254037844387076, 1.000000000000000000, 0.8660254037844387076, 1.000000000000000000, 0.8660254037844387076, 1.000000000000000000, 0.8660254037844387076, 1.000000000000000000, 0.8660254037844387076, 1.000000000000000000, 0.8660254037844387076, 1.000000000000000000, 0.8660254037844387076, 1.000000000000000000, 0.8660254037844387076, 1.000000000000000000, 0.8660254037844387076, 1.000000000000000000, 0.8660254037844387076, 1.000000000000000000, 0.8660254037844387076, 1.000000000000000000, 0.8660254037844387076, 1.000000000000000000, 0.8660254037844387076, 1.000000000000000000, 0.8660254037844387076, 1.000000000000000000, 0.8660254037844387076, 1.000000000000000000, 0.8660254037844387076, 1.000000000000000000, 0.8660254037844387076, 1.000000000000000000, 0.8660254037844387076, 1.000000000000000000, 0.8660254037844387076, 1.000000000000000000, 0.8660254037844387076, 1.000000000000000000, 0.8660254037844387076, 1.000000000000000000, 0.8660254037844387076, 1.000000000000000000, 0.8660254037844387076, 1.000000000000000000, 0.8660254037844387076, 1.000000000000000000, 0.8660254037844387076, 1.000000000000000000, 0.8660254037844387076, 1.000000000000000000, 0.8660254037844387076, 1.000000000000000000, 0.8660254037844387076, 1.000000000000000000, 0.8660254037844387076, 1.000000000000000000, 0.8660254037844387076, 1.000000000000000000, 0.8660254037844387076, 1.000000000000000000, 0.8660254037844387076, 1.000000000000000000, 0.8660254037844387076, 1.000000000000000000, 0.8660254037844387076, 1.000000000000000000, 0.8660254037844387076, 1.000000000000000000, 0.8660254037844387076, 1.000000000000000000, 0.8660254037844387076, 1.000000000000000000, 0.8660254037844387076, 1.000000000000000000, 0.8660254037844387076, 1.000000000000000000, 0.8660254037844387076, 1.000000000000000000, 0.8660254037844387076, 1.000000000000000000, 0.8660254037844387076, 1.000000000000000000, 0.8660254037844387076, 1.000000000000000000, 0.8660254037844387076, 1.000000000000000000, 0.8660254037844387076, 1.000000000000000000, 0.8660254037844387076, 1.000000000000000000, 0.8660254037844387076, 1.000000000000000000, 0.8660254037844387076, 1.000000000000000000, 0.8660254037844387076, 1.000000000000000000, 0.8660254037844387076, 1.000000000000000000, 0.8660254037844387076, 1.000000000000000000, 0.8660254037844387076, 1.000000000000000000, 0.8660254037844387076, 1.000000000000000000, 0.8660254037844387076, 1.000000000000000000, 0.8660254037844387076, 1.000000000000000000, 0.8660254037844387076, 1.000000000000000000, 0.8660254037844387076, 1.000000000000000000, 0.8660254037844387076, 1.000000000000000000, 0.8660254037844387076, 1.000000000000000000, 0.8660254037844387076, 1.000000000000000000, 0.8660254037844387076, 1.000000000000000000, 0.8660254037844387076, 1.000000000000000000, 0.8660254037844387076, 1.000000000000000000, 0.8660254037844387076, 1.000000000000000000, 0.8660254037844387076, 1.000000000000000000, 0.8660254037844387076, 1.000000000000000000, 0.8660254037844387076, 1.000000000000000000, 0.8660254037844387076, 1.000000000000000000, 0.8660254037844387076, 1.000000000000000000, 0.8660254037844387076, 1.000000000000000000, 0.8660254037844387076, 1.000000000000000000, 0.8660254037844387076, 1.000000000000000000, 0.8660254037844387076, 1.000000000000000000, 0.8660254037844387076, 1.000000000000000000, 0.8660254037844387076, 1.000000000000000000, 0.8660254037844387076, 1.000000000000000000, 0.8660254037844387076, 1.000000000000000000, 0.8660254037844387076, 1.000000000000000000, 0.8660254037844387076, 1.000000000000000000, 0.8660254037844387076, 1.000000000000000000, 0.8660254037844387076, 1.000000000000000000, 0.8660254037844387076, 1.000000000000000000, 0.8660254037844387076, 1.000000000000000000, 0.8660254037844387076, 1.000000000000000000, 0.8660254037844387076, 1.000000000000000000, 0.8660254037844387076, 1.000000000000000000, 0.8660254037844387076, 1.000000000000000000, 0.8660254037844387076, 1.000000000000000000, 0.8660254037844387076, 1.000000000000000000, 0.8660254037844387076, 1.000000000000000000, 0.8660254037844387076, 1.000000000000000000, 0.8660254037844387076, 1.000000000000000000, 0.8660254037844387076, 1.000000000000000000, 0.8660254037844387076, 1.000000000000000000, 0.8660254037844387076, 1.000000000000000000, 0.8660254037844387076, 1.000000000000000000, 0.8660254037844387076, 1.000000000000000000, 0.8660254037844387076, 1.000000000000000000, 0.8660254037844387076, 1.000000000000000000, 0.8660254037844387076, 1.000000000000000000, 0.8660254037844387076, 1.000000000000000000, 0.8660254037844387076, 1.000000000000000000, 0.8660254037844387076, 1.000000000000000000, 0.8660254037844387076, 1.000000000000000000, 0.8660254037844387076, 1.000000000000000000, 0.8660254037844387076, 1.000000000000000000, 0.8660254037844387076, 1.000000000000000000, 0.8660254037844387076, 1.000000000000000000, 0.8660254037844387076, 1.000000000000000000, 0.8660254037844387076, 1.000000000000000000, 0.8660254037844387076, 1.000000000000000000, 0.8660254037844387076, 1.000000000000000000, 0.8660254037844387076, 1.000000000000000000, 0.8660254037844387076, 1.000000000000000000, 0.8660254037844387076, 1.000000000000000000, 0.8660254037844387076, 1.000000000000000000, 0.8660254037844387076, 1.000000000000000000, 0.8660254037844387076, 1.000000000000000000, 0.8660254037844387076, 1.000000000000000000, 0.8660254037844387076, 1.000000000000000000, 0.9024577157650929271, 0.9469497795711361299, 0.9469497795711361299, 0.9469497795711361299 ) ) 
 REPRESENTATION_ITEM ( '' )  );
#37823=CARTESIAN_POINT ( 'NONE',  ( 93.84685191531248449, 91.99731107132950569, 88.42572916753381662 ) ) ;
#37824=CARTESIAN_POINT ( 'NONE',  ( 97.64999999999999147, -209.9999999999999716, 90.00000000000000000 ) ) ;
#37825=CARTESIAN_POINT ( 'NONE',  ( 95.00000000000000000, -206.9400435732949575, 81.58624999999999261 ) ) ;
#37832=CARTESIAN_POINT ( 'NONE',  ( -97.30629616937501680, 88.66845928578038638, 85.40947916753380298 ) ) ;
#37834=CYLINDRICAL_SURFACE ( 'NONE', #33828, 2.649999999999985700 ) ;
#37836=CARTESIAN_POINT ( 'NONE',  ( 94.99999999999998579, 90.00000000000002842, 90.00000000000000000 ) ) ;
#37839=CARTESIAN_POINT ( 'NONE',  ( -92.34999999999999432, -208.4700217866474645, 87.27479166840096525 ) ) ;
#37843=CARTESIAN_POINT ( 'NONE',  ( -92.35000000000005116, 88.47002178664754979, 82.08895833506764461 ) ) ;
#37845=CARTESIAN_POINT ( 'NONE',  ( 97.30629616937498838, 88.66845928578037217, 86.25614583420048120 ) ) ;
#37849=CARTESIAN_POINT ( 'NONE',  ( -92.69370383062504004, 89.70433482669615444, 74.79348190356851944 ) ) ;
#37853=EDGE_LOOP ( 'NONE', ( #40921, #44573, #41486, #69960 ) ) ;
#37854=CARTESIAN_POINT ( 'NONE',  ( -96.32500000000001705, 92.29496732002878900, 81.08354166840096866 ) ) ;
#37859=CARTESIAN_POINT ( 'NONE',  ( -0.0004442498525516064278, 0.001194404164626844313, -80.00000000000000000 ) ) ;
#37860=ADVANCED_FACE ( 'NONE', ( #3062 ), #71437, .T. ) ;
#37864=CARTESIAN_POINT ( 'NONE',  ( -96.15314808468747287, -208.0026889286704943, 83.34572916753383254 ) ) ;
#37865=VERTEX_POINT ( 'NONE', #42517 ) ;
#37866=CARTESIAN_POINT ( 'NONE',  ( 95.00000000000000000, -209.9999999999999716, 90.00000000000000000 ) ) ;
#37868=EDGE_LOOP ( 'NONE', ( #71283, #61240, #26266, #41591 ) ) ;
#37871=CARTESIAN_POINT ( 'NONE',  ( -96.32499999999996021, -212.2949673200287179, 76.21520833506762926 ) ) ;
#37872=CARTESIAN_POINT ( 'NONE',  ( 96.15314808468748708, 88.00268892867053694, 77.15447916753380753 ) ) ;
#37880=CARTESIAN_POINT ( 'NONE',  ( 92.35000000030107969, -209.9999754409356854, 87.53856274002261273 ) ) ;
#37884=CARTESIAN_POINT ( 'NONE',  ( -95.00000000000002842, 86.94004357329504273, 78.17312500173430578 ) ) ;
#37886=CARTESIAN_POINT ( 'NONE',  ( -96.15314808468751551, 88.00268892867056536, 82.12864583420046927 ) ) ;
#37895=CARTESIAN_POINT ( 'NONE',  ( 92.35000000000000853, -209.9999999999999716, 90.00000000000000000 ) ) ;
#37898=CARTESIAN_POINT ( 'NONE',  ( 93.84685191531249870, -208.0026889286704943, 78.26572916753382003 ) ) ;
#37903=CARTESIAN_POINT ( 'NONE',  ( 99.99999999999998579, 95.00000000000002842, -90.00000000000000000 ) ) ;
#37906=CARTESIAN_POINT ( 'NONE',  ( 94.26574316504959938, -214.0859151322040645, 74.64692065633562379 ) ) ;
#37912=CARTESIAN_POINT ( 'NONE',  ( -96.32500000000001705, 87.70503267997129626, 83.12083333333332291 ) ) ;
#37916=ORIENTED_EDGE ( 'NONE', *, *, #54399, .T. ) ;
#37918=CARTESIAN_POINT ( 'NONE',  ( 92.35000000000002274, -208.4700217866474645, 80.50145833506765314 ) ) ;
#37919=CARTESIAN_POINT ( 'NONE',  ( 92.34999999999999432, 88.47002178664753558, 86.24291666666665890 ) ) ;
#37927=CARTESIAN_POINT ( 'NONE',  ( -97.30629616937501680, 88.66845928578038638, 84.77447916753381207 ) ) ;
#37928=CARTESIAN_POINT ( 'NONE',  ( 96.15314808468748708, 91.99731107132950569, 83.08114583420048405 ) ) ;
#37943=CARTESIAN_POINT ( 'NONE',  ( -94.99999999999997158, -212.6630814284392557, 79.64156250086713840 ) ) ;
#37946=CARTESIAN_POINT ( 'NONE',  ( -97.64999999999993463, 88.47002178664749295, 86.24291666666667311 ) ) ;
#37952=CARTESIAN_POINT ( 'NONE',  ( 96.15314808468748708, 91.99731107132950569, 88.79614583420047325 ) ) ;
#37954=CARTESIAN_POINT ( 'NONE',  ( 92.34999999999999432, 90.00000000000002842, 81.18937500173430521 ) ) ;
#37968=CARTESIAN_POINT ( 'NONE',  ( -96.32499999999996021, -212.2949673200287179, 89.47083333333333144 ) ) ;
#37984=ORIENTED_EDGE ( 'NONE', *, *, #28697, .F. ) ;
#37985=CARTESIAN_POINT ( 'NONE',  ( 97.30629616937498838, -209.9999999999999716, 82.97531250086714749 ) ) ;
#37986=CARTESIAN_POINT ( 'NONE',  ( 96.15314808468750130, -211.9973110713294489, 84.29822916753381890 ) ) ;
#37987=ORIENTED_EDGE ( 'NONE', *, *, #52995, .T. ) ;
#37988=CARTESIAN_POINT ( 'NONE',  ( 97.30629616937498838, -209.9999999999999716, 85.67406250086715147 ) ) ;
#37992=CARTESIAN_POINT ( 'NONE',  ( -96.15314808468752972, 91.99731107132950569, 78.90072916753382515 ) ) ;
#37996=CARTESIAN_POINT ( 'NONE',  ( -95.00000000000002842, 90.00000000000004263, 90.00000000000000000 ) ) ;
#37998=CARTESIAN_POINT ( 'NONE',  ( 23.50000000000000355, -120.0000000000000000, -80.00000000000000000 ) ) ;
#37999=CARTESIAN_POINT ( 'NONE',  ( 93.67500000000001137, -207.7050326799711968, 89.33854166840096411 ) ) ;
#38000=ORIENTED_EDGE ( 'NONE', *, *, #44122, .F. ) ;
#38002=EDGE_CURVE ( 'NONE', #49491, #13197, #57157, .T. ) ;
#38020=EDGE_CURVE ( 'NONE', #18128, #46834, #28924, .T. ) ;
#38021=CARTESIAN_POINT ( 'NONE',  ( -95.00000000000002842, 87.33691857156074434, 77.89531250086714920 ) ) ;
#38023=CARTESIAN_POINT ( 'NONE',  ( 97.30629616937498838, 90.00000000000002842, 78.53031250086714010 ) ) ;
#38024=( BOUNDED_CURVE ( )  B_SPLINE_CURVE ( 2, ( #20115, #20503, #54708, #61093, #32130, #65263, #13736 ),
 .UNSPECIFIED., .F., .F. ) 
 B_SPLINE_CURVE_WITH_KNOTS ( ( 3, 2, 2, 3 ),
 ( 0.5624999999999997780, 0.5694444444444440867, 0.5763888888888885065, 0.5833333333333329263 ),
 .UNSPECIFIED. ) 
 CURVE ( )  GEOMETRIC_REPRESENTATION_ITEM ( )  RATIONAL_B_SPLINE_CURVE ( ( 1.000000000000004219, 0.8660254037844343777, 1.000000000000000000, 0.8660254037844387076, 1.000000000000000000, 0.8660254037844472563, 0.9999999999999914513 ) ) 
 REPRESENTATION_ITEM ( '' )  );
#38027=CARTESIAN_POINT ( 'NONE',  ( -97.30629616937497417, -211.3315407142195852, 88.42572916753380241 ) ) ;
#38031=DIRECTION ( 'NONE',  ( 1.000000000000000000, 0.000000000000000000, 0.000000000000000000 ) ) ;
#38032=CARTESIAN_POINT ( 'NONE',  ( -92.69370383062498320, -209.9999999999999716, 81.07031250086714635 ) ) ;
#38040=CARTESIAN_POINT ( 'NONE',  ( -92.34999999999999432, -209.9999999999999716, 89.04749999999999943 ) ) ;
#38044=EDGE_CURVE ( 'NONE', #24954, #23224, #33441, .T. ) ;
#38045=CARTESIAN_POINT ( 'NONE',  ( -93.84685191531252713, 88.00268892867056536, 84.77447916753381207 ) ) ;
#38048=VERTEX_POINT ( 'NONE', #62425 ) ;
#38052=VECTOR ( 'NONE', #6673, 1000.000000000000000 ) ;
#38056=CARTESIAN_POINT ( 'NONE',  ( -96.15314808468745866, -211.9973110713294489, 82.92239583420048632 ) ) ;
#38075=FACE_OUTER_BOUND ( 'NONE', #33482, .T. ) ;
#38076=ORIENTED_EDGE ( 'NONE', *, *, #53215, .F. ) ;
#38092=CARTESIAN_POINT ( 'NONE',  ( 92.69370383062498320, 91.33154071421968467, 77.68364583420047609 ) ) ;
#38094=CARTESIAN_POINT ( 'NONE',  ( -92.35000000000009379, 88.47002178664753558, 85.18458333333332178 ) ) ;
#38100=VERTEX_POINT ( 'NONE', #51483 ) ;
#38101=CARTESIAN_POINT ( 'NONE',  ( 97.30629616937498838, -211.3315407142195852, 87.36739583420047950 ) ) ;
#38104=CARTESIAN_POINT ( 'NONE',  ( 93.67499999999998295, 92.29496732002878900, 77.90854166840097150 ) ) ;
#38106=DIRECTION ( 'NONE',  ( 1.000000000000000000, 0.000000000000000000, 0.000000000000000000 ) ) ;
#38108=CARTESIAN_POINT ( 'NONE',  ( -97.64999999999994884, -208.4700217866474645, 77.32645833506762756 ) ) ;
#38111=CARTESIAN_POINT ( 'NONE',  ( 97.30629616937498838, 91.33154071421968467, 86.83822916753381094 ) ) ;
#38112=CARTESIAN_POINT ( 'NONE',  ( -95.00000000000002842, 87.33691857156074434, 87.26156250086714294 ) ) ;
#38113=ORIENTED_EDGE ( 'NONE', *, *, #65481, .F. ) ;
#38119=CARTESIAN_POINT ( 'NONE',  ( -92.69370383062498320, -211.3315407142195852, 88.63739583420047552 ) ) ;
#38125=ORIENTED_EDGE ( 'NONE', *, *, #54631, .T. ) ;
#38127=CARTESIAN_POINT ( 'NONE',  ( -92.35000000000003695, 90.00000000000004263, 80.79249999999998977 ) ) ;
#38130=EDGE_CURVE ( 'NONE', #71136, #47765, #28179, .T. ) ;
#38139=CARTESIAN_POINT ( 'NONE',  ( -96.15314808468751551, 88.00268892867056536, 81.49364583420047836 ) ) ;
#38141=CARTESIAN_POINT ( 'NONE',  ( -97.65000000000007674, 88.47002178664759242, 85.60791666666665378 ) ) ;
#38150=CARTESIAN_POINT ( 'NONE',  ( 97.30629616937498838, 90.00000000000002842, 79.95906250086714806 ) ) ;
#38151=CARTESIAN_POINT ( 'NONE',  ( -92.69370383062498320, -208.6684592857803295, 81.91697916753383879 ) ) ;
#38155=CARTESIAN_POINT ( 'NONE',  ( -92.34999999999999432, -208.4700217866474645, 76.40041666666667197 ) ) ;
#38156=CARTESIAN_POINT ( 'NONE',  ( 93.67500000000001137, -207.7050326799711968, 78.46416666666667084 ) ) ;
#38157=CARTESIAN_POINT ( 'NONE',  ( -95.00000000000002842, 92.66308142843932671, 76.94281250086714863 ) ) ;
#38158=CARTESIAN_POINT ( 'NONE',  ( 97.30629616937498838, -211.3315407142195852, 82.28739583420048120 ) ) ;
#38159=ORIENTED_EDGE ( 'NONE', *, *, #3433, .F. ) ;
#38160=CARTESIAN_POINT ( 'NONE',  ( 97.30629616937497417, 89.70433482669608338, 74.79348190356854786 ) ) ;
#38167=EDGE_CURVE ( 'NONE', #9432, #53104, #36482, .T. ) ;
#38168=CYLINDRICAL_SURFACE ( 'NONE', #65969, 2.649999999999985700 ) ;
#38170=EDGE_LOOP ( 'NONE', ( #27815, #15066, #60407, #44978 ) ) ;
#38171=ORIENTED_EDGE ( 'NONE', *, *, #25300, .T. ) ;
#38174=CARTESIAN_POINT ( 'NONE',  ( 96.15314808468748708, -208.0026889286704943, 79.42989583420049371 ) ) ;
#38177=CARTESIAN_POINT ( 'NONE',  ( -95.12556226663434700, 87.35320520944279110, 74.99648857272262603 ) ) ;
#38178=CARTESIAN_POINT ( 'NONE',  ( 97.30629616937498838, 91.33154071421968467, 85.09197916753380753 ) ) ;
#38180=CARTESIAN_POINT ( 'NONE',  ( 97.64999999999999147, -209.9999999999999716, 82.06250000000000000 ) ) ;
#38197=CARTESIAN_POINT ( 'NONE',  ( -93.67499999999998295, -212.2949673200287179, 85.84604166840097150 ) ) ;
#38200=ORIENTED_EDGE ( 'NONE', *, *, #51365, .T. ) ;
#38201=CARTESIAN_POINT ( 'NONE',  ( -95.00000000000002842, 93.05995642670501411, 81.66562500173431260 ) ) ;
#38203=CARTESIAN_POINT ( 'NONE',  ( 96.15314808468748708, 91.99731107132950569, 82.60489583420049087 ) ) ;
#38206=CARTESIAN_POINT ( 'NONE',  ( -96.32499999999996021, -207.7050326799711968, 75.28916666666665947 ) ) ;
#38214=ORIENTED_EDGE ( 'NONE', *, *, #8579, .T. ) ;
#38220=CARTESIAN_POINT ( 'NONE',  ( -94.99999999999997158, -207.3369185715606307, 84.56281250086716739 ) ) ;
#38227=CARTESIAN_POINT ( 'NONE',  ( 2.500000000000030198, 65.00000000000000000, -90.00000000000000000 ) ) ;
#38231=CARTESIAN_POINT ( 'NONE',  ( 97.30629616937498838, 90.00000000000002842, 77.26031250086714408 ) ) ;
#38234=CARTESIAN_POINT ( 'NONE',  ( 96.32499999999997442, 92.29496732002878900, 86.69270833506763552 ) ) ;
#38238=CARTESIAN_POINT ( 'NONE',  ( -97.64999999999996305, -209.9999999999999716, 86.82500000000000284 ) ) ;
#38240=PLANE ( 'NONE',  #69790 ) ;
#38243=CARTESIAN_POINT ( 'NONE',  ( -97.30629616937501680, 90.00000000000004263, 81.38781250086714181 ) ) ;
#38251=( BOUNDED_CURVE ( )  B_SPLINE_CURVE ( 2, ( #26438, #14034, #36234, #13668, #36603, #14417, #37364 ),
 .UNSPECIFIED., .F., .F. ) 
 B_SPLINE_CURVE_WITH_KNOTS ( ( 3, 2, 2, 3 ),
 ( 0.8466920362367558184, 0.8537476304467666033, 0.8608033959876488783, 0.8678591737214820245 ),
 .UNSPECIFIED. ) 
 CURVE ( )  GEOMETRIC_REPRESENTATION_ITEM ( )  RATIONAL_B_SPLINE_CURVE ( ( 0.9999934937104038024, 0.8660286570082328383, 1.000000000000000000, 0.8660254037844387076, 1.000000000000000000, 0.8660254037844387076, 1.000000000000000000 ) ) 
 REPRESENTATION_ITEM ( '' )  );
#38254=CARTESIAN_POINT ( 'NONE',  ( 26.50000000000000355, -120.0000000000000000, -80.00000000000000000 ) ) ;
#38255=ADVANCED_FACE ( 'NONE', ( #17650 ), #52968, .F. ) ;
#38256=CARTESIAN_POINT ( 'NONE',  ( 97.64999999989933599, 90.00002309722570715, 83.41187580057898288 ) ) ;
#38257=CARTESIAN_POINT ( 'NONE',  ( 95.00000000000000000, -212.6630814284392557, 77.26031250086714408 ) ) ;
#38263=FACE_OUTER_BOUND ( 'NONE', #73681, .T. ) ;
#38267=CIRCLE ( 'NONE', #64687, 3.299999999999983391 ) ;
#38269=CARTESIAN_POINT ( 'NONE',  ( 96.15314808468750130, -211.9973110713294489, 77.31322916753381946 ) ) ;
#38274=LINE ( 'NONE', #4832, #14303 ) ;
#38283=CARTESIAN_POINT ( 'NONE',  ( 93.67500000000001137, -207.7050326799711968, 80.44854166840097776 ) ) ;
#38284=CARTESIAN_POINT ( 'NONE',  ( 96.32499999999997442, 92.29496732002878900, 82.16833333333332234 ) ) ;
#38288=ADVANCED_FACE ( 'NONE', ( #12004 ), #2242, .F. ) ;
#38290=CARTESIAN_POINT ( 'NONE',  ( 97.65000000000000568, 91.52997821335252127, 84.09979166840098230 ) ) ;
#38291=CARTESIAN_POINT ( 'NONE',  ( -97.30629616937501680, 88.66845928578038638, 85.40947916753381719 ) ) ;
#38292=CARTESIAN_POINT ( 'NONE',  ( 96.15314808468748708, 88.00268892867053694, 80.96447916753380980 ) ) ;
#38297=CARTESIAN_POINT ( 'NONE',  ( -94.99999999999997158, -209.9999999999999716, 90.00000000000000000 ) ) ;
#38309=CARTESIAN_POINT ( 'NONE',  ( -96.32499999999996021, -207.7050326799711968, 81.08354166840096866 ) ) ;
#38311=CARTESIAN_POINT ( 'NONE',  ( 97.64999999999997726, 88.47002178664753558, 87.80395833506763381 ) ) ;
#38314=CARTESIAN_POINT ( 'NONE',  ( -97.30629616937497417, -208.6684592857803011, 78.15989583420048348 ) ) ;
#38316=CARTESIAN_POINT ( 'NONE',  ( -97.65000000000001990, 90.00000000000004263, 86.18999999999999773 ) ) ;
#38322=CARTESIAN_POINT ( 'NONE',  ( -92.35000000000003695, 90.00000000000004263, 90.00000000000000000 ) ) ;
#38323=CARTESIAN_POINT ( 'NONE',  ( 92.69370383062498320, 91.33154071421968467, 87.68489583420047495 ) ) ;
#38326=CARTESIAN_POINT ( 'NONE',  ( -97.64999999960637922, 90.00002930319634231, 82.45844277051273252 ) ) ;
#38331=CARTESIAN_POINT ( 'NONE',  ( 97.64999999999999147, -209.9999999999999716, 75.07749999999998636 ) ) ;
#38333=CARTESIAN_POINT ( 'NONE',  ( 92.35001469846373823, 91.52998669951453792, 76.05645774805350356 ) ) ;
#38339=CARTESIAN_POINT ( 'NONE',  ( -92.34999999999999432, -211.5299782133524502, 83.91458333333333997 ) ) ;
#38344=SURFACE_STYLE_FILL_AREA ( #9392 ) ;
#38360=CARTESIAN_POINT ( 'NONE',  ( 97.30629616937498838, -211.3315407142195852, 81.01739583420048518 ) ) ;
#38361=CARTESIAN_POINT ( 'NONE',  ( 93.84685191531249870, -208.0026889286704943, 84.61572916753381435 ) ) ;
#38363=CARTESIAN_POINT ( 'NONE',  ( 97.30629616937498838, -209.9999999999999716, 85.03906250086714635 ) ) ;
#38367=CARTESIAN_POINT ( 'NONE',  ( -96.15314808468752972, 91.99731107132950569, 76.99572916753382401 ) ) ;
#38380=AXIS2_PLACEMENT_3D ( 'NONE', #49577, #48841, #66876 ) ;
#38391=ORIENTED_EDGE ( 'NONE', *, *, #23887, .F. ) ;
#38395=DIRECTION ( 'NONE',  ( -0.000000000000000000, -0.000000000000000000, 1.000000000000000000 ) ) ;
#38397=CARTESIAN_POINT ( 'NONE',  ( -95.00000000000002842, 92.66308142843932671, 75.67281250086716682 ) ) ;
#38399=CARTESIAN_POINT ( 'NONE',  ( 92.69370383062498320, 90.00000000000002842, 77.57781250086713953 ) ) ;
#38400=EDGE_LOOP ( 'NONE', ( #3166, #26835, #55459, #63660 ) ) ;
#38403=CARTESIAN_POINT ( 'NONE',  ( 96.82636346428390084, -211.7597761561304708, 74.93163452119475210 ) ) ;
#38406=CARTESIAN_POINT ( 'NONE',  ( -94.99999999999997158, -212.6630814284392557, 80.27656250086714351 ) ) ;
#38409=DIRECTION ( 'NONE',  ( -3.061616997868382648E-16, -1.000000000000000000, 0.000000000000000000 ) ) ;
#38415=CARTESIAN_POINT ( 'NONE',  ( 100.0010000000000474, -65.00000000000002842, -290.0000000000000568 ) ) ;
#38419=CARTESIAN_POINT ( 'NONE',  ( 93.26435506835497335, -208.2604367189442769, 74.87701898318914573 ) ) ;
#38420=CARTESIAN_POINT ( 'NONE',  ( -93.84685191531254134, 91.99731107132950569, 83.08114583420048405 ) ) ;
#38429=CARTESIAN_POINT ( 'NONE',  ( -93.84685191531247028, -211.9973110713294489, 78.58322916753382970 ) ) ;
#38438=CARTESIAN_POINT ( 'NONE',  ( 94.99999999999998579, 93.05995642670504253, 77.22062500173429100 ) ) ;
#38441=ADVANCED_FACE ( 'NONE', ( #38263 ), #61204, .F. ) ;
#38442=EDGE_CURVE ( 'NONE', #24481, #32344, #13439, .T. ) ;
#38451=PLANE ( 'NONE',  #12354 ) ;
#38452=ORIENTED_EDGE ( 'NONE', *, *, #17223, .T. ) ;
#38464=EDGE_CURVE ( 'NONE', #5801, #49572, #27054, .T. ) ;
#38468=( BOUNDED_CURVE ( )  B_SPLINE_CURVE ( 2, ( #65642, #26138, #55467, #25036, #47977, #48340, #71628 ),
 .UNSPECIFIED., .F., .F. ) 
 B_SPLINE_CURVE_WITH_KNOTS ( ( 3, 2, 2, 3 ),
 ( 0.3749999999999998335, 0.3819444444444441977, 0.3888888888888886730, 0.3958333333333330373 ),
 .UNSPECIFIED. ) 
 CURVE ( )  GEOMETRIC_REPRESENTATION_ITEM ( )  RATIONAL_B_SPLINE_CURVE ( ( 1.000000000000003109, 0.8660254037844354880, 1.000000000000000000, 0.8660254037844387076, 1.000000000000000000, 0.8660254037844440367, 0.9999999999999946709 ) ) 
 REPRESENTATION_ITEM ( '' )  );
#38469=CARTESIAN_POINT ( 'NONE',  ( 92.69370383062498320, 88.66845928578037217, 77.15447916753382174 ) ) ;
#38475=CARTESIAN_POINT ( 'NONE',  ( 96.15314808468748708, 91.99731107132950569, 86.89114583420047211 ) ) ;
#38476=ORIENTED_EDGE ( 'NONE', *, *, #5244, .F. ) ;
#38477=CARTESIAN_POINT ( 'NONE',  ( 96.15314808468750130, -211.9973110713294489, 84.13947916753380696 ) ) ;
#38482=CARTESIAN_POINT ( 'NONE',  ( -94.99999999999997158, -206.9400435732949575, 80.31624999999999659 ) ) ;
#38485=DIRECTION ( 'NONE',  ( 1.000000000000000000, 0.000000000000000000, 0.000000000000000000 ) ) ;
#38487=CARTESIAN_POINT ( 'NONE',  ( -97.30629616937495996, -209.9999999999999716, 87.10281250086714522 ) ) ;
#38488=CARTESIAN_POINT ( 'NONE',  ( -96.15314808468751551, 88.00268892867056536, 86.73239583420048859 ) ) ;
#38490=CARTESIAN_POINT ( 'NONE',  ( 96.15314808468748708, 88.00268892867053694, 88.58447916753381435 ) ) ;
#38491=CARTESIAN_POINT ( 'NONE',  ( -97.30629616937501680, 90.00000000000004263, 88.37281250086715545 ) ) ;
#38496=CARTESIAN_POINT ( 'NONE',  ( -97.65000000000007674, 91.52997821335253548, 86.77208333333334167 ) ) ;
#38504=CARTESIAN_POINT ( 'NONE',  ( -92.35000000000005116, 88.47002178664754979, 82.64458333333331552 ) ) ;
#38513=CARTESIAN_POINT ( 'NONE',  ( -97.30629616937501680, 90.00000000000004263, 82.02281250086714692 ) ) ;
#38528=EDGE_CURVE ( 'NONE', #2356, #50224, #70999, .T. ) ;
#38529=CARTESIAN_POINT ( 'NONE',  ( 93.84685191531248449, 91.99731107132950569, 81.44072916753381719 ) ) ;
#38531=CARTESIAN_POINT ( 'NONE',  ( -97.30629616937495996, -209.9999999999999716, 84.08656250086716000 ) ) ;
#38533=ORIENTED_EDGE ( 'NONE', *, *, #15302, .T. ) ;
#38535=CARTESIAN_POINT ( 'NONE',  ( -94.99999999999997158, -206.9400435732949575, 78.41125000000000966 ) ) ;
#38536=CARTESIAN_POINT ( 'NONE',  ( 96.32499999999998863, -207.7050326799711968, 78.35833333333333428 ) ) ;
#38538=CARTESIAN_POINT ( 'NONE',  ( -97.30629616937501680, 91.33154071421968467, 77.68364583420047609 ) ) ;
#38539=CARTESIAN_POINT ( 'NONE',  ( 92.69370383062501162, -211.3315407142195852, 82.07572916753380809 ) ) ;
#38547=AXIS2_PLACEMENT_3D ( 'NONE', #67805, #10286, #28310 ) ;
#38551=EDGE_LOOP ( 'NONE', ( #31408, #2833, #24350, #22579, #67400 ) ) ;
#38552=CARTESIAN_POINT ( 'NONE',  ( 95.00000000000000000, -207.3369185715606307, 75.67281250086715261 ) ) ;
#38558=CARTESIAN_POINT ( 'NONE',  ( 93.84685191531248449, 88.00268892867053694, 86.73239583420048859 ) ) ;
#38560=CARTESIAN_POINT ( 'NONE',  ( 92.35000000009272014, 90.00001381026685010, 80.55392363656929433 ) ) ;
#38561=CARTESIAN_POINT ( 'NONE',  ( 95.00000000000000000, -206.9400435732949575, 78.41125000000000966 ) ) ;
#38565=VERTEX_POINT ( 'NONE', #30307 ) ;
#38574=DIRECTION ( 'NONE',  ( 1.000000000000000000, 0.000000000000000000, 0.000000000000000000 ) ) ;
#38577=CARTESIAN_POINT ( 'NONE',  ( -94.99999999999997158, -213.0599564267049857, 85.15812500173430521 ) ) ;
#38581=CARTESIAN_POINT ( 'NONE',  ( -93.67500000000003979, 92.29496732002878900, 84.15270833506762926 ) ) ;
#38584=CARTESIAN_POINT ( 'NONE',  ( 94.99999999999998579, 87.33691857156068750, 83.61031250086716682 ) ) ;
#38585=CARTESIAN_POINT ( 'NONE',  ( 96.32499999999997442, 92.29496732002878900, 83.43833333333333258 ) ) ;
#38593=DIRECTION ( 'NONE',  ( -0.000000000000000000, -0.000000000000000000, 1.000000000000000000 ) ) ;
#38594=ORIENTED_EDGE ( 'NONE', *, *, #23544, .F. ) ;
#38596=EDGE_CURVE ( 'NONE', #44409, #74237, #17821, .T. ) ;
#38601=CARTESIAN_POINT ( 'NONE',  ( -97.30629616937497417, -208.6684592857803011, 81.49364583420047836 ) ) ;
#38608=CARTESIAN_POINT ( 'NONE',  ( 93.67499999999999716, 87.70503267997126784, 81.93020833506763267 ) ) ;
#38611=CARTESIAN_POINT ( 'NONE',  ( 97.30629616937498838, 88.66845928578035796, 79.11239583420046984 ) ) ;
#38616=CARTESIAN_POINT ( 'NONE',  ( 92.49008991410269687, 90.12150787501455795, 74.91582548749272519 ) ) ;
#38619=CARTESIAN_POINT ( 'NONE',  ( 96.32499999999998863, -212.2949673200287179, 84.49666666666666970 ) ) ;
#38626=ADVANCED_FACE ( 'NONE', ( #53252 ), #680, .F. ) ;
#38627=CARTESIAN_POINT ( 'NONE',  ( -97.30629616937501680, 91.33154071421968467, 84.50989583420049200 ) ) ;
#38634=CYLINDRICAL_SURFACE ( 'NONE', #19815, 2.649999999999999467 ) ;
#38639=CARTESIAN_POINT ( 'NONE',  ( 93.84685191531251292, -211.9973110713294489, 79.74739583420048916 ) ) ;
#38646=CARTESIAN_POINT ( 'NONE',  ( -92.34999999999999432, -208.4700217866474645, 85.36979166840096411 ) ) ;
#38650=CARTESIAN_POINT ( 'NONE',  ( 95.00000000000000000, -207.3369185715606307, 75.67281250086716682 ) ) ;
#38660=CARTESIAN_POINT ( 'NONE',  ( 97.64999999999999147, -209.9999999999999716, 81.50687500173430067 ) ) ;
#38661=CARTESIAN_POINT ( 'NONE',  ( 97.64999999999997726, 91.52997821335252127, 80.21041666666666003 ) ) ;
#38664=VECTOR ( 'NONE', #27949, 1000.000000000000000 ) ;
#38670=CARTESIAN_POINT ( 'NONE',  ( -96.15314808468752972, 91.99731107132950569, 83.34572916753383254 ) ) ;
#38671=CARTESIAN_POINT ( 'NONE',  ( 96.15314808468748708, 88.00268892867053694, 79.69447916753379957 ) ) ;
#38679=CARTESIAN_POINT ( 'NONE',  ( -94.99999999999997158, -207.3369185715606307, 81.22906250086715829 ) ) ;
#38685=EDGE_CURVE ( 'NONE', #56878, #3617, #3364, .T. ) ;
#38686=( BOUNDED_CURVE ( )  B_SPLINE_CURVE ( 2, ( #16115, #28131, #72500, #43953, #66870, #4866, #72858 ),
 .UNSPECIFIED., .F., .F. ) 
 B_SPLINE_CURVE_WITH_KNOTS ( ( 3, 2, 2, 3 ),
 ( 0.6458333333333334814, 0.6527777777777779011, 0.6597222222222223209, 0.6666666666666667407 ),
 .UNSPECIFIED. ) 
 CURVE ( )  GEOMETRIC_REPRESENTATION_ITEM ( )  RATIONAL_B_SPLINE_CURVE ( ( 0.9999999999999978906, 0.8660254037844408170, 1.000000000000000000, 0.8660254037844387076, 1.000000000000000000, 0.8660254037844365982, 1.000000000000002220 ) ) 
 REPRESENTATION_ITEM ( '' )  );
#38689=CARTESIAN_POINT ( 'NONE',  ( -96.15314808468745866, -211.9973110713294489, 80.85864583420047325 ) ) ;
#38690=EDGE_LOOP ( 'NONE', ( #9238, #8635, #53657, #12915 ) ) ;
#38698=CARTESIAN_POINT ( 'NONE',  ( 97.30629616937498838, 91.33154071421968467, 87.47322916753380184 ) ) ;
#38699=CARTESIAN_POINT ( 'NONE',  ( -92.34999999999999432, -209.9999999999999716, 83.96750000000000114 ) ) ;
#38702=DIRECTION ( 'NONE',  ( 0.000000000000000000, 0.000000000000000000, 1.000000000000000000 ) ) ;
#38708=CARTESIAN_POINT ( 'NONE',  ( -97.64999999999996305, -209.9999999999999716, 90.00000000000000000 ) ) ;
#38710=COLOUR_RGB ( '', 0.66274510, 0.83137255, 0.94901961) ;
#38715=CARTESIAN_POINT ( 'NONE',  ( -92.34999999999999432, -211.5299782133524502, 85.18458333333332178 ) ) ;
#38717=CARTESIAN_POINT ( 'NONE',  ( -94.60587738269765623, 87.35656277621949073, 75.00000000000001421 ) ) ;
#38727=CARTESIAN_POINT ( 'NONE',  ( 96.15314808468748708, -208.0026889286704943, 87.68489583420048916 ) ) ;
#38729=ORIENTED_EDGE ( 'NONE', *, *, #52128, .T. ) ;
#38734=CARTESIAN_POINT ( 'NONE',  ( 97.30629616937498838, -211.3315407142195852, 79.74739583420047495 ) ) ;
#38735=CARTESIAN_POINT ( 'NONE',  ( 93.84685191531249870, -208.0026889286704943, 85.25072916753381946 ) ) ;
#38738=CARTESIAN_POINT ( 'NONE',  ( 92.69370383062501162, -211.3315407142195852, 84.77447916753381207 ) ) ;
#38742=CARTESIAN_POINT ( 'NONE',  ( -92.69370383062504004, 90.00000000000004263, 75.51406250086715488 ) ) ;
#38744=FACE_OUTER_BOUND ( 'NONE', #32844, .T. ) ;
#38746=FACE_OUTER_BOUND ( 'NONE', #62055, .T. ) ;
#38747=CARTESIAN_POINT ( 'NONE',  ( 92.35000000000002274, -211.5299782133524502, 88.86229166840097093 ) ) ;
#38757=LINE ( 'NONE', #73698, #67858 ) ;
#38764=CARTESIAN_POINT ( 'NONE',  ( -95.00000000000002842, 87.33691857156074434, 77.26031250086714408 ) ) ;
#38766=CARTESIAN_POINT ( 'NONE',  ( 92.69370383062498320, 91.33154071421968467, 77.52489583420046415 ) ) ;
#38775=CARTESIAN_POINT ( 'NONE',  ( -97.30629616937497417, -211.3315407142195852, 80.80572916753379786 ) ) ;
#38777=FACE_OUTER_BOUND ( 'NONE', #23661, .T. ) ;
#38780=CARTESIAN_POINT ( 'NONE',  ( -92.34999999999999432, -209.9999999999999716, 79.52249999999999375 ) ) ;
#38787=CARTESIAN_POINT ( 'NONE',  ( -97.64999999999996305, -209.9999999999999716, 88.73000000000000398 ) ) ;
#38788=CARTESIAN_POINT ( 'NONE',  ( 95.77009744696167104, -207.7668333712726962, 74.81945665767624121 ) ) ;
#38789=CARTESIAN_POINT ( 'NONE',  ( -97.30629616937501680, 88.66845928578038638, 82.07572916753380809 ) ) ;
#38799=CARTESIAN_POINT ( 'NONE',  ( -97.30629616937495996, -209.9999999999999716, 79.00656250086716170 ) ) ;
#38811=ADVANCED_FACE ( 'NONE', ( #9227 ), #32149, .F. ) ;
#38820=CARTESIAN_POINT ( 'NONE',  ( 96.15314808468748708, -208.0026889286704943, 87.52614583420047722 ) ) ;
#38821=CARTESIAN_POINT ( 'NONE',  ( -92.35000000000003695, 90.00000000000004263, 77.61749999999999261 ) ) ;
#38827=CARTESIAN_POINT ( 'NONE',  ( -97.65000000000001990, 90.00000000000004263, 83.01499999999998636 ) ) ;
#38832=ORIENTED_EDGE ( 'NONE', *, *, #6858, .T. ) ;
#38837=CARTESIAN_POINT ( 'NONE',  ( 92.69370383062498320, 90.00000000000002842, 77.73656250086715147 ) ) ;
#38843=CARTESIAN_POINT ( 'NONE',  ( 93.84685191531248449, 88.00268892867053694, 89.11364583420048291 ) ) ;
#38845=CARTESIAN_POINT ( 'NONE',  ( 97.30629616937498838, -209.9999999999999716, 83.61031250086713840 ) ) ;
#38847=DIRECTION ( 'NONE',  ( 1.000000000000000000, 0.000000000000000000, 0.000000000000000000 ) ) ;
#38853=CARTESIAN_POINT ( 'NONE',  ( -92.69370383062498320, -208.6684592857803011, 88.10822916753380696 ) ) ;
#38854=CARTESIAN_POINT ( 'NONE',  ( -93.84685191531252713, 88.00268892867056536, 86.83822916753382515 ) ) ;
#38855=ORIENTED_EDGE ( 'NONE', *, *, #29175, .F. ) ;
#38857=CARTESIAN_POINT ( 'NONE',  ( 97.30629616937498838, 91.33154071421968467, 88.74322916753379786 ) ) ;
#38858=CARTESIAN_POINT ( 'NONE',  ( -97.30629616937501680, 91.33154071421968467, 88.95489583420048518 ) ) ;
#38866=CARTESIAN_POINT ( 'NONE',  ( 97.64999999999997726, -208.4700217866474929, 82.11541666666664696 ) ) ;
#38876=CARTESIAN_POINT ( 'NONE',  ( -97.65000000000001990, 90.00000000000004263, 81.74500000000000455 ) ) ;
#38881=DIRECTION ( 'NONE',  ( -1.000000000000000000, -0.000000000000000000, -0.000000000000000000 ) ) ;
#38886=ORIENTED_EDGE ( 'NONE', *, *, #39737, .F. ) ;
#38887=CARTESIAN_POINT ( 'NONE',  ( -93.84685191531252713, 88.00268892867056536, 82.23447916753380582 ) ) ;
#38891=CARTESIAN_POINT ( 'NONE',  ( -97.65000000000001990, 90.00000000000004263, 85.55499999999999261 ) ) ;
#38895=CARTESIAN_POINT ( 'NONE',  ( -93.84685191531247028, -211.9973110713294489, 88.74322916753382628 ) ) ;
#38898=CARTESIAN_POINT ( 'NONE',  ( 92.69370383062498320, 88.66845928578035796, 79.69447916753381378 ) ) ;
#38899=AXIS2_PLACEMENT_3D ( 'NONE', #56722, #21741, #56339 ) ;
#38900=CARTESIAN_POINT ( 'NONE',  ( -96.15314808468745866, -211.9973110713294489, 80.38239583420048007 ) ) ;
#38903=CARTESIAN_POINT ( 'NONE',  ( -93.67500000000003979, 87.70503267997129626, 87.11604166840096752 ) ) ;
#38905=CARTESIAN_POINT ( 'NONE',  ( 92.35000000000000853, -209.9999999999999716, 78.64937500173429896 ) ) ;
#38906=ADVANCED_FACE ( 'NONE', ( #17377 ), #44192, .F. ) ;
#38908=CARTESIAN_POINT ( 'NONE',  ( -97.30629616937501680, 90.00000000000004263, 79.00656250086716170 ) ) ;
#38909=CARTESIAN_POINT ( 'NONE',  ( 97.30629616937498838, -211.3315407142195852, 81.65239583420049030 ) ) ;
#38910=ORIENTED_EDGE ( 'NONE', *, *, #40685, .T. ) ;
#38911=AXIS2_PLACEMENT_3D ( 'NONE', #28796, #51733, #69029 ) ;
#38914=( BOUNDED_CURVE ( )  B_SPLINE_CURVE ( 2, ( #13280, #36212, #1680, #64803, #47863, #36579, #6905 ),
 .UNSPECIFIED., .F., .F. ) 
 B_SPLINE_CURVE_WITH_KNOTS ( ( 3, 2, 2, 3 ),
 ( 0.08333333333333288462, 0.09027777777777759582, 0.09722222222222230703, 0.1041666666666670182 ),
 .UNSPECIFIED. ) 
 CURVE ( )  GEOMETRIC_REPRESENTATION_ITEM ( )  RATIONAL_B_SPLINE_CURVE ( ( 1.000000000000008660, 0.8660254037844301589, 1.000000000000000000, 0.8660254037844387076, 1.000000000000000000, 0.8660254037844320463, 1.000000000000006661 ) ) 
 REPRESENTATION_ITEM ( '' )  );
#38923=CARTESIAN_POINT ( 'NONE',  ( 96.15314808468748708, -208.0026889286704943, 76.25489583420049655 ) ) ;
#38924=ORIENTED_EDGE ( 'NONE', *, *, #11893, .F. ) ;
#38928=CARTESIAN_POINT ( 'NONE',  ( 92.69370383062498320, 90.00000000000002842, 87.89656250086714806 ) ) ;
#38931=CARTESIAN_POINT ( 'NONE',  ( 93.67500000000001137, -207.7050326799711968, 78.46416666666667084 ) ) ;
#38934=ORIENTED_EDGE ( 'NONE', *, *, #54341, .T. ) ;
#38936=ORIENTED_EDGE ( 'NONE', *, *, #37684, .F. ) ;
#38937=DIRECTION ( 'NONE',  ( 0.000000000000000000, 0.000000000000000000, 1.000000000000000000 ) ) ;
#38940=DIRECTION ( 'NONE',  ( 1.000000000000000000, 0.000000000000000000, 0.000000000000000000 ) ) ;
#38943=CARTESIAN_POINT ( 'NONE',  ( 97.65000000000000568, 88.47002178664752137, 83.99395833506763154 ) ) ;
#38946=CARTESIAN_POINT ( 'NONE',  ( -93.67499999999998295, -207.7050326799711968, 83.51770833506763836 ) ) ;
#38949=AXIS2_PLACEMENT_3D ( 'NONE', #72464, #66840, #31503 ) ;
#38952=CARTESIAN_POINT ( 'NONE',  ( 94.99999999999998579, 86.94004357329500010, 81.98312500173430806 ) ) ;
#38953=CARTESIAN_POINT ( 'NONE',  ( -96.32500000000001705, 87.70503267997129626, 83.83520833506763381 ) ) ;
#38955=CARTESIAN_POINT ( 'NONE',  ( 96.15314808468748708, 88.00268892867053694, 83.02822916753380866 ) ) ;
#38956=CARTESIAN_POINT ( 'NONE',  ( -92.35000000000003695, 90.00000000000004263, 76.34749999999999659 ) ) ;
#38960=DIRECTION ( 'NONE',  ( 0.000000000000000000, -0.000000000000000000, 1.000000000000000000 ) ) ;
#38961=CARTESIAN_POINT ( 'NONE',  ( 93.67499999999998295, 92.29496732002878900, 81.71854166840095957 ) ) ;
#38962=CARTESIAN_POINT ( 'NONE',  ( -97.64999999999996305, -209.9999999999999716, 80.47499999999999432 ) ) ;
#38964=CARTESIAN_POINT ( 'NONE',  ( -97.64995694994087216, 91.53000306831579280, 81.13645661577284329 ) ) ;
#38965=CARTESIAN_POINT ( 'NONE',  ( -97.65000000000001990, 90.00003216987890653, 82.45937388908920695 ) ) ;
#38969=VERTEX_POINT ( 'NONE', #28276 ) ;
#38973=LINE ( 'NONE', #63040, #52111 ) ;
#38974=CARTESIAN_POINT ( 'NONE',  ( -92.69370383062498320, -209.9999999999999716, 82.49906250086715431 ) ) ;
#38980=VECTOR ( 'NONE', #9710, 1000.000000000000000 ) ;
#38983=CARTESIAN_POINT ( 'NONE',  ( 96.15314808468748708, 91.99731107132950569, 75.46114583420047950 ) ) ;
#38995=FACE_OUTER_BOUND ( 'NONE', #63384, .T. ) ;
#38998=CARTESIAN_POINT ( 'NONE',  ( -93.84685191531252713, 88.00268892867056536, 82.23447916753380582 ) ) ;
#39003=FACE_OUTER_BOUND ( 'NONE', #73094, .T. ) ;
#39009=CARTESIAN_POINT ( 'NONE',  ( 97.30629616937498838, -209.9999999999999716, 75.51406250086715488 ) ) ;
#39012=EDGE_CURVE ( 'NONE', #4009, #73251, #9700, .T. ) ;
#39018=CARTESIAN_POINT ( 'NONE',  ( 92.35000000000002274, -208.4700217866474645, 86.77208333333334167 ) ) ;
#39022=ORIENTED_EDGE ( 'NONE', *, *, #35315, .T. ) ;
#39023=CYLINDRICAL_SURFACE ( 'NONE', #46550, 2.649999999999985700 ) ;
#39028=CARTESIAN_POINT ( 'NONE',  ( 95.00000000000000000, -206.9400435732949575, 78.49062500173430124 ) ) ;
#39029=CARTESIAN_POINT ( 'NONE',  ( 95.00000000000000000, -213.0599564267049857, 80.71312500173431204 ) ) ;
#39030=CARTESIAN_POINT ( 'NONE',  ( 97.64999999999999147, 90.00000000000002842, 83.33250000000001023 ) ) ;
#39033=CARTESIAN_POINT ( 'NONE',  ( 93.67500000000001137, -207.7050326799711968, 75.36854166840096525 ) ) ;
#39038=CARTESIAN_POINT ( 'NONE',  ( -93.84685191531254134, 91.99731107132950569, 83.87489583420048689 ) ) ;
#39040=CARTESIAN_POINT ( 'NONE',  ( 94.99999999999998579, 87.33691857156068750, 79.00656250086713328 ) ) ;
#39042=ORIENTED_EDGE ( 'NONE', *, *, #72567, .T. ) ;
#39050=VECTOR ( 'NONE', #22452, 1000.000000000000000 ) ;
#39051=CARTESIAN_POINT ( 'NONE',  ( -92.69370383062498320, -208.6684592857803011, 81.75822916753381264 ) ) ;
#39056=ORIENTED_EDGE ( 'NONE', *, *, #71596, .F. ) ;
#39057=DIRECTION ( 'NONE',  ( 1.000000000000000000, 0.000000000000000000, 0.000000000000000000 ) ) ;
#39058=CARTESIAN_POINT ( 'NONE',  ( 93.67499999999999716, 87.70503267997126784, 80.58083333333331666 ) ) ;
#39060=CARTESIAN_POINT ( 'NONE',  ( -97.30629616937497417, -208.6684592857803011, 76.88989583420047325 ) ) ;
#39062=CARTESIAN_POINT ( 'NONE',  ( 92.35000000045006630, 89.99996890530464100, 88.81037122970248276 ) ) ;
#39065=CARTESIAN_POINT ( 'NONE',  ( -92.34999999999999432, -209.9999999999999716, 76.34749999999999659 ) ) ;
#39068=CARTESIAN_POINT ( 'NONE',  ( -97.65000000000001990, 90.00000000000004263, 81.10999999999999943 ) ) ;
#39070=CARTESIAN_POINT ( 'NONE',  ( -97.64999999999997726, 88.47002178664750716, 89.41791666666667027 ) ) ;
#39071=CARTESIAN_POINT ( 'NONE',  ( 94.99999999999998579, 92.66308142843932671, 87.57906250086713840 ) ) ;
#39074=CARTESIAN_POINT ( 'NONE',  ( 97.64999999999992042, -208.4700217866473793, 86.56041666666668277 ) ) ;
#39081=AXIS2_PLACEMENT_3D ( 'NONE', #15693, #72807, #44269 ) ;
#39089=CARTESIAN_POINT ( 'NONE',  ( -92.34999999999999432, -209.9999999999999716, 83.96750000000000114 ) ) ;
#39090=CARTESIAN_POINT ( 'NONE',  ( 97.64999999999999147, 90.00000000000002842, 87.77749999999998920 ) ) ;
#39096=CARTESIAN_POINT ( 'NONE',  ( 96.66077099052525057, -211.6002630214759961, 74.64190534806809296 ) ) ;
#39102=CARTESIAN_POINT ( 'NONE',  ( -93.67499999999998295, -207.7050326799711968, 79.70770833506762187 ) ) ;
#39104=CARTESIAN_POINT ( 'NONE',  ( 92.69370383062501162, -211.3315407142195852, 76.99572916753380980 ) ) ;
#39107=CARTESIAN_POINT ( 'NONE',  ( 92.69370383062501162, -211.3315407142195852, 81.59947916753381492 ) ) ;
#39111=ORIENTED_EDGE ( 'NONE', *, *, #55414, .F. ) ;
#39117=ORIENTED_EDGE ( 'NONE', *, *, #67415, .F. ) ;
#39124=( BOUNDED_CURVE ( )  B_SPLINE_CURVE ( 2, ( #51698, #23140, #6583, #29487, #43403, #14798, #71935 ),
 .UNSPECIFIED., .F., .F. ) 
 B_SPLINE_CURVE_WITH_KNOTS ( ( 3, 2, 2, 3 ),
 ( 0.3749999999999998335, 0.3819444444444441977, 0.3888888888888886730, 0.3958333333333330373 ),
 .UNSPECIFIED. ) 
 CURVE ( )  GEOMETRIC_REPRESENTATION_ITEM ( )  RATIONAL_B_SPLINE_CURVE ( ( 1.000000000000003109, 0.8660254037844354880, 1.000000000000000000, 0.8660254037844387076, 1.000000000000000000, 0.8660254037844440367, 0.9999999999999946709 ) ) 
 REPRESENTATION_ITEM ( '' )  );
#39130=CARTESIAN_POINT ( 'NONE',  ( 96.15314808468750130, -211.9973110713294489, 75.88447916753381151 ) ) ;
#39137=CARTESIAN_POINT ( 'NONE',  ( -92.69370383062502583, 91.33154071421968467, 76.83697916753382628 ) ) ;
#39140=CARTESIAN_POINT ( 'NONE',  ( 96.15314808468748708, 88.00268892867053694, 78.42447916753381776 ) ) ;
#39143=CARTESIAN_POINT ( 'NONE',  ( -97.30629616937497417, -208.6684592857803011, 85.14489583420048291 ) ) ;
#39149=CARTESIAN_POINT ( 'NONE',  ( -93.84685191531247028, -211.9973110713294489, 79.69447916753379957 ) ) ;
#39150=CARTESIAN_POINT ( 'NONE',  ( 93.67499999999999716, 87.70503267997126784, 86.93083333333332519 ) ) ;
#39153=CARTESIAN_POINT ( 'NONE',  ( -96.32499999999996021, -207.7050326799711968, 84.17916666666666003 ) ) ;
#39157=LINE ( 'NONE', #44057, #19230 ) ;
#39159=CARTESIAN_POINT ( 'NONE',  ( 97.64999999999997726, 91.52997821335253548, 84.65541666666669585 ) ) ;
#39162=CARTESIAN_POINT ( 'NONE',  ( -96.15314808468752972, 91.99731107132950569, 83.18697916753382060 ) ) ;
#39170=CARTESIAN_POINT ( 'NONE',  ( 92.35000000000000853, -209.9999999999999716, 81.74500000000000455 ) ) ;
#39174=CARTESIAN_POINT ( 'NONE',  ( -97.65000000000001990, 90.00000000000004263, 87.45999999999999375 ) ) ;
#39175=CARTESIAN_POINT ( 'NONE',  ( -92.69370383062498320, -208.6684592857803011, 78.10697916753383652 ) ) ;
#39183=DIRECTION ( 'NONE',  ( -0.000000000000000000, -0.000000000000000000, 1.000000000000000000 ) ) ;
#39191=CARTESIAN_POINT ( 'NONE',  ( 92.69370383062501162, -208.6684592857803295, 87.04989583420046984 ) ) ;
#39201=EDGE_CURVE ( 'NONE', #25433, #49534, #34081, .T. ) ;
#39211=AXIS2_PLACEMENT_3D ( 'NONE', #16589, #33129, #67731 ) ;
#39214=CARTESIAN_POINT ( 'NONE',  ( 94.99999999999998579, 87.33691857156068750, 76.62531250086715318 ) ) ;
#39219=EDGE_CURVE ( 'NONE', #20422, #57250, #22469, .T. ) ;
#39221=CARTESIAN_POINT ( 'NONE',  ( 94.99999999999998579, 87.33691857156068750, 89.16656250086712987 ) ) ;
#39223=CARTESIAN_POINT ( 'NONE',  ( 97.30629616937498838, -209.9999999999999716, 84.24531250086714351 ) ) ;
#39231=CARTESIAN_POINT ( 'NONE',  ( 92.34999999999999432, 88.47002178664752137, 85.05229166840096866 ) ) ;
#39232=CARTESIAN_POINT ( 'NONE',  ( -94.99999999999997158, -212.6630814284392557, 86.62656250086715204 ) ) ;
#39233=CARTESIAN_POINT ( 'NONE',  ( -92.69370383062502583, 88.66845928578038638, 84.98614583420047097 ) ) ;
#39235=CARTESIAN_POINT ( 'NONE',  ( 96.15314808468748708, 91.99731107132950569, 89.43114583420047836 ) ) ;
#39236=CARTESIAN_POINT ( 'NONE',  ( -95.00000000000002842, 92.66308142843932671, 85.67406250086715147 ) ) ;
#39238=CARTESIAN_POINT ( 'NONE',  ( 97.30629616937498838, 91.33154071421968467, 74.93197916753381094 ) ) ;
#39243=CARTESIAN_POINT ( 'NONE',  ( -97.30629616937497417, -211.3315407142195852, 88.42572916753381662 ) ) ;
#39244=FACE_OUTER_BOUND ( 'NONE', #70591, .T. ) ;
#39253=CARTESIAN_POINT ( 'NONE',  ( -97.65000000000001990, 88.47002178664754979, 81.16291666666666060 ) ) ;
#39262=CARTESIAN_POINT ( 'NONE',  ( -93.84685191531252713, 88.00268892867056536, 83.50447916753381605 ) ) ;
#39265=CYLINDRICAL_SURFACE ( 'NONE', #48972, 2.649999999999985700 ) ;
#39270=CARTESIAN_POINT ( 'NONE',  ( -97.30629616937495996, -209.9999999999999716, 89.80156250086714920 ) ) ;
#39273=( BOUNDED_CURVE ( )  B_SPLINE_CURVE ( 2, ( #7976, #30892, #2384, #25277, #48201, #10188, #21843, #55688, #67339 ),
 .UNSPECIFIED., .F., .F. ) 
 B_SPLINE_CURVE_WITH_KNOTS ( ( 3, 2, 2, 2, 3 ),
 ( 0.7196881748034550386, 0.7267438507108833212, 0.7337996162517648191, 0.7408553817926464280, 0.7408554641864709689 ),
 .UNSPECIFIED. ) 
 CURVE ( )  GEOMETRIC_REPRESENTATION_ITEM ( )  RATIONAL_B_SPLINE_CURVE ( ( 0.9999965961303289852, 0.8660271057408951423, 1.000000000000000000, 0.8660254037844387076, 1.000000000000000000, 0.8660254037844387076, 1.000000000000000000, 0.9999984355093277655, 0.9999968710551943030 ) ) 
 REPRESENTATION_ITEM ( '' )  );
#39275=CARTESIAN_POINT ( 'NONE',  ( 97.30629616937498838, 88.66845928578035796, 80.54114583420049200 ) ) ;
#39276=CARTESIAN_POINT ( 'NONE',  ( -94.99999999999997158, -207.3369185715606307, 80.11781250086714579 ) ) ;
#39278=ORIENTED_EDGE ( 'NONE', *, *, #27692, .T. ) ;
#39279=CARTESIAN_POINT ( 'NONE',  ( 92.34999999999999432, 90.00000000000002842, 88.09499999999999886 ) ) ;
#39281=CARTESIAN_POINT ( 'NONE',  ( 93.67499999999998295, 92.29496732002878900, 85.52854166840096184 ) ) ;
#39283=CARTESIAN_POINT ( 'NONE',  ( -97.30629616937501680, 90.00000000000004263, 79.64156250086715261 ) ) ;
#39284=CARTESIAN_POINT ( 'NONE',  ( 97.30629616937498838, -209.9999999999999716, 79.80031250086713612 ) ) ;
#39292=DIRECTION ( 'NONE',  ( 0.000000000000000000, -0.000000000000000000, 1.000000000000000000 ) ) ;
#39293=ADVANCED_FACE ( 'NONE', ( #41599 ), #18295, .F. ) ;
#39304=CARTESIAN_POINT ( 'NONE',  ( 97.30629616937498838, 88.66845928578037217, 86.25614583420048120 ) ) ;
#39306=CARTESIAN_POINT ( 'NONE',  ( 95.00000000000000000, -206.9400435732949575, 76.50624999999999432 ) ) ;
#39316=DIRECTION ( 'NONE',  ( 1.000000000000000000, 0.000000000000000000, 0.000000000000000000 ) ) ;
#39317=CARTESIAN_POINT ( 'NONE',  ( -97.64999999998384794, -210.0000060634594661, 88.17456390440159453 ) ) ;
#39319=CARTESIAN_POINT ( 'NONE',  ( 92.35000000049315361, 89.99996796133687837, 83.73041644179049570 ) ) ;
#39321=CARTESIAN_POINT ( 'NONE',  ( -92.34999999999999432, -208.4700217866474645, 84.09979166840095388 ) ) ;
#39325=CARTESIAN_POINT ( 'NONE',  ( 97.64999999999997726, 91.52997821335252127, 82.82979166840095786 ) ) ;
#39326=CARTESIAN_POINT ( 'NONE',  ( -95.00000000000002842, 86.94004357329504273, 80.07812500173432113 ) ) ;
#39327=ORIENTED_EDGE ( 'NONE', *, *, #1834, .F. ) ;
#39328=CARTESIAN_POINT ( 'NONE',  ( 97.30629616937498838, 90.00000000000002842, 83.76906250086716454 ) ) ;
#39335=DIRECTION ( 'NONE',  ( -0.000000000000000000, 0.000000000000000000, -1.000000000000000000 ) ) ;
#39340=ORIENTED_EDGE ( 'NONE', *, *, #39219, .T. ) ;
#39341=VECTOR ( 'NONE', #71722, 1000.000000000000000 ) ;
#39343=VECTOR ( 'NONE', #36064, 1000.000000000000000 ) ;
#39347=CARTESIAN_POINT ( 'NONE',  ( -93.84685191531248449, -208.0026889286704943, 80.69989583420047552 ) ) ;
#39349=CARTESIAN_POINT ( 'NONE',  ( -96.15314808468752972, 91.99731107132950569, 88.90197916753380980 ) ) ;
#39354=DIRECTION ( 'NONE',  ( -0.000000000000000000, -0.000000000000000000, 1.000000000000000000 ) ) ;
#39355=DIRECTION ( 'NONE',  ( -0.000000000000000000, -0.000000000000000000, 1.000000000000000000 ) ) ;
#39357=CARTESIAN_POINT ( 'NONE',  ( 97.64999999999999147, 89.99999996655866141, 87.85687500050293863 ) ) ;
#39358=LINE ( 'NONE', #67555, #1686 ) ;
#39361=( BOUNDED_CURVE ( )  B_SPLINE_CURVE ( 2, ( #33975, #9928, #5060, #73449, #62953, #26847, #11055, #51260, #17065 ),
 .UNSPECIFIED., .F., .F. ) 
 B_SPLINE_CURVE_WITH_KNOTS ( ( 3, 2, 2, 2, 3 ),
 ( 0.8255245790604923695, 0.8325803338282082855, 0.8396360993691253105, 0.8466918649100423355, 0.8466920362409167122 ),
 .UNSPECIFIED. ) 
 CURVE ( )  GEOMETRIC_REPRESENTATION_ITEM ( )  RATIONAL_B_SPLINE_CURVE ( ( 1.000000000000000000, 0.8660254037844387076, 1.000000000000000000, 0.8660254037844387076, 1.000000000000000000, 0.8660254037844387076, 1.000000000000000000, 0.9999967467761544659, 0.9999934937103009958 ) ) 
 REPRESENTATION_ITEM ( '' )  );
#39369=CARTESIAN_POINT ( 'NONE',  ( -92.69370383062504004, 90.00000000000004263, 78.53031250086714010 ) ) ;
#39371=CARTESIAN_POINT ( 'NONE',  ( 96.15314808468750130, -211.9973110713294489, 89.21947916753380525 ) ) ;
#39378=CARTESIAN_POINT ( 'NONE',  ( 92.35000000049298308, -210.0000320324309939, 85.63541623677062375 ) ) ;
#39379=CARTESIAN_POINT ( 'NONE',  ( 95.00000000000000000, -207.3369185715606307, 75.03781250086714749 ) ) ;
#39394=CARTESIAN_POINT ( 'NONE',  ( 92.35000000000002274, -211.5299782133524502, 87.51291666666666913 ) ) ;
#39397=VERTEX_POINT ( 'NONE', #46504 ) ;
#39399=DIRECTION ( 'NONE',  ( 1.000000000000000000, 0.000000000000000000, 0.000000000000000000 ) ) ;
#39402=CARTESIAN_POINT ( 'NONE',  ( 96.32499999999998863, -212.2949673200287179, 75.68604166840097491 ) ) ;
#39403=CARTESIAN_POINT ( 'NONE',  ( 92.34999999999999432, 88.47002178664753558, 82.43291666666665662 ) ) ;
#39406=CARTESIAN_POINT ( 'NONE',  ( 92.35000000000000853, -208.4700217866474645, 75.42145833506764063 ) ) ;
#39411=ORIENTED_EDGE ( 'NONE', *, *, #5650, .F. ) ;
#39412=CARTESIAN_POINT ( 'NONE',  ( -92.69370383062504004, 90.00000000000004263, 84.40406250086715545 ) ) ;
#39413=CARTESIAN_POINT ( 'NONE',  ( 97.30629616937498838, 90.00000000000002842, 78.53031250086714010 ) ) ;
#39420=CYLINDRICAL_SURFACE ( 'NONE', #41938, 2.649999999999985700 ) ;
#39424=CARTESIAN_POINT ( 'NONE',  ( -97.30629616937497417, -211.3315407142195852, 78.90072916753381094 ) ) ;
#39429=CARTESIAN_POINT ( 'NONE',  ( -92.35000000053402403, -209.9999467984910382, 78.96687695417375608 ) ) ;
#39430=ORIENTED_EDGE ( 'NONE', *, *, #15289, .T. ) ;
#39431=DIRECTION ( 'NONE',  ( 1.000000000000000000, 0.000000000000000000, 0.000000000000000000 ) ) ;
#39432=CARTESIAN_POINT ( 'NONE',  ( 92.34999999999999432, 90.00000000000002842, 89.90078125043358170 ) ) ;
#39434=CARTESIAN_POINT ( 'NONE',  ( -97.30629616937497417, -211.3315407142195852, 77.63072916753380071 ) ) ;
#39444=CARTESIAN_POINT ( 'NONE',  ( 92.69370383062498320, 88.66845928578035796, 85.25072916753379104 ) ) ;
#39448=CARTESIAN_POINT ( 'NONE',  ( -2.500000000000015543, -73.00000000000001421, -255.0000000000000000 ) ) ;
#39452=CARTESIAN_POINT ( 'NONE',  ( 94.99999999999998579, 86.94004357329502852, 86.42812500173430124 ) ) ;
#39462=CARTESIAN_POINT ( 'NONE',  ( -97.64999999999994884, -208.4700217866474645, 84.86708333333334053 ) ) ;
#39467=CARTESIAN_POINT ( 'NONE',  ( 92.34999999999999432, 90.00000000000002842, 90.00000000000000000 ) ) ;
#39473=CARTESIAN_POINT ( 'NONE',  ( 97.30629616937498838, -211.3315407142195852, 86.89114583420050053 ) ) ;
#39477=ORIENTED_EDGE ( 'NONE', *, *, #56665, .F. ) ;
#39478=CARTESIAN_POINT ( 'NONE',  ( 15.69955575014744831, 0.001194404164628767254, -85.59999999999999432 ) ) ;
#39481=CARTESIAN_POINT ( 'NONE',  ( 92.69370383062501162, -209.9999999999999716, 79.48281250086714067 ) ) ;
#39482=EDGE_CURVE ( 'NONE', #6061, #47426, #9232, .T. ) ;
#39484=CARTESIAN_POINT ( 'NONE',  ( 97.30629616937498838, -209.9999999999999716, 82.49906250086715431 ) ) ;
#39489=VERTEX_POINT ( 'NONE', #65651 ) ;
#39498=EDGE_CURVE ( 'NONE', #14250, #10456, #64828, .T. ) ;
#39507=VERTEX_POINT ( 'NONE', #49458 ) ;
#39508=ORIENTED_EDGE ( 'NONE', *, *, #65216, .F. ) ;
#39509=CARTESIAN_POINT ( 'NONE',  ( 97.30629616937498838, -211.3315407142195852, 75.93739583420047268 ) ) ;
#39512=ORIENTED_EDGE ( 'NONE', *, *, #70463, .T. ) ;
#39514=LINE ( 'NONE', #62457, #42123 ) ;
#39516=CARTESIAN_POINT ( 'NONE',  ( -96.15314808468752972, 91.99731107132950569, 76.99572916753382401 ) ) ;
#39520=CARTESIAN_POINT ( 'NONE',  ( 97.65000000000006253, 91.52997821335249284, 75.13041666666666174 ) ) ;
#39521=CARTESIAN_POINT ( 'NONE',  ( -93.84685191531247028, -211.9973110713294489, 84.77447916753381207 ) ) ;
#39526=CARTESIAN_POINT ( 'NONE',  ( -97.30629616937497417, -208.6684592857803295, 78.79489583420047438 ) ) ;
#39528=DIRECTION ( 'NONE',  ( -0.000000000000000000, -0.000000000000000000, 1.000000000000000000 ) ) ;
#39533=CARTESIAN_POINT ( 'NONE',  ( 92.34999999999999432, 90.00000000000002842, 79.83999999999998920 ) ) ;
#39534=CARTESIAN_POINT ( 'NONE',  ( -95.00000000000002842, 92.66308142843932671, 83.13406250086714522 ) ) ;
#39547=CARTESIAN_POINT ( 'NONE',  ( -97.30629616937497417, -211.3315407142195852, 80.32947916753381890 ) ) ;
#39548=ADVANCED_FACE ( 'NONE', ( #37460 ), #54004, .F. ) ;
#39550=EDGE_CURVE ( 'NONE', #17922, #28278, #42867, .T. ) ;
#39558=CARTESIAN_POINT ( 'NONE',  ( 94.99999999999998579, 90.00000000000002842, 90.00000000000000000 ) ) ;
#39559=CARTESIAN_POINT ( 'NONE',  ( 97.64999999999999147, 90.00000000000002842, 90.00000000000000000 ) ) ;
#39562=DIRECTION ( 'NONE',  ( 1.000000000000000000, -0.000000000000000000, 0.000000000000000000 ) ) ;
#39564=( BOUNDED_CURVE ( )  B_SPLINE_CURVE ( 2, ( #38040, #21474, #49675, #44439, #21859, #72599, #38787 ),
 .UNSPECIFIED., .F., .F. ) 
 B_SPLINE_CURVE_WITH_KNOTS ( ( 3, 2, 2, 3 ),
 ( 0.06249999999999966693, 0.06944444444444407283, 0.07638888888888849260, 0.08333333333333288462 ),
 .UNSPECIFIED. ) 
 CURVE ( )  GEOMETRIC_REPRESENTATION_ITEM ( )  RATIONAL_B_SPLINE_CURVE ( ( 1.000000000000006439, 0.8660254037844322683, 1.000000000000000000, 0.8660254037844387076, 1.000000000000000000, 0.8660254037844472563, 0.9999999999999914513 ) ) 
 REPRESENTATION_ITEM ( '' )  );
#39565=CARTESIAN_POINT ( 'NONE',  ( 97.30629616937498838, -208.6684592857803295, 88.10822916753380696 ) ) ;
#39573=ORIENTED_EDGE ( 'NONE', *, *, #58384, .F. ) ;
#39574=CARTESIAN_POINT ( 'NONE',  ( -94.99999999999997158, -213.0599564267049857, 80.07812500173429271 ) ) ;
#39584=CARTESIAN_POINT ( 'NONE',  ( 96.32499999999997442, 92.29496732002878900, 88.51833333333333087 ) ) ;
#39585=CARTESIAN_POINT ( 'NONE',  ( -95.00000000000002842, 90.00000000000004263, 90.00000000000000000 ) ) ;
#39591=CARTESIAN_POINT ( 'NONE',  ( 97.30629616937498838, 90.00000000000002842, 86.78531250086714977 ) ) ;
#39593=CARTESIAN_POINT ( 'NONE',  ( 92.69370383062501162, -208.6684592857803011, 85.14489583420048291 ) ) ;
#39598=CARTESIAN_POINT ( 'NONE',  ( 95.00000000000000000, -209.9999999999999716, 90.00000000000000000 ) ) ;
#39605=CARTESIAN_POINT ( 'NONE',  ( -97.30629616937495996, -209.9999999999999716, 89.00781250086714635 ) ) ;
#39606=CARTESIAN_POINT ( 'NONE',  ( -96.15314808468752972, 91.99731107132950569, 86.52072916753382970 ) ) ;
#39608=CARTESIAN_POINT ( 'NONE',  ( 92.69370383062498320, 90.00000000000002842, 85.19781250086714408 ) ) ;
#39609=CARTESIAN_POINT ( 'NONE',  ( -93.84685191531254134, 91.99731107132950569, 84.35114583420048007 ) ) ;
#39610=ORIENTED_EDGE ( 'NONE', *, *, #18591, .F. ) ;
#39614=CARTESIAN_POINT ( 'NONE',  ( 96.32499999999997442, 92.29496732002878900, 87.24833333333333485 ) ) ;
#39615=CARTESIAN_POINT ( 'NONE',  ( -94.99999999999997158, -212.6630814284392557, 89.16656250086712987 ) ) ;
#39616=DIRECTION ( 'NONE',  ( -0.000000000000000000, -0.000000000000000000, 1.000000000000000000 ) ) ;
#39621=VERTEX_POINT ( 'NONE', #9974 ) ;
#39622=CARTESIAN_POINT ( 'NONE',  ( -95.00000000000002842, 86.94004357329504273, 78.72875000000001933 ) ) ;
#39624=CARTESIAN_POINT ( 'NONE',  ( -92.35000000000003695, 90.00000000000004263, 78.88750000000000284 ) ) ;
#39627=CARTESIAN_POINT ( 'NONE',  ( 94.99999999999998579, 93.05995642670504253, 87.38062500173430180 ) ) ;
#39633=CARTESIAN_POINT ( 'NONE',  ( -92.69370383062502583, 88.66845928578038638, 77.20739583420046870 ) ) ;
#39644=CARTESIAN_POINT ( 'NONE',  ( -96.15314808468747287, -208.0026889286704943, 88.42572916753381662 ) ) ;
#39646=CARTESIAN_POINT ( 'NONE',  ( 93.84685191531248449, 91.99731107132950569, 78.26572916753382003 ) ) ;
#39647=CARTESIAN_POINT ( 'NONE',  ( -97.30629616937497417, -211.3315407142195852, 79.69447916753381378 ) ) ;
#39652=CARTESIAN_POINT ( 'NONE',  ( -92.35000000000003695, 90.00000000000004263, 87.22187500173430408 ) ) ;
#39653=CARTESIAN_POINT ( 'NONE',  ( -95.84368202074679743, -214.6948328857849049, 74.84535815546854565 ) ) ;
#39659=CARTESIAN_POINT ( 'NONE',  ( -95.00000000000002842, 87.33691857156074434, 77.26031250086714408 ) ) ;
#39660=CARTESIAN_POINT ( 'NONE',  ( 92.69370383062501162, -209.9999999999999716, 78.84781250086714977 ) ) ;
#39672=ORIENTED_EDGE ( 'NONE', *, *, #52217, .T. ) ;
#39674=CARTESIAN_POINT ( 'NONE',  ( 97.30629616937498838, -209.9999999999999716, 74.87906250086714977 ) ) ;
#39679=CARTESIAN_POINT ( 'NONE',  ( 97.30629616937498838, 90.00000000000002842, 84.40406250086715545 ) ) ;
#39681=CARTESIAN_POINT ( 'NONE',  ( 92.35000000000000853, -209.9999999999999716, 79.20499999999999829 ) ) ;
#39698=CARTESIAN_POINT ( 'NONE',  ( -97.64999999999994884, -208.4700217866474645, 81.13645833506764404 ) ) ;
#39701=ORIENTED_EDGE ( 'NONE', *, *, #29611, .F. ) ;
#39702=CARTESIAN_POINT ( 'NONE',  ( 94.99999999999998579, 86.94004357329500010, 80.07812500173432113 ) ) ;
#39703=CARTESIAN_POINT ( 'NONE',  ( -92.35000000000005116, 88.47002178664754979, 80.81895833506764859 ) ) ;
#39705=CARTESIAN_POINT ( 'NONE',  ( 92.69370383062498320, 88.66845928578037217, 84.77447916753381207 ) ) ;
#39706=CYLINDRICAL_SURFACE ( 'NONE', #66192, 2.649999999999985700 ) ;
#39707=LINE ( 'NONE', #34049, #51105 ) ;
#39713=CARTESIAN_POINT ( 'NONE',  ( -92.35000000002600018, 89.99998827382285072, 82.77687459617033028 ) ) ;
#39720=CARTESIAN_POINT ( 'NONE',  ( -92.35000000000177067, -209.9999969335172807, 75.79187510780353421 ) ) ;
#39723=CARTESIAN_POINT ( 'NONE',  ( -92.69370383062498320, -208.6684592857803011, 82.55197916753382970 ) ) ;
#39725=CARTESIAN_POINT ( 'NONE',  ( -93.84685191531254134, 91.99731107132950569, 88.79614583420047325 ) ) ;
#39726=VERTEX_POINT ( 'NONE', #33264 ) ;
#39728=CARTESIAN_POINT ( 'NONE',  ( 95.00000000000000000, -209.9999999999999716, 90.00000000000000000 ) ) ;
#39730=EDGE_CURVE ( 'NONE', #8961, #8129, #71163, .T. ) ;
#39735=CARTESIAN_POINT ( 'NONE',  ( -92.34999999999999432, -209.9999999999999716, 78.88750000000000284 ) ) ;
#39737=EDGE_CURVE ( 'NONE', #66290, #16867, #61496, .T. ) ;
#39738=DIRECTION ( 'NONE',  ( -0.000000000000000000, -0.000000000000000000, -1.000000000000000000 ) ) ;
#39741=CARTESIAN_POINT ( 'NONE',  ( 97.30629616937498838, 90.00000000000002842, 87.57906250086715261 ) ) ;
#39747=CARTESIAN_POINT ( 'NONE',  ( -93.84685191531252713, 88.00268892867056536, 80.32947916753380468 ) ) ;
#39753=CARTESIAN_POINT ( 'NONE',  ( 92.34999999999990905, 88.47002178664756400, 83.06791666666666174 ) ) ;
#39756=CARTESIAN_POINT ( 'NONE',  ( 93.67500000000001137, -212.2949673200287179, 85.74020833506763495 ) ) ;
#39759=LINE ( 'NONE', #62708, #40562 ) ;
#39769=CARTESIAN_POINT ( 'NONE',  ( 92.35000000000000853, -209.9999999999999716, 89.36499999999999488 ) ) ;
#39779=CARTESIAN_POINT ( 'NONE',  ( 92.35000000000000853, -209.9999999999999716, 76.10937500173430692 ) ) ;
#39780=CARTESIAN_POINT ( 'NONE',  ( 94.99999999999998579, 93.05995642670504253, 80.95125000000000171 ) ) ;
#39782=CARTESIAN_POINT ( 'NONE',  ( 92.35000000000000853, -210.0000123297515984, 75.47437542817786493 ) ) ;
#39786=CARTESIAN_POINT ( 'NONE',  ( 94.99999999999998579, 86.94004357329502852, 84.52312500173428589 ) ) ;
#39787=CARTESIAN_POINT ( 'NONE',  ( -92.69370383062505425, 88.66845928578038638, 81.81114583420048803 ) ) ;
#39788=CARTESIAN_POINT ( 'NONE',  ( 92.69370383062498320, 88.66845928578037217, 76.99572916753380980 ) ) ;
#39796=CARTESIAN_POINT ( 'NONE',  ( -97.30629616937495996, -209.9999999999999716, 76.30781250086714351 ) ) ;
#39797=ORIENTED_EDGE ( 'NONE', *, *, #57378, .F. ) ;
#39802=VERTEX_POINT ( 'NONE', #18487 ) ;
#39806=( BOUNDED_CURVE ( )  B_SPLINE_CURVE ( 2, ( #70251, #12017, #2260, #58618, #24408, #7123, #30040 ),
 .UNSPECIFIED., .F., .F. ) 
 B_SPLINE_CURVE_WITH_KNOTS ( ( 3, 2, 2, 3 ),
 ( 0.3749999999999998335, 0.3819444444444441977, 0.3888888888888886730, 0.3958333333333330373 ),
 .UNSPECIFIED. ) 
 CURVE ( )  GEOMETRIC_REPRESENTATION_ITEM ( )  RATIONAL_B_SPLINE_CURVE ( ( 1.000000000000003109, 0.8660254037844354880, 1.000000000000000000, 0.8660254037844387076, 1.000000000000000000, 0.8660254037844440367, 0.9999999999999946709 ) ) 
 REPRESENTATION_ITEM ( '' )  );
#39807=CARTESIAN_POINT ( 'NONE',  ( -94.99999999999997158, -212.6630814284392557, 76.46656250086712703 ) ) ;
#39809=CARTESIAN_POINT ( 'NONE',  ( -92.34999999999999432, -209.9999999999999716, 81.42749999999999488 ) ) ;
#39818=CARTESIAN_POINT ( 'NONE',  ( 96.32499999999998863, -207.7050326799711968, 86.05770833506763040 ) ) ;
#39819=CARTESIAN_POINT ( 'NONE',  ( 92.69370383062498320, 88.66845928578035796, 86.52072916753381548 ) ) ;
#39820=CARTESIAN_POINT ( 'NONE',  ( -92.34999999999999432, -209.9999999999999716, 75.07749999999998636 ) ) ;
#39821=VECTOR ( 'NONE', #26504, 1000.000000000000000 ) ;
#39824=CARTESIAN_POINT ( 'NONE',  ( 96.66734480923264528, -212.0887925413173321, 75.00000000000000000 ) ) ;
#39833=DIRECTION ( 'NONE',  ( -0.000000000000000000, -0.000000000000000000, 1.000000000000000000 ) ) ;
#39836=CARTESIAN_POINT ( 'NONE',  ( -92.34999999999999432, -211.5299782133524502, 83.27958333333333485 ) ) ;
#39837=ADVANCED_FACE ( 'NONE', ( #8321 ), #2357, .F. ) ;
#39838=CARTESIAN_POINT ( 'NONE',  ( -95.00000000000002842, 86.94004357329504273, 79.99874999999998693 ) ) ;
#39847=ADVANCED_FACE ( 'NONE', ( #35769 ), #53811, .F. ) ;
#39849=CARTESIAN_POINT ( 'NONE',  ( 92.69370383062501162, -209.9999999999999716, 86.62656250086715204 ) ) ;
#39858=CARTESIAN_POINT ( 'NONE',  ( 92.69370383062501162, -211.3315407142195852, 77.63072916753380071 ) ) ;
#39860=CARTESIAN_POINT ( 'NONE',  ( 97.30629616937498838, -209.9999999999999716, 81.86406250086714920 ) ) ;
#39863=ORIENTED_EDGE ( 'NONE', *, *, #25300, .F. ) ;
#39871=CARTESIAN_POINT ( 'NONE',  ( 93.67500000000001137, -212.2949673200287179, 76.85020833506763438 ) ) ;
#39872=CARTESIAN_POINT ( 'NONE',  ( 93.67500000000001137, -212.2949673200287179, 87.64520833506762187 ) ) ;
#39873=ORIENTED_EDGE ( 'NONE', *, *, #55685, .T. ) ;
#39876=CARTESIAN_POINT ( 'NONE',  ( -97.30629616937501680, 91.33154071421968467, 89.74864583420048803 ) ) ;
#39878=ORIENTED_EDGE ( 'NONE', *, *, #26144, .F. ) ;
#39882=EDGE_LOOP ( 'NONE', ( #38214, #29730, #64523, #7200 ) ) ;
#39889=CARTESIAN_POINT ( 'NONE',  ( -97.30629616937501680, 90.00000000000004263, 77.10156250086714635 ) ) ;
#39891=CARTESIAN_POINT ( 'NONE',  ( 92.69370383062498320, 90.00000000000002842, 89.80156250086714920 ) ) ;
#39895=CARTESIAN_POINT ( 'NONE',  ( -92.69370383062498320, -209.9999999999999716, 86.15031250086714465 ) ) ;
#39897=CARTESIAN_POINT ( 'NONE',  ( -93.07557990970633455, 88.17815826261617929, 75.00000000000001421 ) ) ;
#39900=CARTESIAN_POINT ( 'NONE',  ( -97.30629616937497417, -211.3315407142195852, 75.09072916753380866 ) ) ;
#39909=LINE ( 'NONE', #23354, #49551 ) ;
#39910=CARTESIAN_POINT ( 'NONE',  ( 92.34999999999999432, 88.47002178664752137, 79.97229166840095615 ) ) ;
#39912=CARTESIAN_POINT ( 'NONE',  ( -92.69370383062502583, 88.66845928578038638, 81.01739583420048518 ) ) ;
#39924=CARTESIAN_POINT ( 'NONE',  ( -96.32500000000001705, 92.29496732002878900, 85.52854166840096184 ) ) ;
#39925=CARTESIAN_POINT ( 'NONE',  ( -94.99999999999997158, -207.3369185715606307, 80.75281250086715090 ) ) ;
#39926=ADVANCED_FACE ( 'NONE', ( #27451 ), #26708, .F. ) ;
#39928=ADVANCED_FACE ( 'NONE', ( #60936 ), #8696, .F. ) ;
#39939=CARTESIAN_POINT ( 'NONE',  ( 97.30629616937498838, -209.9999999999999716, 88.05531250086713158 ) ) ;
#39942=CARTESIAN_POINT ( 'NONE',  ( 97.65000000000000568, -211.5299782133524502, 89.62958333333334338 ) ) ;
#39946=CARTESIAN_POINT ( 'NONE',  ( -92.34999999999999432, -211.5299782133524218, 80.18395833506764347 ) ) ;
#39950=ORIENTED_EDGE ( 'NONE', *, *, #2151, .F. ) ;
#39955=AXIS2_PLACEMENT_3D ( 'NONE', #64912, #29192, #70152 ) ;
#39961=CARTESIAN_POINT ( 'NONE',  ( 92.69370383062498320, 91.33154071421968467, 86.41489583420047893 ) ) ;
#39964=CARTESIAN_POINT ( 'NONE',  ( 93.84685191531249870, -208.0026889286704943, 83.82197916753381151 ) ) ;
#39973=CARTESIAN_POINT ( 'NONE',  ( -96.15314808468747287, -208.0026889286704943, 88.26697916753380468 ) ) ;
#39975=CARTESIAN_POINT ( 'NONE',  ( -97.30629616937501680, 90.00000000000004263, 86.62656250086715204 ) ) ;
#39977=CARTESIAN_POINT ( 'NONE',  ( 96.15314808468748708, 88.00268892867053694, 85.40947916753380298 ) ) ;
#39978=CARTESIAN_POINT ( 'NONE',  ( -95.00000000000002842, 92.66308142843932671, 83.76906250086713612 ) ) ;
#39980=CARTESIAN_POINT ( 'NONE',  ( -95.00000000000002842, 93.05995642670504253, 87.93624999999998693 ) ) ;
#39984=CARTESIAN_POINT ( 'NONE',  ( -94.99999999999997158, -212.6630814284392557, 84.72156250086713669 ) ) ;
#39988=FACE_OUTER_BOUND ( 'NONE', #22427, .T. ) ;
#39993=CARTESIAN_POINT ( 'NONE',  ( -92.35000000000003695, 90.00000000000004263, 78.25249999999999773 ) ) ;
#40001=ORIENTED_EDGE ( 'NONE', *, *, #65710, .F. ) ;
#40002=CARTESIAN_POINT ( 'NONE',  ( -93.84685191531254134, 91.99731107132950569, 79.90614583420047268 ) ) ;
#40008=DIRECTION ( 'NONE',  ( 1.000000000000000000, 0.000000000000000000, 0.000000000000000000 ) ) ;
#40013=( BOUNDED_CURVE ( )  B_SPLINE_CURVE ( 2, ( #22342, #28338, #33233, #32498, #10315, #33613, #67835 ),
 .UNSPECIFIED., .F., .F. ) 
 B_SPLINE_CURVE_WITH_KNOTS ( ( 3, 2, 2, 3 ),
 ( 0.5000000000000000000, 0.5069444444444444198, 0.5138888888888887285, 0.5208333333333332593 ),
 .UNSPECIFIED. ) 
 CURVE ( )  GEOMETRIC_REPRESENTATION_ITEM ( )  RATIONAL_B_SPLINE_CURVE ( ( 1.000000000000000000, 0.8660254037844387076, 1.000000000000000000, 0.8660254037844387076, 1.000000000000000000, 0.8660254037844408170, 0.9999999999999978906 ) ) 
 REPRESENTATION_ITEM ( '' )  );
#40016=CARTESIAN_POINT ( 'NONE',  ( 97.30629616937498838, 90.00000000000002842, 76.14906250086716000 ) ) ;
#40017=CARTESIAN_POINT ( 'NONE',  ( -96.15314808468747287, -208.0026889286704943, 79.53572916753381605 ) ) ;
#40021=DIRECTION ( 'NONE',  ( -0.000000000000000000, -0.000000000000000000, 1.000000000000000000 ) ) ;
#40026=CARTESIAN_POINT ( 'NONE',  ( 93.84685191531251292, -211.9973110713294489, 80.22364583420046813 ) ) ;
#40033=ORIENTED_EDGE ( 'NONE', *, *, #49113, .F. ) ;
#40036=CARTESIAN_POINT ( 'NONE',  ( 93.84685191531251292, -211.9973110713294489, 75.93739583420048689 ) ) ;
#40039=CARTESIAN_POINT ( 'NONE',  ( 96.15314808468748708, 88.00268892867053694, 82.39322916753381776 ) ) ;
#40040=CARTESIAN_POINT ( 'NONE',  ( 96.32499999999998863, -212.2949673200287179, 78.78166666666666629 ) ) ;
#40045=ORIENTED_EDGE ( 'NONE', *, *, #15712, .T. ) ;
#40054=ORIENTED_EDGE ( 'NONE', *, *, #57956, .F. ) ;
#40055=CARTESIAN_POINT ( 'NONE',  ( -92.34999999999999432, -211.5299782133524502, 82.72395833506762131 ) ) ;
#40056=ORIENTED_EDGE ( 'NONE', *, *, #64317, .T. ) ;
#40060=CARTESIAN_POINT ( 'NONE',  ( 92.34999999999999432, 91.52997821335252127, 80.50145833506765314 ) ) ;
#40061=CARTESIAN_POINT ( 'NONE',  ( -95.00000000000002842, 93.05995642670501411, 78.49062500173430124 ) ) ;
#40064=CARTESIAN_POINT ( 'NONE',  ( 96.15314808468748708, 91.99731107132950569, 80.06489583420048461 ) ) ;
#40083=CARTESIAN_POINT ( 'NONE',  ( -97.30629616937497417, -211.3315407142195852, 80.32947916753381890 ) ) ;
#40093=CARTESIAN_POINT ( 'NONE',  ( 92.69370383062498320, 88.66845928578035796, 75.72572916753381378 ) ) ;
#40097=CARTESIAN_POINT ( 'NONE',  ( -92.34999999999999432, -208.4700217866474645, 76.47979166840096354 ) ) ;
#40098=LINE ( 'NONE', #11512, #51998 ) ;
#40102=CARTESIAN_POINT ( 'NONE',  ( 96.15314808468748708, 91.99731107132950569, 88.31989583420048007 ) ) ;
#40104=CARTESIAN_POINT ( 'NONE',  ( -96.15314808468747287, -208.0026889286704943, 88.42572916753381662 ) ) ;
#40108=CARTESIAN_POINT ( 'NONE',  ( -92.69370383062504004, 90.00000000000004263, 80.43531250086714124 ) ) ;
#40109=AXIS2_PLACEMENT_3D ( 'NONE', #41788, #19223, #12837 ) ;
#40118=CARTESIAN_POINT ( 'NONE',  ( 95.00000000000000000, -213.0599564267049857, 85.79312500173431033 ) ) ;
#40120=CARTESIAN_POINT ( 'NONE',  ( 92.69370383062501162, -209.9999999999999716, 75.83156250086716454 ) ) ;
#40121=ORIENTED_EDGE ( 'NONE', *, *, #1744, .F. ) ;
#40122=ORIENTED_EDGE ( 'NONE', *, *, #38464, .F. ) ;
#40123=CARTESIAN_POINT ( 'NONE',  ( 92.69370383062501162, -209.9999999999999716, 85.35656250086715602 ) ) ;
#40124=CARTESIAN_POINT ( 'NONE',  ( -94.99999999999997158, -206.9400435732949575, 81.66562500173431260 ) ) ;
#40129=CARTESIAN_POINT ( 'NONE',  ( 96.32499999999998863, -212.2949673200287179, 87.67166666666666686 ) ) ;
#40132=VERTEX_POINT ( 'NONE', #57901 ) ;
#40141=CARTESIAN_POINT ( 'NONE',  ( 92.35000000000000853, -209.9999999999999716, 77.37937500173428873 ) ) ;
#40143=CARTESIAN_POINT ( 'NONE',  ( 94.99999999999998579, 86.94004357329500010, 79.36374999999999602 ) ) ;
#40147=CARTESIAN_POINT ( 'NONE',  ( -94.99999999999997158, -206.9400435732949575, 82.93562500173430863 ) ) ;
#40150=DIRECTION ( 'NONE',  ( 0.000000000000000000, -1.000000000000000000, 0.000000000000000000 ) ) ;
#40152=CARTESIAN_POINT ( 'NONE',  ( -93.84685191531252713, 88.00268892867056536, 81.75822916753382685 ) ) ;
#40153=CARTESIAN_POINT ( 'NONE',  ( 96.15314808468748708, 91.99731107132950569, 77.36614583420046642 ) ) ;
#40154=ORIENTED_EDGE ( 'NONE', *, *, #60357, .F. ) ;
#40156=FACE_OUTER_BOUND ( 'NONE', #67999, .T. ) ;
#40162=CARTESIAN_POINT ( 'NONE',  ( -97.30629616937497417, -211.3315407142195852, 76.36072916753381890 ) ) ;
#40167=ORIENTED_EDGE ( 'NONE', *, *, #20951, .T. ) ;
#40168=CYLINDRICAL_SURFACE ( 'NONE', #44363, 2.649999999999985700 ) ;
#40172=CARTESIAN_POINT ( 'NONE',  ( -92.69370383062498320, -211.3315407142195852, 76.57239583420046358 ) ) ;
#40186=CARTESIAN_POINT ( 'NONE',  ( 97.30629616937498838, 88.66845928578035796, 84.82739583420048746 ) ) ;
#40203=CARTESIAN_POINT ( 'NONE',  ( 97.64999999954044085, 90.00004935162768049, 87.22187670868791542 ) ) ;
#40204=CARTESIAN_POINT ( 'NONE',  ( 95.00000000000000000, -209.9999999999999716, 90.00000000000000000 ) ) ;
#40208=CARTESIAN_POINT ( 'NONE',  ( 93.84685191531249870, -208.0026889286704943, 83.98072916753382344 ) ) ;
#40214=CARTESIAN_POINT ( 'NONE',  ( 95.00000000000000000, -207.3369185715606307, 79.95906250086713385 ) ) ;
#40217=CARTESIAN_POINT ( 'NONE',  ( 97.30629616937498838, -209.9999999999999716, 83.13406250086715943 ) ) ;
#40225=CARTESIAN_POINT ( 'NONE',  ( 92.35000000000009379, -208.4700217866474361, 80.42208333333330472 ) ) ;
#40229=CARTESIAN_POINT ( 'NONE',  ( 92.35000000000000853, -209.9999999999999716, 88.17437500173430465 ) ) ;
#40234=( BOUNDED_CURVE ( )  B_SPLINE_CURVE ( 2, ( #71083, #19587, #60213, #48539, #31975, #36882, #44387, #59834, #71454 ),
 .UNSPECIFIED., .F., .F. ) 
 B_SPLINE_CURVE_WITH_KNOTS ( ( 3, 2, 2, 2, 3 ),
 ( 0.08466915177892317401, 0.08466918649058879920, 0.09172495203147107423, 0.09878071757235334927, 0.1058364832022827134 ),
 .UNSPECIFIED. ) 
 CURVE ( )  GEOMETRIC_REPRESENTATION_ITEM ( )  RATIONAL_B_SPLINE_CURVE ( ( 0.9999986817990250687, 0.9999993408962699615, 1.000000000000000000, 0.8660254037844387076, 1.000000000000000000, 0.8660254037844387076, 1.000000000000000000, 0.8660254037844387076, 1.000000000000000000 ) ) 
 REPRESENTATION_ITEM ( '' )  );
#40246=CARTESIAN_POINT ( 'NONE',  ( 92.35002740377129271, 91.52999403492727026, 79.86645724064027263 ) ) ;
#40249=CARTESIAN_POINT ( 'NONE',  ( -96.32500000000001705, 92.29496732002878900, 89.25916666666667254 ) ) ;
#40251=ORIENTED_EDGE ( 'NONE', *, *, #8345, .F. ) ;
#40254=DIRECTION ( 'NONE',  ( -0.000000000000000000, -0.000000000000000000, 1.000000000000000000 ) ) ;
#40255=CARTESIAN_POINT ( 'NONE',  ( -97.30629616937497417, -211.3315407142195852, 86.52072916753381548 ) ) ;
#40260=CARTESIAN_POINT ( 'NONE',  ( -94.99999999999997158, -212.6630814284392557, 75.19656250086714522 ) ) ;
#40266=CARTESIAN_POINT ( 'NONE',  ( -97.65000000000001990, 90.00000000000004263, 84.99937500173429328 ) ) ;
#40267=CARTESIAN_POINT ( 'NONE',  ( 92.35000000000000853, -209.9999999999999716, 81.10999999999999943 ) ) ;
#40269=CARTESIAN_POINT ( 'NONE',  ( -97.30629616937501680, 88.66845928578038638, 78.90072916753381094 ) ) ;
#40276=AXIS2_PLACEMENT_3D ( 'NONE', #39558, #33907, #56850 ) ;
#40282=CARTESIAN_POINT ( 'NONE',  ( -92.69370383062498320, -208.6684592857803011, 76.20197916753382117 ) ) ;
#40283=AXIS2_PLACEMENT_3D ( 'NONE', #11146, #57015, #44627 ) ;
#40289=CARTESIAN_POINT ( 'NONE',  ( -92.35000000000003695, 90.00000000000004263, 88.41249999999999432 ) ) ;
#40315=ORIENTED_EDGE ( 'NONE', *, *, #45772, .F. ) ;
#40321=ORIENTED_EDGE ( 'NONE', *, *, #34135, .T. ) ;
#40322=CARTESIAN_POINT ( 'NONE',  ( 97.30629616937498838, 88.66845928578037217, 84.82739583420045903 ) ) ;
#40325=CARTESIAN_POINT ( 'NONE',  ( 93.84685191531251292, -211.9973110713294489, 83.39864583420047950 ) ) ;
#40327=CARTESIAN_POINT ( 'NONE',  ( -94.99999999999997158, -206.9400435732949575, 76.50624999999999432 ) ) ;
#40330=CARTESIAN_POINT ( 'NONE',  ( 93.67500000000001137, -207.7050326799711968, 79.09916666666666174 ) ) ;
#40335=CARTESIAN_POINT ( 'NONE',  ( -92.69370383062498320, -209.9999999999999716, 84.88031250086713442 ) ) ;
#40337=CARTESIAN_POINT ( 'NONE',  ( -92.69370383062502583, 88.66845928578038638, 81.81114583420048803 ) ) ;
#40338=EDGE_CURVE ( 'NONE', #23224, #47350, #45511, .T. ) ;
#40340=CARTESIAN_POINT ( 'NONE',  ( 92.69370383062498320, 91.33154071421968467, 84.50989583420046358 ) ) ;
#40341=CARTESIAN_POINT ( 'NONE',  ( -95.00000000000002842, 87.33691857156074434, 84.08656250086713158 ) ) ;
#40347=FACE_OUTER_BOUND ( 'NONE', #21072, .T. ) ;
#40348=CARTESIAN_POINT ( 'NONE',  ( -92.69370383062498320, -208.6684592857803295, 86.20322916753380582 ) ) ;
#40349=CARTESIAN_POINT ( 'NONE',  ( 97.64999999999999147, -209.9999999999999716, 82.06250000000000000 ) ) ;
#40356=CARTESIAN_POINT ( 'NONE',  ( -97.65000000000001990, 88.47002178664754979, 77.98791666666664923 ) ) ;
#40359=CARTESIAN_POINT ( 'NONE',  ( 97.64999999999999147, 90.00000000000002842, 76.34749999999999659 ) ) ;
#40364=CARTESIAN_POINT ( 'NONE',  ( -95.00000000000002842, 92.66308142843932671, 78.05406250086714692 ) ) ;
#40369=CARTESIAN_POINT ( 'NONE',  ( -97.64998576286728849, 88.47001356683513507, 75.52729223699087413 ) ) ;
#40370=CARTESIAN_POINT ( 'NONE',  ( -92.69370383062498320, -208.6684592857803011, 88.26697916753381890 ) ) ;
#40372=CARTESIAN_POINT ( 'NONE',  ( 94.99999999999998579, 87.33691857156068750, 77.26031250086714408 ) ) ;
#40374=CARTESIAN_POINT ( 'NONE',  ( -93.84685191531248449, -208.0026889286704943, 78.15989583420049769 ) ) ;
#40378=CARTESIAN_POINT ( 'NONE',  ( 97.65000000000000568, -211.5299782133524218, 78.91395833506763324 ) ) ;
#40382=CARTESIAN_POINT ( 'NONE',  ( -93.84685191531252713, 88.00268892867056536, 76.04322916753382344 ) ) ;
#40383=CARTESIAN_POINT ( 'NONE',  ( 92.69370383062501162, -209.9999999999999716, 75.67281250086713840 ) ) ;
#40390=CARTESIAN_POINT ( 'NONE',  ( -92.34999999999999432, -208.4700217866474645, 87.90979166840097037 ) ) ;
#40392=EDGE_CURVE ( 'NONE', #48178, #60576, #50988, .T. ) ;
#40395=ORIENTED_EDGE ( 'NONE', *, *, #20030, .T. ) ;
#40401=CARTESIAN_POINT ( 'NONE',  ( 92.69370383062498320, 90.00000000000002842, 84.08656250086716000 ) ) ;
#40403=CARTESIAN_POINT ( 'NONE',  ( 97.64999999999999147, -209.9999999999999716, 76.34749999999999659 ) ) ;
#40405=VERTEX_POINT ( 'NONE', #71365 ) ;
#40411=DIRECTION ( 'NONE',  ( 1.000000000000000000, 0.000000000000000000, 0.000000000000000000 ) ) ;
#40413=DIRECTION ( 'NONE',  ( 1.000000000000000000, 0.000000000000000000, 0.000000000000000000 ) ) ;
#40414=FACE_BOUND ( 'NONE', #15797, .T. ) ;
#40418=CARTESIAN_POINT ( 'NONE',  ( -97.64999999999994884, -208.4700217866474645, 79.86645833506761960 ) ) ;
#40424=CARTESIAN_POINT ( 'NONE',  ( 96.32499999999997442, 92.29496732002878900, 78.43770833506764006 ) ) ;
#40425=CARTESIAN_POINT ( 'NONE',  ( -93.67500000000003979, 87.70503267997129626, 80.76604166840097321 ) ) ;
#40428=CARTESIAN_POINT ( 'NONE',  ( 97.30629616937498838, 88.66845928578037217, 79.27114583420048177 ) ) ;
#40430=DIRECTION ( 'NONE',  ( 0.000000000000000000, -1.000000000000000000, 0.000000000000000000 ) ) ;
#40432=CARTESIAN_POINT ( 'NONE',  ( 95.00000000000000000, -213.0599564267049857, 79.44312500173430180 ) ) ;
#40433=CARTESIAN_POINT ( 'NONE',  ( 97.64999999999999147, 90.00000000000002842, 90.00000000000000000 ) ) ;
#40435=CYLINDRICAL_SURFACE ( 'NONE', #54386, 2.649999999999985700 ) ;
#40437=LINE ( 'NONE', #45737, #58802 ) ;
#40438=VERTEX_POINT ( 'NONE', #54461 ) ;
#40447=( BOUNDED_CURVE ( )  B_SPLINE_CURVE ( 2, ( #39820, #33405, #28149 ),
 .UNSPECIFIED., .F., .T. ) 
 B_SPLINE_CURVE_WITH_KNOTS ( ( 3, 3 ),
 ( 0.9791666666666669627, 0.9841647806526082620 ),
 .UNSPECIFIED. ) 
 CURVE ( )  GEOMETRIC_REPRESENTATION_ITEM ( )  RATIONAL_B_SPLINE_CURVE ( ( 0.9999999999999935607, 0.9035746763527574554, 0.9459494432169380795 ) ) 
 REPRESENTATION_ITEM ( '' )  );
#40448=CARTESIAN_POINT ( 'NONE',  ( -97.30629616937497417, -211.3315407142195852, 78.42447916753380355 ) ) ;
#40454=LINE ( 'NONE', #46104, #30917 ) ;
#40455=CARTESIAN_POINT ( 'NONE',  ( 93.84685191531248449, 91.99731107132950569, 76.20197916753380696 ) ) ;
#40456=CYLINDRICAL_SURFACE ( 'NONE', #16130, 2.649999999999985700 ) ;
#40459=CARTESIAN_POINT ( 'NONE',  ( 2.500000000000034639, 90.00000000000000000, -310.0000000000000000 ) ) ;
#40463=CARTESIAN_POINT ( 'NONE',  ( 92.69370383062498320, 88.66845928578035796, 86.04447916753382231 ) ) ;
#40465=CARTESIAN_POINT ( 'NONE',  ( 96.32499999999998863, 87.70503267997126784, 82.59166666666665435 ) ) ;
#40469=CARTESIAN_POINT ( 'NONE',  ( -95.00000000000002842, 92.66308142843932671, 78.68906250086713783 ) ) ;
#40473=ORIENTED_EDGE ( 'NONE', *, *, #18401, .T. ) ;
#40475=DIRECTION ( 'NONE',  ( 1.000000000000000000, 0.000000000000000000, 0.000000000000000000 ) ) ;
#40481=CARTESIAN_POINT ( 'NONE',  ( 97.30629616937498838, -208.6684592857803011, 75.56697916753383026 ) ) ;
#40485=AXIS2_PLACEMENT_3D ( 'NONE', #16328, #33232, #40008 ) ;
#40487=CARTESIAN_POINT ( 'NONE',  ( 92.69370383062501162, -209.9999999999999716, 82.81656250086714977 ) ) ;
#40495=CARTESIAN_POINT ( 'NONE',  ( 92.35000000000002274, -211.5299782133524502, 84.97291666666666288 ) ) ;
#40497=ORIENTED_EDGE ( 'NONE', *, *, #24116, .F. ) ;
#40498=VERTEX_POINT ( 'NONE', #20239 ) ;
#40502=CARTESIAN_POINT ( 'NONE',  ( -97.30629616937501680, 90.00000000000004263, 85.99156250086716113 ) ) ;
#40504=DIRECTION ( 'NONE',  ( 1.000000000000000000, 0.000000000000000000, 0.000000000000000000 ) ) ;
#40505=CARTESIAN_POINT ( 'NONE',  ( 92.35000000000002274, -208.4700217866474645, 75.42145833506764063 ) ) ;
#40506=CARTESIAN_POINT ( 'NONE',  ( 93.67499999999998295, 92.29496732002878900, 77.82916666666665151 ) ) ;
#40512=CARTESIAN_POINT ( 'NONE',  ( -97.64999999999996305, -209.9999999999999716, 83.09437500173430635 ) ) ;
#40514=ORIENTED_EDGE ( 'NONE', *, *, #6046, .F. ) ;
#40515=CARTESIAN_POINT ( 'NONE',  ( -92.35000000000003695, 90.00000000000004263, 88.49187500173430010 ) ) ;
#40516=CARTESIAN_POINT ( 'NONE',  ( -96.15314808468752972, 91.99731107132950569, 81.44072916753381719 ) ) ;
#40517=CARTESIAN_POINT ( 'NONE',  ( 94.99999999999998579, 87.33691857156068750, 88.69031250086716511 ) ) ;
#40521=CARTESIAN_POINT ( 'NONE',  ( 97.64997490602121388, 88.47000729863215440, 89.07395733288670669 ) ) ;
#40523=ORIENTED_EDGE ( 'NONE', *, *, #51009, .F. ) ;
#40525=CARTESIAN_POINT ( 'NONE',  ( -97.30629616937495996, -209.9999999999999716, 78.84781250086714977 ) ) ;
#40526=EDGE_LOOP ( 'NONE', ( #11429, #67579, #5494, #6760 ) ) ;
#40531=CARTESIAN_POINT ( 'NONE',  ( 97.64999999999999147, 90.00000000000002842, 80.79249999999998977 ) ) ;
#40532=ORIENTED_EDGE ( 'NONE', *, *, #17302, .F. ) ;
#40533=CARTESIAN_POINT ( 'NONE',  ( -92.69370383062498320, -209.9999999999999716, 75.99031250086714806 ) ) ;
#40545=CARTESIAN_POINT ( 'NONE',  ( 97.30629616937498838, 91.33154071421968467, 84.93322916753379559 ) ) ;
#40548=CARTESIAN_POINT ( 'NONE',  ( -92.34999999999995168, 88.47002178664756400, 75.65958333333333030 ) ) ;
#40550=CARTESIAN_POINT ( 'NONE',  ( 97.64999999999999147, -209.9999999999999716, 88.41249999999999432 ) ) ;
#40555=CARTESIAN_POINT ( 'NONE',  ( 92.35000000000005116, 88.47002178664747873, 78.62291666666668277 ) ) ;
#40562=VECTOR ( 'NONE', #57408, 1000.000000000000000 ) ;
#40563=B_SPLINE_CURVE_WITH_KNOTS ( 'NONE', 1,
 ( #60435, #36368 ),
 .UNSPECIFIED., .F., .F.,
 ( 2, 2 ),
 ( 0.000000000000000000, 1.000000000000000000 ),
 .UNSPECIFIED. ) ;
#40567=ORIENTED_EDGE ( 'NONE', *, *, #60062, .F. ) ;
#40575=CARTESIAN_POINT ( 'NONE',  ( 95.00000000000000000, -212.6630814284392557, 84.24531250086715772 ) ) ;
#40581=CARTESIAN_POINT ( 'NONE',  ( -97.64997259622820991, -208.4700059650725450, 79.86645724064025842 ) ) ;
#40582=CARTESIAN_POINT ( 'NONE',  ( 97.30629616937498838, -208.6684592857803295, 76.04322916753380923 ) ) ;
#40587=CARTESIAN_POINT ( 'NONE',  ( 97.30629616937498838, -208.6684592857803011, 81.91697916753381037 ) ) ;
#40592=ORIENTED_EDGE ( 'NONE', *, *, #35560, .F. ) ;
#40594=EDGE_CURVE ( 'NONE', #56929, #45497, #6846, .T. ) ;
#40598=CARTESIAN_POINT ( 'NONE',  ( 97.64999999999999147, -209.9999999999999716, 90.00000000000000000 ) ) ;
#40602=CARTESIAN_POINT ( 'NONE',  ( 97.64999999999999147, -209.9999999999999716, 85.95187500173430806 ) ) ;
#40603=ORIENTED_EDGE ( 'NONE', *, *, #3502, .F. ) ;
#40615=AXIS2_PLACEMENT_3D ( 'NONE', #49636, #61680, #14695 ) ;
#40619=CARTESIAN_POINT ( 'NONE',  ( 97.65000000000004832, -211.5299782133523934, 76.29458333333333542 ) ) ;
#40623=CARTESIAN_POINT ( 'NONE',  ( -92.35000000000005116, 91.52997821335253548, 87.83041666666666458 ) ) ;
#40625=CARTESIAN_POINT ( 'NONE',  ( 96.66078690017486963, 88.39975348990186887, 74.64190636928353229 ) ) ;
#40626=MECHANICAL_DESIGN_GEOMETRIC_PRESENTATION_REPRESENTATION('',(#56244),#7011);
#40628=DIRECTION ( 'NONE',  ( -0.000000000000000000, -0.000000000000000000, 1.000000000000000000 ) ) ;
#40629=CARTESIAN_POINT ( 'NONE',  ( -96.15314808468747287, -208.0026889286704943, 86.99697916753380866 ) ) ;
#40631=CARTESIAN_POINT ( 'NONE',  ( -97.64999999999996305, -211.5299782133524218, 79.33729166840096525 ) ) ;
#40634=CARTESIAN_POINT ( 'NONE',  ( -97.30629616937495996, -209.9999999999999716, 77.57781250086713953 ) ) ;
#40635=CARTESIAN_POINT ( 'NONE',  ( 97.64999999999999147, 90.00000000000002842, 90.00000000000000000 ) ) ;
#40640=CARTESIAN_POINT ( 'NONE',  ( -92.69370383062502583, 91.33154071421968467, 77.94822916753381037 ) ) ;
#40649=CARTESIAN_POINT ( 'NONE',  ( 93.67500000000001137, -207.7050326799711968, 89.33854166840096411 ) ) ;
#40656=CARTESIAN_POINT ( 'NONE',  ( -92.69370383062498320, -211.3315407142195852, 76.73114583420048973 ) ) ;
#40658=EDGE_CURVE ( 'NONE', #48987, #16386, #11929, .T. ) ;
#40659=ADVANCED_FACE ( 'NONE', ( #17212 ), #62731, .F. ) ;
#40677=( BOUNDED_CURVE ( )  B_SPLINE_CURVE ( 2, ( #64681, #48496, #60531, #48855, #18799, #3038, #3396 ),
 .UNSPECIFIED., .F., .F. ) 
 B_SPLINE_CURVE_WITH_KNOTS ( ( 3, 2, 2, 3 ),
 ( 0.1693384224428226559, 0.1763941385229248482, 0.1834499040638421785, 0.1905056698846566698 ),
 .UNSPECIFIED. ) 
 CURVE ( )  GEOMETRIC_REPRESENTATION_ITEM ( )  RATIONAL_B_SPLINE_CURVE ( ( 0.9999981216931748129, 0.8660263429444348127, 1.000000000000000000, 0.8660254037844387076, 1.000000000000000000, 0.8660254037844387076, 1.000000000000000000 ) ) 
 REPRESENTATION_ITEM ( '' )  );
#40678=CARTESIAN_POINT ( 'NONE',  ( 95.00000000000000000, -207.3369185715606307, 85.03906250086714635 ) ) ;
#40685=EDGE_CURVE ( 'NONE', #5670, #30842, #55368, .T. ) ;
#40687=CARTESIAN_POINT ( 'NONE',  ( -96.15314808468751551, 88.00268892867056536, 81.65239583420049030 ) ) ;
#40694=EDGE_LOOP ( 'NONE', ( #27737, #20230, #30577, #43134 ) ) ;
#40701=CARTESIAN_POINT ( 'NONE',  ( 92.69370383062498320, 88.66845928578037217, 85.25072916753379104 ) ) ;
#40703=CARTESIAN_POINT ( 'NONE',  ( 96.15314808468750130, -211.9973110713294489, 83.50447916753381605 ) ) ;
#40712=CARTESIAN_POINT ( 'NONE',  ( -97.30629616937497417, -211.3315407142195852, 82.71072916753379900 ) ) ;
#40713=CARTESIAN_POINT ( 'NONE',  ( -93.84685191531252713, 88.00268892867056536, 81.12322916753382174 ) ) ;
#40715=CARTESIAN_POINT ( 'NONE',  ( 94.99999999999998579, 87.33691857156068750, 84.08656250086713158 ) ) ;
#40719=DIRECTION ( 'NONE',  ( 1.000000000000000000, 0.000000000000000000, 0.000000000000000000 ) ) ;
#40722=CARTESIAN_POINT ( 'NONE',  ( -96.15314808468747287, -208.0026889286704943, 85.72697916753379843 ) ) ;
#40730=ORIENTED_EDGE ( 'NONE', *, *, #24363, .F. ) ;
#40733=CARTESIAN_POINT ( 'NONE',  ( -92.35000000000005116, 91.52997821335253548, 78.30541666666668732 ) ) ;
#40736=CARTESIAN_POINT ( 'NONE',  ( -92.35000000000005116, 91.52997821335253548, 79.65479166840096070 ) ) ;
#40742=CARTESIAN_POINT ( 'NONE',  ( -92.69370383062504004, 90.00000000000004263, 77.89531250086714920 ) ) ;
#40751=CARTESIAN_POINT ( 'NONE',  ( -92.69370383062498320, -208.6684592857803011, 86.36197916753383197 ) ) ;
#40752=EDGE_CURVE ( 'NONE', #70258, #5237, #7031, .T. ) ;
#40754=ADVANCED_FACE ( 'NONE', ( #42000 ), #61085, .F. ) ;
#40755=CARTESIAN_POINT ( 'NONE',  ( 94.99999999999998579, 92.66308142843932671, 75.67281250086715261 ) ) ;
#40756=VECTOR ( 'NONE', #16265, 1000.000000000000000 ) ;
#40758=CARTESIAN_POINT ( 'NONE',  ( -94.99999999999997158, -212.6630814284392557, 77.26031250086714408 ) ) ;
#40761=CARTESIAN_POINT ( 'NONE',  ( -93.67500000000003979, 92.29496732002878900, 82.88270833506763324 ) ) ;
#40764=CARTESIAN_POINT ( 'NONE',  ( -95.00000000000002842, 90.00000000000004263, 75.00000000000000000 ) ) ;
#40767=CARTESIAN_POINT ( 'NONE',  ( 96.15314808468748708, -208.0026889286704943, 78.63614583420047666 ) ) ;
#40769=ORIENTED_EDGE ( 'NONE', *, *, #40825, .T. ) ;
#40772=ORIENTED_EDGE ( 'NONE', *, *, #54841, .F. ) ;
#40777=CIRCLE ( 'NONE', #57581, 12.75000000000000000 ) ;
#40782=VERTEX_POINT ( 'NONE', #53286 ) ;
#40786=CARTESIAN_POINT ( 'NONE',  ( -93.67499999999998295, -212.2949673200287179, 77.51166666666665606 ) ) ;
#40789=CARTESIAN_POINT ( 'NONE',  ( 96.15314808468748708, 91.99731107132950569, 84.50989583420049200 ) ) ;
#40790=CYLINDRICAL_SURFACE ( 'NONE', #44059, 23.50000000000000355 ) ;
#40805=CARTESIAN_POINT ( 'NONE',  ( -94.99999999999997158, -206.9400435732949575, 79.12562500173429214 ) ) ;
#40809=CARTESIAN_POINT ( 'NONE',  ( 92.34999999999999432, 88.47002178664753558, 78.70229166840096013 ) ) ;
#40810=CARTESIAN_POINT ( 'NONE',  ( -96.32500000000001705, 92.29496732002878900, 78.54354166840096241 ) ) ;
#40812=CARTESIAN_POINT ( 'NONE',  ( 93.84685191531248449, 88.00268892867053694, 81.01739583420049939 ) ) ;
#40816=CARTESIAN_POINT ( 'NONE',  ( -95.00000000000002842, 93.05995642670504253, 86.74562500173429669 ) ) ;
#40820=CARTESIAN_POINT ( 'NONE',  ( 97.64999999999999147, -209.9999999999999716, 76.98250000000000171 ) ) ;
#40825=EDGE_CURVE ( 'NONE', #7101, #41677, #29891, .T. ) ;
#40831=CARTESIAN_POINT ( 'NONE',  ( -92.69370383062498320, -208.6684592857803011, 79.37697916753381833 ) ) ;
#40835=FACE_OUTER_BOUND ( 'NONE', #21055, .T. ) ;
#40838=AXIS2_PLACEMENT_3D ( 'NONE', #29510, #30621, #24267 ) ;
#40842=DIRECTION ( 'NONE',  ( -0.000000000000000000, -0.000000000000000000, 1.000000000000000000 ) ) ;
#40847=CARTESIAN_POINT ( 'NONE',  ( -97.64999999999996305, -211.5299782133524218, 85.05229166840096866 ) ) ;
#40851=CARTESIAN_POINT ( 'NONE',  ( 92.69370383062498320, 88.66845928578035796, 88.58447916753382856 ) ) ;
#40856=CARTESIAN_POINT ( 'NONE',  ( -95.00000000000002842, 92.66308142843932671, 75.51406250086714067 ) ) ;
#40857=CARTESIAN_POINT ( 'NONE',  ( 93.84685191531249870, -208.0026889286704943, 87.63197916753379957 ) ) ;
#40858=EDGE_CURVE ( 'NONE', #57250, #62567, #26182, .T. ) ;
#40860=ORIENTED_EDGE ( 'NONE', *, *, #948, .F. ) ;
#40870=EDGE_LOOP ( 'NONE', ( #12919, #21992, #31974, #57424, #1871 ) ) ;
#40871=CARTESIAN_POINT ( 'NONE',  ( 97.30629616937498838, -208.6684592857803295, 83.18697916753382060 ) ) ;
#40873=LINE ( 'NONE', #52885, #12409 ) ;
#40877=CARTESIAN_POINT ( 'NONE',  ( 97.64999999999997726, -208.4700217866474645, 84.02041666666667652 ) ) ;
#40882=EDGE_LOOP ( 'NONE', ( #23114, #61661, #47061, #13764 ) ) ;
#40884=CARTESIAN_POINT ( 'NONE',  ( -96.15314808468751551, 88.00268892867056536, 86.73239583420048859 ) ) ;
#40888=CARTESIAN_POINT ( 'NONE',  ( 97.64999999999997726, -211.5299782133524502, 77.64395833506762301 ) ) ;
#40889=CARTESIAN_POINT ( 'NONE',  ( 97.64999999999999147, 90.00000000000002842, 78.88750000000000284 ) ) ;
#40891=CARTESIAN_POINT ( 'NONE',  ( -93.67499999999998295, -212.2949673200287179, 88.38604166840097776 ) ) ;
#40893=VERTEX_POINT ( 'NONE', #55881 ) ;
#40896=CARTESIAN_POINT ( 'NONE',  ( -96.32500000000001705, 92.29496732002878900, 88.70354166840097321 ) ) ;
#40897=( BOUNDED_CURVE ( )  B_SPLINE_CURVE ( 2, ( #47565, #22897, #35536 ),
 .UNSPECIFIED., .F., .F. ) 
 B_SPLINE_CURVE_WITH_KNOTS ( ( 3, 3 ),
 ( 0.000000000000000000, 2.334341054553106638E-05 ),
 .UNSPECIFIED. ) 
 CURVE ( )  GEOMETRIC_REPRESENTATION_ITEM ( )  RATIONAL_B_SPLINE_CURVE ( ( 0.9459494467533928752, 0.9464399322879002430, 0.9469490141588231547 ) ) 
 REPRESENTATION_ITEM ( '' )  );
#40898=CARTESIAN_POINT ( 'NONE',  ( -97.30629616937501680, 90.00000000000004263, 82.81656250086714977 ) ) ;
#40899=CARTESIAN_POINT ( 'NONE',  ( 97.30629616937498838, 91.33154071421968467, 75.40822916753381833 ) ) ;
#40903=CARTESIAN_POINT ( 'NONE',  ( 95.00000000000000000, -209.9999999999999716, 90.00000000000000000 ) ) ;
#40904=CARTESIAN_POINT ( 'NONE',  ( -93.67499999999998295, -207.7050326799711968, 86.05770833506763040 ) ) ;
#40907=CARTESIAN_POINT ( 'NONE',  ( -92.69370383062498320, -211.3315407142195852, 77.20739583420046870 ) ) ;
#40912=ADVANCED_FACE ( 'NONE', ( #60786 ), #26558, .F. ) ;
#40917=CARTESIAN_POINT ( 'NONE',  ( -93.84685191531247028, -211.9973110713294489, 89.37822916753381719 ) ) ;
#40919=CARTESIAN_POINT ( 'NONE',  ( -94.99999999999997158, -206.9400435732949575, 81.58624999999999261 ) ) ;
#40921=ORIENTED_EDGE ( 'NONE', *, *, #791, .F. ) ;
#40929=CARTESIAN_POINT ( 'NONE',  ( 92.69370383062498320, 88.66845928578035796, 85.88572916753381037 ) ) ;
#40937=EDGE_CURVE ( 'NONE', #18134, #46588, #20920, .T. ) ;
#40941=CARTESIAN_POINT ( 'NONE',  ( -97.30629616937501680, 88.66845928578038638, 89.06072916753382174 ) ) ;
#40942=VECTOR ( 'NONE', #58462, 1000.000000000000000 ) ;
#40953=CARTESIAN_POINT ( 'NONE',  ( 92.35000000046504454, -210.0000309987310061, 83.09538598081256566 ) ) ;
#40955=CARTESIAN_POINT ( 'NONE',  ( -95.00000000000002842, 86.94004357329504273, 77.53812500173428646 ) ) ;
#40957=CARTESIAN_POINT ( 'NONE',  ( 97.30629616937498838, -209.9999999999999716, 85.03906250086714635 ) ) ;
#40963=CARTESIAN_POINT ( 'NONE',  ( 97.30629616937498838, -211.3315407142195852, 76.57239583420046358 ) ) ;
#40965=CARTESIAN_POINT ( 'NONE',  ( 92.69370383062501162, -211.3315407142195852, 79.05947916753382287 ) ) ;
#40966=AXIS2_PLACEMENT_3D ( 'NONE', #41180, #40430, #29503 ) ;
#40972=CARTESIAN_POINT ( 'NONE',  ( 92.35000000003287823, -209.9999916080746516, 86.90410584365268676 ) ) ;
#40975=ORIENTED_EDGE ( 'NONE', *, *, #26965, .T. ) ;
#40977=CARTESIAN_POINT ( 'NONE',  ( 92.35000000000000853, -209.9999999999999716, 85.63437500173431260 ) ) ;
#40978=CARTESIAN_POINT ( 'NONE',  ( 94.26574316504957096, 85.91408486779583598, 74.64692065633562379 ) ) ;
#40986=CARTESIAN_POINT ( 'NONE',  ( 93.67499999999998295, 92.29496732002878900, 84.89354166840095672 ) ) ;
#41001=CARTESIAN_POINT ( 'NONE',  ( -95.00000000000002842, 86.94004357329504273, 88.25374999999999659 ) ) ;
#41004=ORIENTED_EDGE ( 'NONE', *, *, #40594, .T. ) ;
#41005=DIRECTION ( 'NONE',  ( -0.000000000000000000, -0.000000000000000000, 1.000000000000000000 ) ) ;
#41006=CARTESIAN_POINT ( 'NONE',  ( -92.69370383062498320, -209.9999999999999716, 81.70531250086713726 ) ) ;
#41010=CARTESIAN_POINT ( 'NONE',  ( 97.65000000000000568, -208.4700217866474645, 87.83041666666669300 ) ) ;
#41011=CARTESIAN_POINT ( 'NONE',  ( -93.84685191531247028, -211.9973110713294489, 77.78947916753381264 ) ) ;
#41013=DIRECTION ( 'NONE',  ( -0.000000000000000000, -0.000000000000000000, 1.000000000000000000 ) ) ;
#41016=CARTESIAN_POINT ( 'NONE',  ( 95.00000000000000000, -209.9999999999999716, 90.00000000000000000 ) ) ;
#41019=CARTESIAN_POINT ( 'NONE',  ( -93.84685191531254134, 91.99731107132950569, 78.00114583420048575 ) ) ;
#41032=FACE_OUTER_BOUND ( 'NONE', #47551, .T. ) ;
#41036=CARTESIAN_POINT ( 'NONE',  ( -94.99999999999997158, -207.3369185715606307, 76.30781250086715772 ) ) ;
#41041=CARTESIAN_POINT ( 'NONE',  ( 90.00000000000001421, -204.9999999999999716, 90.00000000000000000 ) ) ;
#41051=CARTESIAN_POINT ( 'NONE',  ( 92.69370383062501162, -211.3315407142195852, 84.61572916753380014 ) ) ;
#41057=ORIENTED_EDGE ( 'NONE', *, *, #27490, .F. ) ;
#41058=CARTESIAN_POINT ( 'NONE',  ( -97.30629616937501680, 90.00000000000004263, 79.00656250086716170 ) ) ;
#41065=ORIENTED_EDGE ( 'NONE', *, *, #61962, .F. ) ;
#41069=CARTESIAN_POINT ( 'NONE',  ( 92.35000000000000853, -209.9999999999999716, 80.55437500173430010 ) ) ;
#41071=EDGE_CURVE ( 'NONE', #48479, #27645, #50601, .T. ) ;
#41072=VECTOR ( 'NONE', #30075, 1000.000000000000000 ) ;
#41076=CARTESIAN_POINT ( 'NONE',  ( 97.30629616937498838, -209.9999999999999716, 81.07031250086714635 ) ) ;
#41078=CARTESIAN_POINT ( 'NONE',  ( -97.65000000000003411, -208.4700217866475214, 76.61208333333333087 ) ) ;
#41086=CARTESIAN_POINT ( 'NONE',  ( 97.64999999999999147, -209.9999999999999716, 76.34749999999999659 ) ) ;
#41087=CARTESIAN_POINT ( 'NONE',  ( -97.30629616937497417, -208.6684592857803011, 83.87489583420047268 ) ) ;
#41088=CARTESIAN_POINT ( 'NONE',  ( -97.30629616937501680, 91.33154071421968467, 81.49364583420047836 ) ) ;
#41090=CARTESIAN_POINT ( 'NONE',  ( 92.69370383062498320, 91.33154071421968467, 85.14489583420048291 ) ) ;
#41092=EDGE_CURVE ( 'NONE', #41316, #44409, #37179, .T. ) ;
#41099=CARTESIAN_POINT ( 'NONE',  ( -97.30629616937497417, -208.6684592857803295, 85.14489583420045449 ) ) ;
#41107=CARTESIAN_POINT ( 'NONE',  ( -93.67500000000003979, 92.29496732002878900, 78.35833333333333428 ) ) ;
#41109=CARTESIAN_POINT ( 'NONE',  ( -95.00000000000002842, 92.66308142843932671, 86.94406250086714749 ) ) ;
#41110=CARTESIAN_POINT ( 'NONE',  ( 92.34999999999993747, -208.4700217866474929, 81.05708333333332405 ) ) ;
#41115=CARTESIAN_POINT ( 'NONE',  ( -93.84685191531254134, 91.99731107132950569, 79.27114583420046756 ) ) ;
#41122=CARTESIAN_POINT ( 'NONE',  ( -92.35000000000005116, 88.47002178664754979, 75.73895833506765030 ) ) ;
#41123=CARTESIAN_POINT ( 'NONE',  ( -92.69370383062498320, -208.6684592857803011, 87.63197916753382799 ) ) ;
#41126=EDGE_CURVE ( 'NONE', #33969, #60251, #40437, .T. ) ;
#41127=( BOUNDED_SURFACE ( )  B_SPLINE_SURFACE ( 1, 2, ( 
 ( #39270, #62587, #15955, #56572, #73832, #17077, #5072, #27971, #4328, #21589, #68955, #57298, #5809, #68591, #16330, #28339, #4701, #28716, #51657, #23096, #38895, #50907, #68210, #17443, #16704, #27218, #39644, #50150, #51275, #40370, #11781, #21966, #34730, #10316, #27607, #73460, #41849, #13637, #65166, #18542, #12162, #41123, #70396, #47853, #18179, #1310, #563, #64421, #58032, #41480, #19282, #57678, #53134, #12896, #13276, #18904, #64058, #42236, #7637, #47133, #23456, #35825, #64793, #12532, #2039, #40751, #7277, #36206, #47496, #30556, #30191, #6182, #24202, #29080, #52383, #35469, #59147, #70038, #1672, #24561, #58779, #6538, #53505, #46386, #35105, #24925, #70779, #69313, #17799, #69683, #52013, #63693, #29441, #933, #23820, #46760, #58399, #6897, #29815, #52767, #36570, #26403, #49688, #8752, #32402, #14003, #72614, #60633, #72259, #9113, #31667, #30925, #15117, #71515, #20402, #25307, #20013, #54612, #49332, #42971, #65907, #59521, #53868, #3867, #43713, #20759, #54972, #48602, #43355, #36948, #38056, #9478, #55345, #48235, #14385, #37333, #3496, #60271, #8006, #3136, #2415, #14747, #66636, #26028, #54254, #60985, #71143, #26761, #48954, #21122, #66990, #44070, #71884, #65533, #66275, #19647, #42593, #37701, #32032, #59896, #8381, #31299, #2779, #25667, #45940, #10972, #22251, #45571, #51183, #21875, #51561, #39925, #4981, #55717, #73735, #74114, #44818, #34263, #72986, #39547, #22625, #5349, #62873, #62494, #112, #33514, #61369, #10220, #67744, #28246, #27884, #33900, #56841, #45194, #15870, #68494, #4233, #44450, #16986, #11331, #27126, #50058, #27510, #73366, #38799, #21490, #10587, #15490, #23004, #57211, #33143, #67366, #38429, #56476, #61738, #68113, #5716, #56088, #28619, #9854, #32769, #39175, #4608, #62106, #50444, #50806, #16234, #16604, #11690, #57948, #6449, #30463, #12440, #35383, #57587, #13184, #41391, #69951, #52668, #472, #1220, #23726, #844, #53412, #46662, #58683, #53046, #40656, #52298, #69593, #18094, #23369, #46298, #30098, #1950, #41036, #63603, #40282, #6806, #36116, #29355, #69228, #63969, #35732, #58312, #68864, #35016, #6091, #29719, #64330, #41752, #24114, #47040, #34635, #59060, #24834, #47405, #7553, #51927, #17349, #18450, #7183, #12806, #1583, #64696, #24470, #70308 ),
 ( #63230, #28993, #18812, #17714, #12076, #55258, #8665, #2319, #31211, #60543, #37968, #8284, #65807, #65076, #54522, #48144, #31576, #9387, #3777, #43265, #3049, #3409, #9023, #54162, #32313, #72168, #37242, #13550, #25940, #31945, #2693, #66549, #30832, #71790, #54885, #37612, #20674, #20301, #47761, #14292, #19193, #42503, #25576, #26310, #60183, #66183, #14659, #48872, #71056, #49242, #36478, #60903, #43627, #42880, #71420, #15026, #19558, #70679, #25217, #42144, #59424, #7914, #53773, #19922, #48508, #65446, #13908, #36853, #59801, #49973, #55631, #16517, #33812, #44356, #44735, #57125, #72892, #50723, #27415, #21397, #67283, #51100, #73651, #73281, #22165, #5266, #15395, #33052, #45105, #55996, #27798, #38715, #62023, #43985, #15777, #4519, #26675, #39462, #4902, #10888, #72530, #68028, #50354, #62408, #21784, #21035, #16150, #74025, #27039, #66906, #61648, #10133, #62788, #67658, #39089, #38339, #45482, #56761, #28167, #10501, #32680, #33425, #56386, #22540, #11252, #68410, #16903, #39836, #34183, #49604, #61278, #9764, #4146, #35566, #42331, #65632, #58881, #1407, #52481, #19007, #25405, #70136, #58496, #18636, #47965, #24658, #5632, #47226, #69777, #53235, #2138, #53979, #12995, #70493, #46865, #48331, #14103, #59620, #71240, #64153, #37053, #35933, #19381, #41576, #64517, #2523, #7374, #8103, #1771, #29916, #41959, #42694, #30291, #31026, #47589, #28529, #65264, #23925, #18278, #12628, #30653, #13737, #70881, #19745, #53599, #1032, #64896, #41215, #24299, #13372, #36674, #36303, #25022, #6992, #59246, #52868, #7738, #48695, #14483, #21220, #15599, #71619, #25766, #71991, #43457, #8852, #20116, #55076, #60000, #67473, #67097, #3238, #43077, #44553, #26507, #66009, #66735, #3969, #26128, #38535, #37437, #61094, #60368, #31766, #32873, #31400, #15224, #4335, #61473, #8484, #49794, #73095, #32131, #55822, #54709, #21599, #9591, #44173, #32510, #3608, #54349, #9951, #20504, #43818, #49064, #66375, #49437, #72715, #14856, #37802, #2873, #60734, #27229, #50162, #15964, #26868, #9212, #38155, #72364, #20861, #55452, #34744, #27617, #73840, #45301, #57308, #16715, #61841, #5453, #10324, #17087, #51664, #56945, #56581, #28725, #33241, #57687, #68220, #23105, #69321, #46394, #74219, #67846, #22352, #211, #29087, #39653 ) ),
 .UNSPECIFIED., .F., .F., .F. ) 
 B_SPLINE_SURFACE_WITH_KNOTS ( ( 2, 2 ),
 ( 3, 2, 2, 2, 2, 2, 2, 2, 2, 2, 2, 2, 2, 2, 2, 2, 2, 2, 2, 2, 2, 2, 2, 2, 2, 2, 2, 2, 2, 2, 2, 2, 2, 2, 2, 2, 2, 2, 2, 2, 2, 2, 2, 2, 2, 2, 2, 2, 2, 2, 2, 2, 2, 2, 2, 2, 2, 2, 2, 2, 2, 2, 2, 2, 2, 2, 2, 2, 2, 2, 2, 2, 2, 2, 2, 2, 2, 2, 2, 2, 2, 2, 2, 2, 2, 2, 2, 2, 2, 2, 2, 2, 2, 2, 2, 2, 2, 2, 2, 2, 2, 2, 2, 2, 2, 2, 2, 2, 2, 2, 2, 2, 2, 2, 2, 2, 2, 2, 2, 2, 2, 2, 2, 2, 2, 2, 2, 2, 2, 2, 2, 2, 2, 2, 2, 2, 2, 2, 2, 2, 2, 2, 2, 3 ),
 ( 0.000000000000000000, 1.000000000000000000 ),
 ( 0.000000000000000000, 0.006944444444444444059, 0.01388888888888888812, 0.02083333333333333218, 0.02777777777777777624, 0.03472222222222222376, 0.04166666666666666435, 0.04861111111111111188, 0.05555555555555555247, 0.06250000000000000000, 0.06944444444444444753, 0.07638888888888889506, 0.08333333333333332871, 0.09027777777777777624, 0.09722222222222222376, 0.1041666666666666713, 0.1111111111111111049, 0.1180555555555555525, 0.1250000000000000000, 0.1319444444444444475, 0.1388888888888888951, 0.1458333333333333426, 0.1527777777777777901, 0.1597222222222222099, 0.1666666666666666574, 0.1736111111111111049, 0.1805555555555555525, 0.1875000000000000000, 0.1944444444444444475, 0.2013888888888888951, 0.2083333333333333426, 0.2152777777777777901, 0.2222222222222222099, 0.2291666666666666574, 0.2361111111111111049, 0.2430555555555555525, 0.2500000000000000000, 0.2569444444444444198, 0.2638888888888888951, 0.2708333333333333148, 0.2777777777777777901, 0.2847222222222222099, 0.2916666666666666852, 0.2986111111111111049, 0.3055555555555555802, 0.3125000000000000000, 0.3194444444444444198, 0.3263888888888888951, 0.3333333333333333148, 0.3402777777777777901, 0.3472222222222222099, 0.3541666666666666852, 0.3611111111111111049, 0.3680555555555555802, 0.3750000000000000000, 0.3819444444444444198, 0.3888888888888888951, 0.3958333333333333148, 0.4027777777777777901, 0.4097222222222222099, 0.4166666666666666852, 0.4236111111111111049, 0.4305555555555555802, 0.4375000000000000000, 0.4444444444444444198, 0.4513888888888888951, 0.4583333333333333148, 0.4652777777777777901, 0.4722222222222222099, 0.4791666666666666852, 0.4861111111111111049, 0.4930555555555555802, 0.5000000000000000000, 0.5069444444444444198, 0.5138888888888888395, 0.5208333333333333703, 0.5277777777777777901, 0.5347222222222222099, 0.5416666666666666297, 0.5486111111111111605, 0.5555555555555555802, 0.5625000000000000000, 0.5694444444444444198, 0.5763888888888888395, 0.5833333333333333703, 0.5902777777777777901, 0.5972222222222222099, 0.6041666666666666297, 0.6111111111111111605, 0.6180555555555555802, 0.6250000000000000000, 0.6319444444444444198, 0.6388888888888888395, 0.6458333333333333703, 0.6527777777777777901, 0.6597222222222222099, 0.6666666666666666297, 0.6736111111111111605, 0.6805555555555555802, 0.6875000000000000000, 0.6944444444444444198, 0.7013888888888888395, 0.7083333333333333703, 0.7152777777777777901, 0.7222222222222222099, 0.7291666666666666297, 0.7361111111111111605, 0.7430555555555555802, 0.7500000000000000000, 0.7569444444444444198, 0.7638888888888888395, 0.7708333333333333703, 0.7777777777777777901, 0.7847222222222222099, 0.7916666666666666297, 0.7986111111111111605, 0.8055555555555555802, 0.8125000000000000000, 0.8194444444444444198, 0.8263888888888888395, 0.8333333333333333703, 0.8402777777777777901, 0.8472222222222222099, 0.8541666666666666297, 0.8611111111111111605, 0.8680555555555555802, 0.8750000000000000000, 0.8819444444444444198, 0.8888888888888888395, 0.8958333333333333703, 0.9027777777777777901, 0.9097222222222222099, 0.9166666666666666297, 0.9236111111111111605, 0.9305555555555555802, 0.9375000000000000000, 0.9444444444444444198, 0.9513888888888888395, 0.9583333333333333703, 0.9652777777777777901, 0.9722222222222222099, 0.9791666666666666297, 0.9842226772312641092, 0.9940649040035767214 ),
 .UNSPECIFIED. ) 
 GEOMETRIC_REPRESENTATION_ITEM ( )  RATIONAL_B_SPLINE_SURFACE ( (
 ( 1.000000000000000000, 0.8660254037844387076, 1.000000000000000000, 0.8660254037844387076, 1.000000000000000000, 0.8660254037844387076, 1.000000000000000000, 0.8660254037844387076, 1.000000000000000000, 0.8660254037844387076, 1.000000000000000000, 0.8660254037844387076, 1.000000000000000000, 0.8660254037844387076, 1.000000000000000000, 0.8660254037844387076, 1.000000000000000000, 0.8660254037844387076, 1.000000000000000000, 0.8660254037844387076, 1.000000000000000000, 0.8660254037844387076, 1.000000000000000000, 0.8660254037844387076, 1.000000000000000000, 0.8660254037844387076, 1.000000000000000000, 0.8660254037844387076, 1.000000000000000000, 0.8660254037844387076, 1.000000000000000000, 0.8660254037844387076, 1.000000000000000000, 0.8660254037844387076, 1.000000000000000000, 0.8660254037844387076, 1.000000000000000000, 0.8660254037844387076, 1.000000000000000000, 0.8660254037844387076, 1.000000000000000000, 0.8660254037844387076, 1.000000000000000000, 0.8660254037844387076, 1.000000000000000000, 0.8660254037844387076, 1.000000000000000000, 0.8660254037844387076, 1.000000000000000000, 0.8660254037844387076, 1.000000000000000000, 0.8660254037844387076, 1.000000000000000000, 0.8660254037844387076, 1.000000000000000000, 0.8660254037844387076, 1.000000000000000000, 0.8660254037844387076, 1.000000000000000000, 0.8660254037844387076, 1.000000000000000000, 0.8660254037844387076, 1.000000000000000000, 0.8660254037844387076, 1.000000000000000000, 0.8660254037844387076, 1.000000000000000000, 0.8660254037844387076, 1.000000000000000000, 0.8660254037844387076, 1.000000000000000000, 0.8660254037844387076, 1.000000000000000000, 0.8660254037844387076, 1.000000000000000000, 0.8660254037844387076, 1.000000000000000000, 0.8660254037844387076, 1.000000000000000000, 0.8660254037844387076, 1.000000000000000000, 0.8660254037844387076, 1.000000000000000000, 0.8660254037844387076, 1.000000000000000000, 0.8660254037844387076, 1.000000000000000000, 0.8660254037844387076, 1.000000000000000000, 0.8660254037844387076, 1.000000000000000000, 0.8660254037844387076, 1.000000000000000000, 0.8660254037844387076, 1.000000000000000000, 0.8660254037844387076, 1.000000000000000000, 0.8660254037844387076, 1.000000000000000000, 0.8660254037844387076, 1.000000000000000000, 0.8660254037844387076, 1.000000000000000000, 0.8660254037844387076, 1.000000000000000000, 0.8660254037844387076, 1.000000000000000000, 0.8660254037844387076, 1.000000000000000000, 0.8660254037844387076, 1.000000000000000000, 0.8660254037844387076, 1.000000000000000000, 0.8660254037844387076, 1.000000000000000000, 0.8660254037844387076, 1.000000000000000000, 0.8660254037844387076, 1.000000000000000000, 0.8660254037844387076, 1.000000000000000000, 0.8660254037844387076, 1.000000000000000000, 0.8660254037844387076, 1.000000000000000000, 0.8660254037844387076, 1.000000000000000000, 0.8660254037844387076, 1.000000000000000000, 0.8660254037844387076, 1.000000000000000000, 0.8660254037844387076, 1.000000000000000000, 0.8660254037844387076, 1.000000000000000000, 0.8660254037844387076, 1.000000000000000000, 0.8660254037844387076, 1.000000000000000000, 0.8660254037844387076, 1.000000000000000000, 0.8660254037844387076, 1.000000000000000000, 0.8660254037844387076, 1.000000000000000000, 0.8660254037844387076, 1.000000000000000000, 0.8660254037844387076, 1.000000000000000000, 0.8660254037844387076, 1.000000000000000000, 0.8660254037844387076, 1.000000000000000000, 0.8660254037844387076, 1.000000000000000000, 0.8660254037844387076, 1.000000000000000000, 0.8660254037844387076, 1.000000000000000000, 0.8660254037844387076, 1.000000000000000000, 0.8660254037844387076, 1.000000000000000000, 0.8660254037844387076, 1.000000000000000000, 0.8660254037844387076, 1.000000000000000000, 0.8660254037844387076, 1.000000000000000000, 0.8660254037844387076, 1.000000000000000000, 0.8660254037844387076, 1.000000000000000000, 0.8660254037844387076, 1.000000000000000000, 0.8660254037844387076, 1.000000000000000000, 0.8660254037844387076, 1.000000000000000000, 0.8660254037844387076, 1.000000000000000000, 0.8660254037844387076, 1.000000000000000000, 0.8660254037844387076, 1.000000000000000000, 0.8660254037844387076, 1.000000000000000000, 0.8660254037844387076, 1.000000000000000000, 0.8660254037844387076, 1.000000000000000000, 0.8660254037844387076, 1.000000000000000000, 0.8660254037844387076, 1.000000000000000000, 0.8660254037844387076, 1.000000000000000000, 0.8660254037844387076, 1.000000000000000000, 0.8660254037844387076, 1.000000000000000000, 0.8660254037844387076, 1.000000000000000000, 0.8660254037844387076, 1.000000000000000000, 0.8660254037844387076, 1.000000000000000000, 0.8660254037844387076, 1.000000000000000000, 0.8660254037844387076, 1.000000000000000000, 0.8660254037844387076, 1.000000000000000000, 0.8660254037844387076, 1.000000000000000000, 0.8660254037844387076, 1.000000000000000000, 0.8660254037844387076, 1.000000000000000000, 0.8660254037844387076, 1.000000000000000000, 0.8660254037844387076, 1.000000000000000000, 0.8660254037844387076, 1.000000000000000000, 0.8660254037844387076, 1.000000000000000000, 0.8660254037844387076, 1.000000000000000000, 0.8660254037844387076, 1.000000000000000000, 0.8660254037844387076, 1.000000000000000000, 0.8660254037844387076, 1.000000000000000000, 0.8660254037844387076, 1.000000000000000000, 0.8660254037844387076, 1.000000000000000000, 0.8660254037844387076, 1.000000000000000000, 0.8660254037844387076, 1.000000000000000000, 0.8660254037844387076, 1.000000000000000000, 0.8660254037844387076, 1.000000000000000000, 0.8660254037844387076, 1.000000000000000000, 0.8660254037844387076, 1.000000000000000000, 0.8660254037844387076, 1.000000000000000000, 0.8660254037844387076, 1.000000000000000000, 0.8660254037844387076, 1.000000000000000000, 0.8660254037844387076, 1.000000000000000000, 0.8660254037844387076, 1.000000000000000000, 0.8660254037844387076, 1.000000000000000000, 0.8660254037844387076, 1.000000000000000000, 0.8660254037844387076, 1.000000000000000000, 0.8660254037844387076, 1.000000000000000000, 0.8660254037844387076, 1.000000000000000000, 0.8660254037844387076, 1.000000000000000000, 0.8660254037844387076, 1.000000000000000000, 0.8660254037844387076, 1.000000000000000000, 0.8660254037844387076, 1.000000000000000000, 0.8660254037844387076, 1.000000000000000000, 0.8660254037844387076, 1.000000000000000000, 0.9024577157650887083, 0.9469497795711399046, 0.9469497795711399046, 0.9469497795711399046),
 ( 1.000000000000000000, 0.8660254037844387076, 1.000000000000000000, 0.8660254037844387076, 1.000000000000000000, 0.8660254037844387076, 1.000000000000000000, 0.8660254037844387076, 1.000000000000000000, 0.8660254037844387076, 1.000000000000000000, 0.8660254037844387076, 1.000000000000000000, 0.8660254037844387076, 1.000000000000000000, 0.8660254037844387076, 1.000000000000000000, 0.8660254037844387076, 1.000000000000000000, 0.8660254037844387076, 1.000000000000000000, 0.8660254037844387076, 1.000000000000000000, 0.8660254037844387076, 1.000000000000000000, 0.8660254037844387076, 1.000000000000000000, 0.8660254037844387076, 1.000000000000000000, 0.8660254037844387076, 1.000000000000000000, 0.8660254037844387076, 1.000000000000000000, 0.8660254037844387076, 1.000000000000000000, 0.8660254037844387076, 1.000000000000000000, 0.8660254037844387076, 1.000000000000000000, 0.8660254037844387076, 1.000000000000000000, 0.8660254037844387076, 1.000000000000000000, 0.8660254037844387076, 1.000000000000000000, 0.8660254037844387076, 1.000000000000000000, 0.8660254037844387076, 1.000000000000000000, 0.8660254037844387076, 1.000000000000000000, 0.8660254037844387076, 1.000000000000000000, 0.8660254037844387076, 1.000000000000000000, 0.8660254037844387076, 1.000000000000000000, 0.8660254037844387076, 1.000000000000000000, 0.8660254037844387076, 1.000000000000000000, 0.8660254037844387076, 1.000000000000000000, 0.8660254037844387076, 1.000000000000000000, 0.8660254037844387076, 1.000000000000000000, 0.8660254037844387076, 1.000000000000000000, 0.8660254037844387076, 1.000000000000000000, 0.8660254037844387076, 1.000000000000000000, 0.8660254037844387076, 1.000000000000000000, 0.8660254037844387076, 1.000000000000000000, 0.8660254037844387076, 1.000000000000000000, 0.8660254037844387076, 1.000000000000000000, 0.8660254037844387076, 1.000000000000000000, 0.8660254037844387076, 1.000000000000000000, 0.8660254037844387076, 1.000000000000000000, 0.8660254037844387076, 1.000000000000000000, 0.8660254037844387076, 1.000000000000000000, 0.8660254037844387076, 1.000000000000000000, 0.8660254037844387076, 1.000000000000000000, 0.8660254037844387076, 1.000000000000000000, 0.8660254037844387076, 1.000000000000000000, 0.8660254037844387076, 1.000000000000000000, 0.8660254037844387076, 1.000000000000000000, 0.8660254037844387076, 1.000000000000000000, 0.8660254037844387076, 1.000000000000000000, 0.8660254037844387076, 1.000000000000000000, 0.8660254037844387076, 1.000000000000000000, 0.8660254037844387076, 1.000000000000000000, 0.8660254037844387076, 1.000000000000000000, 0.8660254037844387076, 1.000000000000000000, 0.8660254037844387076, 1.000000000000000000, 0.8660254037844387076, 1.000000000000000000, 0.8660254037844387076, 1.000000000000000000, 0.8660254037844387076, 1.000000000000000000, 0.8660254037844387076, 1.000000000000000000, 0.8660254037844387076, 1.000000000000000000, 0.8660254037844387076, 1.000000000000000000, 0.8660254037844387076, 1.000000000000000000, 0.8660254037844387076, 1.000000000000000000, 0.8660254037844387076, 1.000000000000000000, 0.8660254037844387076, 1.000000000000000000, 0.8660254037844387076, 1.000000000000000000, 0.8660254037844387076, 1.000000000000000000, 0.8660254037844387076, 1.000000000000000000, 0.8660254037844387076, 1.000000000000000000, 0.8660254037844387076, 1.000000000000000000, 0.8660254037844387076, 1.000000000000000000, 0.8660254037844387076, 1.000000000000000000, 0.8660254037844387076, 1.000000000000000000, 0.8660254037844387076, 1.000000000000000000, 0.8660254037844387076, 1.000000000000000000, 0.8660254037844387076, 1.000000000000000000, 0.8660254037844387076, 1.000000000000000000, 0.8660254037844387076, 1.000000000000000000, 0.8660254037844387076, 1.000000000000000000, 0.8660254037844387076, 1.000000000000000000, 0.8660254037844387076, 1.000000000000000000, 0.8660254037844387076, 1.000000000000000000, 0.8660254037844387076, 1.000000000000000000, 0.8660254037844387076, 1.000000000000000000, 0.8660254037844387076, 1.000000000000000000, 0.8660254037844387076, 1.000000000000000000, 0.8660254037844387076, 1.000000000000000000, 0.8660254037844387076, 1.000000000000000000, 0.8660254037844387076, 1.000000000000000000, 0.8660254037844387076, 1.000000000000000000, 0.8660254037844387076, 1.000000000000000000, 0.8660254037844387076, 1.000000000000000000, 0.8660254037844387076, 1.000000000000000000, 0.8660254037844387076, 1.000000000000000000, 0.8660254037844387076, 1.000000000000000000, 0.8660254037844387076, 1.000000000000000000, 0.8660254037844387076, 1.000000000000000000, 0.8660254037844387076, 1.000000000000000000, 0.8660254037844387076, 1.000000000000000000, 0.8660254037844387076, 1.000000000000000000, 0.8660254037844387076, 1.000000000000000000, 0.8660254037844387076, 1.000000000000000000, 0.8660254037844387076, 1.000000000000000000, 0.8660254037844387076, 1.000000000000000000, 0.8660254037844387076, 1.000000000000000000, 0.8660254037844387076, 1.000000000000000000, 0.8660254037844387076, 1.000000000000000000, 0.8660254037844387076, 1.000000000000000000, 0.8660254037844387076, 1.000000000000000000, 0.8660254037844387076, 1.000000000000000000, 0.8660254037844387076, 1.000000000000000000, 0.8660254037844387076, 1.000000000000000000, 0.8660254037844387076, 1.000000000000000000, 0.8660254037844387076, 1.000000000000000000, 0.8660254037844387076, 1.000000000000000000, 0.8660254037844387076, 1.000000000000000000, 0.8660254037844387076, 1.000000000000000000, 0.8660254037844387076, 1.000000000000000000, 0.8660254037844387076, 1.000000000000000000, 0.8660254037844387076, 1.000000000000000000, 0.8660254037844387076, 1.000000000000000000, 0.8660254037844387076, 1.000000000000000000, 0.8660254037844387076, 1.000000000000000000, 0.8660254037844387076, 1.000000000000000000, 0.8660254037844387076, 1.000000000000000000, 0.8660254037844387076, 1.000000000000000000, 0.8660254037844387076, 1.000000000000000000, 0.8660254037844387076, 1.000000000000000000, 0.8660254037844387076, 1.000000000000000000, 0.8660254037844387076, 1.000000000000000000, 0.8660254037844387076, 1.000000000000000000, 0.8660254037844387076, 1.000000000000000000, 0.8660254037844387076, 1.000000000000000000, 0.8660254037844387076, 1.000000000000000000, 0.8660254037844387076, 1.000000000000000000, 0.8660254037844387076, 1.000000000000000000, 0.8660254037844387076, 1.000000000000000000, 0.9024577157650887083, 0.9469497795711399046, 0.9469497795711399046, 0.9469497795711399046) ) ) 
 REPRESENTATION_ITEM ( '' )  SURFACE ( )  );
#41128=CARTESIAN_POINT ( 'NONE',  ( 92.69370383062498320, 88.66845928578035796, 78.42447916753380355 ) ) ;
#41129=CARTESIAN_POINT ( 'NONE',  ( -97.30629616937495996, -209.9999999999999716, 75.19656250086714522 ) ) ;
#41136=CARTESIAN_POINT ( 'NONE',  ( -97.30629616937501680, 88.66845928578038638, 75.24947916753383481 ) ) ;
#41137=CARTESIAN_POINT ( 'NONE',  ( 93.84685191531249870, -208.0026889286704943, 77.47197916753380298 ) ) ;
#41145=VECTOR ( 'NONE', #48128, 1000.000000000000000 ) ;
#41152=CARTESIAN_POINT ( 'NONE',  ( 96.15314808468748708, 91.99731107132950569, 82.60489583420049087 ) ) ;
#41154=CARTESIAN_POINT ( 'NONE',  ( 95.00000000000000000, -206.9400435732949575, 75.87125000000000341 ) ) ;
#41155=ORIENTED_EDGE ( 'NONE', *, *, #47985, .F. ) ;
#41156=ORIENTED_EDGE ( 'NONE', *, *, #27490, .T. ) ;
#41158=EDGE_LOOP ( 'NONE', ( #58536, #7304, #11114, #8698 ) ) ;
#41162=CARTESIAN_POINT ( 'NONE',  ( -97.64999999994212487, -210.0000112241608292, 75.47473230080855444 ) ) ;
#41164=CARTESIAN_POINT ( 'NONE',  ( 92.35000000000007958, 88.47002178664747873, 83.70291666666668107 ) ) ;
#41167=CARTESIAN_POINT ( 'NONE',  ( -97.65000000000001990, 90.00000000000004263, 90.00000000000000000 ) ) ;
#41168=CARTESIAN_POINT ( 'NONE',  ( 92.34999999999999432, 90.00000000000002842, 77.93499999999998806 ) ) ;
#41170=CARTESIAN_POINT ( 'NONE',  ( -93.67499999999998295, -207.7050326799711968, 80.34270833506762699 ) ) ;
#41172=DIRECTION ( 'NONE',  ( -0.000000000000000000, -0.000000000000000000, 1.000000000000000000 ) ) ;
#41174=ORIENTED_EDGE ( 'NONE', *, *, #3942, .F. ) ;
#41175=CARTESIAN_POINT ( 'NONE',  ( 92.34999999999999432, 90.00000000000002842, 78.01437500173430806 ) ) ;
#41176=CARTESIAN_POINT ( 'NONE',  ( -96.32500000000001705, 92.29496732002878900, 77.27354166840096639 ) ) ;
#41179=CARTESIAN_POINT ( 'NONE',  ( 92.69370383062498320, 88.66845928578037217, 80.32947916753381890 ) ) ;
#41180=CARTESIAN_POINT ( 'NONE',  ( -2.500000000000020428, -90.00000000000000000, -310.0000000000000000 ) ) ;
#41195=CARTESIAN_POINT ( 'NONE',  ( -96.15314808468747287, -208.0026889286704943, 76.36072916753381890 ) ) ;
#41197=CARTESIAN_POINT ( 'NONE',  ( -92.35000000000400178, 89.99999541993113894, 76.42687486206344261 ) ) ;
#41207=CARTESIAN_POINT ( 'NONE',  ( 94.99999999999998579, 93.05995642670504253, 86.11062500173430578 ) ) ;
#41210=CARTESIAN_POINT ( 'NONE',  ( 96.15314808468748708, 91.99731107132950569, 86.41489583420049314 ) ) ;
#41211=CARTESIAN_POINT ( 'NONE',  ( -92.69370383062498320, -211.3315407142195852, 87.52614583420049144 ) ) ;
#41215=CARTESIAN_POINT ( 'NONE',  ( -92.34999999999999432, -211.5299782133524502, 80.10458333333332348 ) ) ;
#41216=CARTESIAN_POINT ( 'NONE',  ( -93.51319757292682766, 91.80467564693685745, 74.81083481226639265 ) ) ;
#41217=CARTESIAN_POINT ( 'NONE',  ( 96.15314808468748708, -208.0026889286704943, 86.89114583420047211 ) ) ;
#41226=ORIENTED_EDGE ( 'NONE', *, *, #74284, .F. ) ;
#41228=CARTESIAN_POINT ( 'NONE',  ( 97.30629616937498838, -208.6684592857803295, 82.55197916753380127 ) ) ;
#41233=CARTESIAN_POINT ( 'NONE',  ( -92.35000000000306386, -210.0000040461925437, 77.06187486178056645 ) ) ;
#41237=CARTESIAN_POINT ( 'NONE',  ( 96.32499999999998863, -212.2949673200287179, 85.13166666666666060 ) ) ;
#41239=EDGE_CURVE ( 'NONE', #17937, #12034, #8363, .T. ) ;
#41248=CARTESIAN_POINT ( 'NONE',  ( -97.30629616937501680, 88.66845928578038638, 86.04447916753382231 ) ) ;
#41251=CARTESIAN_POINT ( 'NONE',  ( -97.65000000000001990, 90.00000000000004263, 90.00000000000000000 ) ) ;
#41252=CARTESIAN_POINT ( 'NONE',  ( 95.00000000000000000, -212.6630814284392557, 88.53156250086713897 ) ) ;
#41253=CARTESIAN_POINT ( 'NONE',  ( 96.32499999999997442, 92.29496732002878900, 78.99333333333332519 ) ) ;
#41256=CARTESIAN_POINT ( 'NONE',  ( -93.67499999999998295, -212.2949673200287179, 89.02104166840096866 ) ) ;
#41257=ORIENTED_EDGE ( 'NONE', *, *, #42306, .T. ) ;
#41259=ORIENTED_EDGE ( 'NONE', *, *, #14582, .F. ) ;
#41262=CARTESIAN_POINT ( 'NONE',  ( 94.99999999999998579, 92.66308142843935514, 76.14906250086716000 ) ) ;
#41263=ORIENTED_EDGE ( 'NONE', *, *, #25325, .T. ) ;
#41271=CARTESIAN_POINT ( 'NONE',  ( -96.15314808468747287, -208.0026889286704943, 75.56697916753381605 ) ) ;
#41281=CARTESIAN_POINT ( 'NONE',  ( -93.84685191531247028, -211.9973110713294489, 88.74322916753382628 ) ) ;
#41286=CARTESIAN_POINT ( 'NONE',  ( 97.30629616937498838, 88.66845928578037217, 77.20739583420046870 ) ) ;
#41289=FACE_OUTER_BOUND ( 'NONE', #33996, .T. ) ;
#41290=CARTESIAN_POINT ( 'NONE',  ( 93.84685191531248449, 88.00268892867053694, 82.12864583420046927 ) ) ;
#41293=CARTESIAN_POINT ( 'NONE',  ( -97.65000000000001990, 90.00000000000004263, 81.10999999999999943 ) ) ;
#41300=CARTESIAN_POINT ( 'NONE',  ( 92.35000000000000853, -209.9999999999999716, 85.63437500173431260 ) ) ;
#41302=CARTESIAN_POINT ( 'NONE',  ( -95.00000000000002842, 87.33691857156074434, 85.35656250086714181 ) ) ;
#41308=CARTESIAN_POINT ( 'NONE',  ( 92.35000000006147047, -209.9999881782113107, 76.10900611559200968 ) ) ;
#41313=CARTESIAN_POINT ( 'NONE',  ( 95.00000000000000000, -207.3369185715606307, 82.65781250086715204 ) ) ;
#41314=VERTEX_POINT ( 'NONE', #23520 ) ;
#41316=VERTEX_POINT ( 'NONE', #47562 ) ;
#41317=EDGE_CURVE ( 'NONE', #73338, #5282, #35898, .T. ) ;
#41322=( BOUNDED_CURVE ( )  B_SPLINE_CURVE ( 2, ( #3320, #4806, #72443, #44644, #48777, #49152, #43539 ),
 .UNSPECIFIED., .F., .F. ) 
 B_SPLINE_CURVE_WITH_KNOTS ( ( 3, 2, 2, 3 ),
 ( 0.04166666666666644231, 0.04861111111111085514, 0.05555555555555525410, 0.06249999999999966693 ),
 .UNSPECIFIED. ) 
 CURVE ( )  GEOMETRIC_REPRESENTATION_ITEM ( )  RATIONAL_B_SPLINE_CURVE ( ( 1.000000000000004219, 0.8660254037844343777, 1.000000000000000000, 0.8660254037844387076, 1.000000000000000000, 0.8660254037844451469, 0.9999999999999935607 ) ) 
 REPRESENTATION_ITEM ( '' )  );
#41325=CARTESIAN_POINT ( 'NONE',  ( 96.15314808468748708, -208.0026889286704943, 78.15989583420049769 ) ) ;
#41327=VERTEX_POINT ( 'NONE', #37016 ) ;
#41336=CARTESIAN_POINT ( 'NONE',  ( 93.67500000000001137, -207.7050326799711968, 86.16354166840096696 ) ) ;
#41337=CARTESIAN_POINT ( 'NONE',  ( 97.64999999999999147, 90.00000000000002842, 89.68250000000000455 ) ) ;
#41339=CARTESIAN_POINT ( 'NONE',  ( 94.99999999999998579, 93.05995642670504253, 84.84062500173429555 ) ) ;
#41347=CARTESIAN_POINT ( 'NONE',  ( 97.64999999999997726, 91.52997821335252127, 84.73479166840097321 ) ) ;
#41360=CARTESIAN_POINT ( 'NONE',  ( -95.00000000000002842, 93.05995642670501411, 89.20624999999999716 ) ) ;
#41361=ADVANCED_FACE ( 'NONE', ( #54679 ), #2488, .F. ) ;
#41366=ORIENTED_EDGE ( 'NONE', *, *, #11949, .T. ) ;
#41367=CARTESIAN_POINT ( 'NONE',  ( 96.32499999999998863, -212.2949673200287179, 85.13166666666666060 ) ) ;
#41368=CARTESIAN_POINT ( 'NONE',  ( -92.69370383062498320, -208.6684592857803011, 84.29822916753380468 ) ) ;
#41369=ORIENTED_EDGE ( 'NONE', *, *, #57836, .F. ) ;
#41371=CARTESIAN_POINT ( 'NONE',  ( -93.08359813425042262, 88.16968857444109631, 74.99954695036826990 ) ) ;
#41374=CARTESIAN_POINT ( 'NONE',  ( -92.69370383062498320, -211.3315407142195852, 77.20739583420046870 ) ) ;
#41375=VECTOR ( 'NONE', #8709, 1000.000000000000000 ) ;
#41380=CARTESIAN_POINT ( 'NONE',  ( 96.32499999999998863, 87.70503267997126784, 88.30666666666665776 ) ) ;
#41381=CARTESIAN_POINT ( 'NONE',  ( -97.30629616937501680, 88.66845928578038638, 79.53572916753380184 ) ) ;
#41388=CARTESIAN_POINT ( 'NONE',  ( 97.64999999999999147, 90.00000000000002842, 87.14249999999999829 ) ) ;
#41389=CARTESIAN_POINT ( 'NONE',  ( 95.73180504966251192, -212.6374485842880233, 75.02735117824599342 ) ) ;
#41391=CARTESIAN_POINT ( 'NONE',  ( -93.84685191531247028, -211.9973110713294489, 77.31322916753381946 ) ) ;
#41392=PLANE ( 'NONE',  #54876 ) ;
#41396=AXIS2_PLACEMENT_3D ( 'NONE', #32816, #5026, #22298 ) ;
#41401=VECTOR ( 'NONE', #39183, 1000.000000000000000 ) ;
#41404=ORIENTED_EDGE ( 'NONE', *, *, #12235, .F. ) ;
#41409=CARTESIAN_POINT ( 'NONE',  ( 93.84685191531249870, -208.0026889286704943, 85.09197916753380753 ) ) ;
#41410=CARTESIAN_POINT ( 'NONE',  ( 95.00000000000000000, -207.3369185715606307, 87.73781250086715033 ) ) ;
#41411=VERTEX_POINT ( 'NONE', #54316 ) ;
#41413=CARTESIAN_POINT ( 'NONE',  ( 92.69370383062501162, -209.9999999999999716, 89.80156250086714920 ) ) ;
#41418=CARTESIAN_POINT ( 'NONE',  ( -97.30629616937501680, 91.33154071421968467, 80.85864583420048746 ) ) ;
#41419=ORIENTED_EDGE ( 'NONE', *, *, #36729, .T. ) ;
#41423=CARTESIAN_POINT ( 'NONE',  ( 97.64999999999999147, -210.0000001167898631, 84.68187499741277691 ) ) ;
#41434=CARTESIAN_POINT ( 'NONE',  ( 97.30629616937498838, -209.9999999999999716, 80.43531250086714124 ) ) ;
#41441=CARTESIAN_POINT ( 'NONE',  ( 92.35000000000000853, -209.9999999999999716, 76.66499999999999204 ) ) ;
#41442=CARTESIAN_POINT ( 'NONE',  ( -97.30629616937497417, -208.6684592857803011, 85.77989583420048803 ) ) ;
#41443=CARTESIAN_POINT ( 'NONE',  ( -97.30629616937501680, 88.66845928578038638, 81.59947916753381492 ) ) ;
#41444=ADVANCED_FACE ( 'NONE', ( #48670, #61439 ), #32103, .T. ) ;
#41447=CARTESIAN_POINT ( 'NONE',  ( 97.30629616937498838, 91.33154071421968467, 80.48822916753383083 ) ) ;
#41449=CARTESIAN_POINT ( 'NONE',  ( -97.65000000000001990, 88.47002178664754979, 78.70229166840096013 ) ) ;
#41452=CARTESIAN_POINT ( 'NONE',  ( 93.67500000000001137, -212.2949673200287179, 76.21520833506762926 ) ) ;
#41455=DIRECTION ( 'NONE',  ( -0.000000000000000000, -0.000000000000000000, 1.000000000000000000 ) ) ;
#41456=CARTESIAN_POINT ( 'NONE',  ( -94.99999999999997158, -207.3369185715606307, 85.03906250086714635 ) ) ;
#41458=CARTESIAN_POINT ( 'NONE',  ( -96.32500000000001705, 87.70503267997129626, 88.91520833506763211 ) ) ;
#41460=CONICAL_SURFACE ( 'NONE', #715, 2.649999999999999467, 1.029744258676654312 ) ;
#41465=CARTESIAN_POINT ( 'NONE',  ( -93.67500000000003979, 87.70503267997129626, 75.60666666666665492 ) ) ;
#41467=CARTESIAN_POINT ( 'NONE',  ( -95.00000000000002842, 92.66308142843932671, 87.57906250086713840 ) ) ;
#41470=CARTESIAN_POINT ( 'NONE',  ( 96.32499999999998863, -207.7050326799711968, 77.80270833506763495 ) ) ;
#41471=CARTESIAN_POINT ( 'NONE',  ( -92.35000000000010800, -208.4700217866473793, 78.30541666666667311 ) ) ;
#41475=CARTESIAN_POINT ( 'NONE',  ( 97.64999999999999147, -209.9999999999999716, 87.77749999999998920 ) ) ;
#41480=CARTESIAN_POINT ( 'NONE',  ( -97.30629616937497417, -208.6684592857803011, 87.20864583420049598 ) ) ;
#41482=CARTESIAN_POINT ( 'NONE',  ( 92.69370383062498320, 88.66845928578035796, 75.24947916753383481 ) ) ;
#41484=CARTESIAN_POINT ( 'NONE',  ( -94.99999999999997158, -207.3369185715606307, 75.03781250086714749 ) ) ;
#41486=ORIENTED_EDGE ( 'NONE', *, *, #6809, .T. ) ;
#41487=CARTESIAN_POINT ( 'NONE',  ( 93.67499999999999716, 87.70503267997126784, 87.64520833506762187 ) ) ;
#41494=CARTESIAN_POINT ( 'NONE',  ( -92.69370383062504004, 90.00000000000004263, 74.87906250086714977 ) ) ;
#41495=CARTESIAN_POINT ( 'NONE',  ( 93.84685191531249870, -208.0026889286704943, 76.20197916753380696 ) ) ;
#41514=CARTESIAN_POINT ( 'NONE',  ( 97.30629616937498838, 91.33154071421968467, 78.74197916753382742 ) ) ;
#41517=CARTESIAN_POINT ( 'NONE',  ( 96.32499999999998863, -207.7050326799711968, 75.18333333333332291 ) ) ;
#41523=ORIENTED_EDGE ( 'NONE', *, *, #4241, .T. ) ;
#41525=CARTESIAN_POINT ( 'NONE',  ( -95.00000000000002842, 86.94004357329504273, 87.61874999999999147 ) ) ;
#41532=CARTESIAN_POINT ( 'NONE',  ( -93.67499999999998295, -207.7050326799711968, 79.70770833506762187 ) ) ;
#41533=DIRECTION ( 'NONE',  ( 0.000000000000000000, -0.000000000000000000, -1.000000000000000000 ) ) ;
#41535=ORIENTED_EDGE ( 'NONE', *, *, #42022, .F. ) ;
#41536=CARTESIAN_POINT ( 'NONE',  ( 96.90829146052656995, 88.16127117233635602, 74.44346887015069569 ) ) ;
#41537=CARTESIAN_POINT ( 'NONE',  ( -95.00000000000002842, 86.94004357329504273, 76.90312500173429555 ) ) ;
#41538=( BOUNDED_CURVE ( )  B_SPLINE_CURVE ( 2, ( #13903, #60178, #3044, #65802, #25209, #24465, #47399 ),
 .UNSPECIFIED., .F., .F. ) 
 B_SPLINE_CURVE_WITH_KNOTS ( ( 3, 2, 2, 3 ),
 ( 0.3175094496522546383, 0.3245652148821828731, 0.3316209804230999536, 0.3386766260354857061 ),
 .UNSPECIFIED. ) 
 CURVE ( )  GEOMETRIC_REPRESENTATION_ITEM ( )  RATIONAL_B_SPLINE_CURVE ( ( 1.000000000000000000, 0.8660254037844387076, 1.000000000000000000, 0.8660254037844387076, 1.000000000000000000, 0.8660276809826341626, 0.9999954456810212777 ) ) 
 REPRESENTATION_ITEM ( '' )  );
#41540=CARTESIAN_POINT ( 'NONE',  ( 93.84685191531248449, 91.99731107132950569, 78.90072916753382515 ) ) ;
#41541=DIRECTION ( 'NONE',  ( 0.000000000000000000, 0.000000000000000000, 1.000000000000000000 ) ) ;
#41546=ORIENTED_EDGE ( 'NONE', *, *, #58384, .T. ) ;
#41549=ORIENTED_EDGE ( 'NONE', *, *, #55414, .T. ) ;
#41554=CARTESIAN_POINT ( 'NONE',  ( -92.69370383062498320, -209.9999999999999716, 78.68906250086715204 ) ) ;
#41555=( BOUNDED_CURVE ( )  B_SPLINE_CURVE ( 2, ( #45857, #62026, #27 ),
 .UNSPECIFIED., .F., .F. ) 
 B_SPLINE_CURVE_WITH_KNOTS ( ( 3, 3 ),
 ( 0.9791666666666669627, 0.9841647806526082620 ),
 .UNSPECIFIED. ) 
 CURVE ( )  GEOMETRIC_REPRESENTATION_ITEM ( )  RATIONAL_B_SPLINE_CURVE ( ( 0.9999999999999935607, 0.9035746763527574554, 0.9459494432169380795 ) ) 
 REPRESENTATION_ITEM ( '' )  );
#41556=ORIENTED_EDGE ( 'NONE', *, *, #45247, .F. ) ;
#41559=CYLINDRICAL_SURFACE ( 'NONE', #32199, 15.70000000000000284 ) ;
#41562=LINE ( 'NONE', #69040, #12424 ) ;
#41566=CARTESIAN_POINT ( 'NONE',  ( -97.64999999999996305, -209.9999999999999716, 84.99937500173429328 ) ) ;
#41567=CARTESIAN_POINT ( 'NONE',  ( -97.64999999999996305, -209.9999999999999716, 78.57000000000000739 ) ) ;
#41571=CARTESIAN_POINT ( 'NONE',  ( 94.99999999999998579, 92.66308142843932671, 83.29281250086715715 ) ) ;
#41572=CARTESIAN_POINT ( 'NONE',  ( -92.69370383062498320, -211.3315407142195852, 88.16114583420048234 ) ) ;
#41576=CARTESIAN_POINT ( 'NONE',  ( -92.34999999999999432, -211.5299782133524502, 81.37458333333333371 ) ) ;
#41578=CARTESIAN_POINT ( 'NONE',  ( -92.69370383062505425, 88.66845928578038638, 75.93739583420050110 ) ) ;
#41583=CARTESIAN_POINT ( 'NONE',  ( 97.30629616937498838, -208.6684592857803011, 88.10822916753380696 ) ) ;
#41585=ORIENTED_EDGE ( 'NONE', *, *, #30735, .F. ) ;
#41587=CARTESIAN_POINT ( 'NONE',  ( 92.34999999999995168, -211.5299782133524502, 75.44791666666667140 ) ) ;
#41591=ORIENTED_EDGE ( 'NONE', *, *, #53374, .F. ) ;
#41592=EDGE_CURVE ( 'NONE', #66094, #38048, #21565, .T. ) ;
#41594=CARTESIAN_POINT ( 'NONE',  ( 96.15314808468750130, -211.9973110713294489, 83.02822916753380866 ) ) ;
#41597=CARTESIAN_POINT ( 'NONE',  ( 97.65000000000000568, -211.5299782133524218, 76.92958333333332632 ) ) ;
#41599=FACE_OUTER_BOUND ( 'NONE', #26512, .T. ) ;
#41600=CARTESIAN_POINT ( 'NONE',  ( 97.64999999999997726, -208.4700217866474645, 83.38541666666667140 ) ) ;
#41604=ORIENTED_EDGE ( 'NONE', *, *, #20574, .F. ) ;
#41607=EDGE_CURVE ( 'NONE', #74237, #66421, #74031, .T. ) ;
#41609=CARTESIAN_POINT ( 'NONE',  ( -96.15314808468752972, 91.99731107132950569, 87.79072916753381151 ) ) ;
#41613=CARTESIAN_POINT ( 'NONE',  ( 97.30629616937498838, -209.9999999999999716, 88.05531250086713158 ) ) ;
#41614=CARTESIAN_POINT ( 'NONE',  ( 94.99999999999998579, 93.05995642670504253, 79.04625000000000057 ) ) ;
#41615=ORIENTED_EDGE ( 'NONE', *, *, #11965, .T. ) ;
#41617=EDGE_LOOP ( 'NONE', ( #2916, #35412, #37522, #12395 ) ) ;
#41618=CARTESIAN_POINT ( 'NONE',  ( -94.99999999999997158, -213.0599564267049857, 85.07875000000001364 ) ) ;
#41621=CARTESIAN_POINT ( 'NONE',  ( -96.32500000000001705, 87.70503267997129626, 85.74020833506763495 ) ) ;
#41622=CARTESIAN_POINT ( 'NONE',  ( 97.30629616937498838, 88.66845928578037217, 76.57239583420046358 ) ) ;
#41632=ORIENTED_EDGE ( 'NONE', *, *, #26636, .F. ) ;
#41637=CARTESIAN_POINT ( 'NONE',  ( -97.30629616937497417, -208.6684592857803011, 88.47864583420047779 ) ) ;
#41639=CARTESIAN_POINT ( 'NONE',  ( -92.34999999999999432, -209.9999999999999716, 82.69749999999999091 ) ) ;
#41646=CARTESIAN_POINT ( 'NONE',  ( 97.30629616937498838, 88.66845928578035796, 82.28739583420048120 ) ) ;
#41648=CARTESIAN_POINT ( 'NONE',  ( -92.35000000000005116, 91.52997821335253548, 80.28979166840095161 ) ) ;
#41653=CARTESIAN_POINT ( 'NONE',  ( 95.00000000000000000, -209.9999999999999716, 90.00000000000000000 ) ) ;
#41659=CARTESIAN_POINT ( 'NONE',  ( -97.30629616937501680, 90.00000000000004263, 87.73781250086713612 ) ) ;
#41664=( BOUNDED_CURVE ( )  B_SPLINE_CURVE ( 2, ( #35984, #17591, #1088, #6681, #29587, #7428, #40904, #47281, #46534 ),
 .UNSPECIFIED., .F., .F. ) 
 B_SPLINE_CURVE_WITH_KNOTS ( ( 3, 2, 2, 2, 3 ),
 ( 0.2116728463017078510, 0.2116729662275106394, 0.2187287317684276922, 0.2257844973093446894, 0.2328402629031412763 ),
 .UNSPECIFIED. ) 
 CURVE ( )  GEOMETRIC_REPRESENTATION_ITEM ( )  RATIONAL_B_SPLINE_CURVE ( ( 0.9999954457846356171, 0.9999977228536134355, 1.000000000000000000, 0.8660254037844387076, 1.000000000000000000, 0.8660254037844387076, 1.000000000000000000, 0.8660254037844387076, 1.000000000000000000 ) ) 
 REPRESENTATION_ITEM ( '' )  );
#41675=CARTESIAN_POINT ( 'NONE',  ( 95.00000000000000000, -212.6630814284392557, 81.07031250086716057 ) ) ;
#41677=VERTEX_POINT ( 'NONE', #63671 ) ;
#41678=ORIENTED_EDGE ( 'NONE', *, *, #70111, .F. ) ;
#41680=EDGE_CURVE ( 'NONE', #63633, #47974, #4445, .T. ) ;
#41683=CARTESIAN_POINT ( 'NONE',  ( -12.75044424985254921, 0.001194404164626844313, -80.00000000000001421 ) ) ;
#41686=CARTESIAN_POINT ( 'NONE',  ( 96.15314808468748708, -208.0026889286704943, 80.06489583420048461 ) ) ;
#41692=EDGE_CURVE ( 'NONE', #41704, #15433, #30171, .T. ) ;
#41695=VERTEX_POINT ( 'NONE', #41825 ) ;
#41697=CARTESIAN_POINT ( 'NONE',  ( 92.35000000000002274, -208.4700217866474645, 82.40645833506762585 ) ) ;
#41698=CARTESIAN_POINT ( 'NONE',  ( 97.64999999999999147, 90.00000000000002842, 89.04749999999999943 ) ) ;
#41700=CARTESIAN_POINT ( 'NONE',  ( 93.67499999999998295, 92.29496732002878900, 84.89354166840095672 ) ) ;
#41704=VERTEX_POINT ( 'NONE', #70016 ) ;
#41705=CARTESIAN_POINT ( 'NONE',  ( -92.69370383062504004, 90.00000000000004263, 87.57906250086715261 ) ) ;
#41709=CARTESIAN_POINT ( 'NONE',  ( 97.64999999999997726, 88.47002178664753558, 84.62895833506763665 ) ) ;
#41714=VERTEX_POINT ( 'NONE', #29418 ) ;
#41717=CARTESIAN_POINT ( 'NONE',  ( -97.65000000000009095, 91.52997821335247863, 86.13708333333332234 ) ) ;
#41719=CARTESIAN_POINT ( 'NONE',  ( -96.32500000000001705, 87.70503267997129626, 88.83583333333334053 ) ) ;
#41725=CARTESIAN_POINT ( 'NONE',  ( -94.99999999999997158, -207.3369185715606307, 81.86406250086714920 ) ) ;
#41727=FACE_OUTER_BOUND ( 'NONE', #28215, .T. ) ;
#41730=CARTESIAN_POINT ( 'NONE',  ( -97.64999999989197477, 90.00001510551047090, 78.64888723592453346 ) ) ;
#41740=ADVANCED_FACE ( 'NONE', ( #64036 ), #57656, .F. ) ;
#41742=CARTESIAN_POINT ( 'NONE',  ( -92.69370383062502583, 88.66845928578038638, 76.57239583420046358 ) ) ;
#41752=CARTESIAN_POINT ( 'NONE',  ( -92.69370383062498320, -209.9999999999999716, 75.51406250086715488 ) ) ;
#41754=( BOUNDED_CURVE ( )  B_SPLINE_CURVE ( 2, ( #69568, #57927, #27857, #29330, #51906, #45914, #22604 ),
 .UNSPECIFIED., .F., .F. ) 
 B_SPLINE_CURVE_WITH_KNOTS ( ( 3, 2, 2, 3 ),
 ( 0.5624999999999997780, 0.5694444444444440867, 0.5763888888888885065, 0.5833333333333329263 ),
 .UNSPECIFIED. ) 
 CURVE ( )  GEOMETRIC_REPRESENTATION_ITEM ( )  RATIONAL_B_SPLINE_CURVE ( ( 1.000000000000004219, 0.8660254037844343777, 1.000000000000000000, 0.8660254037844387076, 1.000000000000000000, 0.8660254037844472563, 0.9999999999999914513 ) ) 
 REPRESENTATION_ITEM ( '' )  );
#41765=DIRECTION ( 'NONE',  ( 1.000000000000000000, 0.000000000000000000, 0.000000000000000000 ) ) ;
#41772=CARTESIAN_POINT ( 'NONE',  ( 92.69370383062501162, -209.9999999999999716, 83.92781250086714806 ) ) ;
#41773=CARTESIAN_POINT ( 'NONE',  ( 96.15314808468748708, -208.0026889286704943, 87.04989583420048405 ) ) ;
#41776=CARTESIAN_POINT ( 'NONE',  ( -97.65000000000000568, 91.52997821335254969, 79.78708333333331382 ) ) ;
#41777=ORIENTED_EDGE ( 'NONE', *, *, #29611, .T. ) ;
#41780=CARTESIAN_POINT ( 'NONE',  ( -96.15314808468752972, 91.99731107132950569, 80.17072916753382117 ) ) ;
#41782=ORIENTED_EDGE ( 'NONE', *, *, #13728, .T. ) ;
#41788=CARTESIAN_POINT ( 'NONE',  ( 7.103376864691351012E-17, -120.0000000000000000, -85.59999999999999432 ) ) ;
#41799=CARTESIAN_POINT ( 'NONE',  ( 93.84685191531251292, -211.9973110713294489, 82.12864583420046927 ) ) ;
#41800=LINE ( 'NONE', #53820, #68918 ) ;
#41802=CARTESIAN_POINT ( 'NONE',  ( 97.64999999999999147, -209.9999999999999716, 90.00000000000000000 ) ) ;
#41803=LINE ( 'NONE', #64378, #513 ) ;
#41806=CARTESIAN_POINT ( 'NONE',  ( -97.64999999999996305, -210.0000343786549308, 88.80937619077334944 ) ) ;
#41807=CARTESIAN_POINT ( 'NONE',  ( -0.0004442498525516064278, 0.001194404164626844313, -85.59999999999999432 ) ) ;
#41808=CARTESIAN_POINT ( 'NONE',  ( -94.99999999999997158, -207.3369185715606307, 85.03906250086714635 ) ) ;
#41809=CARTESIAN_POINT ( 'NONE',  ( -96.15314808468752972, 91.99731107132950569, 82.07572916753382231 ) ) ;
#41811=CARTESIAN_POINT ( 'NONE',  ( 92.69370383062498320, 91.33154071421968467, 81.96989583420048575 ) ) ;
#41816=CARTESIAN_POINT ( 'NONE',  ( -94.99999999999997158, -213.0599564267049857, 83.25312500173430408 ) ) ;
#41819=CARTESIAN_POINT ( 'NONE',  ( -97.30629616937495996, -209.9999999999999716, 82.02281250086714692 ) ) ;
#41825=CARTESIAN_POINT ( 'NONE',  ( 23.50000000000000355, -120.0000000000000000, -64.00000000000000000 ) ) ;
#41828=ORIENTED_EDGE ( 'NONE', *, *, #46082, .T. ) ;
#41831=CARTESIAN_POINT ( 'NONE',  ( -92.35000000000005116, 91.52997821335253548, 75.76541666666666686 ) ) ;
#41834=CARTESIAN_POINT ( 'NONE',  ( -95.00000000000002842, 92.66308142843932671, 88.84906250086713442 ) ) ;
#41840=CARTESIAN_POINT ( 'NONE',  ( -97.30629616937501680, 91.33154071421968467, 75.61989583420047722 ) ) ;
#41848=CARTESIAN_POINT ( 'NONE',  ( 95.00000000000000000, -213.0599564267049857, 82.53874999999999318 ) ) ;
#41849=CARTESIAN_POINT ( 'NONE',  ( -97.30629616937495996, -209.9999999999999716, 87.89656250086714806 ) ) ;
#41855=CARTESIAN_POINT ( 'NONE',  ( -94.99999999999997158, -207.3369185715606307, 76.94281250086714863 ) ) ;
#41859=FACE_OUTER_BOUND ( 'NONE', #57696, .T. ) ;
#41861=CARTESIAN_POINT ( 'NONE',  ( 94.99999999999998579, 90.00000000000002842, 90.00000000000000000 ) ) ;
#41862=CARTESIAN_POINT ( 'NONE',  ( 93.84685191531251292, -211.9973110713294489, 77.04864583420047097 ) ) ;
#41864=AXIS2_PLACEMENT_3D ( 'NONE', #19697, #55027, #65585 ) ;
#41881=ORIENTED_EDGE ( 'NONE', *, *, #5227, .T. ) ;
#41884=EDGE_LOOP ( 'NONE', ( #53441, #61185, #29924, #53353 ) ) ;
#41885=CARTESIAN_POINT ( 'NONE',  ( 96.15314808468748708, 91.99731107132950569, 81.33489583420049485 ) ) ;
#41892=ORIENTED_EDGE ( 'NONE', *, *, #41092, .T. ) ;
#41899=CARTESIAN_POINT ( 'NONE',  ( -94.22990255303845686, 92.23316662872736060, 74.81945665767621279 ) ) ;
#41900=FACE_OUTER_BOUND ( 'NONE', #40526, .T. ) ;
#41901=CARTESIAN_POINT ( 'NONE',  ( -97.64999999980585699, -210.0000198431789897, 84.36502761000342332 ) ) ;
#41906=CARTESIAN_POINT ( 'NONE',  ( -92.34999999999999432, -211.5299782133524502, 80.81895833506764859 ) ) ;
#41909=CARTESIAN_POINT ( 'NONE',  ( 92.69370383062498320, 91.33154071421968467, 89.58989583420047609 ) ) ;
#41910=CARTESIAN_POINT ( 'NONE',  ( -97.65000000000001990, 91.52997821335253548, 74.78645833506763552 ) ) ;
#41912=ORIENTED_EDGE ( 'NONE', *, *, #53995, .T. ) ;
#41913=CARTESIAN_POINT ( 'NONE',  ( 97.30629616937498838, 88.66845928578037217, 77.36614583420048064 ) ) ;
#41914=DIRECTION ( 'NONE',  ( -0.000000000000000000, -0.000000000000000000, 1.000000000000000000 ) ) ;
#41916=CARTESIAN_POINT ( 'NONE',  ( 95.00000000000000000, -206.9400435732949575, 77.22062500173429100 ) ) ;
#41918=CARTESIAN_POINT ( 'NONE',  ( 97.64999999999999147, -209.9999998456624155, 79.60187500750917877 ) ) ;
#41931=CARTESIAN_POINT ( 'NONE',  ( -93.17363653571617021, -211.7597761561306129, 74.93163452119476631 ) ) ;
#41932=CARTESIAN_POINT ( 'NONE',  ( -96.15314808468747287, -208.0026889286704943, 78.90072916753382515 ) ) ;
#41938=AXIS2_PLACEMENT_3D ( 'NONE', #16107, #51060, #51804 ) ;
#41939=CARTESIAN_POINT ( 'NONE',  ( -92.35000000002600018, 89.99998827382285072, 82.77687459617033028 ) ) ;
#41944=CIRCLE ( 'NONE', #26311, 3.299999999999997158 ) ;
#41949=CARTESIAN_POINT ( 'NONE',  ( -94.99999999999997158, -206.9400435732949575, 77.85562500173431033 ) ) ;
#41953=CARTESIAN_POINT ( 'NONE',  ( 96.15314808468748708, 91.99731107132950569, 85.14489583420048291 ) ) ;
#41954=CARTESIAN_POINT ( 'NONE',  ( -94.99999999999997158, -212.6630814284392557, 85.51531250086715374 ) ) ;
#41959=CARTESIAN_POINT ( 'NONE',  ( -96.32499999999996021, -207.7050326799711968, 81.00416666666666288 ) ) ;
#41960=CARTESIAN_POINT ( 'NONE',  ( -95.00000000000002842, 87.33691857156074434, 77.10156250086711793 ) ) ;
#41966=CARTESIAN_POINT ( 'NONE',  ( 97.30629616937498838, -209.9999999999999716, 88.05531250086713158 ) ) ;
#41972=CARTESIAN_POINT ( 'NONE',  ( -97.65000000000001990, 90.00000000000004263, 75.39499999999999602 ) ) ;
#41977=CARTESIAN_POINT ( 'NONE',  ( 92.69370383062501162, -211.3315407142195852, 80.96447916753382401 ) ) ;
#41978=CARTESIAN_POINT ( 'NONE',  ( 96.32499999999997442, 92.29496732002878900, 89.78833333333332689 ) ) ;
#41980=( BOUNDED_CURVE ( )  B_SPLINE_CURVE ( 2, ( #58004, #29407, #23066, #52356, #28681, #1282, #69286, #41449, #24169, #58368, #11748 ),
 .UNSPECIFIED., .F., .F. ) 
 B_SPLINE_CURVE_WITH_KNOTS ( ( 3, 2, 2, 2, 2, 3 ),
 ( 0.6985206468843497829, 0.6985207885473544431, 0.7055765540882368292, 0.7126323196291192152, 0.7196880851700017123, 0.7196881748034551496 ),
 .UNSPECIFIED. ) 
 CURVE ( )  GEOMETRIC_REPRESENTATION_ITEM ( )  RATIONAL_B_SPLINE_CURVE ( ( 0.9999946203249847620, 0.9999973101084858040, 1.000000000000000000, 0.8660254037844387076, 1.000000000000000000, 0.8660254037844387076, 1.000000000000000000, 0.8660254037844387076, 1.000000000000000000, 0.9999982980435414559, 0.9999965961303247663 ) ) 
 REPRESENTATION_ITEM ( '' )  );
#41985=CARTESIAN_POINT ( 'NONE',  ( 97.64999999999997726, -211.5299782133524502, 83.27958333333333485 ) ) ;
#41992=CARTESIAN_POINT ( 'NONE',  ( 93.67500000000001137, -212.2949673200287179, 86.93083333333332519 ) ) ;
#41993=CARTESIAN_POINT ( 'NONE',  ( -93.84685191531254134, 91.99731107132950569, 86.41489583420049314 ) ) ;
#41995=AXIS2_PLACEMENT_3D ( 'NONE', #41016, #56166, #69576 ) ;
#41997=CARTESIAN_POINT ( 'NONE',  ( 93.84685191531251292, -211.9973110713294489, 87.20864583420046756 ) ) ;
#41998=CARTESIAN_POINT ( 'NONE',  ( 96.90829729882592858, 88.16127723152901297, 74.99909419456535886 ) ) ;
#42000=FACE_OUTER_BOUND ( 'NONE', #6251, .T. ) ;
#42004=CARTESIAN_POINT ( 'NONE',  ( -92.35000000000005116, 91.52997821335253548, 86.00479166840096923 ) ) ;
#42005=CARTESIAN_POINT ( 'NONE',  ( 97.30629616937498838, 89.06967028092473981, 74.68334033237941583 ) ) ;
#42010=EDGE_CURVE ( 'NONE', #54593, #71746, #73577, .T. ) ;
#42015=VECTOR ( 'NONE', #70467, 1000.000000000000000 ) ;
#42016=CARTESIAN_POINT ( 'NONE',  ( -92.35000000000005116, 91.52997821335253548, 81.55979166840097605 ) ) ;
#42022=EDGE_CURVE ( 'NONE', #7004, #9907, #37600, .T. ) ;
#42026=CARTESIAN_POINT ( 'NONE',  ( -93.84685191531248449, -208.0026889286704943, 86.41489583420049314 ) ) ;
#42034=CARTESIAN_POINT ( 'NONE',  ( 93.84685191531248449, 88.00268892867053694, 81.49364583420047836 ) ) ;
#42044=DIRECTION ( 'NONE',  ( 1.000000000000000000, 0.000000000000000000, 0.000000000000000000 ) ) ;
#42046=ORIENTED_EDGE ( 'NONE', *, *, #9829, .F. ) ;
#42048=CARTESIAN_POINT ( 'NONE',  ( -97.30629616937501680, 91.33154071421968467, 85.77989583420048803 ) ) ;
#42055=ORIENTED_EDGE ( 'NONE', *, *, #2409, .F. ) ;
#42057=CARTESIAN_POINT ( 'NONE',  ( 95.00000000000000000, -206.9400435732949575, 75.95062500173428077 ) ) ;
#42063=CARTESIAN_POINT ( 'NONE',  ( 95.00000000000000000, -212.6630814284392557, 82.34031250086714238 ) ) ;
#42071=CARTESIAN_POINT ( 'NONE',  ( 96.15314808468748708, -208.0026889286704943, 76.09614583420047040 ) ) ;
#42073=CARTESIAN_POINT ( 'NONE',  ( 95.00000000000000000, -212.6630814284392557, 79.16531250086715943 ) ) ;
#42079=CARTESIAN_POINT ( 'NONE',  ( -92.35000000000674447, -209.9999940177768565, 82.14187520865739600 ) ) ;
#42080=CARTESIAN_POINT ( 'NONE',  ( -97.64999999999996305, 91.52997821335257811, 82.96208333333332519 ) ) ;
#42083=CARTESIAN_POINT ( 'NONE',  ( 93.67500000000001137, -207.7050326799711968, 82.98854166840096980 ) ) ;
#42084=CARTESIAN_POINT ( 'NONE',  ( 93.67499999999999716, 87.70503267997126784, 88.20083333333332121 ) ) ;
#42085=ORIENTED_EDGE ( 'NONE', *, *, #8500, .F. ) ;
#42090=CARTESIAN_POINT ( 'NONE',  ( -95.00000000000002842, 92.66308142843932671, 89.00781250086716057 ) ) ;
#42091=CARTESIAN_POINT ( 'NONE',  ( 94.99999999999998579, 87.33691857156068750, 84.72156250086713669 ) ) ;
#42092=ORIENTED_EDGE ( 'NONE', *, *, #17931, .T. ) ;
#42093=CARTESIAN_POINT ( 'NONE',  ( 92.34999999999999432, 90.00000000000002842, 86.26937500173430351 ) ) ;
#42096=ORIENTED_EDGE ( 'NONE', *, *, #13890, .F. ) ;
#42099=CARTESIAN_POINT ( 'NONE',  ( -93.67500000000003979, 87.70503267997129626, 85.84604166840097150 ) ) ;
#42102=EDGE_CURVE ( 'NONE', #34388, #57700, #11662, .T. ) ;
#42106=CARTESIAN_POINT ( 'NONE',  ( 94.99999999999998579, 93.05995642670504253, 75.31562500173430408 ) ) ;
#42108=CARTESIAN_POINT ( 'NONE',  ( -97.65000000000001990, 88.47002178664754979, 83.70291666666668107 ) ) ;
#42110=LINE ( 'NONE', #24084, #67172 ) ;
#42113=CYLINDRICAL_SURFACE ( 'NONE', #71968, 2.649999999999999467 ) ;
#42114=CARTESIAN_POINT ( 'NONE',  ( -92.69370383062498320, -208.6684592857803011, 81.12322916753382174 ) ) ;
#42117=DIRECTION ( 'NONE',  ( -2.628368902995175337E-16, -1.000000000000000000, 0.000000000000000000 ) ) ;
#42123=VECTOR ( 'NONE', #56805, 1000.000000000000000 ) ;
#42126=LINE ( 'NONE', #74198, #32748 ) ;
#42130=EDGE_CURVE ( 'NONE', #52827, #57700, #73175, .T. ) ;
#42133=CARTESIAN_POINT ( 'NONE',  ( -97.30629616937501680, 88.66845928578038638, 76.36072916753381890 ) ) ;
#42139=EDGE_CURVE ( 'NONE', #16487, #47350, #10399, .T. ) ;
#42144=CARTESIAN_POINT ( 'NONE',  ( -97.64999999999994884, -211.5299782133524502, 86.87791666666664980 ) ) ;
#42156=CARTESIAN_POINT ( 'NONE',  ( 97.64999999999999147, -210.0000000024471092, 75.15687493081163950 ) ) ;
#42158=EDGE_LOOP ( 'NONE', ( #30522, #14162 ) ) ;
#42159=CARTESIAN_POINT ( 'NONE',  ( 96.15314808468748708, -208.0026889286704943, 84.35114583420048007 ) ) ;
#42160=CARTESIAN_POINT ( 'NONE',  ( 96.15314808468750130, -211.9973110713294489, 88.74322916753382628 ) ) ;
#42162=CARTESIAN_POINT ( 'NONE',  ( 96.15314808468748708, -208.0026889286704943, 88.95489583420049939 ) ) ;
#42163=VECTOR ( 'NONE', #19817, 1000.000000000000000 ) ;
#42165=CARTESIAN_POINT ( 'NONE',  ( -92.35000000000007958, -211.5299782133525071, 80.73958333333335702 ) ) ;
#42168=CARTESIAN_POINT ( 'NONE',  ( -93.84685191531252713, 88.00268892867056536, 81.75822916753382685 ) ) ;
#42170=EDGE_LOOP ( 'NONE', ( #54936, #65755, #51507, #68452 ) ) ;
#42172=CARTESIAN_POINT ( 'NONE',  ( -97.64999999969889188, -209.9999754409357422, 87.53856274002470172 ) ) ;
#42187=CARTESIAN_POINT ( 'NONE',  ( 96.15314808468750130, -211.9973110713294489, 77.78947916753381264 ) ) ;
#42193=EDGE_CURVE ( 'NONE', #34217, #16870, #27502, .T. ) ;
#42194=CARTESIAN_POINT ( 'NONE',  ( -92.34999999999988063, -211.5299782133523649, 75.65958333333333030 ) ) ;
#42196=CARTESIAN_POINT ( 'NONE',  ( 97.64999999999993463, -208.4700217866474077, 76.40041666666667197 ) ) ;
#42197=CARTESIAN_POINT ( 'NONE',  ( -93.84685191531247028, -211.9973110713294489, 82.23447916753380582 ) ) ;
#42198=CARTESIAN_POINT ( 'NONE',  ( -95.00000000000002842, 92.66308142843932671, 78.21281250086717307 ) ) ;
#42200=CARTESIAN_POINT ( 'NONE',  ( 96.15314808468748708, 91.99731107132950569, 80.54114583420046358 ) ) ;
#42202=DIRECTION ( 'NONE',  ( 1.000000000000000000, 0.000000000000000000, 0.000000000000000000 ) ) ;
#42205=CARTESIAN_POINT ( 'NONE',  ( 96.32499999999998863, 87.70503267997126784, 77.59104166840097605 ) ) ;
#42208=CARTESIAN_POINT ( 'NONE',  ( -94.99999999999997158, -207.3369185715606307, 83.76906250086715033 ) ) ;
#42218=CARTESIAN_POINT ( 'NONE',  ( 92.35000000049315361, 89.99996796133687837, 83.73041644179049570 ) ) ;
#42223=CARTESIAN_POINT ( 'NONE',  ( -95.00000000000002842, 87.33691857156074434, 84.08656250086713158 ) ) ;
#42228=( BOUNDED_CURVE ( )  B_SPLINE_CURVE ( 2, ( #1271, #7234, #40330, #35062, #58736, #69641, #12121 ),
 .UNSPECIFIED., .F., .F. ) 
 B_SPLINE_CURVE_WITH_KNOTS ( ( 3, 2, 2, 3 ),
 ( 0.7083333333333331483, 0.7152777777777775681, 0.7222222222222220989, 0.7291666666666665186 ),
 .UNSPECIFIED. ) 
 CURVE ( )  GEOMETRIC_REPRESENTATION_ITEM ( )  RATIONAL_B_SPLINE_CURVE ( ( 1.000000000000004219, 0.8660254037844343777, 1.000000000000000000, 0.8660254037844387076, 1.000000000000000000, 0.8660254037844408170, 0.9999999999999978906 ) ) 
 REPRESENTATION_ITEM ( '' )  );
#42230=CARTESIAN_POINT ( 'NONE',  ( -92.69370383062502583, 91.33154071421968467, 75.40822916753381833 ) ) ;
#42232=AXIS2_PLACEMENT_3D ( 'NONE', #56623, #46072, #33285 ) ;
#42235=CARTESIAN_POINT ( 'NONE',  ( -96.32499999999996021, -207.7050326799711968, 79.17854166840096752 ) ) ;
#42236=CARTESIAN_POINT ( 'NONE',  ( -94.99999999999997158, -212.6630814284392557, 86.78531250086716398 ) ) ;
#42240=CARTESIAN_POINT ( 'NONE',  ( -97.30629616937495996, -209.9999999999999716, 76.46656250086715545 ) ) ;
#42242=ORIENTED_EDGE ( 'NONE', *, *, #9312, .F. ) ;
#42243=CARTESIAN_POINT ( 'NONE',  ( 92.34999999999999432, 90.00000000000002842, 87.45999999999999375 ) ) ;
#42247=CARTESIAN_POINT ( 'NONE',  ( 92.69370383062501162, -208.6684592857803011, 87.20864583420049598 ) ) ;
#42248=ORIENTED_EDGE ( 'NONE', *, *, #64890, .T. ) ;
#42250=CARTESIAN_POINT ( 'NONE',  ( 96.32499999999998863, 87.70503267997126784, 87.11604166840096752 ) ) ;
#42264=DIRECTION ( 'NONE',  ( -0.000000000000000000, -0.000000000000000000, 1.000000000000000000 ) ) ;
#42270=CARTESIAN_POINT ( 'NONE',  ( 96.15314808468748708, 91.99731107132950569, 79.42989583420049371 ) ) ;
#42285=CARTESIAN_POINT ( 'NONE',  ( -95.00000000000002842, 90.00000000000004263, 90.00000000000000000 ) ) ;
#42289=CARTESIAN_POINT ( 'NONE',  ( -93.67499999999998295, -212.2949673200287179, 75.05104166840095559 ) ) ;
#42291=CARTESIAN_POINT ( 'NONE',  ( 97.64999999999999147, 90.00000000000002842, 76.42687500173430237 ) ) ;
#42292=CARTESIAN_POINT ( 'NONE',  ( -95.00000000000002842, 93.05995642670501411, 75.95062500173428077 ) ) ;
#42294=CARTESIAN_POINT ( 'NONE',  ( 92.69370383062498320, 88.66845928578037217, 77.78947916753381264 ) ) ;
#42296=CARTESIAN_POINT ( 'NONE',  ( 95.00000000000000000, -209.9999999999999716, 90.00000000000000000 ) ) ;
#42297=LINE ( 'NONE', #65226, #72708 ) ;
#42306=EDGE_CURVE ( 'NONE', #10235, #27941, #32984, .T. ) ;
#42312=CARTESIAN_POINT ( 'NONE',  ( -93.84685191531248449, -208.0026889286704943, 74.98489583420048632 ) ) ;
#42326=CARTESIAN_POINT ( 'NONE',  ( 96.15314808468748708, 88.00268892867053694, 83.02822916753380866 ) ) ;
#42327=CARTESIAN_POINT ( 'NONE',  ( -92.69370383062498320, -208.6684592857803295, 88.26697916753381890 ) ) ;
#42331=CARTESIAN_POINT ( 'NONE',  ( -96.32499999999996021, -207.7050326799711968, 82.90916666666666401 ) ) ;
#42332=CARTESIAN_POINT ( 'NONE',  ( -96.15314808468751551, 88.00268892867056536, 77.68364583420047609 ) ) ;
#42335=CARTESIAN_POINT ( 'NONE',  ( 92.69370383062501162, -209.9999999999999716, 87.73781250086713612 ) ) ;
#42343=ORIENTED_EDGE ( 'NONE', *, *, #24846, .F. ) ;
#42345=CARTESIAN_POINT ( 'NONE',  ( 96.15314808468750130, -211.9973110713294489, 79.85322916753381151 ) ) ;
#42350=CYLINDRICAL_SURFACE ( 'NONE', #12266, 2.649999999999985700 ) ;
#42352=CARTESIAN_POINT ( 'NONE',  ( 96.32499999999998863, -212.2949673200287179, 80.68666666666665321 ) ) ;
#42359=CARTESIAN_POINT ( 'NONE',  ( 92.35000000000000853, -209.9999999999999716, 86.82500000000000284 ) ) ;
#42361=CARTESIAN_POINT ( 'NONE',  ( -92.69370383062502583, 88.66845928578038638, 84.98614583420047097 ) ) ;
#42364=CARTESIAN_POINT ( 'NONE',  ( 92.34999999999999432, 90.00000000000002842, 76.03000000000000114 ) ) ;
#42371=CARTESIAN_POINT ( 'NONE',  ( -92.35000000000005116, 88.47002178664754979, 86.53395833506763779 ) ) ;
#42373=CARTESIAN_POINT ( 'NONE',  ( 97.30629616937498838, 91.33154071421968467, 87.63197916753382799 ) ) ;
#42375=CARTESIAN_POINT ( 'NONE',  ( 97.64999999994533653, -210.0000170172949367, 88.49187441316098557 ) ) ;
#42377=CARTESIAN_POINT ( 'NONE',  ( -92.34999999999999432, -210.0000154727988217, 78.33187446658357089 ) ) ;
#42383=CARTESIAN_POINT ( 'NONE',  ( -94.99999999999997158, -207.3369185715606307, 74.87906250086713555 ) ) ;
#42384=VERTEX_POINT ( 'NONE', #42676 ) ;
#42389=CARTESIAN_POINT ( 'NONE',  ( -97.65000000000001990, 91.52997821335253548, 75.42145833506764063 ) ) ;
#42390=CARTESIAN_POINT ( 'NONE',  ( -92.69370383062498320, -211.3315407142195852, 86.25614583420048120 ) ) ;
#42391=VERTEX_POINT ( 'NONE', #7359 ) ;
#42392=LINE ( 'NONE', #37123, #9291 ) ;
#42398=CARTESIAN_POINT ( 'NONE',  ( 97.30629616937498838, 88.66845928578035796, 81.01739583420048518 ) ) ;
#42411=CARTESIAN_POINT ( 'NONE',  ( -96.15314808468752972, 91.99731107132950569, 87.63197916753379957 ) ) ;
#42413=VECTOR ( 'NONE', #23301, 1000.000000000000000 ) ;
#42417=( BOUNDED_CURVE ( )  B_SPLINE_CURVE ( 2, ( #22999, #57204, #40649, #10967, #69586, #1213, #28242, #5711, #51177 ),
 .UNSPECIFIED., .F., .F. ) 
 B_SPLINE_CURVE_WITH_KNOTS ( ( 3, 2, 2, 2, 3 ),
 ( 0.000000000000000000, 0.007055765540882327075, 0.01411153108176465415, 0.02116729662264698122, 0.02116741234828206988 ),
 .UNSPECIFIED. ) 
 CURVE ( )  GEOMETRIC_REPRESENTATION_ITEM ( )  RATIONAL_B_SPLINE_CURVE ( ( 1.000000000000000000, 0.8660254037844387076, 1.000000000000000000, 0.8660254037844387076, 1.000000000000000000, 0.8660254037844387076, 1.000000000000000000, 0.9999978026062312786, 0.9999956052845440091 ) ) 
 REPRESENTATION_ITEM ( '' )  );
#42426=CARTESIAN_POINT ( 'NONE',  ( 97.30629616937498838, -209.9999999999999716, 83.13406250086715943 ) ) ;
#42431=EDGE_LOOP ( 'NONE', ( #26928, #67620, #13426, #15885 ) ) ;
#42433=ORIENTED_EDGE ( 'NONE', *, *, #47134, .T. ) ;
#42438=CARTESIAN_POINT ( 'NONE',  ( 93.84685191531251292, -211.9973110713294489, 79.11239583420048405 ) ) ;
#42445=CARTESIAN_POINT ( 'NONE',  ( -96.32500000000001705, 92.29496732002878900, 82.90916666666666401 ) ) ;
#42448=CARTESIAN_POINT ( 'NONE',  ( 93.67500000000001137, -207.7050326799711968, 84.25854166840096582 ) ) ;
#42449=CARTESIAN_POINT ( 'NONE',  ( 97.64999999999999147, 90.00000000000002842, 86.50750000000000739 ) ) ;
#42451=CARTESIAN_POINT ( 'NONE',  ( -0.0004442498525516064278, 0.001194404164626844313, -90.00000000000000000 ) ) ;
#42453=VECTOR ( 'NONE', #3229, 1000.000000000000000 ) ;
#42455=VERTEX_POINT ( 'NONE', #6975 ) ;
#42456=CARTESIAN_POINT ( 'NONE',  ( -93.84685191531252713, 88.00268892867056536, 88.10822916753382117 ) ) ;
#42457=CARTESIAN_POINT ( 'NONE',  ( 92.69370383062498320, 88.66845928578037217, 80.80572916753382628 ) ) ;
#42458=ADVANCED_FACE ( 'NONE', ( #29898 ), #52852, .F. ) ;
#42460=CARTESIAN_POINT ( 'NONE',  ( 96.32499999999998863, 87.70503267997126784, 85.21104166840096639 ) ) ;
#42466=EDGE_CURVE ( 'NONE', #40405, #28568, #2060, .T. ) ;
#42471=CARTESIAN_POINT ( 'NONE',  ( -92.34999999999996589, 91.52997821335250705, 85.92541666666664923 ) ) ;
#42473=CARTESIAN_POINT ( 'NONE',  ( -92.35000000000005116, 91.52997821335253548, 84.65541666666666742 ) ) ;
#42474=VERTEX_POINT ( 'NONE', #9938 ) ;
#42481=CARTESIAN_POINT ( 'NONE',  ( -93.84685191531248449, -208.0026889286704943, 83.71614583420047495 ) ) ;
#42482=VERTEX_POINT ( 'NONE', #67832 ) ;
#42487=CARTESIAN_POINT ( 'NONE',  ( 92.35000000049316782, -210.0000320386632495, 83.73041644179299681 ) ) ;
#42491=CARTESIAN_POINT ( 'NONE',  ( -96.32499999999996021, -212.2949673200287179, 85.66083333333332916 ) ) ;
#42492=CARTESIAN_POINT ( 'NONE',  ( 96.32499999999997442, 92.29496732002878900, 82.88270833506763324 ) ) ;
#42494=CARTESIAN_POINT ( 'NONE',  ( -95.00000000000002842, 92.66308142843932671, 89.64281250086715147 ) ) ;
#42502=CARTESIAN_POINT ( 'NONE',  ( 92.35000000005783249, 89.99998877583867340, 75.47473230081648410 ) ) ;
#42503=CARTESIAN_POINT ( 'NONE',  ( -92.34999999999999432, -208.4700217866474645, 87.83041666666666458 ) ) ;
#42504=DIRECTION ( 'NONE',  ( 1.000000000000000000, 0.000000000000000000, 0.000000000000000000 ) ) ;
#42512=ADVANCED_FACE ( 'NONE', ( #32861 ), #44911, .F. ) ;
#42514=ORIENTED_EDGE ( 'NONE', *, *, #10449, .F. ) ;
#42517=CARTESIAN_POINT ( 'NONE',  ( -92.34999999999999432, -210.0000000207151629, 80.87187500099602744 ) ) ;
#42520=CARTESIAN_POINT ( 'NONE',  ( 95.00000000000000000, -207.3369185715606307, 81.86406250086713499 ) ) ;
#42521=CARTESIAN_POINT ( 'NONE',  ( 92.69370383062501162, -208.6684592857803295, 87.20864583420048177 ) ) ;
#42523=CARTESIAN_POINT ( 'NONE',  ( 97.30629616937498838, -208.6684592857803011, 88.26697916753381890 ) ) ;
#42529=CARTESIAN_POINT ( 'NONE',  ( -95.00000000000002842, 87.33691857156074434, 75.99031250086716227 ) ) ;
#42534=DIRECTION ( 'NONE',  ( -1.000000000000000000, 0.000000000000000000, 0.000000000000000000 ) ) ;
#42535=CARTESIAN_POINT ( 'NONE',  ( 93.67500000000001137, -212.2949673200287179, 79.31083333333333485 ) ) ;
#42537=ORIENTED_EDGE ( 'NONE', *, *, #45249, .F. ) ;
#42539=AXIS2_PLACEMENT_3D ( 'NONE', #48799, #20607, #14211 ) ;
#42540=ORIENTED_EDGE ( 'NONE', *, *, #2840, .F. ) ;
#42541=CARTESIAN_POINT ( 'NONE',  ( -26.50000000000000355, -120.0000000000000000, -64.00000000000000000 ) ) ;
#42545=VERTEX_POINT ( 'NONE', #27603 ) ;
#42546=CARTESIAN_POINT ( 'NONE',  ( 97.30629616937498838, -208.6684592857803011, 79.21822916753380639 ) ) ;
#42549=ADVANCED_FACE ( 'NONE', ( #26856 ), #31751, .F. ) ;
#42550=CARTESIAN_POINT ( 'NONE',  ( -97.65000000000000568, 88.47002178664753558, 81.79791666666665151 ) ) ;
#42554=CARTESIAN_POINT ( 'NONE',  ( -95.00000000000002842, 86.94004357329504273, 80.63375000000000625 ) ) ;
#42558=CARTESIAN_POINT ( 'NONE',  ( -97.30629616937497417, -211.3315407142195852, 82.07572916753380809 ) ) ;
#42559=CARTESIAN_POINT ( 'NONE',  ( -97.30629616937501680, 88.66845928578038638, 78.42447916753380355 ) ) ;
#42562=CARTESIAN_POINT ( 'NONE',  ( 97.30629616937498838, 91.33154071421968467, 82.39322916753381776 ) ) ;
#42566=CARTESIAN_POINT ( 'NONE',  ( 92.35004024445044024, 88.46999855150322389, 77.43229327564787923 ) ) ;
#42569=CARTESIAN_POINT ( 'NONE',  ( -96.15314808468747287, -208.0026889286704943, 81.91697916753381037 ) ) ;
#42570=CARTESIAN_POINT ( 'NONE',  ( 97.65000000000000568, 88.47002178664753558, 87.08958333333333712 ) ) ;
#42579=CARTESIAN_POINT ( 'NONE',  ( -93.84685191531254134, 91.99731107132950569, 84.35114583420048007 ) ) ;
#42584=ORIENTED_EDGE ( 'NONE', *, *, #52217, .F. ) ;
#42586=CARTESIAN_POINT ( 'NONE',  ( -93.84685191531254134, 91.99731107132950569, 76.73114583420047552 ) ) ;
#42587=AXIS2_PLACEMENT_3D ( 'NONE', #40764, #29451, #70050 ) ;
#42592=CARTESIAN_POINT ( 'NONE',  ( 92.35000000000007958, 88.47002178664747873, 86.24291666666667311 ) ) ;
#42593=CARTESIAN_POINT ( 'NONE',  ( -97.30629616937495996, -209.9999999999999716, 81.54656250086715374 ) ) ;
#42604=ORIENTED_EDGE ( 'NONE', *, *, #50257, .F. ) ;
#42606=CARTESIAN_POINT ( 'NONE',  ( -97.65000000000001990, 90.00000000000004263, 90.00000000000000000 ) ) ;
#42610=CARTESIAN_POINT ( 'NONE',  ( 97.30629616937498838, -209.9999999999999716, 88.84906250086716284 ) ) ;
#42613=CARTESIAN_POINT ( 'NONE',  ( 92.34999999999999432, 88.47002178664752137, 86.95729166840096980 ) ) ;
#42622=ORIENTED_EDGE ( 'NONE', *, *, #4867, .F. ) ;
#42624=LINE ( 'NONE', #59178, #55124 ) ;
#42628=VERTEX_POINT ( 'NONE', #68951 ) ;
#42629=CARTESIAN_POINT ( 'NONE',  ( 92.69370383062498320, 88.66845928578037217, 80.96447916753382401 ) ) ;
#42637=LINE ( 'NONE', #19689, #50278 ) ;
#42648=CARTESIAN_POINT ( 'NONE',  ( -92.34999999999999432, -211.0689600337108232, 74.48490336299448700 ) ) ;
#42649=CARTESIAN_POINT ( 'NONE',  ( -97.30629616937501680, 88.66845928578038638, 87.94947916753382344 ) ) ;
#42650=CARTESIAN_POINT ( 'NONE',  ( 92.34999999999999432, 90.00000000000002842, 77.37937500173428873 ) ) ;
#42651=CARTESIAN_POINT ( 'NONE',  ( -95.00000000000002842, 93.05995642670501411, 74.68062500173429896 ) ) ;
#42652=( BOUNDED_CURVE ( )  B_SPLINE_CURVE ( 2, ( #33567, #9537, #26451, #72664, #44115, #56139, #4657, #32454, #32818 ),
 .UNSPECIFIED., .F., .F. ) 
 B_SPLINE_CURVE_WITH_KNOTS ( ( 3, 2, 2, 2, 3 ),
 ( 0.8043570860654217780, 0.8043572716605901229, 0.8114130372014725090, 0.8184688027423548951, 0.8255245790564514907 ),
 .UNSPECIFIED. ) 
 CURVE ( )  GEOMETRIC_REPRESENTATION_ITEM ( )  RATIONAL_B_SPLINE_CURVE ( ( 0.9999929520380047565, 0.9999964759263050285, 1.000000000000000000, 0.8660254037844387076, 1.000000000000000000, 0.8660254037844387076, 1.000000000000000000, 0.8660254037844387076, 1.000000000000000000 ) ) 
 REPRESENTATION_ITEM ( '' )  );
#42654=CARTESIAN_POINT ( 'NONE',  ( 92.69370383062498320, 88.66845928578037217, 75.88447916753382572 ) ) ;
#42657=DIRECTION ( 'NONE',  ( 1.000000000000000000, 0.000000000000000000, 0.000000000000000000 ) ) ;
#42663=DIRECTION ( 'NONE',  ( -1.000000000000000000, 0.000000000000000000, -0.000000000000000000 ) ) ;
#42670=CARTESIAN_POINT ( 'NONE',  ( -97.65000000000001990, 90.00000000000004263, 76.10937500173430692 ) ) ;
#42676=CARTESIAN_POINT ( 'NONE',  ( 97.64999999999996305, 90.00000034979572661, 77.69687501385438111 ) ) ;
#42682=LINE ( 'NONE', #66725, #1404 ) ;
#42688=CARTESIAN_POINT ( 'NONE',  ( 92.69370383062498320, 90.00000000000002842, 84.72156250086715090 ) ) ;
#42690=CARTESIAN_POINT ( 'NONE',  ( -92.69370383062498320, -208.6684592857803295, 86.36197916753383197 ) ) ;
#42694=CARTESIAN_POINT ( 'NONE',  ( -94.99999999999997158, -206.9400435732949575, 80.95125000000000171 ) ) ;
#42697=AXIS2_PLACEMENT_3D ( 'NONE', #7358, #59986, #31008 ) ;
#42698=CARTESIAN_POINT ( 'NONE',  ( 96.15314808468750130, -211.9973110713294489, 83.50447916753381605 ) ) ;
#42710=CARTESIAN_POINT ( 'NONE',  ( 93.84685191531251292, -211.9973110713294489, 79.74739583420048916 ) ) ;
#42712=CARTESIAN_POINT ( 'NONE',  ( -92.34999999999988063, -208.4700217866474929, 80.84541666666663673 ) ) ;
#42719=CARTESIAN_POINT ( 'NONE',  ( 97.64999999999997726, -208.4700217866474645, 82.75041666666665208 ) ) ;
#42725=CARTESIAN_POINT ( 'NONE',  ( -96.15314808468752972, 91.99731107132950569, 83.98072916753382344 ) ) ;
#42726=CARTESIAN_POINT ( 'NONE',  ( -97.65000000000001990, 90.00001272874953884, 81.82437456149077093 ) ) ;
#42727=B_SPLINE_CURVE_WITH_KNOTS ( 'NONE', 1,
 ( #29409, #11395 ),
 .UNSPECIFIED., .F., .F.,
 ( 2, 2 ),
 ( 0.000000000000000000, 1.000000000000000000 ),
 .UNSPECIFIED. ) ;
#42729=CARTESIAN_POINT ( 'NONE',  ( 97.64999999999996305, 88.93104485797731229, 75.04052853044674976 ) ) ;
#42730=CARTESIAN_POINT ( 'NONE',  ( -95.00000000000002842, 90.00000000000004263, 90.00000000000000000 ) ) ;
#42732=CARTESIAN_POINT ( 'NONE',  ( -94.99999999999997158, -213.0599564267049857, 86.42812500173430124 ) ) ;
#42736=CARTESIAN_POINT ( 'NONE',  ( -95.00000000000002842, 93.05995642670501411, 86.74562500173429669 ) ) ;
#42738=CARTESIAN_POINT ( 'NONE',  ( 96.15314808468748708, 91.99731107132950569, 88.31989583420048007 ) ) ;
#42741=CARTESIAN_POINT ( 'NONE',  ( -93.33864827737279768, 88.39919842643631398, 74.79754476654878204 ) ) ;
#42742=CARTESIAN_POINT ( 'NONE',  ( 93.67499999999999716, 87.70503267997126784, 88.83583333333334053 ) ) ;
#42747=DIRECTION ( 'NONE',  ( -4.476705744456276711E-17, 1.000000000000000000, -0.000000000000000000 ) ) ;
#42752=FACE_BOUND ( 'NONE', #27338, .T. ) ;
#42758=CARTESIAN_POINT ( 'NONE',  ( -93.84685191531247028, -211.9973110713294489, 83.02822916753380866 ) ) ;
#42760=FACE_OUTER_BOUND ( 'NONE', #19995, .T. ) ;
#42765=CARTESIAN_POINT ( 'NONE',  ( 92.69370383062498320, 91.33154071421968467, 88.47864583420047779 ) ) ;
#42768=CARTESIAN_POINT ( 'NONE',  ( 92.69370383062498320, 90.00000000000002842, 81.38781250086714181 ) ) ;
#42773=CARTESIAN_POINT ( 'NONE',  ( 96.40521225739021816, 91.86781405990345206, 74.80441578173235939 ) ) ;
#42779=LINE ( 'NONE', #18357, #61383 ) ;
#42781=CARTESIAN_POINT ( 'NONE',  ( -97.30629616937501680, 88.66845928578038638, 87.15572916753380639 ) ) ;
#42786=CARTESIAN_POINT ( 'NONE',  ( 96.32499999999998863, -207.7050326799711968, 83.43833333333333258 ) ) ;
#42791=CARTESIAN_POINT ( 'NONE',  ( 97.30629616937498838, -209.9999999999999716, 83.76906250086716454 ) ) ;
#42796=ADVANCED_FACE ( 'NONE', ( #928 ), #39265, .F. ) ;
#42806=CARTESIAN_POINT ( 'NONE',  ( 97.30629616937498838, -208.6684592857803011, 74.93197916753381094 ) ) ;
#42808=CARTESIAN_POINT ( 'NONE',  ( 97.65000000000000568, 88.47002178664752137, 79.46958333333331836 ) ) ;
#42810=VERTEX_POINT ( 'NONE', #70033 ) ;
#42814=CARTESIAN_POINT ( 'NONE',  ( -95.00000000000002842, 93.05995642670504253, 89.28562500173430294 ) ) ;
#42817=CARTESIAN_POINT ( 'NONE',  ( 92.35000000000002274, -208.4700217866474645, 84.94645833506763211 ) ) ;
#42818=CARTESIAN_POINT ( 'NONE',  ( 96.32499999999997442, 92.29496732002878900, 85.34333333333333371 ) ) ;
#42821=CARTESIAN_POINT ( 'NONE',  ( 93.67499999999998295, 92.29496732002878900, 81.08354166840096866 ) ) ;
#42824=CARTESIAN_POINT ( 'NONE',  ( -92.69370383062504004, 90.00000000000004263, 86.30906250086715659 ) ) ;
#42825=CARTESIAN_POINT ( 'NONE',  ( 94.99999999999998579, 92.66308142843935514, 81.22906250086715829 ) ) ;
#42827=CARTESIAN_POINT ( 'NONE',  ( 92.34999999999999432, 88.47002178664753558, 83.78229166840095843 ) ) ;
#42830=CARTESIAN_POINT ( 'NONE',  ( -92.34999999999990905, -211.5299782133523934, 86.45458333333331780 ) ) ;
#42834=VERTEX_POINT ( 'NONE', #41475 ) ;
#42836=CARTESIAN_POINT ( 'NONE',  ( 92.35000000005783249, 89.99998877583867340, 75.47473230081648410 ) ) ;
#42837=CARTESIAN_POINT ( 'NONE',  ( -95.00000000000002842, 86.94004357329504273, 83.17374999999999829 ) ) ;
#42841=CARTESIAN_POINT ( 'NONE',  ( 92.34999999999999432, 90.00000000000002842, 89.44437500173430067 ) ) ;
#42843=CARTESIAN_POINT ( 'NONE',  ( 92.35000000000000853, -209.9999999999999716, 84.92000000000000171 ) ) ;
#42844=CARTESIAN_POINT ( 'NONE',  ( -97.30629616937495996, -209.9999999999999716, 78.84781250086714977 ) ) ;
#42846=CARTESIAN_POINT ( 'NONE',  ( 2.500000000000029754, 73.00000000000001421, -255.0000000000000000 ) ) ;
#42852=AXIS2_PLACEMENT_3D ( 'NONE', #17381, #18127, #23401 ) ;
#42863=CARTESIAN_POINT ( 'NONE',  ( -92.69370383062502583, 88.66845928578038638, 75.30239583420048177 ) ) ;
#42867=( BOUNDED_CURVE ( )  B_SPLINE_CURVE ( 2, ( #2895, #20886, #32532, #66757, #15246 ),
 .UNSPECIFIED., .F., .F. ) 
 B_SPLINE_CURVE_WITH_KNOTS ( ( 3, 2, 3 ),
 ( 0.9525283480321510288, 0.9595841135600021721, 0.9629953541049922627 ),
 .UNSPECIFIED. ) 
 CURVE ( )  GEOMETRIC_REPRESENTATION_ITEM ( )  RATIONAL_B_SPLINE_CURVE ( ( 1.000000000000000000, 0.8660254037844387076, 1.000000000000000000, 0.9352274998423413255, 0.9330859296547716619 ) ) 
 REPRESENTATION_ITEM ( '' )  );
#42871=CIRCLE ( 'NONE', #52460, 26.50000000000000355 ) ;
#42880=CARTESIAN_POINT ( 'NONE',  ( -92.34999999999999432, -208.4700217866474645, 87.19541666666667368 ) ) ;
#42891=ORIENTED_EDGE ( 'NONE', *, *, #45061, .T. ) ;
#42896=CARTESIAN_POINT ( 'NONE',  ( 93.84685191531251292, -211.9973110713294489, 81.49364583420047836 ) ) ;
#42897=CARTESIAN_POINT ( 'NONE',  ( 92.69370383062501162, -211.3315407142195852, 89.21947916753381946 ) ) ;
#42899=ORIENTED_EDGE ( 'NONE', *, *, #21651, .F. ) ;
#42900=CARTESIAN_POINT ( 'NONE',  ( 95.00000000000000000, -212.6630814284392557, 87.42031250086715488 ) ) ;
#42906=CARTESIAN_POINT ( 'NONE',  ( -92.69370383062502583, 88.66845928578038638, 77.36614583420048064 ) ) ;
#42907=ORIENTED_EDGE ( 'NONE', *, *, #21034, .T. ) ;
#42914=ORIENTED_EDGE ( 'NONE', *, *, #32179, .T. ) ;
#42921=CARTESIAN_POINT ( 'NONE',  ( 97.30629616937498838, -211.3315407142195852, 77.20739583420046870 ) ) ;
#42923=CARTESIAN_POINT ( 'NONE',  ( -93.67500000000003979, 87.70503267997129626, 81.95666666666666345 ) ) ;
#42931=CARTESIAN_POINT ( 'NONE',  ( -93.67499999999998295, -207.7050326799711968, 88.59770833506763665 ) ) ;
#42933=CARTESIAN_POINT ( 'NONE',  ( -97.30629616937497417, -211.3315407142195852, 80.80572916753382628 ) ) ;
#42935=CARTESIAN_POINT ( 'NONE',  ( -93.84685191531254134, 91.99731107132950569, 77.52489583420047836 ) ) ;
#42937=CARTESIAN_POINT ( 'NONE',  ( 96.15314808468748708, 88.00268892867053694, 80.96447916753380980 ) ) ;
#42944=CARTESIAN_POINT ( 'NONE',  ( -97.30629616937497417, -208.6684592857803295, 81.33489583420048064 ) ) ;
#42955=CARTESIAN_POINT ( 'NONE',  ( -92.35000000000003695, 90.00000000000004263, 75.71250000000000568 ) ) ;
#42957=CARTESIAN_POINT ( 'NONE',  ( -97.30629616937501680, 90.00000000000004263, 85.19781250086714408 ) ) ;
#42958=CARTESIAN_POINT ( 'NONE',  ( -97.45337789172090481, -209.5154774236565061, 74.90854212414869551 ) ) ;
#42960=DIRECTION ( 'NONE',  ( -1.000000000000000000, -0.000000000000000000, -0.000000000000000000 ) ) ;
#42966=CARTESIAN_POINT ( 'NONE',  ( -97.64996285368390261, 91.52999965978816022, 82.40645685155122635 ) ) ;
#42968=DIRECTION ( 'NONE',  ( -0.000000000000000000, -0.000000000000000000, 1.000000000000000000 ) ) ;
#42971=CARTESIAN_POINT ( 'NONE',  ( -97.30629616937497417, -211.3315407142195852, 83.50447916753383026 ) ) ;
#42975=CARTESIAN_POINT ( 'NONE',  ( 97.30629616937498838, 90.00000000000002842, 74.87906250086714977 ) ) ;
#42988=CARTESIAN_POINT ( 'NONE',  ( 93.84685191531249870, -208.0026889286704943, 88.42572916753381662 ) ) ;
#42994=EDGE_LOOP ( 'NONE', ( #39117, #7307, #2940, #70727 ) ) ;
#43000=LINE ( 'NONE', #66305, #59920 ) ;
#43003=CARTESIAN_POINT ( 'NONE',  ( 96.15314808468748708, 88.00268892867053694, 81.12322916753382174 ) ) ;
#43008=ORIENTED_EDGE ( 'NONE', *, *, #68143, .F. ) ;
#43020=CARTESIAN_POINT ( 'NONE',  ( 97.64999999999999147, 90.00000000000002842, 90.00000000000000000 ) ) ;
#43023=CARTESIAN_POINT ( 'NONE',  ( -97.30629616937495996, -209.9999999999999716, 89.64281250086713726 ) ) ;
#43024=CARTESIAN_POINT ( 'NONE',  ( -93.84685191531254134, 91.99731107132950569, 89.58989583420049030 ) ) ;
#43026=CARTESIAN_POINT ( 'NONE',  ( 94.99999999999998579, 86.94004357329500010, 77.53812500173428646 ) ) ;
#43027=CARTESIAN_POINT ( 'NONE',  ( -93.84685191531252713, 88.00268892867056536, 89.21947916753380525 ) ) ;
#43029=CARTESIAN_POINT ( 'NONE',  ( 96.15314808468748708, 91.99731107132950569, 76.25489583420049655 ) ) ;
#43031=CYLINDRICAL_SURFACE ( 'NONE', #59487, 2.649999999999985700 ) ;
#43033=CARTESIAN_POINT ( 'NONE',  ( -97.64999999989197477, 90.00001510551047090, 78.64888723592453346 ) ) ;
#43036=ORIENTED_EDGE ( 'NONE', *, *, #19005, .T. ) ;
#43038=CARTESIAN_POINT ( 'NONE',  ( -93.67499999999998295, -212.2949673200287179, 80.05166666666666231 ) ) ;
#43050=LINE ( 'NONE', #20839, #12301 ) ;
#43053=CARTESIAN_POINT ( 'NONE',  ( -97.30629616937497417, -211.3315407142195852, 75.24947916753383481 ) ) ;
#43066=EDGE_CURVE ( 'NONE', #9907, #55876, #54967, .T. ) ;
#43070=CARTESIAN_POINT ( 'NONE',  ( 97.30629616937498838, 90.00000000000002842, 83.13406250086715943 ) ) ;
#43073=CARTESIAN_POINT ( 'NONE',  ( -92.69370383062498320, -211.3315407142195852, 84.35114583420050849 ) ) ;
#43077=CARTESIAN_POINT ( 'NONE',  ( -93.67499999999998295, -212.2949673200287179, 78.78166666666666629 ) ) ;
#43083=CARTESIAN_POINT ( 'NONE',  ( 95.00000000000000000, -212.6630814284392557, 83.45156250086714067 ) ) ;
#43095=CARTESIAN_POINT ( 'NONE',  ( 96.15314808468748708, -208.0026889286704943, 77.52489583420047836 ) ) ;
#43097=DIRECTION ( 'NONE',  ( -0.000000000000000000, -0.000000000000000000, 1.000000000000000000 ) ) ;
#43100=( BOUNDED_CURVE ( )  B_SPLINE_CURVE ( 2, ( #34615, #35368, #11317, #74096, #57192, #63582, #40266, #22233, #62856 ),
 .UNSPECIFIED., .F., .F. ) 
 B_SPLINE_CURVE_WITH_KNOTS ( ( 3, 2, 2, 2, 3 ),
 ( 0.2751748541904413536, 0.2822306216352944430, 0.2892863871761764960, 0.2963421527170586045, 0.2963422021981254040 ),
 .UNSPECIFIED. ) 
 CURVE ( )  GEOMETRIC_REPRESENTATION_ITEM ( )  RATIONAL_B_SPLINE_CURVE ( ( 1.000000000000000000, 0.8660254037844387076, 1.000000000000000000, 0.8660254037844387076, 1.000000000000000000, 0.8660254037844387076, 1.000000000000000000, 0.9999990604554662710, 0.9999981209241102231 ) ) 
 REPRESENTATION_ITEM ( '' )  );
#43102=CARTESIAN_POINT ( 'NONE',  ( 92.35000000000002274, -211.5299782133524502, 80.52791666666665549 ) ) ;
#43108=CARTESIAN_POINT ( 'NONE',  ( -92.69370383062502583, 91.33154071421968467, 85.09197916753380753 ) ) ;
#43112=DIRECTION ( 'NONE',  ( 1.000000000000000000, 0.000000000000000000, 0.000000000000000000 ) ) ;
#43116=CARTESIAN_POINT ( 'NONE',  ( -96.32499999999996021, -212.2949673200287179, 87.64520833506762187 ) ) ;
#43121=CARTESIAN_POINT ( 'NONE',  ( -93.67500000000003979, 92.29496732002878900, 87.96270833506763154 ) ) ;
#43124=CARTESIAN_POINT ( 'NONE',  ( 92.69370383062498320, 91.33154071421968467, 85.30364583420048064 ) ) ;
#43127=EDGE_CURVE ( 'NONE', #61999, #7767, #55342, .T. ) ;
#43134=ORIENTED_EDGE ( 'NONE', *, *, #70463, .F. ) ;
#43137=EDGE_LOOP ( 'NONE', ( #59075, #3532 ) ) ;
#43142=CARTESIAN_POINT ( 'NONE',  ( -96.15314808468747287, -208.0026889286704943, 84.61572916753381435 ) ) ;
#43145=CARTESIAN_POINT ( 'NONE',  ( -99.99999999999997158, -214.9999999999999716, 90.00000000000000000 ) ) ;
#43154=CARTESIAN_POINT ( 'NONE',  ( 92.69370383062498320, 90.00000000000002842, 78.21281250086714465 ) ) ;
#43163=ADVANCED_FACE ( 'NONE', ( #14380 ), #10216, .F. ) ;
#43170=B_SPLINE_CURVE_WITH_KNOTS ( 'NONE', 1,
 ( #46562, #28898 ),
 .UNSPECIFIED., .F., .F.,
 ( 2, 2 ),
 ( 0.000000000000000000, 1.000000000000000000 ),
 .UNSPECIFIED. ) ;
#43171=CARTESIAN_POINT ( 'NONE',  ( -95.00000000000002842, 87.33691857156074434, 82.81656250086712134 ) ) ;
#43176=CARTESIAN_POINT ( 'NONE',  ( -97.65000000000001990, 90.00000000000004263, 90.00000000000000000 ) ) ;
#43182=CARTESIAN_POINT ( 'NONE',  ( 92.69370383062501162, -211.3315407142195852, 79.05947916753382287 ) ) ;
#43190=ORIENTED_EDGE ( 'NONE', *, *, #19825, .F. ) ;
#43192=CARTESIAN_POINT ( 'NONE',  ( 92.69370383062501162, -208.6684592857803011, 77.68364583420047609 ) ) ;
#43193=CIRCLE ( 'NONE', #13110, 15.70000000000000284 ) ;
#43195=CARTESIAN_POINT ( 'NONE',  ( 97.64999999999999147, 90.00000000000002842, 90.00000000000000000 ) ) ;
#43198=CARTESIAN_POINT ( 'NONE',  ( -97.65000000000010516, 88.47002178664759242, 83.06791666666666174 ) ) ;
#43200=VECTOR ( 'NONE', #22411, 1000.000000000000000 ) ;
#43202=EDGE_CURVE ( 'NONE', #66290, #29385, #54607, .T. ) ;
#43206=CARTESIAN_POINT ( 'NONE',  ( 93.67500000000001137, -207.7050326799711968, 81.71854166840095957 ) ) ;
#43207=CARTESIAN_POINT ( 'NONE',  ( 96.32499999999997442, 92.29496732002878900, 84.70833333333332860 ) ) ;
#43208=EDGE_CURVE ( 'NONE', #58563, #18479, #24635, .T. ) ;
#43214=CARTESIAN_POINT ( 'NONE',  ( -97.30629616937501680, 88.66845928578038638, 87.31447916753381833 ) ) ;
#43215=CARTESIAN_POINT ( 'NONE',  ( 92.69370383062498320, 91.33154071421968467, 81.33489583420048064 ) ) ;
#43217=CARTESIAN_POINT ( 'NONE',  ( 94.99999999999998579, 86.94004357329500010, 82.61812500173428475 ) ) ;
#43222=CARTESIAN_POINT ( 'NONE',  ( 95.00000000000000000, -213.0599564267049857, 78.09374999999998579 ) ) ;
#43228=CARTESIAN_POINT ( 'NONE',  ( -96.32500000000001705, 87.70503267997129626, 84.39083333333333314 ) ) ;
#43233=DIRECTION ( 'NONE',  ( 0.000000000000000000, 0.000000000000000000, 1.000000000000000000 ) ) ;
#43234=CARTESIAN_POINT ( 'NONE',  ( -94.99999999999997158, -212.6630814284392557, 77.73656250086713726 ) ) ;
#43237=CYLINDRICAL_SURFACE ( 'NONE', #9828, 15.69999999999999929 ) ;
#43242=AXIS2_PLACEMENT_3D ( 'NONE', #64855, #36634, #42657 ) ;
#43244=CARTESIAN_POINT ( 'NONE',  ( 97.64998666484373757, -208.4700140875914087, 83.46479220096851748 ) ) ;
#43247=CARTESIAN_POINT ( 'NONE',  ( 93.84685191531248449, 91.99731107132950569, 88.90197916753380980 ) ) ;
#43248=CARTESIAN_POINT ( 'NONE',  ( -97.65000000000003411, -211.5299782133523934, 85.60791666666665378 ) ) ;
#43252=CARTESIAN_POINT ( 'NONE',  ( -97.30629616937501680, 91.33154071421968467, 76.25489583420049655 ) ) ;
#43255=FACE_OUTER_BOUND ( 'NONE', #22659, .T. ) ;
#43256=EDGE_CURVE ( 'NONE', #51311, #14366, #57944, .T. ) ;
#43260=AXIS2_PLACEMENT_3D ( 'NONE', #71939, #20453, #2088 ) ;
#43263=CARTESIAN_POINT ( 'NONE',  ( 97.64999999999999147, -209.9999999999999716, 77.61749999999999261 ) ) ;
#43265=CARTESIAN_POINT ( 'NONE',  ( -92.34999999999999432, -211.5299782133524502, 88.99458333333333826 ) ) ;
#43280=CARTESIAN_POINT ( 'NONE',  ( 95.00000000000000000, -207.3369185715606307, 80.59406250086715318 ) ) ;
#43281=CARTESIAN_POINT ( 'NONE',  ( 92.69370383062501162, -208.6684592857803295, 85.30364583420048064 ) ) ;
#43283=CARTESIAN_POINT ( 'NONE',  ( 92.69370383062501162, -208.6684592857803011, 85.93864583420048575 ) ) ;
#43288=CARTESIAN_POINT ( 'NONE',  ( -93.84685191531254134, 91.99731107132950569, 78.15989583420049769 ) ) ;
#43300=ORIENTED_EDGE ( 'NONE', *, *, #58478, .F. ) ;
#43301=CARTESIAN_POINT ( 'NONE',  ( 92.35000000000000853, -209.9999627172523162, 81.18937371225271704 ) ) ;
#43302=VERTEX_POINT ( 'NONE', #108 ) ;
#43307=CARTESIAN_POINT ( 'NONE',  ( 95.00000000000000000, -207.3369185715606307, 78.05406250086714692 ) ) ;
#43311=VERTEX_POINT ( 'NONE', #39170 ) ;
#43318=CARTESIAN_POINT ( 'NONE',  ( -97.30629616937501680, 91.33154071421968467, 80.22364583420048234 ) ) ;
#43319=ORIENTED_EDGE ( 'NONE', *, *, #65447, .F. ) ;
#43321=CARTESIAN_POINT ( 'NONE',  ( 96.15314808468748708, 88.00268892867053694, 76.51947916753380241 ) ) ;
#43322=( BOUNDED_CURVE ( )  B_SPLINE_CURVE ( 2, ( #60610, #53480, #71490, #19990, #53112, #13617, #36922 ),
 .UNSPECIFIED., .F., .F. ) 
 B_SPLINE_CURVE_WITH_KNOTS ( ( 3, 2, 2, 3 ),
 ( 0.02083333333333322115, 0.02777777777777762705, 0.03472222222222204335, 0.04166666666666644231 ),
 .UNSPECIFIED. ) 
 CURVE ( )  GEOMETRIC_REPRESENTATION_ITEM ( )  RATIONAL_B_SPLINE_CURVE ( ( 1.000000000000002220, 0.8660254037844365982, 1.000000000000000000, 0.8660254037844387076, 1.000000000000000000, 0.8660254037844430375, 0.9999999999999956701 ) ) 
 REPRESENTATION_ITEM ( '' )  );
#43326=CARTESIAN_POINT ( 'NONE',  ( 96.91640186574962001, 88.16968857444116736, 74.99954695036821306 ) ) ;
#43331=CARTESIAN_POINT ( 'NONE',  ( -96.15314808468747287, -208.0026889286704943, 84.45697916753380241 ) ) ;
#43341=CARTESIAN_POINT ( 'NONE',  ( -95.00000000000002842, 92.66308142843932671, 85.03906250086714635 ) ) ;
#43342=CARTESIAN_POINT ( 'NONE',  ( -96.73564493164495559, -208.2604367189442200, 74.87701898318920257 ) ) ;
#43345=ORIENTED_EDGE ( 'NONE', *, *, #2840, .T. ) ;
#43352=FACE_OUTER_BOUND ( 'NONE', #25583, .T. ) ;
#43355=CARTESIAN_POINT ( 'NONE',  ( -93.84685191531247028, -211.9973110713294489, 83.02822916753380866 ) ) ;
#43359=CARTESIAN_POINT ( 'NONE',  ( 92.34999999999999432, 90.00000000000002842, 88.73000000000000398 ) ) ;
#43362=LINE ( 'NONE', #59906, #1729 ) ;
#43385=CARTESIAN_POINT ( 'NONE',  ( 94.99999999999998579, 90.00000000000002842, 90.00000000000000000 ) ) ;
#43386=EDGE_LOOP ( 'NONE', ( #8453, #72712, #50385, #27733 ) ) ;
#43387=PRODUCT_DEFINITION_SHAPE ( 'NONE', 'NONE',  #63750 ) ;
#43390=CARTESIAN_POINT ( 'NONE',  ( 96.15314808468748708, 88.00268892867053694, 76.67822916753381435 ) ) ;
#43392=LINE ( 'NONE', #9149, #30833 ) ;
#43394=EDGE_LOOP ( 'NONE', ( #1899, #9331, #72904, #26811 ) ) ;
#43395=AXIS2_PLACEMENT_3D ( 'NONE', #48320, #71232, #19735 ) ;
#43398=CARTESIAN_POINT ( 'NONE',  ( 97.30629616937498838, 91.33154071421968467, 88.74322916753379786 ) ) ;
#43401=CARTESIAN_POINT ( 'NONE',  ( 92.69370383062501162, -209.9999999999999716, 89.00781250086714635 ) ) ;
#43403=CARTESIAN_POINT ( 'NONE',  ( 96.32499999999997442, 92.29496732002878900, 84.07333333333333769 ) ) ;
#43404=CARTESIAN_POINT ( 'NONE',  ( -97.49696879394610960, 90.24436280099767771, 74.91343443312149475 ) ) ;
#43410=CARTESIAN_POINT ( 'NONE',  ( -94.99999999999997158, -207.3369185715606307, 89.48406250086713953 ) ) ;
#43411=CARTESIAN_POINT ( 'NONE',  ( -97.30629616937501680, 90.00000000000004263, 88.53156250086716739 ) ) ;
#43414=CARTESIAN_POINT ( 'NONE',  ( 96.15314808468748708, 88.00268892867053694, 87.31447916753380412 ) ) ;
#43415=CARTESIAN_POINT ( 'NONE',  ( -92.69370383062504004, 90.00000000000004263, 89.32531250086714181 ) ) ;
#43417=CARTESIAN_POINT ( 'NONE',  ( 93.84685191531248449, 88.00268892867053694, 76.57239583420049200 ) ) ;
#43418=CARTESIAN_POINT ( 'NONE',  ( 97.64999999999999147, 90.00000000000002842, 82.06250000000000000 ) ) ;
#43419=CARTESIAN_POINT ( 'NONE',  ( 93.67500000000001137, -212.2949673200287179, 87.56583333333333030 ) ) ;
#43421=CARTESIAN_POINT ( 'NONE',  ( -92.35000000018069954, 89.99996905681452120, 78.33187387208522523 ) ) ;
#43423=CARTESIAN_POINT ( 'NONE',  ( -96.32499999999996021, -212.2949673200287179, 79.94583333333332575 ) ) ;
#43435=CARTESIAN_POINT ( 'NONE',  ( -97.64999999950680376, -210.0000320386661485, 83.73041644189096644 ) ) ;
#43438=CARTESIAN_POINT ( 'NONE',  ( 97.65000000000000568, 88.47002178664753558, 84.54958333333334508 ) ) ;
#43440=CARTESIAN_POINT ( 'NONE',  ( -92.69370383062504004, 90.00000000000004263, 81.70531250086713726 ) ) ;
#43447=CARTESIAN_POINT ( 'NONE',  ( 97.64999999999999147, -209.9999998456624155, 79.60187500750917877 ) ) ;
#43450=CARTESIAN_POINT ( 'NONE',  ( 97.30629616937498838, 90.00000000000002842, 79.32406250086715715 ) ) ;
#43451=CARTESIAN_POINT ( 'NONE',  ( -93.84685191531247028, -211.9973110713294489, 83.66322916753382799 ) ) ;
#43457=CARTESIAN_POINT ( 'NONE',  ( -97.64999999999996305, -209.9999999999999716, 79.20499999999999829 ) ) ;
#43458=CARTESIAN_POINT ( 'NONE',  ( 95.00000000000000000, -206.9400435732949575, 78.41125000000000966 ) ) ;
#43460=CARTESIAN_POINT ( 'NONE',  ( 95.00000000000000000, -207.3369185715606307, 83.76906250086713612 ) ) ;
#43462=CIRCLE ( 'NONE', #49442, 15.70000000000000284 ) ;
#43475=CARTESIAN_POINT ( 'NONE',  ( 97.30629616937498838, -208.6684592857803295, 77.47197916753381719 ) ) ;
#43478=CARTESIAN_POINT ( 'NONE',  ( -97.50728577674146891, 89.65937732759918788, 74.92458348457971340 ) ) ;
#43481=DIRECTION ( 'NONE',  ( 1.000000000000000000, 0.000000000000000000, 0.000000000000000000 ) ) ;
#43482=CARTESIAN_POINT ( 'NONE',  ( 92.35000000000002274, -208.4700217866474645, 82.32708333333332007 ) ) ;
#43486=ORIENTED_EDGE ( 'NONE', *, *, #47771, .T. ) ;
#43487=CARTESIAN_POINT ( 'NONE',  ( 92.35000000000006537, -211.5299782133524218, 86.87791666666664980 ) ) ;
#43488=CARTESIAN_POINT ( 'NONE',  ( -92.69370383062504004, 90.00000000000004263, 85.03906250086714635 ) ) ;
#43491=CARTESIAN_POINT ( 'NONE',  ( 94.99999999999998579, 86.94004357329500010, 76.18874999999999886 ) ) ;
#43495=CARTESIAN_POINT ( 'NONE',  ( -92.34999999999999432, -208.4700217866474645, 84.73479166840097321 ) ) ;
#43500=CARTESIAN_POINT ( 'NONE',  ( -92.35000000000003695, 90.00000000000004263, 82.14187500173429157 ) ) ;
#43503=CARTESIAN_POINT ( 'NONE',  ( 92.69370383062498320, 90.00000000000002842, 87.26156250086715715 ) ) ;
#43517=ORIENTED_EDGE ( 'NONE', *, *, #1834, .T. ) ;
#43523=CARTESIAN_POINT ( 'NONE',  ( -96.15314808468747287, -208.0026889286704943, 83.98072916753382344 ) ) ;
#43526=ORIENTED_EDGE ( 'NONE', *, *, #64244, .F. ) ;
#43528=CIRCLE ( 'NONE', #62749, 23.50000000000000355 ) ;
#43531=CARTESIAN_POINT ( 'NONE',  ( 96.15314808468748708, 91.99731107132950569, 79.27114583420046756 ) ) ;
#43533=CARTESIAN_POINT ( 'NONE',  ( 94.99999999999998579, 93.05995642670504253, 86.74562500173429669 ) ) ;
#43537=CARTESIAN_POINT ( 'NONE',  ( 92.35000000000000853, -209.9999999999999716, 84.28499999999999659 ) ) ;
#43539=CARTESIAN_POINT ( 'NONE',  ( 97.64999999999999147, 90.00000000000002842, 89.04749999999999943 ) ) ;
#43541=CARTESIAN_POINT ( 'NONE',  ( -96.15314808468751551, 88.00268892867056536, 84.03364583420047040 ) ) ;
#43546=( BOUNDED_CURVE ( )  B_SPLINE_CURVE ( 2, ( #53663, #70938, #2200, #42389, #13793, #36737, #46921, #69835, #3670 ),
 .UNSPECIFIED., .F., .F. ) 
 B_SPLINE_CURVE_WITH_KNOTS ( ( 3, 2, 2, 2, 3 ),
 ( 0.9313609857393202462, 0.9313610513964741822, 0.9384168169373561241, 0.9454725824782379551, 0.9525283480321510288 ),
 .UNSPECIFIED. ) 
 CURVE ( )  GEOMETRIC_REPRESENTATION_ITEM ( )  RATIONAL_B_SPLINE_CURVE ( ( 0.9999975066323323336, 0.9999987533045651134, 1.000000000000000000, 0.8660254037844387076, 1.000000000000000000, 0.8660254037844387076, 1.000000000000000000, 0.8660254037844387076, 1.000000000000000000 ) ) 
 REPRESENTATION_ITEM ( '' )  );
#43549=CARTESIAN_POINT ( 'NONE',  ( 96.66135172262724495, 88.39919842643632819, 74.79754476654878204 ) ) ;
#43553=CARTESIAN_POINT ( 'NONE',  ( 92.69370383062501162, -211.3315407142195852, 78.42447916753380355 ) ) ;
#43561=FACE_BOUND ( 'NONE', #59558, .T. ) ;
#43565=CARTESIAN_POINT ( 'NONE',  ( 93.84685191531249870, -208.0026889286704943, 76.36072916753381890 ) ) ;
#43569=CIRCLE ( 'NONE', #14727, 3.299999999999983391 ) ;
#43576=CARTESIAN_POINT ( 'NONE',  ( 93.67500000000001137, -212.2949673200287179, 80.02520833506763154 ) ) ;
#43577=CARTESIAN_POINT ( 'NONE',  ( 92.34999999999999432, 88.47002178664753558, 85.60791666666665378 ) ) ;
#43581=EDGE_CURVE ( 'NONE', #64357, #18753, #37237, .T. ) ;
#43582=CARTESIAN_POINT ( 'NONE',  ( 92.35000000052950497, 90.00003365185392568, 81.18829462297337329 ) ) ;
#43585=CARTESIAN_POINT ( 'NONE',  ( -93.84685191531252713, 88.00268892867056536, 84.29822916753381890 ) ) ;
#43586=CARTESIAN_POINT ( 'NONE',  ( 92.69370383062498320, 88.66845928578037217, 82.71072916753379900 ) ) ;
#43593=ORIENTED_EDGE ( 'NONE', *, *, #54355, .T. ) ;
#43594=DIRECTION ( 'NONE',  ( 0.000000000000000000, -0.000000000000000000, -1.000000000000000000 ) ) ;
#43596=CARTESIAN_POINT ( 'NONE',  ( 94.99999999999998579, 90.00000000000002842, 90.00000000000000000 ) ) ;
#43600=FACE_OUTER_BOUND ( 'NONE', #64735, .T. ) ;
#43601=CARTESIAN_POINT ( 'NONE',  ( -92.69370383062498320, -211.3315407142195852, 80.38239583420049428 ) ) ;
#43603=CARTESIAN_POINT ( 'NONE',  ( -96.32500000000001705, 87.70503267997129626, 86.29583333333333428 ) ) ;
#43609=VECTOR ( 'NONE', #62330, 1000.000000000000000 ) ;
#43611=CARTESIAN_POINT ( 'NONE',  ( 94.99999999999998579, 87.33691857156068750, 87.89656250086713385 ) ) ;
#43614=CARTESIAN_POINT ( 'NONE',  ( -97.65000000000001990, 91.52997821335253548, 88.75645833506762017 ) ) ;
#43617=CARTESIAN_POINT ( 'NONE',  ( -97.65000000000001990, 88.47002178664754979, 87.59229166840096070 ) ) ;
#43622=ADVANCED_FACE ( 'NONE', ( #45010 ), #59797, .F. ) ;
#43626=CYLINDRICAL_SURFACE ( 'NONE', #18424, 2.649999999999985700 ) ;
#43627=CARTESIAN_POINT ( 'NONE',  ( -93.67499999999998295, -207.7050326799711968, 87.24833333333333485 ) ) ;
#43635=EDGE_CURVE ( 'NONE', #32074, #24150, #63081, .T. ) ;
#43643=CARTESIAN_POINT ( 'NONE',  ( 95.00000000000000000, -212.6630814284392557, 80.91156250086714863 ) ) ;
#43644=CARTESIAN_POINT ( 'NONE',  ( 97.30629616937498838, -211.3315407142195852, 83.71614583420048916 ) ) ;
#43646=ORIENTED_EDGE ( 'NONE', *, *, #27041, .T. ) ;
#43647=CARTESIAN_POINT ( 'NONE',  ( 92.69370383062501162, -211.3315407142195852, 87.31447916753381833 ) ) ;
#43650=EDGE_LOOP ( 'NONE', ( #52, #57884, #39477, #51597 ) ) ;
#43651=CARTESIAN_POINT ( 'NONE',  ( -92.69370383062502583, 91.33154071421968467, 76.83697916753382628 ) ) ;
#43653=ORIENTED_EDGE ( 'NONE', *, *, #70111, .T. ) ;
#43660=VERTEX_POINT ( 'NONE', #53875 ) ;
#43663=AXIS2_PLACEMENT_3D ( 'NONE', #23311, #51876, #34576 ) ;
#43664=ORIENTED_EDGE ( 'NONE', *, *, #63076, .T. ) ;
#43665=CARTESIAN_POINT ( 'NONE',  ( 92.35000000052950497, -209.9999663481461027, 81.18829462297289012 ) ) ;
#43672=CARTESIAN_POINT ( 'NONE',  ( 95.00000000000000000, -212.6630814284392557, 77.73656250086713726 ) ) ;
#43675=VERTEX_POINT ( 'NONE', #1678 ) ;
#43676=ORIENTED_EDGE ( 'NONE', *, *, #5722, .F. ) ;
#43680=CARTESIAN_POINT ( 'NONE',  ( -92.69370383062504004, 90.00000000000004263, 78.05406250086716113 ) ) ;
#43682=CARTESIAN_POINT ( 'NONE',  ( 96.15314808468748708, 91.99731107132950569, 79.27114583420046756 ) ) ;
#43685=CARTESIAN_POINT ( 'NONE',  ( -94.99999999999997158, -207.3369185715606307, 89.48406250086713953 ) ) ;
#43689=CARTESIAN_POINT ( 'NONE',  ( -96.15314808468747287, -208.0026889286704943, 81.28197916753380525 ) ) ;
#43699=CARTESIAN_POINT ( 'NONE',  ( -93.84685191531252713, 88.00268892867056536, 85.40947916753380298 ) ) ;
#43713=CARTESIAN_POINT ( 'NONE',  ( -93.84685191531248449, -208.0026889286704943, 83.23989583420049598 ) ) ;
#43716=CARTESIAN_POINT ( 'NONE',  ( -97.64999999999996305, -211.5299782133524218, 86.95729166840096980 ) ) ;
#43725=CARTESIAN_POINT ( 'NONE',  ( 93.67500000000001137, -207.7050326799711968, 79.73416666666666686 ) ) ;
#43726=VECTOR ( 'NONE', #21588, 1000.000000000000000 ) ;
#43732=EDGE_CURVE ( 'NONE', #32439, #23087, #48606, .T. ) ;
#43734=CARTESIAN_POINT ( 'NONE',  ( 92.35000000000000853, -209.9999999999999716, 75.39499999999999602 ) ) ;
#43747=VERTEX_POINT ( 'NONE', #35834 ) ;
#43751=( BOUNDED_CURVE ( )  B_SPLINE_CURVE ( 2, ( #4820, #10054, #23201, #40118, #39756, #62707, #39378 ),
 .UNSPECIFIED., .F., .F. ) 
 B_SPLINE_CURVE_WITH_KNOTS ( ( 3, 2, 2, 3 ),
 ( 0.2328402629019980796, 0.2398960283900005708, 0.2469517939308829568, 0.2540073681283129825 ),
 .UNSPECIFIED. ) 
 CURVE ( )  GEOMETRIC_REPRESENTATION_ITEM ( )  RATIONAL_B_SPLINE_CURVE ( ( 1.000000000000000000, 0.8660254037844387076, 1.000000000000000000, 0.8660254037844387076, 1.000000000000000000, 0.8660290370063220555, 0.9999927337532901195 ) ) 
 REPRESENTATION_ITEM ( '' )  );
#43752=CARTESIAN_POINT ( 'NONE',  ( 93.84685191531248449, 91.99731107132950569, 75.09072916753380866 ) ) ;
#43754=CARTESIAN_POINT ( 'NONE',  ( -97.65000000000006253, 88.47002178664754979, 84.97291666666667709 ) ) ;
#43756=ORIENTED_EDGE ( 'NONE', *, *, #4341, .T. ) ;
#43758=CARTESIAN_POINT ( 'NONE',  ( 92.69370383062498320, 91.33154071421968467, 88.95489583420048518 ) ) ;
#43760=CARTESIAN_POINT ( 'NONE',  ( 97.30629616937498838, -208.6684592857803011, 88.10822916753380696 ) ) ;
#43765=DIRECTION ( 'NONE',  ( -1.000000000000000000, 0.000000000000000000, 0.000000000000000000 ) ) ;
#43768=CARTESIAN_POINT ( 'NONE',  ( -97.64999999999996305, -209.9999999999999716, 76.74437500173429783 ) ) ;
#43769=CARTESIAN_POINT ( 'NONE',  ( -96.15314808468752972, 91.99731107132950569, 89.06072916753382174 ) ) ;
#43772=CARTESIAN_POINT ( 'NONE',  ( 93.84685191531248449, 88.00268892867053694, 87.84364583420047268 ) ) ;
#43773=CARTESIAN_POINT ( 'NONE',  ( -92.69370383062502583, 88.66845928578038638, 86.73239583420047438 ) ) ;
#43780=CARTESIAN_POINT ( 'NONE',  ( 97.65000000000000568, 91.52997821335252127, 82.19479166840095274 ) ) ;
#43790=CARTESIAN_POINT ( 'NONE',  ( -96.32500000000001705, 87.70503267997129626, 79.94583333333332575 ) ) ;
#43797=CARTESIAN_POINT ( 'NONE',  ( -92.69370383062498320, -211.3315407142195852, 75.46114583420049371 ) ) ;
#43799=CARTESIAN_POINT ( 'NONE',  ( -97.30629616937501680, 91.33154071421968467, 81.96989583420048575 ) ) ;
#43808=CARTESIAN_POINT ( 'NONE',  ( -97.64999999999996305, -208.4700217866474645, 87.40708333333333258 ) ) ;
#43812=CARTESIAN_POINT ( 'NONE',  ( 97.30629616937498838, 91.33154071421968467, 81.91697916753383879 ) ) ;
#43813=CARTESIAN_POINT ( 'NONE',  ( -93.84685191531248449, -208.0026889286704943, 82.60489583420049087 ) ) ;
#43818=CARTESIAN_POINT ( 'NONE',  ( -94.99999999999997158, -206.9400435732949575, 77.14124999999999943 ) ) ;
#43819=CARTESIAN_POINT ( 'NONE',  ( 95.00000000000000000, -209.9999999999999716, 90.00000000000000000 ) ) ;
#43821=CARTESIAN_POINT ( 'NONE',  ( -97.30629616937501680, 88.66845928578038638, 77.15447916753382174 ) ) ;
#43822=CARTESIAN_POINT ( 'NONE',  ( 97.30629616937498838, -208.6684592857803011, 83.02822916753379445 ) ) ;
#43834=CARTESIAN_POINT ( 'NONE',  ( 97.30629616937498838, -209.9999999999999716, 76.78406250086715090 ) ) ;
#43839=CARTESIAN_POINT ( 'NONE',  ( 93.84685191531248449, 88.00268892867053694, 86.09739583420049769 ) ) ;
#43840=CARTESIAN_POINT ( 'NONE',  ( -97.64999999953499810, 89.99996900126896548, 83.09538598081491045 ) ) ;
#43841=CARTESIAN_POINT ( 'NONE',  ( 95.00000000000000000, -213.0599564267049857, 81.90374999999998806 ) ) ;
#43848=CARTESIAN_POINT ( 'NONE',  ( -92.69370383062502583, 88.66845928578038638, 83.08114583420048405 ) ) ;
#43850=CARTESIAN_POINT ( 'NONE',  ( -97.64999999999992042, -208.4700217866474929, 77.24708333333332178 ) ) ;
#43853=CARTESIAN_POINT ( 'NONE',  ( -94.99999999999997158, -213.0599564267049857, 83.88812500173429498 ) ) ;
#43854=ORIENTED_EDGE ( 'NONE', *, *, #2229, .F. ) ;
#43855=CARTESIAN_POINT ( 'NONE',  ( -92.34999999999999432, -211.5299782133524502, 87.16895833506762870 ) ) ;
#43858=ORIENTED_EDGE ( 'NONE', *, *, #49580, .T. ) ;
#43859=CARTESIAN_POINT ( 'NONE',  ( -97.65000000000001990, 91.52997821335253548, 83.04145833506763097 ) ) ;
#43861=CARTESIAN_POINT ( 'NONE',  ( 93.84685191531248449, 88.00268892867053694, 86.73239583420048859 ) ) ;
#43866=DIRECTION ( 'NONE',  ( 1.000000000000000000, 0.000000000000000000, 0.000000000000000000 ) ) ;
#43868=CARTESIAN_POINT ( 'NONE',  ( 92.35000000000009379, -208.4700217866474361, 77.88208333333332689 ) ) ;
#43876=CARTESIAN_POINT ( 'NONE',  ( -94.99999999999997158, -212.6630814284392557, 85.51531250086713953 ) ) ;
#43879=DIRECTION ( 'NONE',  ( 1.000000000000000000, 0.000000000000000000, 0.000000000000000000 ) ) ;
#43888=CARTESIAN_POINT ( 'NONE',  ( 93.84685191531248449, 88.00268892867053694, 78.31864583420048120 ) ) ;
#43897=CARTESIAN_POINT ( 'NONE',  ( -97.64999999999989200, -211.5299782133524218, 86.87791666666664980 ) ) ;
#43898=CARTESIAN_POINT ( 'NONE',  ( -92.74366017909918014, -209.4495095149826511, 74.79348190356849102 ) ) ;
#43901=EDGE_LOOP ( 'NONE', ( #25691, #51118, #13569, #14700 ) ) ;
#43902=CARTESIAN_POINT ( 'NONE',  ( -95.00000000000002842, 87.33691857156074434, 81.54656250086713953 ) ) ;
#43909=FACE_OUTER_BOUND ( 'NONE', #3246, .T. ) ;
#43915=CARTESIAN_POINT ( 'NONE',  ( 96.15314808468750130, -211.9973110713294489, 77.31322916753381946 ) ) ;
#43916=VERTEX_POINT ( 'NONE', #4984 ) ;
#43919=DIRECTION ( 'NONE',  ( 1.000000000000000000, 0.000000000000000000, -0.000000000000000000 ) ) ;
#43922=AXIS2_PLACEMENT_3D ( 'NONE', #49400, #32098, #47922 ) ;
#43924=CARTESIAN_POINT ( 'NONE',  ( 92.69370383062501162, -209.9999999999999716, 77.73656250086715147 ) ) ;
#43936=CARTESIAN_POINT ( 'NONE',  ( 96.32499999999998863, -212.2949673200287179, 80.13104166840095388 ) ) ;
#43937=CARTESIAN_POINT ( 'NONE',  ( 97.64999999999997726, 88.47002178664753558, 84.54958333333333087 ) ) ;
#43944=CARTESIAN_POINT ( 'NONE',  ( 92.34999999999999432, 91.52997821335252127, 84.31145833506762699 ) ) ;
#43945=CARTESIAN_POINT ( 'NONE',  ( -96.15314808468751551, 88.00268892867056536, 84.82739583420048746 ) ) ;
#43946=CARTESIAN_POINT ( 'NONE',  ( 94.99999999999998579, 87.33691857156068750, 81.54656250086715374 ) ) ;
#43948=CYLINDRICAL_SURFACE ( 'NONE', #27653, 2.649999999999985700 ) ;
#43953=CARTESIAN_POINT ( 'NONE',  ( 94.99999999999998579, 86.94004357329502852, 79.99874999999998693 ) ) ;
#43956=( BOUNDED_CURVE ( )  B_SPLINE_CURVE ( 2, ( #29990, #52187, #735, #52935, #6702, #63135, #18708, #36004, #17247 ),
 .UNSPECIFIED., .F., .F. ) 
 B_SPLINE_CURVE_WITH_KNOTS ( ( 3, 2, 2, 2, 3 ),
 ( 0.3810111478265171270, 0.3810113392076479588, 0.3880671047485307334, 0.3951228702894135636, 0.4021785743327777052 ),
 .UNSPECIFIED. ) 
 CURVE ( )  GEOMETRIC_REPRESENTATION_ITEM ( )  RATIONAL_B_SPLINE_CURVE ( ( 0.9999927323224930831, 0.9999963660626793871, 1.000000000000000000, 0.8660254037844387076, 1.000000000000000000, 0.8660254037844387076, 1.000000000000000000, 0.8660265714968831130, 0.9999976645954666843 ) ) 
 REPRESENTATION_ITEM ( '' )  );
#43959=DIRECTION ( 'NONE',  ( -0.000000000000000000, -0.000000000000000000, 1.000000000000000000 ) ) ;
#43960=CARTESIAN_POINT ( 'NONE',  ( -92.69370383062498320, -209.9999999999999716, 77.89531250086714920 ) ) ;
#43965=CARTESIAN_POINT ( 'NONE',  ( -92.34999999999999432, -209.9999999999999716, 89.12687500173430521 ) ) ;
#43970=CARTESIAN_POINT ( 'NONE',  ( 94.99999999999998579, 87.33691857156068750, 86.62656250086713783 ) ) ;
#43981=CYLINDRICAL_SURFACE ( 'NONE', #50838, 2.649999999999985700 ) ;
#43982=DIRECTION ( 'NONE',  ( -0.000000000000000000, -0.000000000000000000, 1.000000000000000000 ) ) ;
#43983=CARTESIAN_POINT ( 'NONE',  ( 97.64999999999999147, 90.00000000000002842, 80.79249999999998977 ) ) ;
#43985=CARTESIAN_POINT ( 'NONE',  ( -94.99999999999997158, -213.0599564267049857, 85.07874999999999943 ) ) ;
#43987=ADVANCED_FACE ( 'NONE', ( #23010 ), #46666, .F. ) ;
#43993=DIRECTION ( 'NONE',  ( 0.000000000000000000, -0.000000000000000000, -1.000000000000000000 ) ) ;
#44004=CARTESIAN_POINT ( 'NONE',  ( 96.15314808468748708, -208.0026889286704943, 83.08114583420048405 ) ) ;
#44005=CARTESIAN_POINT ( 'NONE',  ( 97.30629616937498838, -208.6684592857803295, 85.09197916753380753 ) ) ;
#44007=CARTESIAN_POINT ( 'NONE',  ( 92.69370383062501162, -209.9999999999999716, 85.99156250086716113 ) ) ;
#44011=CARTESIAN_POINT ( 'NONE',  ( -96.15314808468752972, 91.99731107132950569, 76.36072916753381890 ) ) ;
#44016=EDGE_LOOP ( 'NONE', ( #68617, #25334, #27812, #48641 ) ) ;
#44038=CARTESIAN_POINT ( 'NONE',  ( 92.35000000000000853, -209.9999999999999716, 90.00000000000000000 ) ) ;
#44040=CARTESIAN_POINT ( 'NONE',  ( -93.84685191531252713, 88.00268892867056536, 76.04322916753382344 ) ) ;
#44043=CARTESIAN_POINT ( 'NONE',  ( 93.84685191531248449, 88.00268892867053694, 78.31864583420048120 ) ) ;
#44046=CARTESIAN_POINT ( 'NONE',  ( -96.15314808468747287, -208.0026889286704943, 88.90197916753380980 ) ) ;
#44050=CARTESIAN_POINT ( 'NONE',  ( -93.84685191531247028, -211.9973110713294489, 80.96447916753380980 ) ) ;
#44054=CARTESIAN_POINT ( 'NONE',  ( -93.67499999999998295, -207.7050326799711968, 84.07333333333333769 ) ) ;
#44057=CARTESIAN_POINT ( 'NONE',  ( 100.0010000000000190, -123.9999999999999858, 39.99999999999996447 ) ) ;
#44059=AXIS2_PLACEMENT_3D ( 'NONE', #68986, #17474, #11816 ) ;
#44060=CARTESIAN_POINT ( 'NONE',  ( -96.15314808468751551, 88.00268892867056536, 80.85864583420047325 ) ) ;
#44070=CARTESIAN_POINT ( 'NONE',  ( -92.69370383062498320, -211.3315407142195852, 81.81114583420048803 ) ) ;
#44083=CARTESIAN_POINT ( 'NONE',  ( 92.35000000000000853, -209.9999999999999716, 79.83999999999998920 ) ) ;
#44103=ORIENTED_EDGE ( 'NONE', *, *, #15261, .T. ) ;
#44105=CARTESIAN_POINT ( 'NONE',  ( 96.15314808468748708, 88.00268892867053694, 77.94822916753382458 ) ) ;
#44111=CARTESIAN_POINT ( 'NONE',  ( 96.15314808468748708, 91.99731107132950569, 88.79614583420047325 ) ) ;
#44113=CARTESIAN_POINT ( 'NONE',  ( 92.69370383062501162, -209.9999999999999716, 85.83281250086714920 ) ) ;
#44115=CARTESIAN_POINT ( 'NONE',  ( -96.32500000000001705, 92.29496732002878900, 77.27354166840096639 ) ) ;
#44119=CARTESIAN_POINT ( 'NONE',  ( 94.99999999999998579, 90.00000000000002842, 90.00000000000000000 ) ) ;
#44121=CARTESIAN_POINT ( 'NONE',  ( -94.99999999999997158, -207.3369185715606307, 88.21406250086714351 ) ) ;
#44122=EDGE_CURVE ( 'NONE', #69246, #44776, #19561, .T. ) ;
#44123=CARTESIAN_POINT ( 'NONE',  ( -93.84685191531254134, 91.99731107132950569, 84.50989583420049200 ) ) ;
#44126=CARTESIAN_POINT ( 'NONE',  ( 92.69370383062498320, 90.00000000000002842, 87.73781250086713612 ) ) ;
#44127=CARTESIAN_POINT ( 'NONE',  ( -97.30629616937501680, 90.00000000000004263, 87.10281250086714522 ) ) ;
#44129=CARTESIAN_POINT ( 'NONE',  ( 92.35002600533573514, -211.5299932275399897, 84.41729270697884147 ) ) ;
#44141=VECTOR ( 'NONE', #6, 1000.000000000000000 ) ;
#44144=CARTESIAN_POINT ( 'NONE',  ( -95.00000000000002842, 93.05995642670501411, 81.58624999999999261 ) ) ;
#44150=CARTESIAN_POINT ( 'NONE',  ( -92.35000000000003695, 89.99999989488615881, 86.58687499784845443 ) ) ;
#44153=EDGE_LOOP ( 'NONE', ( #41155, #70103, #43517, #11948 ) ) ;
#44154=CARTESIAN_POINT ( 'NONE',  ( -95.00000000000002842, 87.33691857156074434, 80.91156250086714863 ) ) ;
#44155=CARTESIAN_POINT ( 'NONE',  ( 93.67499999999999716, 87.70503267997126784, 82.56520833506762358 ) ) ;
#44160=CARTESIAN_POINT ( 'NONE',  ( -92.34999999999999432, -209.9999999999999716, 87.14249999999999829 ) ) ;
#44169=CARTESIAN_POINT ( 'NONE',  ( 97.30629616937498838, 88.66845928578035796, 81.17614583420049712 ) ) ;
#44170=CARTESIAN_POINT ( 'NONE',  ( -92.69370383062498320, -209.9999999999999716, 84.40406250086715545 ) ) ;
#44173=CARTESIAN_POINT ( 'NONE',  ( -94.99999999999997158, -213.0599564267049857, 77.45874999999999488 ) ) ;
#44175=CARTESIAN_POINT ( 'NONE',  ( -96.15314808468752972, 91.99731107132950569, 78.26572916753382003 ) ) ;
#44176=CARTESIAN_POINT ( 'NONE',  ( 92.69370383062501162, -208.6684592857803011, 84.50989583420046358 ) ) ;
#44177=VERTEX_POINT ( 'NONE', #48512 ) ;
#44178=CARTESIAN_POINT ( 'NONE',  ( 96.85456758451087467, 88.62117599715715244, 74.79348190356851944 ) ) ;
#44180=( BOUNDED_CURVE ( )  B_SPLINE_CURVE ( 2, ( #69357, #18227, #5853, #17852, #12211, #29863, #63736, #6586, #17120, #57343, #7325 ),
 .UNSPECIFIED., .F., .F. ) 
 B_SPLINE_CURVE_WITH_KNOTS ( ( 3, 2, 2, 2, 2, 3 ),
 ( 0.1481709449575358828, 0.1481710763585298851, 0.1552268418994119104, 0.1622826074402939078, 0.1693383729811759331, 0.1693384224419982043 ),
 .UNSPECIFIED. ) 
 CURVE ( )  GEOMETRIC_REPRESENTATION_ITEM ( )  RATIONAL_B_SPLINE_CURVE ( ( 0.9999950100192072089, 0.9999975049631379953, 1.000000000000000000, 0.8660254037844387076, 1.000000000000000000, 0.8660254037844387076, 1.000000000000000000, 0.8660254037844387076, 1.000000000000000000, 0.9999990608398684477, 0.9999981216929038075 ) ) 
 REPRESENTATION_ITEM ( '' )  );
#44186=CARTESIAN_POINT ( 'NONE',  ( -96.32499999999996021, -207.7050326799711968, 83.54416666666666913 ) ) ;
#44187=AXIS2_PLACEMENT_3D ( 'NONE', #67820, #15194, #16316 ) ;
#44189=VERTEX_POINT ( 'NONE', #41041 ) ;
#44192=CYLINDRICAL_SURFACE ( 'NONE', #18917, 2.649999999999985700 ) ;
#44195=DIRECTION ( 'NONE',  ( 1.000000000000000000, 0.000000000000000000, 0.000000000000000000 ) ) ;
#44196=CARTESIAN_POINT ( 'NONE',  ( 94.99999999999998579, 87.33691857156068750, 88.05531250086716000 ) ) ;
#44197=CARTESIAN_POINT ( 'NONE',  ( 92.34999999999999432, 90.00000000000002842, 80.55437500173430010 ) ) ;
#44198=CARTESIAN_POINT ( 'NONE',  ( 92.35000000000000853, -209.9999999999999716, 78.57000000000000739 ) ) ;
#44202=VERTEX_POINT ( 'NONE', #13553 ) ;
#44209=AXIS2_PLACEMENT_3D ( 'NONE', #64562, #11938, #13041 ) ;
#44211=EDGE_CURVE ( 'NONE', #21245, #2928, #3197, .T. ) ;
#44213=AXIS2_PLACEMENT_3D ( 'NONE', #16352, #61487, #15976 ) ;
#44217=CARTESIAN_POINT ( 'NONE',  ( -93.67499999999998295, -212.2949673200287179, 85.21104166840096639 ) ) ;
#44221=CARTESIAN_POINT ( 'NONE',  ( -92.35000000000005116, 88.47002178664754979, 84.62895833506763665 ) ) ;
#44224=CARTESIAN_POINT ( 'NONE',  ( 96.15314808468748708, 91.99731107132950569, 81.96989583420048575 ) ) ;
#44240=CARTESIAN_POINT ( 'NONE',  ( -97.30629616937497417, -211.3315407142195852, 85.40947916753380298 ) ) ;
#44247=CARTESIAN_POINT ( 'NONE',  ( -15.70044424985254850, 0.001194404164626844313, -85.59999999999999432 ) ) ;
#44249=CARTESIAN_POINT ( 'NONE',  ( 92.69370383062498320, 88.66845928578035796, 78.26572916753380582 ) ) ;
#44254=CARTESIAN_POINT ( 'NONE',  ( 92.48632958231164025, 89.99999999999990052, 74.91808492278045151 ) ) ;
#44263=ORIENTED_EDGE ( 'NONE', *, *, #35393, .T. ) ;
#44264=CARTESIAN_POINT ( 'NONE',  ( -95.00000000000002842, 92.66308142843932671, 84.40406250086714124 ) ) ;
#44269=DIRECTION ( 'NONE',  ( -1.000000000000000000, 0.000000000000000000, 0.000000000000000000 ) ) ;
#44276=CARTESIAN_POINT ( 'NONE',  ( 97.30629616937498838, -211.3315407142195852, 79.90614583420048689 ) ) ;
#44284=CARTESIAN_POINT ( 'NONE',  ( 95.00000000000000000, -212.6630814284392557, 76.62531250086715318 ) ) ;
#44293=CARTESIAN_POINT ( 'NONE',  ( -96.32500000000001705, 92.29496732002878900, 89.33854166840096411 ) ) ;
#44296=CARTESIAN_POINT ( 'NONE',  ( 94.99999999999998579, 86.94004357329502852, 87.61874999999999147 ) ) ;
#44297=CARTESIAN_POINT ( 'NONE',  ( 92.35000000000000853, -209.9999999999999716, 78.64937500173429896 ) ) ;
#44299=CARTESIAN_POINT ( 'NONE',  ( 96.32499999999997442, 92.29496732002878900, 83.43833333333333258 ) ) ;
#44300=ORIENTED_EDGE ( 'NONE', *, *, #40685, .F. ) ;
#44306=CARTESIAN_POINT ( 'NONE',  ( -92.69370383062505425, 91.33154071421968467, 85.09197916753380753 ) ) ;
#44307=CARTESIAN_POINT ( 'NONE',  ( 92.69370383062498320, 90.00000000000002842, 79.48281250086714067 ) ) ;
#44316=CARTESIAN_POINT ( 'NONE',  ( -92.69370383062498320, -208.6684592857803011, 82.39322916753381776 ) ) ;
#44317=AXIS2_PLACEMENT_3D ( 'NONE', #42451, #65388, #8226 ) ;
#44324=CARTESIAN_POINT ( 'NONE',  ( -92.34999999999999432, -210.0000000207151629, 80.87187500099602744 ) ) ;
#44326=CARTESIAN_POINT ( 'NONE',  ( 94.99999999999998579, 86.94004357329500010, 88.96812500173430749 ) ) ;
#44328=CARTESIAN_POINT ( 'NONE',  ( -93.84685191531248449, -208.0026889286704943, 79.90614583420047268 ) ) ;
#44334=CARTESIAN_POINT ( 'NONE',  ( -93.67500000000003979, 87.70503267997129626, 81.32166666666667254 ) ) ;
#44338=CARTESIAN_POINT ( 'NONE',  ( 93.84685191531248449, 88.00268892867053694, 87.84364583420047268 ) ) ;
#44345=CARTESIAN_POINT ( 'NONE',  ( -92.35000000000003695, 89.99999996655868983, 87.85687500050293863 ) ) ;
#44349=DIRECTION ( 'NONE',  ( -0.000000000000000000, -0.000000000000000000, 1.000000000000000000 ) ) ;
#44356=CARTESIAN_POINT ( 'NONE',  ( -97.64999999999994884, -208.4700217866474645, 86.13708333333332234 ) ) ;
#44358=CARTESIAN_POINT ( 'NONE',  ( 7.103376864691351012E-17, -120.0000000000000000, -80.00000000000000000 ) ) ;
#44363=AXIS2_PLACEMENT_3D ( 'NONE', #16871, #73249, #39431 ) ;
#44366=CARTESIAN_POINT ( 'NONE',  ( 95.00000000000000000, -212.6630814284392557, 88.69031250086716511 ) ) ;
#44367=ORIENTED_EDGE ( 'NONE', *, *, #59406, .T. ) ;
#44369=EDGE_LOOP ( 'NONE', ( #43653, #1001, #56589, #47153 ) ) ;
#44374=CARTESIAN_POINT ( 'NONE',  ( 95.00000000000000000, -207.3369185715606307, 79.32406250086714294 ) ) ;
#44375=CARTESIAN_POINT ( 'NONE',  ( 92.69370383062501162, -211.3315407142195852, 86.04447916753382231 ) ) ;
#44377=CARTESIAN_POINT ( 'NONE',  ( 92.69370383062501162, -211.3315407142195852, 86.04447916753382231 ) ) ;
#44387=CARTESIAN_POINT ( 'NONE',  ( 96.32499999999997442, 92.29496732002878900, 87.96270833506763154 ) ) ;
#44388=CARTESIAN_POINT ( 'NONE',  ( 95.00000000000000000, -213.0599564267049857, 88.96812500173430749 ) ) ;
#44392=ORIENTED_EDGE ( 'NONE', *, *, #68849, .F. ) ;
#44393=( BOUNDED_CURVE ( )  B_SPLINE_CURVE ( 2, ( #12981, #64506, #1021, #47580, #23914, #41207, #46854, #53226, #37695 ),
 .UNSPECIFIED., .F., .F. ) 
 B_SPLINE_CURVE_WITH_KNOTS ( ( 3, 2, 2, 2, 3 ),
 ( 0.2116728463006668226, 0.2116729662264711376, 0.2187287317673534959, 0.2257844973082358264, 0.2328402629019979686 ),
 .UNSPECIFIED. ) 
 CURVE ( )  GEOMETRIC_REPRESENTATION_ITEM ( )  RATIONAL_B_SPLINE_CURVE ( ( 0.9999954457845777744, 0.9999977228535845697, 1.000000000000000000, 0.8660254037844387076, 1.000000000000000000, 0.8660254037844387076, 1.000000000000000000, 0.8660254037844387076, 1.000000000000000000 ) ) 
 REPRESENTATION_ITEM ( '' )  );
#44397=ORIENTED_EDGE ( 'NONE', *, *, #1486, .F. ) ;
#44409=VERTEX_POINT ( 'NONE', #39467 ) ;
#44411=CARTESIAN_POINT ( 'NONE',  ( -92.34999999999999432, -209.9999999999999716, 88.41249999999999432 ) ) ;
#44413=CARTESIAN_POINT ( 'NONE',  ( -97.65000000000001990, 90.00000000000004263, 89.36499999999999488 ) ) ;
#44416=CARTESIAN_POINT ( 'NONE',  ( 93.84685191531248449, 91.99731107132950569, 77.47197916753380298 ) ) ;
#44418=CARTESIAN_POINT ( 'NONE',  ( -94.99999999999997158, -209.9999999999999716, 90.00000000000000000 ) ) ;
#44419=CARTESIAN_POINT ( 'NONE',  ( -97.30629616937497417, -208.6684592857803011, 88.31989583420046586 ) ) ;
#44422=LINE ( 'NONE', #32742, #58402 ) ;
#44424=CARTESIAN_POINT ( 'NONE',  ( -96.15314808468745866, -211.9973110713294489, 80.85864583420047325 ) ) ;
#44429=CARTESIAN_POINT ( 'NONE',  ( -92.35000000000006537, -208.4700217866474361, 84.02041666666666231 ) ) ;
#44439=CARTESIAN_POINT ( 'NONE',  ( -94.99999999999997158, -213.0599564267049857, 88.88875000000000171 ) ) ;
#44440=CARTESIAN_POINT ( 'NONE',  ( 96.40521225739051658, -208.1321859400968606, 74.80441578173235939 ) ) ;
#44441=CARTESIAN_POINT ( 'NONE',  ( -92.69370383062502583, 91.33154071421968467, 80.48822916753383083 ) ) ;
#44450=CARTESIAN_POINT ( 'NONE',  ( -92.69370383062498320, -208.6684592857803011, 79.37697916753381833 ) ) ;
#44454=CARTESIAN_POINT ( 'NONE',  ( 96.32499999999997442, 92.29496732002878900, 76.53270833506762472 ) ) ;
#44457=CARTESIAN_POINT ( 'NONE',  ( 92.34999999999999432, 90.00000000000002842, 77.37937500173428873 ) ) ;
#44469=EDGE_CURVE ( 'NONE', #41714, #32656, #66369, .T. ) ;
#44470=CARTESIAN_POINT ( 'NONE',  ( 92.69370383062501162, -211.3315407142195852, 89.06072916753382174 ) ) ;
#44471=CARTESIAN_POINT ( 'NONE',  ( 95.00000000000000000, -206.9400435732949575, 86.03125000000000000 ) ) ;
#44477=CARTESIAN_POINT ( 'NONE',  ( -92.35000000000003695, 90.00000000000004263, 88.41249999999999432 ) ) ;
#44480=CARTESIAN_POINT ( 'NONE',  ( 93.67500000000001137, -212.2949673200287179, 81.85083333333332689 ) ) ;
#44490=CARTESIAN_POINT ( 'NONE',  ( 92.69370383062498320, 90.00000000000002842, 76.46656250086715545 ) ) ;
#44494=VERTEX_POINT ( 'NONE', #39090 ) ;
#44497=CARTESIAN_POINT ( 'NONE',  ( 96.15314808468748708, 88.00268892867053694, 87.94947916753380923 ) ) ;
#44499=CARTESIAN_POINT ( 'NONE',  ( 96.15314808468750130, -211.9973110713294489, 85.40947916753380298 ) ) ;
#44501=DIRECTION ( 'NONE',  ( 1.000000000000000000, 0.000000000000000000, 0.000000000000000000 ) ) ;
#44506=CARTESIAN_POINT ( 'NONE',  ( -92.69370383062498320, -208.6684592857803011, 88.74322916753379786 ) ) ;
#44508=CARTESIAN_POINT ( 'NONE',  ( -95.00000000000002842, 87.33691857156074434, 87.42031250086715488 ) ) ;
#44511=CARTESIAN_POINT ( 'NONE',  ( 92.69370383062498320, 88.66845928578037217, 88.42572916753380241 ) ) ;
#44512=CARTESIAN_POINT ( 'NONE',  ( -97.30629616937501680, 90.00000000000004263, 86.46781250086714010 ) ) ;
#44518=CARTESIAN_POINT ( 'NONE',  ( -93.67500000000003979, 92.29496732002878900, 86.61333333333332973 ) ) ;
#44519=CARTESIAN_POINT ( 'NONE',  ( 95.00000000000000000, -206.9400435732949575, 82.22124999999999773 ) ) ;
#44522=CARTESIAN_POINT ( 'NONE',  ( 94.99999999999998579, 86.94004357329502852, 89.52374999999999261 ) ) ;
#44525=CARTESIAN_POINT ( 'NONE',  ( -93.67500000000003979, 92.29496732002878900, 80.89833333333332632 ) ) ;
#44534=CARTESIAN_POINT ( 'NONE',  ( -96.15314808468751551, 88.00268892867056536, 83.39864583420047950 ) ) ;
#44538=CARTESIAN_POINT ( 'NONE',  ( -92.35000000000015064, 88.47002178664750716, 85.81958333333332689 ) ) ;
#44541=CARTESIAN_POINT ( 'NONE',  ( 89.99999999999998579, 85.00000000000002842, 90.00000000000000000 ) ) ;
#44545=( BOUNDED_CURVE ( )  B_SPLINE_CURVE ( 2, ( #11212, #67988, #63112, #34140, #57087, #22880, #68740 ),
 .UNSPECIFIED., .F., .F. ) 
 B_SPLINE_CURVE_WITH_KNOTS ( ( 3, 2, 2, 3 ),
 ( 0.7916666666666669627, 0.7986111111111114935, 0.8055555555555558023, 0.8125000000000002220 ),
 .UNSPECIFIED. ) 
 CURVE ( )  GEOMETRIC_REPRESENTATION_ITEM ( )  RATIONAL_B_SPLINE_CURVE ( ( 0.9999999999999935607, 0.8660254037844451469, 1.000000000000000000, 0.8660254037844387076, 1.000000000000000000, 0.8660254037844343777, 1.000000000000004219 ) ) 
 REPRESENTATION_ITEM ( '' )  );
#44548=CARTESIAN_POINT ( 'NONE',  ( 94.99999999999998579, 92.66308142843932671, 80.75281250086716511 ) ) ;
#44549=CARTESIAN_POINT ( 'NONE',  ( -94.99999999999997158, -207.3369185715606307, 84.56281250086716739 ) ) ;
#44551=ORIENTED_EDGE ( 'NONE', *, *, #20343, .T. ) ;
#44552=CARTESIAN_POINT ( 'NONE',  ( -97.65000000000001990, 91.52997821335253548, 83.04145833506764518 ) ) ;
#44553=CARTESIAN_POINT ( 'NONE',  ( -94.99999999999997158, -213.0599564267049857, 78.72875000000001933 ) ) ;
#44556=CARTESIAN_POINT ( 'NONE',  ( -95.00000000000002842, 92.66308142843932671, 78.84781250086714977 ) ) ;
#44557=CARTESIAN_POINT ( 'NONE',  ( 95.00000000000000000, -212.6630814284392557, 80.91156250086714863 ) ) ;
#44566=VECTOR ( 'NONE', #41914, 1000.000000000000000 ) ;
#44572=LINE ( 'NONE', #55842, #53961 ) ;
#44573=ORIENTED_EDGE ( 'NONE', *, *, #26377, .T. ) ;
#44576=CARTESIAN_POINT ( 'NONE',  ( 97.65000000000006253, -211.5299782133524218, 83.91458333333333997 ) ) ;
#44577=CARTESIAN_POINT ( 'NONE',  ( 94.99999999999998579, 87.33691857156068750, 86.15031250086714465 ) ) ;
#44579=CARTESIAN_POINT ( 'NONE',  ( 97.65000000000000568, 88.47002178664752137, 80.81895833506763438 ) ) ;
#44580=CARTESIAN_POINT ( 'NONE',  ( 92.35000000000002274, -208.4700217866474645, 79.15208333333332291 ) ) ;
#44584=ORIENTED_EDGE ( 'NONE', *, *, #55860, .F. ) ;
#44591=AXIS2_PLACEMENT_3D ( 'NONE', #31763, #66006, #66372 ) ;
#44593=CYLINDRICAL_SURFACE ( 'NONE', #11944, 2.649999999999985700 ) ;
#44596=CARTESIAN_POINT ( 'NONE',  ( -94.99999999999997158, -213.0599564267049857, 82.61812500173428475 ) ) ;
#44600=ORIENTED_EDGE ( 'NONE', *, *, #23923, .F. ) ;
#44601=CARTESIAN_POINT ( 'NONE',  ( 97.64999999999997726, 88.47002178664753558, 82.72395833506762131 ) ) ;
#44602=CARTESIAN_POINT ( 'NONE',  ( -96.32500000000001705, 87.70503267997129626, 83.20020833506764291 ) ) ;
#44605=EDGE_CURVE ( 'NONE', #33726, #2166, #59715, .T. ) ;
#44606=CARTESIAN_POINT ( 'NONE',  ( 97.30629616937498838, 88.66845928578037217, 83.08114583420048405 ) ) ;
#44607=CARTESIAN_POINT ( 'NONE',  ( -96.32500000000001705, 87.70503267997129626, 76.13583333333333769 ) ) ;
#44608=CARTESIAN_POINT ( 'NONE',  ( -97.64999999999996305, -209.9999999999999716, 82.45937500173430124 ) ) ;
#44611=LINE ( 'NONE', #73897, #70894 ) ;
#44620=CARTESIAN_POINT ( 'NONE',  ( -93.67500000000003979, 87.70503267997129626, 80.13104166840095388 ) ) ;
#44621=CARTESIAN_POINT ( 'NONE',  ( -92.35000000000000853, -209.9999996502046429, 77.69687501385436690 ) ) ;
#44622=CARTESIAN_POINT ( 'NONE',  ( -94.99999999999997158, -207.3369185715606307, 81.38781250086715602 ) ) ;
#44624=DIRECTION ( 'NONE',  ( 1.000000000000000000, 0.000000000000000000, 0.000000000000000000 ) ) ;
#44627=DIRECTION ( 'NONE',  ( 1.000000000000000000, 0.000000000000000000, 0.000000000000000000 ) ) ;
#44628=AXIS2_PLACEMENT_3D ( 'NONE', #66088, #15680, #61550 ) ;
#44629=CARTESIAN_POINT ( 'NONE',  ( 97.65000000000000568, 88.47002178664752137, 82.08895833506764461 ) ) ;
#44632=CARTESIAN_POINT ( 'NONE',  ( 97.30629616937498838, 88.66845928578035796, 77.20739583420046870 ) ) ;
#44634=LINE ( 'NONE', #9286, #73412 ) ;
#44636=CARTESIAN_POINT ( 'NONE',  ( -92.35000000000395914, -210.0000045800647115, 76.42687486209126746 ) ) ;
#44640=( BOUNDED_CURVE ( )  B_SPLINE_CURVE ( 2, ( #48375, #14156, #3652, #26177, #48744, #3288, #32183 ),
 .UNSPECIFIED., .F., .F. ) 
 B_SPLINE_CURVE_WITH_KNOTS ( ( 3, 2, 2, 3 ),
 ( 0.3598440426530882807, 0.3668998081258831867, 0.3739555736667656283, 0.3810111478265171270 ),
 .UNSPECIFIED. ) 
 CURVE ( )  GEOMETRIC_REPRESENTATION_ITEM ( )  RATIONAL_B_SPLINE_CURVE ( ( 1.000000000000000000, 0.8660254037844387076, 1.000000000000000000, 0.8660254037844387076, 1.000000000000000000, 0.8660290377217593205, 0.9999927323224930831 ) ) 
 REPRESENTATION_ITEM ( '' )  );
#44642=CARTESIAN_POINT ( 'NONE',  ( 92.69370383062498320, 91.33154071421968467, 89.11364583420049712 ) ) ;
#44644=CARTESIAN_POINT ( 'NONE',  ( 94.99999999999998579, 93.05995642670504253, 89.20624999999999716 ) ) ;
#44647=CARTESIAN_POINT ( 'NONE',  ( -93.84685191531252713, 88.00268892867056536, 84.13947916753380696 ) ) ;
#44653=CARTESIAN_POINT ( 'NONE',  ( 92.35000000000000853, -209.9999999999999716, 90.00000000000000000 ) ) ;
#44654=EDGE_CURVE ( 'NONE', #64184, #61415, #23647, .T. ) ;
#44655=ORIENTED_EDGE ( 'NONE', *, *, #4077, .T. ) ;
#44661=CARTESIAN_POINT ( 'NONE',  ( 92.69370383062501162, -211.3315407142195852, 80.32947916753381890 ) ) ;
#44663=ORIENTED_EDGE ( 'NONE', *, *, #38442, .F. ) ;
#44664=CARTESIAN_POINT ( 'NONE',  ( -97.64998530214792538, -208.4700133008386445, 81.77145774807794965 ) ) ;
#44665=EDGE_CURVE ( 'NONE', #4451, #40893, #45295, .T. ) ;
#44667=DIRECTION ( 'NONE',  ( -1.000000000000000000, 3.061616997868383141E-16, 0.000000000000000000 ) ) ;
#44671=CARTESIAN_POINT ( 'NONE',  ( 92.35000000000002274, -211.5299782133524502, 86.87791666666664980 ) ) ;
#44674=CARTESIAN_POINT ( 'NONE',  ( -97.64999999999996305, -209.9999999999999716, 88.09499999999999886 ) ) ;
#44679=FACE_OUTER_BOUND ( 'NONE', #57920, .T. ) ;
#44680=ORIENTED_EDGE ( 'NONE', *, *, #53988, .F. ) ;
#44681=CARTESIAN_POINT ( 'NONE',  ( 93.67500000000001137, -207.7050326799711968, 78.54354166840096241 ) ) ;
#44682=CARTESIAN_POINT ( 'NONE',  ( 92.35000000000002274, -211.5299782133524502, 80.60729166840097548 ) ) ;
#44683=CARTESIAN_POINT ( 'NONE',  ( 93.67499999999998295, 92.29496732002878900, 81.63916666666666799 ) ) ;
#44692=CARTESIAN_POINT ( 'NONE',  ( -96.15314808468752972, 91.99731107132950569, 85.25072916753381946 ) ) ;
#44693=CARTESIAN_POINT ( 'NONE',  ( 96.15314808468748708, 91.99731107132950569, 78.63614583420047666 ) ) ;
#44694=ORIENTED_EDGE ( 'NONE', *, *, #51838, .F. ) ;
#44696=CARTESIAN_POINT ( 'NONE',  ( -92.35000000000312070, 89.99999595380251094, 77.06187486178039592 ) ) ;
#44703=CARTESIAN_POINT ( 'NONE',  ( -97.30629616937495996, -209.9999999999999716, 81.38781250086714181 ) ) ;
#44704=VERTEX_POINT ( 'NONE', #53693 ) ;
#44705=ORIENTED_EDGE ( 'NONE', *, *, #8766, .T. ) ;
#44707=ORIENTED_EDGE ( 'NONE', *, *, #8831, .T. ) ;
#44709=CARTESIAN_POINT ( 'NONE',  ( 97.64999999999989200, 88.47002178664749295, 80.73958333333335702 ) ) ;
#44711=CARTESIAN_POINT ( 'NONE',  ( -96.15314808468747287, -208.0026889286704943, 76.83697916753381207 ) ) ;
#44715=CARTESIAN_POINT ( 'NONE',  ( 97.64999999999999147, 90.00000000000002842, 89.12687500173430521 ) ) ;
#44720=CARTESIAN_POINT ( 'NONE',  ( 97.30629616937498838, 88.66845928578035796, 88.63739583420047552 ) ) ;
#44721=DIRECTION ( 'NONE',  ( 3.061616997868382648E-16, 1.000000000000000000, 0.000000000000000000 ) ) ;
#44724=CARTESIAN_POINT ( 'NONE',  ( 92.35000000019410038, 89.99998015720535705, 86.27002759516707897 ) ) ;
#44725=DIRECTION ( 'NONE',  ( -0.000000000000000000, -0.000000000000000000, 1.000000000000000000 ) ) ;
#44729=EDGE_CURVE ( 'NONE', #50232, #41327, #71612, .T. ) ;
#44735=CARTESIAN_POINT ( 'NONE',  ( -96.32499999999996021, -207.7050326799711968, 86.08416666666666117 ) ) ;
#44739=CARTESIAN_POINT ( 'NONE',  ( -94.26002770235261607, 87.43182282693500440, 75.00000000000000000 ) ) ;
#44747=CARTESIAN_POINT ( 'NONE',  ( 97.30629616937498838, -211.3315407142195852, 87.52614583420049144 ) ) ;
#44748=VERTEX_POINT ( 'NONE', #71333 ) ;
#44749=EDGE_LOOP ( 'NONE', ( #48843, #18065, #70704, #71675 ) ) ;
#44751=ORIENTED_EDGE ( 'NONE', *, *, #1486, .T. ) ;
#44753=CARTESIAN_POINT ( 'NONE',  ( 95.00000000000000000, -212.6630814284392557, 79.64156250086713840 ) ) ;
#44756=CARTESIAN_POINT ( 'NONE',  ( 92.69370383062501162, -211.3315407142195852, 82.86947916753382515 ) ) ;
#44763=ORIENTED_EDGE ( 'NONE', *, *, #3695, .F. ) ;
#44764=DIRECTION ( 'NONE',  ( -0.000000000000000000, -0.000000000000000000, 1.000000000000000000 ) ) ;
#44766=DIRECTION ( 'NONE',  ( -0.000000000000000000, -0.000000000000000000, 1.000000000000000000 ) ) ;
#44773=VERTEX_POINT ( 'NONE', #31863 ) ;
#44776=VERTEX_POINT ( 'NONE', #14578 ) ;
#44784=CARTESIAN_POINT ( 'NONE',  ( -97.64999999999996305, -209.9999999999999716, 84.28499999999999659 ) ) ;
#44786=CARTESIAN_POINT ( 'NONE',  ( -92.69370383062502583, 91.33154071421968467, 75.56697916753383026 ) ) ;
#44787=ORIENTED_EDGE ( 'NONE', *, *, #214, .T. ) ;
#44788=CARTESIAN_POINT ( 'NONE',  ( 94.99999999999998579, 87.33691857156068750, 77.73656250086713726 ) ) ;
#44790=VERTEX_POINT ( 'NONE', #2612 ) ;
#44792=CARTESIAN_POINT ( 'NONE',  ( -94.99999999999997158, -212.6630814284392557, 85.35656250086714181 ) ) ;
#44796=CYLINDRICAL_SURFACE ( 'NONE', #36878, 2.649999999999999467 ) ;
#44797=CARTESIAN_POINT ( 'NONE',  ( -97.30629616937497417, -208.6684592857803295, 78.15989583420048348 ) ) ;
#44806=CARTESIAN_POINT ( 'NONE',  ( -97.30629616937501680, 88.66845928578038638, 80.17072916753379275 ) ) ;
#44809=VERTEX_POINT ( 'NONE', #25491 ) ;
#44811=ADVANCED_FACE ( 'NONE', ( #37526 ), #57642, .F. ) ;
#44818=CARTESIAN_POINT ( 'NONE',  ( -93.84685191531247028, -211.9973110713294489, 80.48822916753381662 ) ) ;
#44819=EDGE_CURVE ( 'NONE', #4256, #60757, #72087, .T. ) ;
#44823=VERTEX_POINT ( 'NONE', #20597 ) ;
#44825=CARTESIAN_POINT ( 'NONE',  ( -97.65000000000010516, 91.52997821335249284, 88.67708333333332860 ) ) ;
#44829=CARTESIAN_POINT ( 'NONE',  ( 92.34999999999999432, 91.52997821335252127, 77.32645833506762756 ) ) ;
#44838=( BOUNDED_CURVE ( )  B_SPLINE_CURVE ( 2, ( #29124, #52422, #68995, #41525, #6223, #53179, #12936 ),
 .UNSPECIFIED., .F., .F. ) 
 B_SPLINE_CURVE_WITH_KNOTS ( ( 3, 2, 2, 3 ),
 ( 0.1458333333333334536, 0.1527777777777778734, 0.1597222222222222654, 0.1666666666666666852 ),
 .UNSPECIFIED. ) 
 CURVE ( )  GEOMETRIC_REPRESENTATION_ITEM ( )  RATIONAL_B_SPLINE_CURVE ( ( 0.9999999999999978906, 0.8660254037844408170, 1.000000000000000000, 0.8660254037844387076, 1.000000000000000000, 0.8660254037844381525, 1.000000000000000444 ) ) 
 REPRESENTATION_ITEM ( '' )  );
#44839=CARTESIAN_POINT ( 'NONE',  ( 97.30629616937498838, -211.3315407142195852, 87.36739583420047950 ) ) ;
#44840=CARTESIAN_POINT ( 'NONE',  ( -97.65000000000001990, 90.00000000000004263, 77.93499999999998806 ) ) ;
#44844=VERTEX_POINT ( 'NONE', #62318 ) ;
#44851=ADVANCED_FACE ( 'NONE', ( #23198 ), #10801, .F. ) ;
#44852=DIRECTION ( 'NONE',  ( -0.000000000000000000, -0.000000000000000000, 1.000000000000000000 ) ) ;
#44854=VERTEX_POINT ( 'NONE', #16816 ) ;
#44859=CARTESIAN_POINT ( 'NONE',  ( 94.99999999999998579, 87.33691857156068750, 75.35531250086715715 ) ) ;
#44862=ORIENTED_EDGE ( 'NONE', *, *, #35488, .F. ) ;
#44865=CARTESIAN_POINT ( 'NONE',  ( 94.99999999999998579, 92.66308142843935514, 86.94406250086714749 ) ) ;
#44867=CARTESIAN_POINT ( 'NONE',  ( 96.15314808468750130, -211.9973110713294489, 84.77447916753381207 ) ) ;
#44874=CARTESIAN_POINT ( 'NONE',  ( -2.499999999999973355, 65.00000000000000000, -90.00000000000000000 ) ) ;
#44875=CARTESIAN_POINT ( 'NONE',  ( -93.84685191531248449, -208.0026889286704943, 88.79614583420047325 ) ) ;
#44876=CARTESIAN_POINT ( 'NONE',  ( -96.15314808468752972, 91.99731107132950569, 85.25072916753381946 ) ) ;
#44879=CARTESIAN_POINT ( 'NONE',  ( 92.69370383062498320, 90.00000000000002842, 89.00781250086714635 ) ) ;
#44880=CARTESIAN_POINT ( 'NONE',  ( -92.69370383062504004, 90.00000000000004263, 84.88031250086713442 ) ) ;
#44885=CARTESIAN_POINT ( 'NONE',  ( 95.00000000000000000, -209.9999999999999716, 90.00000000000000000 ) ) ;
#44886=CARTESIAN_POINT ( 'NONE',  ( -97.30629616937495996, -209.9999999999999716, 88.37281250086715545 ) ) ;
#44889=CARTESIAN_POINT ( 'NONE',  ( -97.30629616937501680, 88.66845928578038638, 82.23447916753383424 ) ) ;
#44895=ORIENTED_EDGE ( 'NONE', *, *, #18109, .T. ) ;
#44896=CARTESIAN_POINT ( 'NONE',  ( -96.32500000000001705, 87.70503267997129626, 81.85083333333332689 ) ) ;
#44898=CARTESIAN_POINT ( 'NONE',  ( -95.00000000000002842, 86.94004357329504273, 78.72875000000001933 ) ) ;
#44900=CARTESIAN_POINT ( 'NONE',  ( -97.64999999994212487, -210.0000112241608292, 75.47473230080855444 ) ) ;
#44907=CARTESIAN_POINT ( 'NONE',  ( -97.30629616937501680, 88.66845928578038638, 80.17072916753379275 ) ) ;
#44911=CYLINDRICAL_SURFACE ( 'NONE', #11421, 2.649999999999985700 ) ;
#44915=CARTESIAN_POINT ( 'NONE',  ( -92.35000000000003695, 90.00000000000004263, 90.00000000000000000 ) ) ;
#44920=CARTESIAN_POINT ( 'NONE',  ( 93.84685191531248449, 88.00268892867053694, 81.65239583420049030 ) ) ;
#44921=AXIS2_PLACEMENT_3D ( 'NONE', #42285, #3918, #65211 ) ;
#44922=CARTESIAN_POINT ( 'NONE',  ( -92.69370383062498320, -208.6684592857803295, 78.74197916753381321 ) ) ;
#44924=ORIENTED_EDGE ( 'NONE', *, *, #53995, .F. ) ;
#44927=CARTESIAN_POINT ( 'NONE',  ( -97.30629616937501680, 90.00000000000004263, 77.73656250086715147 ) ) ;
#44928=CARTESIAN_POINT ( 'NONE',  ( 97.30629616937498838, -211.3315407142195852, 79.74739583420047495 ) ) ;
#44931=EDGE_CURVE ( 'NONE', #30791, #66690, #70720, .T. ) ;
#44935=CARTESIAN_POINT ( 'NONE',  ( -96.32499999999996021, -207.7050326799711968, 88.06854166840095388 ) ) ;
#44937=DIRECTION ( 'NONE',  ( 0.000000000000000000, 1.000000000000000000, 0.000000000000000000 ) ) ;
#44939=VECTOR ( 'NONE', #42534, 1000.000000000000000 ) ;
#44941=VERTEX_POINT ( 'NONE', #4431 ) ;
#44943=CARTESIAN_POINT ( 'NONE',  ( 93.84685191531249870, -208.0026889286704943, 75.72572916753382799 ) ) ;
#44947=CARTESIAN_POINT ( 'NONE',  ( 92.69370383062498320, 88.66845928578037217, 87.31447916753381833 ) ) ;
#44950=CARTESIAN_POINT ( 'NONE',  ( 97.64999999999997726, -211.5299782133524502, 78.19958333333332234 ) ) ;
#44954=VERTEX_POINT ( 'NONE', #51020 ) ;
#44958=CYLINDRICAL_SURFACE ( 'NONE', #1825, 2.649999999999985700 ) ;
#44959=CARTESIAN_POINT ( 'NONE',  ( -93.67499999999998295, -212.2949673200287179, 88.38604166840097776 ) ) ;
#44962=CARTESIAN_POINT ( 'NONE',  ( -94.99999999999997158, -206.9400435732949575, 84.20562500173429044 ) ) ;
#44967=CARTESIAN_POINT ( 'NONE',  ( 97.64999999999999147, 90.00000000000002842, 82.14187500173429157 ) ) ;
#44968=CARTESIAN_POINT ( 'NONE',  ( -93.67500000000003979, 87.70503267997129626, 82.67104166840096013 ) ) ;
#44970=CARTESIAN_POINT ( 'NONE',  ( 97.30629616937498838, 88.66845928578037217, 84.35114583420049428 ) ) ;
#44974=CIRCLE ( 'NONE', #27021, 23.50000000000000355 ) ;
#44978=ORIENTED_EDGE ( 'NONE', *, *, #25903, .T. ) ;
#44987=CARTESIAN_POINT ( 'NONE',  ( -92.34999999999999432, -209.9999999999999716, 85.87249999999998806 ) ) ;
#44989=CARTESIAN_POINT ( 'NONE',  ( -92.69370383062498320, -208.6684592857803011, 81.91697916753381037 ) ) ;
#44991=CARTESIAN_POINT ( 'NONE',  ( -93.84685191531252713, 88.00268892867056536, 89.21947916753380525 ) ) ;
#44999=CARTESIAN_POINT ( 'NONE',  ( 96.15314808468748708, 91.99731107132950569, 76.09614583420047040 ) ) ;
#45002=CARTESIAN_POINT ( 'NONE',  ( 97.64999999999990621, -209.9999992849081139, 85.31687502647973531 ) ) ;
#45010=FACE_OUTER_BOUND ( 'NONE', #29479, .T. ) ;
#45011=CARTESIAN_POINT ( 'NONE',  ( -92.69370383062498320, -209.9999999999999716, 89.48406250086715374 ) ) ;
#45015=CARTESIAN_POINT ( 'NONE',  ( -96.15314808468752972, 91.99731107132950569, 78.74197916753381321 ) ) ;
#45021=ORIENTED_EDGE ( 'NONE', *, *, #62824, .F. ) ;
#45022=CARTESIAN_POINT ( 'NONE',  ( 92.35000000000002274, -209.9999762675151658, 79.91937418090955703 ) ) ;
#45026=CARTESIAN_POINT ( 'NONE',  ( 96.15314808468748708, -208.0026889286704943, 76.25489583420049655 ) ) ;
#45034=CARTESIAN_POINT ( 'NONE',  ( 92.35000000000000853, -211.5299782133524218, 81.87729166840097150 ) ) ;
#45035=CARTESIAN_POINT ( 'NONE',  ( 97.64999999999997726, -211.5299782133524502, 87.72458333333332803 ) ) ;
#45037=DIRECTION ( 'NONE',  ( 0.000000000000000000, -0.000000000000000000, -1.000000000000000000 ) ) ;
#45043=CARTESIAN_POINT ( 'NONE',  ( -95.00000000000002842, 90.00000000000004263, 90.00000000000000000 ) ) ;
#45046=CARTESIAN_POINT ( 'NONE',  ( 97.64999999999999147, -209.9999999999999716, 75.79187500173429726 ) ) ;
#45047=CARTESIAN_POINT ( 'NONE',  ( 93.67499999999999716, 87.70503267997126784, 81.85083333333332689 ) ) ;
#45054=CARTESIAN_POINT ( 'NONE',  ( -93.84685191531252713, 88.00268892867056536, 86.20322916753382003 ) ) ;
#45056=CARTESIAN_POINT ( 'NONE',  ( 96.15314808468748708, 91.99731107132950569, 79.27114583420046756 ) ) ;
#45061=EDGE_CURVE ( 'NONE', #7474, #65748, #30335, .T. ) ;
#45065=CARTESIAN_POINT ( 'NONE',  ( -97.64999999999989200, -211.5299782133525071, 86.24291666666667311 ) ) ;
#45067=CARTESIAN_POINT ( 'NONE',  ( -92.69370383062498320, -211.3315407142195852, 78.47739583420047893 ) ) ;
#45073=EDGE_CURVE ( 'NONE', #70981, #56782, #60652, .T. ) ;
#45078=( BOUNDED_CURVE ( )  B_SPLINE_CURVE ( 2, ( #68808, #40225, #12379, #36790, #2258, #30768, #13495 ),
 .UNSPECIFIED., .F., .F. ) 
 B_SPLINE_CURVE_WITH_KNOTS ( ( 3, 2, 2, 3 ),
 ( 0.6250000000000003331, 0.6319444444444446418, 0.6388888888888890616, 0.6458333333333334814 ),
 .UNSPECIFIED. ) 
 CURVE ( )  GEOMETRIC_REPRESENTATION_ITEM ( )  RATIONAL_B_SPLINE_CURVE ( ( 0.9999999999999935607, 0.8660254037844451469, 1.000000000000000000, 0.8660254037844387076, 1.000000000000000000, 0.8660254037844365982, 1.000000000000002220 ) ) 
 REPRESENTATION_ITEM ( '' )  );
#45079=CARTESIAN_POINT ( 'NONE',  ( -93.84685191531248449, -208.0026889286704943, 76.73114583420047552 ) ) ;
#45080=EDGE_LOOP ( 'NONE', ( #71494, #67769, #10717, #41632 ) ) ;
#45090=CARTESIAN_POINT ( 'NONE',  ( 92.69370383062498320, 90.00000000000002842, 85.19781250086714408 ) ) ;
#45092=CARTESIAN_POINT ( 'NONE',  ( -97.65000000000001990, 90.00000000000004263, 75.39499999999999602 ) ) ;
#45093=DIRECTION ( 'NONE',  ( -2.628368902995175337E-16, -1.000000000000000000, 0.000000000000000000 ) ) ;
#45102=CARTESIAN_POINT ( 'NONE',  ( -95.00000000000002842, 87.33691857156074434, 88.53156250086716739 ) ) ;
#45105=CARTESIAN_POINT ( 'NONE',  ( -93.67499999999998295, -207.7050326799711968, 85.34333333333333371 ) ) ;
#45111=DIRECTION ( 'NONE',  ( 1.000000000000000000, 0.000000000000000000, 0.000000000000000000 ) ) ;
#45115=CARTESIAN_POINT ( 'NONE',  ( 92.69370383062501162, -211.3315407142195852, 86.04447916753382231 ) ) ;
#45116=VERTEX_POINT ( 'NONE', #63798 ) ;
#45118=ORIENTED_EDGE ( 'NONE', *, *, #57784, .F. ) ;
#45125=CARTESIAN_POINT ( 'NONE',  ( 92.69370383062501162, -211.3315407142195852, 79.53572916753380184 ) ) ;
#45127=CARTESIAN_POINT ( 'NONE',  ( 95.00000000000000000, -207.3369185715606307, 83.92781250086716227 ) ) ;
#45135=CARTESIAN_POINT ( 'NONE',  ( 94.99999999999998579, 93.05995642670504253, 86.03125000000000000 ) ) ;
#45146=CARTESIAN_POINT ( 'NONE',  ( 93.84685191531251292, -211.9973110713294489, 75.77864583420047495 ) ) ;
#45156=CARTESIAN_POINT ( 'NONE',  ( -92.69370383062504004, 90.00000000000004263, 74.87906250086714977 ) ) ;
#45158=CARTESIAN_POINT ( 'NONE',  ( 94.99999999999998579, 87.33691857156068750, 75.19656250086714522 ) ) ;
#45161=CARTESIAN_POINT ( 'NONE',  ( -92.69370383062498320, -211.3315407142195852, 86.09739583420048348 ) ) ;
#45164=AXIS2_PLACEMENT_3D ( 'NONE', #46360, #69288, #40719 ) ;
#45167=CARTESIAN_POINT ( 'NONE',  ( -92.69370383062498320, -209.9999999999999716, 78.53031250086714010 ) ) ;
#45176=CARTESIAN_POINT ( 'NONE',  ( -12.75000000000000000, -120.0000000000000000, -85.60000000000000853 ) ) ;
#45177=CARTESIAN_POINT ( 'NONE',  ( 96.73972734126404305, -208.4859488783623362, 74.79348190356850523 ) ) ;
#45178=CARTESIAN_POINT ( 'NONE',  ( -93.84685191531254134, 91.99731107132950569, 82.44614583420046472 ) ) ;
#45179=CARTESIAN_POINT ( 'NONE',  ( -97.65000000000001990, 90.00000000000004263, 85.55499999999999261 ) ) ;
#45181=VECTOR ( 'NONE', #4220, 1000.000000000000000 ) ;
#45186=CARTESIAN_POINT ( 'NONE',  ( -0.0004442498525516064278, 0.001194404164626844313, -85.59999999999999432 ) ) ;
#45194=CARTESIAN_POINT ( 'NONE',  ( -97.30629616937497417, -208.6684592857803011, 79.58864583420047722 ) ) ;
#45197=ORIENTED_EDGE ( 'NONE', *, *, #50132, .F. ) ;
#45199=CARTESIAN_POINT ( 'NONE',  ( -97.65000000000001990, 90.00001557635633276, 80.55437446300187787 ) ) ;
#45206=EDGE_LOOP ( 'NONE', ( #45118, #46508, #62911, #31518, #58406, #27837, #23680, #2818, #29302, #56484, #6172, #34667, #16277, #62792, #37396, #6482, #45252, #48822, #41535, #60578, #343, #20047, #18569, #59468, #44694, #22076, #21422, #44763, #13678, #3349, #68487, #34938, #54433, #55577, #8156, #6864, #69185, #63109, #26915, #25776, #41259, #40603, #48198, #18508, #13800, #36875, #50551, #8109, #26356, #50630, #28776, #10211 ) ) ;
#45209=EDGE_LOOP ( 'NONE', ( #35483, #53116, #31432, #10179 ) ) ;
#45210=CARTESIAN_POINT ( 'NONE',  ( 95.00000000000000000, -207.3369185715606307, 86.94406250086714749 ) ) ;
#45214=CARTESIAN_POINT ( 'NONE',  ( 95.00000000000000000, -213.0599564267049857, 89.52374999999999261 ) ) ;
#45220=CIRCLE ( 'NONE', #55995, 12.74999999999999822 ) ;
#45229=CARTESIAN_POINT ( 'NONE',  ( 93.67499999999998295, 92.29496732002878900, 87.35416666666665719 ) ) ;
#45236=CARTESIAN_POINT ( 'NONE',  ( 96.15314808468748708, 91.99731107132950569, 85.62114583420046188 ) ) ;
#45238=CARTESIAN_POINT ( 'NONE',  ( 95.00000000000000000, -212.6630814284392557, 86.62656250086715204 ) ) ;
#45243=CARTESIAN_POINT ( 'NONE',  ( -93.67499999999998295, -207.7050326799711968, 80.26333333333332121 ) ) ;
#45247=EDGE_CURVE ( 'NONE', #58433, #41314, #14527, .T. ) ;
#45249=EDGE_CURVE ( 'NONE', #44844, #47502, #58224, .T. ) ;
#45250=CARTESIAN_POINT ( 'NONE',  ( -93.84685191531247028, -211.9973110713294489, 87.31447916753380412 ) ) ;
#45251=CARTESIAN_POINT ( 'NONE',  ( -97.30629616937501680, 88.66845928578038638, 87.31447916753381833 ) ) ;
#45252=ORIENTED_EDGE ( 'NONE', *, *, #5365, .F. ) ;
#45253=CARTESIAN_POINT ( 'NONE',  ( 94.99999999999998579, 92.66308142843935514, 84.40406250086712703 ) ) ;
#45254=CARTESIAN_POINT ( 'NONE',  ( -92.69370383062504004, 90.00000000000004263, 85.51531250086713953 ) ) ;
#45255=ORIENTED_EDGE ( 'NONE', *, *, #7778, .T. ) ;
#45260=CARTESIAN_POINT ( 'NONE',  ( -93.84685191531248449, -208.0026889286704943, 88.16114583420046813 ) ) ;
#45270=CARTESIAN_POINT ( 'NONE',  ( -93.67500000000003979, 87.70503267997129626, 81.95666666666666345 ) ) ;
#45280=CARTESIAN_POINT ( 'NONE',  ( -95.00000000000002842, 87.33691857156074434, 77.73656250086713726 ) ) ;
#45287=VECTOR ( 'NONE', #18150, 1000.000000000000000 ) ;
#45288=DIRECTION ( 'NONE',  ( 0.000000000000000000, 0.000000000000000000, -1.000000000000000000 ) ) ;
#45290=FACE_OUTER_BOUND ( 'NONE', #45206, .T. ) ;
#45295=( BOUNDED_CURVE ( )  B_SPLINE_CURVE ( 2, ( #41308, #29635, #64250, #42057, #13093, #46578, #7092 ),
 .UNSPECIFIED., .F., .F. ) 
 B_SPLINE_CURVE_WITH_KNOTS ( ( 3, 2, 2, 3 ),
 ( 0.8890265259358470784, 0.8960822236920598094, 0.9031379892329425285, 0.9101937466091534201 ),
 .UNSPECIFIED. ) 
 CURVE ( )  GEOMETRIC_REPRESENTATION_ITEM ( )  RATIONAL_B_SPLINE_CURVE ( ( 0.9999974258394741522, 0.8660266908770667404, 1.000000000000000000, 0.8660254037844387076, 1.000000000000000000, 0.8660254037844387076, 1.000000000000000000 ) ) 
 REPRESENTATION_ITEM ( '' )  );
#45296=CARTESIAN_POINT ( 'NONE',  ( 97.30629616937498838, 91.33154071421968467, 76.83697916753382628 ) ) ;
#45297=CARTESIAN_POINT ( 'NONE',  ( -93.84685191531248449, -208.0026889286704943, 79.42989583420049371 ) ) ;
#45301=CARTESIAN_POINT ( 'NONE',  ( -97.64999999999996305, -209.9999999999999716, 76.03000000000000114 ) ) ;
#45304=CARTESIAN_POINT ( 'NONE',  ( -92.69370383062505425, 88.66845928578038638, 78.00114583420049996 ) ) ;
#45305=CARTESIAN_POINT ( 'NONE',  ( 95.00000000000000000, -212.6630814284392557, 79.00656250086713328 ) ) ;
#45307=AXIS2_PLACEMENT_3D ( 'NONE', #56498, #5739, #29378 ) ;
#45316=CARTESIAN_POINT ( 'NONE',  ( 96.15314808468750130, -211.9973110713294489, 75.40822916753381833 ) ) ;
#45319=CARTESIAN_POINT ( 'NONE',  ( -94.95306897617113862, 87.35041560265752025, 75.00000002508417651 ) ) ;
#45320=CARTESIAN_POINT ( 'NONE',  ( 97.30629616937498838, 88.66845928578037217, 84.98614583420047097 ) ) ;
#45321=AXIS2_PLACEMENT_3D ( 'NONE', #71682, #9279, #8916 ) ;
#45323=CARTESIAN_POINT ( 'NONE',  ( 97.64999999999997726, -211.5299782133524502, 77.56458333333333144 ) ) ;
#45328=EDGE_LOOP ( 'NONE', ( #33640, #58598, #9218, #2813 ) ) ;
#45340=CARTESIAN_POINT ( 'NONE',  ( -97.64999999999994884, -211.5299782133524502, 83.78229166840095843 ) ) ;
#45343=VERTEX_POINT ( 'NONE', #63617 ) ;
#45344=CARTESIAN_POINT ( 'NONE',  ( 92.34999999999999432, 91.52997821335252127, 84.31145833506762699 ) ) ;
#45345=CARTESIAN_POINT ( 'NONE',  ( -97.65000000000001990, 90.00000000000004263, 80.55437500173430010 ) ) ;
#45348=CARTESIAN_POINT ( 'NONE',  ( 94.99999999999998579, 87.33691857156068750, 82.97531250086716170 ) ) ;
#45356=CARTESIAN_POINT ( 'NONE',  ( -15.70044424985254850, 0.001194404164626844313, -90.00000000000000000 ) ) ;
#45358=ORIENTED_EDGE ( 'NONE', *, *, #33153, .F. ) ;
#45362=CARTESIAN_POINT ( 'NONE',  ( -94.95306897617061281, -212.6495843973424655, 75.00000002508416230 ) ) ;
#45366=CARTESIAN_POINT ( 'NONE',  ( 92.69370383062498320, 90.00000000000002842, 89.80156250086714920 ) ) ;
#45368=CARTESIAN_POINT ( 'NONE',  ( -96.15314808468745866, -211.9973110713294489, 80.38239583420048007 ) ) ;
#45370=CARTESIAN_POINT ( 'NONE',  ( -92.69370383062502583, 91.33154071421968467, 87.47322916753381605 ) ) ;
#45372=CYLINDRICAL_SURFACE ( 'NONE', #54712, 2.649999999999985700 ) ;
#45375=CARTESIAN_POINT ( 'NONE',  ( -97.44941226939890555, -210.6792855350397815, 74.93153462041274793 ) ) ;
#45380=DIRECTION ( 'NONE',  ( -0.000000000000000000, -0.000000000000000000, 1.000000000000000000 ) ) ;
#45385=CARTESIAN_POINT ( 'NONE',  ( 94.99999999999998579, 87.33691857156068750, 89.32531250086715602 ) ) ;
#45387=CARTESIAN_POINT ( 'NONE',  ( -96.15314808468747287, -208.0026889286704943, 89.06072916753382174 ) ) ;
#45388=LINE ( 'NONE', #29171, #61443 ) ;
#45391=CARTESIAN_POINT ( 'NONE',  ( -92.69370383062505425, 88.66845928578038638, 79.11239583420046984 ) ) ;
#45392=CARTESIAN_POINT ( 'NONE',  ( -92.35000000000306386, -210.0000040461925437, 77.06187486178056645 ) ) ;
#45394=CARTESIAN_POINT ( 'NONE',  ( 92.35000000000000853, -209.9999999999999716, 79.91937500173429498 ) ) ;
#45398=CARTESIAN_POINT ( 'NONE',  ( 97.30629616937498838, -208.6684592857803011, 74.93197916753381094 ) ) ;
#45412=CARTESIAN_POINT ( 'NONE',  ( 97.65000000000000568, -211.5299782133524218, 82.08895833506764461 ) ) ;
#45413=CARTESIAN_POINT ( 'NONE',  ( 96.32499999999998863, -212.2949673200287179, 88.30666666666665776 ) ) ;
#45415=VERTEX_POINT ( 'NONE', #58697 ) ;
#45417=CARTESIAN_POINT ( 'NONE',  ( -97.65000000000000568, 90.00003728274772641, 81.18937371225271704 ) ) ;
#45418=ORIENTED_EDGE ( 'NONE', *, *, #578, .F. ) ;
#45425=CARTESIAN_POINT ( 'NONE',  ( 93.67500000000001137, -212.2949673200287179, 75.58020833506763836 ) ) ;
#45426=CARTESIAN_POINT ( 'NONE',  ( 97.64999999999997726, 88.47002178664753558, 82.00958333333332462 ) ) ;
#45430=LINE ( 'NONE', #62734, #3805 ) ;
#45432=CARTESIAN_POINT ( 'NONE',  ( -93.67500000000003979, 92.29496732002878900, 88.59770833506763665 ) ) ;
#45433=CARTESIAN_POINT ( 'NONE',  ( -95.00000000000002842, 87.33691857156074434, 82.34031250086714238 ) ) ;
#45435=AXIS2_PLACEMENT_3D ( 'NONE', #55854, #38937, #50574 ) ;
#45436=CARTESIAN_POINT ( 'NONE',  ( 97.30629616937498838, 91.33154071421968467, 78.58322916753381548 ) ) ;
#45439=CARTESIAN_POINT ( 'NONE',  ( -97.64999999999997726, -209.9999999999999716, 75.00000000000000000 ) ) ;
#45440=CARTESIAN_POINT ( 'NONE',  ( 92.35003969675449298, 88.46999886771558863, 88.86229325377449584 ) ) ;
#45444=CARTESIAN_POINT ( 'NONE',  ( -93.84685191531248449, -208.0026889286704943, 77.36614583420046642 ) ) ;
#45447=EDGE_LOOP ( 'NONE', ( #42092, #50814, #64453, #40154 ) ) ;
#45456=CARTESIAN_POINT ( 'NONE',  ( -93.84685191531248449, -208.0026889286704943, 89.58989583420049030 ) ) ;
#45457=EDGE_LOOP ( 'NONE', ( #63564, #63477, #60011, #73204 ) ) ;
#45458=CARTESIAN_POINT ( 'NONE',  ( -92.35000000000003695, -208.4700217866474077, 81.48041666666665606 ) ) ;
#45465=CARTESIAN_POINT ( 'NONE',  ( 92.35000000000000853, -209.9999999999999716, 86.26937500173430351 ) ) ;
#45466=CARTESIAN_POINT ( 'NONE',  ( 96.15314808468748708, 91.99731107132950569, 86.25614583420048120 ) ) ;
#45468=DIRECTION ( 'NONE',  ( 1.000000000000000000, 0.000000000000000000, 0.000000000000000000 ) ) ;
#45482=CARTESIAN_POINT ( 'NONE',  ( -93.67499999999998295, -212.2949673200287179, 83.86166666666666458 ) ) ;
#45485=ORIENTED_EDGE ( 'NONE', *, *, #47204, .F. ) ;
#45492=CARTESIAN_POINT ( 'NONE',  ( 97.30629616937498838, -208.6684592857803011, 85.09197916753380753 ) ) ;
#45494=AXIS2_PLACEMENT_3D ( 'NONE', #21041, #71426, #43993 ) ;
#45497=VERTEX_POINT ( 'NONE', #42156 ) ;
#45499=EDGE_LOOP ( 'NONE', ( #50140, #53439, #50759, #23755 ) ) ;
#45501=CARTESIAN_POINT ( 'NONE',  ( 96.15314808468748708, -208.0026889286704943, 79.90614583420047268 ) ) ;
#45503=CARTESIAN_POINT ( 'NONE',  ( 96.15314808468750130, -211.9973110713294489, 83.02822916753380866 ) ) ;
#45510=CARTESIAN_POINT ( 'NONE',  ( -92.69370383062502583, 91.33154071421968467, 74.93197916753381094 ) ) ;
#45511=CIRCLE ( 'NONE', #44317, 15.69999999999999929 ) ;
#45514=ORIENTED_EDGE ( 'NONE', *, *, #69412, .F. ) ;
#45515=CARTESIAN_POINT ( 'NONE',  ( 15.69955575014744831, 0.001194404164628767254, -85.59999999999999432 ) ) ;
#45516=CARTESIAN_POINT ( 'NONE',  ( 96.32499999999998863, -212.2949673200287179, 88.38604166840097776 ) ) ;
#45522=( BOUNDED_CURVE ( )  B_SPLINE_CURVE ( 2, ( #54128, #29687, #30430, #24803, #7882, #47733, #52636 ),
 .UNSPECIFIED., .F., .F. ) 
 B_SPLINE_CURVE_WITH_KNOTS ( ( 3, 2, 2, 3 ),
 ( 0.5208333333333332593, 0.5277777777777776791, 0.5347222222222220989, 0.5416666666666665186 ),
 .UNSPECIFIED. ) 
 CURVE ( )  GEOMETRIC_REPRESENTATION_ITEM ( )  RATIONAL_B_SPLINE_CURVE ( ( 1.000000000000002220, 0.8660254037844365982, 1.000000000000000000, 0.8660254037844387076, 1.000000000000000000, 0.8660254037844408170, 0.9999999999999978906 ) ) 
 REPRESENTATION_ITEM ( '' )  );
#45536=VECTOR ( 'NONE', #1636, 1000.000000000000114 ) ;
#45537=CARTESIAN_POINT ( 'NONE',  ( -96.15314808468752972, 91.99731107132950569, 75.72572916753382799 ) ) ;
#45540=CARTESIAN_POINT ( 'NONE',  ( 92.69370383062498320, 91.33154071421968467, 75.61989583420047722 ) ) ;
#45542=CARTESIAN_POINT ( 'NONE',  ( 97.64999999997404245, -210.0000117261773198, 82.77687459617033028 ) ) ;
#45543=CARTESIAN_POINT ( 'NONE',  ( -92.69370383062498320, -211.3315407142195852, 86.73239583420047438 ) ) ;
#45544=ORIENTED_EDGE ( 'NONE', *, *, #56807, .F. ) ;
#45548=CARTESIAN_POINT ( 'NONE',  ( 94.20702885560676521, -212.5043059284880087, 74.98272308147871001 ) ) ;
#45554=LINE ( 'NONE', #40635, #48228 ) ;
#45559=CARTESIAN_POINT ( 'NONE',  ( 94.56602944578247616, -207.6412937382897894, 74.84690984288795335 ) ) ;
#45560=CARTESIAN_POINT ( 'NONE',  ( -95.00000000000002842, 87.33691857156074434, 83.45156250086714067 ) ) ;
#45561=CARTESIAN_POINT ( 'NONE',  ( 2.499999999999984457, -73.00000000000001421, -255.0000000000000000 ) ) ;
#45564=CARTESIAN_POINT ( 'NONE',  ( 97.64999999999999147, 90.00000015433757028, 79.60187500750917877 ) ) ;
#45566=VECTOR ( 'NONE', #56012, 1000.000000000000000 ) ;
#45570=LINE ( 'NONE', #52667, #50950 ) ;
#45571=CARTESIAN_POINT ( 'NONE',  ( -97.30629616937497417, -211.3315407142195852, 80.96447916753382401 ) ) ;
#45574=DIRECTION ( 'NONE',  ( 1.000000000000000000, 0.000000000000000000, 0.000000000000000000 ) ) ;
#45577=EDGE_LOOP ( 'NONE', ( #8875, #33459 ) ) ;
#45579=CARTESIAN_POINT ( 'NONE',  ( -92.35000000000005116, 88.47002178664754979, 80.81895833506763438 ) ) ;
#45590=CARTESIAN_POINT ( 'NONE',  ( 95.00000000000000000, -207.3369185715606307, 89.48406250086713953 ) ) ;
#45595=EDGE_CURVE ( 'NONE', #4573, #67765, #30111, .T. ) ;
#45597=CARTESIAN_POINT ( 'NONE',  ( -97.64998927049083477, -208.4700155919624933, 84.94645790656207396 ) ) ;
#45609=CARTESIAN_POINT ( 'NONE',  ( 92.34999999999999432, 91.52997821335252127, 89.94708333333333883 ) ) ;
#45613=ORIENTED_EDGE ( 'NONE', *, *, #46962, .T. ) ;
#45616=EDGE_LOOP ( 'NONE', ( #3643, #12328, #8310, #57165 ) ) ;
#45617=CARTESIAN_POINT ( 'NONE',  ( 97.30629616937498838, 91.33154071421968467, 83.66322916753379957 ) ) ;
#45620=CARTESIAN_POINT ( 'NONE',  ( 96.15314808468748708, -208.0026889286704943, 86.89114583420047211 ) ) ;
#45623=PRODUCT_CONTEXT ( 'NONE', #33461, 'mechanical' ) ;
#45624=CARTESIAN_POINT ( 'NONE',  ( -97.64999999999996305, -209.9999627172523446, 81.18937371225273125 ) ) ;
#45632=CARTESIAN_POINT ( 'NONE',  ( -92.69370383062498320, -211.3315407142195852, 86.09739583420048348 ) ) ;
#45633=CARTESIAN_POINT ( 'NONE',  ( -92.69370383062502583, 91.33154071421968467, 85.09197916753380753 ) ) ;
#45636=CARTESIAN_POINT ( 'NONE',  ( 93.84685191531248449, 91.99731107132950569, 83.82197916753381151 ) ) ;
#45637=CARTESIAN_POINT ( 'NONE',  ( -96.15314808468752972, 91.99731107132950569, 84.45697916753380241 ) ) ;
#45642=CARTESIAN_POINT ( 'NONE',  ( 92.34999999999999432, 90.00000000000002842, 87.45999999999999375 ) ) ;
#45643=CARTESIAN_POINT ( 'NONE',  ( -94.99999999999997158, -212.6630814284392557, 86.62656250086713783 ) ) ;
#45644=CARTESIAN_POINT ( 'NONE',  ( -93.67499999999998295, -212.2949673200287179, 81.95666666666666345 ) ) ;
#45645=CARTESIAN_POINT ( 'NONE',  ( -93.67500000000003979, 87.70503267997129626, 89.02104166840096866 ) ) ;
#45650=CARTESIAN_POINT ( 'NONE',  ( -97.65000000000001990, 90.00000000000004263, 77.93499999999998806 ) ) ;
#45654=CARTESIAN_POINT ( 'NONE',  ( -96.32499999999996021, -207.7050326799711968, 89.89416666666666345 ) ) ;
#45658=CARTESIAN_POINT ( 'NONE',  ( -92.69370383062504004, 90.00000000000004263, 79.16531250086714522 ) ) ;
#45668=CARTESIAN_POINT ( 'NONE',  ( 93.84685191531248449, 88.00268892867053694, 76.57239583420049200 ) ) ;
#45670=CARTESIAN_POINT ( 'NONE',  ( -93.84685191531248449, -208.0026889286704943, 80.69989583420047552 ) ) ;
#45683=CARTESIAN_POINT ( 'NONE',  ( 92.69370383062501162, -209.9999999999999716, 79.48281250086714067 ) ) ;
#45684=ORIENTED_EDGE ( 'NONE', *, *, #58545, .F. ) ;
#45690=LINE ( 'NONE', #49809, #28581 ) ;
#45691=VERTEX_POINT ( 'NONE', #54531 ) ;
#45694=CARTESIAN_POINT ( 'NONE',  ( 95.00000000000000000, -207.3369185715606307, 76.30781250086715772 ) ) ;
#45698=CARTESIAN_POINT ( 'NONE',  ( 97.30629616937498838, 88.66845928578037217, 81.81114583420048803 ) ) ;
#45700=CARTESIAN_POINT ( 'NONE',  ( 96.32499999999998863, -212.2949673200287179, 77.51166666666665606 ) ) ;
#45703=AXIS2_PLACEMENT_3D ( 'NONE', #45844, #69136, #45093 ) ;
#45718=ORIENTED_EDGE ( 'NONE', *, *, #8212, .T. ) ;
#45719=CARTESIAN_POINT ( 'NONE',  ( -93.67499999999998295, -212.2949673200287179, 83.94104166840097037 ) ) ;
#45722=EDGE_CURVE ( 'NONE', #53141, #45993, #64708, .T. ) ;
#45724=CARTESIAN_POINT ( 'NONE',  ( 93.67499999999999716, 87.70503267997126784, 80.66020833506763665 ) ) ;
#45725=CARTESIAN_POINT ( 'NONE',  ( -97.65000000000001990, 91.52997821335253548, 78.59645833506763779 ) ) ;
#45727=CARTESIAN_POINT ( 'NONE',  ( 92.69370383062498320, 88.66845928578037217, 81.59947916753381492 ) ) ;
#45732=CARTESIAN_POINT ( 'NONE',  ( 94.99999999999998579, 93.05995642670504253, 87.93624999999998693 ) ) ;
#45735=CARTESIAN_POINT ( 'NONE',  ( -92.35000677010287973, 88.47001787792684979, 82.72395806468928470 ) ) ;
#45737=CARTESIAN_POINT ( 'NONE',  ( 92.34999999999999432, 90.00000000000002842, 90.00000000000000000 ) ) ;
#45745=( BOUNDED_CURVE ( )  B_SPLINE_CURVE ( 2, ( #47192, #999, #35167, #17506, #23519, #11491, #40820 ),
 .UNSPECIFIED., .F., .F. ) 
 B_SPLINE_CURVE_WITH_KNOTS ( ( 3, 2, 2, 3 ),
 ( 0.8333333333333334814, 0.8402777777777779011, 0.8472222222222222099, 0.8541666666666666297 ),
 .UNSPECIFIED. ) 
 CURVE ( )  GEOMETRIC_REPRESENTATION_ITEM ( )  RATIONAL_B_SPLINE_CURVE ( ( 0.9999999999999978906, 0.8660254037844408170, 1.000000000000000000, 0.8660254037844387076, 1.000000000000000000, 0.8660254037844387076, 1.000000000000000000 ) ) 
 REPRESENTATION_ITEM ( '' )  );
#45746=CARTESIAN_POINT ( 'NONE',  ( -92.69370383062498320, -209.9999999999999716, 80.59406250086715318 ) ) ;
#45755=CARTESIAN_POINT ( 'NONE',  ( -96.32499999999996021, -207.7050326799711968, 79.09916666666666174 ) ) ;
#45759=CARTESIAN_POINT ( 'NONE',  ( 94.99999999999998579, 87.33691857156068750, 87.42031250086715488 ) ) ;
#45760=CARTESIAN_POINT ( 'NONE',  ( -96.15314808468745866, -211.9973110713294489, 88.63739583420048973 ) ) ;
#45765=CIRCLE ( 'NONE', #52977, 26.50000000000000355 ) ;
#45766=CARTESIAN_POINT ( 'NONE',  ( -97.30629616937501680, 90.00000000000004263, 78.21281250086714465 ) ) ;
#45770=CARTESIAN_POINT ( 'NONE',  ( 93.84685191531251292, -211.9973110713294489, 89.11364583420048291 ) ) ;
#45772=EDGE_CURVE ( 'NONE', #29385, #54357, #10145, .T. ) ;
#45774=CARTESIAN_POINT ( 'NONE',  ( 94.99999999999998579, 86.94004357329502852, 83.17374999999999829 ) ) ;
#45784=CARTESIAN_POINT ( 'NONE',  ( 93.84685191531251292, -211.9973110713294489, 86.09739583420049769 ) ) ;
#45788=CARTESIAN_POINT ( 'NONE',  ( -96.32499999999996021, -207.7050326799711968, 77.27354166840096639 ) ) ;
#45791=CARTESIAN_POINT ( 'NONE',  ( 96.32499999999998863, -207.7050326799711968, 89.15333333333333599 ) ) ;
#45794=VERTEX_POINT ( 'NONE', #24729 ) ;
#45801=CARTESIAN_POINT ( 'NONE',  ( 96.32499999999998863, -207.7050326799711968, 76.53270833506762472 ) ) ;
#45802=CARTESIAN_POINT ( 'NONE',  ( 96.32499999999998863, 87.70503267997126784, 83.22666666666665947 ) ) ;
#45808=CARTESIAN_POINT ( 'NONE',  ( 97.64999999999999147, 89.99999988321010846, 84.68187499741277691 ) ) ;
#45809=CARTESIAN_POINT ( 'NONE',  ( -97.30629616937501680, 90.00000000000004263, 80.27656250086714351 ) ) ;
#45810=CARTESIAN_POINT ( 'NONE',  ( 94.99999999999998579, 87.33691857156068750, 79.64156250086713840 ) ) ;
#45814=CARTESIAN_POINT ( 'NONE',  ( 94.99999999999998579, 86.94004357329502852, 88.96812500173430749 ) ) ;
#45821=CARTESIAN_POINT ( 'NONE',  ( -92.69370383062498320, -211.3315407142195852, 79.11239583420046984 ) ) ;
#45830=CARTESIAN_POINT ( 'NONE',  ( -94.99999999999997158, -212.6630814284392557, 75.19656250086714522 ) ) ;
#45832=CARTESIAN_POINT ( 'NONE',  ( 97.64999999999999147, 90.00000000000002842, 88.49187500173430010 ) ) ;
#45835=CARTESIAN_POINT ( 'NONE',  ( 93.67500000000001137, -207.7050326799711968, 81.63916666666666799 ) ) ;
#45840=CARTESIAN_POINT ( 'NONE',  ( 93.84685191531248449, 88.00268892867053694, 83.39864583420047950 ) ) ;
#45843=CARTESIAN_POINT ( 'NONE',  ( -97.65000000000009095, 88.47002178664760663, 75.44791666666667140 ) ) ;
#45844=CARTESIAN_POINT ( 'NONE',  ( 2.500000000000029754, 73.00000000000001421, -204.9999999999999716 ) ) ;
#45847=CARTESIAN_POINT ( 'NONE',  ( 92.35000000000000853, -209.9999999999999716, 87.53937500173429953 ) ) ;
#45853=CARTESIAN_POINT ( 'NONE',  ( -93.84685191531254134, 91.99731107132950569, 89.43114583420047836 ) ) ;
#45856=EDGE_CURVE ( 'NONE', #69332, #51295, #48134, .T. ) ;
#45857=CARTESIAN_POINT ( 'NONE',  ( -92.35000000000003695, 90.00000000000004263, 75.07749999999998636 ) ) ;
#45868=CARTESIAN_POINT ( 'NONE',  ( 93.84685191531249870, -208.0026889286704943, 84.61572916753381435 ) ) ;
#45874=ADVANCED_FACE ( 'NONE', ( #71686 ), #68333, .F. ) ;
#45879=CARTESIAN_POINT ( 'NONE',  ( 93.84685191531249870, -208.0026889286704943, 77.47197916753380298 ) ) ;
#45881=CARTESIAN_POINT ( 'NONE',  ( 92.69370383062501162, -208.6684592857803011, 84.03364583420049883 ) ) ;
#45889=CARTESIAN_POINT ( 'NONE',  ( 97.64999999989935020, -209.9999769027737671, 83.41187580057901130 ) ) ;
#45890=CARTESIAN_POINT ( 'NONE',  ( 95.00000000000000000, -213.0599564267049857, 87.06312500173430635 ) ) ;
#45904=CARTESIAN_POINT ( 'NONE',  ( 96.32499999999997442, 92.29496732002878900, 81.53333333333333144 ) ) ;
#45905=CARTESIAN_POINT ( 'NONE',  ( -92.35000000000003695, 90.00000000000004263, 89.04749999999999943 ) ) ;
#45910=CARTESIAN_POINT ( 'NONE',  ( -93.84685191531248449, -208.0026889286704943, 87.52614583420047722 ) ) ;
#45913=CARTESIAN_POINT ( 'NONE',  ( 94.87443773336561037, -212.6467947905572089, 74.99648857272262603 ) ) ;
#45914=CARTESIAN_POINT ( 'NONE',  ( 92.35000000000007958, 88.47002178664749295, 81.16291666666667481 ) ) ;
#45915=CARTESIAN_POINT ( 'NONE',  ( -97.30629616937497417, -211.3315407142195852, 77.63072916753380071 ) ) ;
#45916=ADVANCED_FACE ( 'NONE', ( #47625 ), #48730, .F. ) ;
#45926=CARTESIAN_POINT ( 'NONE',  ( -97.30629616937501680, 91.33154071421968467, 79.42989583420046529 ) ) ;
#45931=CYLINDRICAL_SURFACE ( 'NONE', #46200, 23.50000000000000355 ) ;
#45938=CARTESIAN_POINT ( 'NONE',  ( -97.65000000000001990, 91.52997821335253548, 89.94708333333332462 ) ) ;
#45940=CARTESIAN_POINT ( 'NONE',  ( -93.84685191531247028, -211.9973110713294489, 81.12322916753382174 ) ) ;
#45944=CARTESIAN_POINT ( 'NONE',  ( -95.00000000000002842, 90.00000000000004263, 90.00000000000000000 ) ) ;
#45952=ADVANCED_FACE ( 'NONE', ( #19416 ), #44593, .F. ) ;
#45955=( BOUNDED_CURVE ( )  B_SPLINE_CURVE ( 2, ( #269, #23161, #62272, #69021, #57739, #6245, #628 ),
 .UNSPECIFIED., .F., .F. ) 
 B_SPLINE_CURVE_WITH_KNOTS ( ( 3, 2, 2, 3 ),
 ( 0.6250000000000003331, 0.6319444444444446418, 0.6388888888888890616, 0.6458333333333334814 ),
 .UNSPECIFIED. ) 
 CURVE ( )  GEOMETRIC_REPRESENTATION_ITEM ( )  RATIONAL_B_SPLINE_CURVE ( ( 0.9999999999999935607, 0.8660254037844451469, 1.000000000000000000, 0.8660254037844387076, 1.000000000000000000, 0.8660254037844365982, 1.000000000000002220 ) ) 
 REPRESENTATION_ITEM ( '' )  );
#45956=CARTESIAN_POINT ( 'NONE',  ( 97.30629616937498838, -208.6684592857803295, 87.47322916753380184 ) ) ;
#45969=CYLINDRICAL_SURFACE ( 'NONE', #42852, 12.75000000000000000 ) ;
#45971=VECTOR ( 'NONE', #5875, 1000.000000000000000 ) ;
#45976=CARTESIAN_POINT ( 'NONE',  ( 96.15314808468748708, 88.00268892867053694, 86.04447916753380809 ) ) ;
#45979=CARTESIAN_POINT ( 'NONE',  ( 92.69370383062501162, -209.9999999999999716, 80.75281250086715090 ) ) ;
#45982=CARTESIAN_POINT ( 'NONE',  ( 7.103376864691351012E-17, -120.0000000000000000, -64.00000000000000000 ) ) ;
#45984=DIRECTION ( 'NONE',  ( 0.000000000000000000, 0.000000000000000000, 1.000000000000000000 ) ) ;
#45987=CARTESIAN_POINT ( 'NONE',  ( 92.35000000003287823, 90.00000839536618003, 84.99910573348789455 ) ) ;
#45988=CARTESIAN_POINT ( 'NONE',  ( -94.99999999999997158, -212.6630814284392557, 85.99156250086714692 ) ) ;
#45989=CARTESIAN_POINT ( 'NONE',  ( -93.84685191531254134, 91.99731107132950569, 83.87489583420048689 ) ) ;
#45991=CARTESIAN_POINT ( 'NONE',  ( 94.99999999999998579, 92.66308142843935514, 85.03906250086714635 ) ) ;
#45992=CARTESIAN_POINT ( 'NONE',  ( -97.30629616937501680, 91.33154071421968467, 84.50989583420046358 ) ) ;
#45993=VERTEX_POINT ( 'NONE', #9987 ) ;
#45994=CARTESIAN_POINT ( 'NONE',  ( -97.64999999999997726, 91.52997821335256390, 88.04208333333330927 ) ) ;
#45995=CARTESIAN_POINT ( 'NONE',  ( -99.99999999999998579, -124.0000000000000142, 39.99999999999996447 ) ) ;
#45997=LINE ( 'NONE', #29784, #52449 ) ;
#45998=CARTESIAN_POINT ( 'NONE',  ( -93.84685191531248449, -208.0026889286704943, 86.89114583420047211 ) ) ;
#46007=CARTESIAN_POINT ( 'NONE',  ( -97.65000000000001990, 91.52997821335253548, 76.61208333333333087 ) ) ;
#46011=CARTESIAN_POINT ( 'NONE',  ( 96.32499999999997442, 92.29496732002878900, 76.45333333333333314 ) ) ;
#46013=CARTESIAN_POINT ( 'NONE',  ( 97.64999999999996305, -209.9999996502043018, 77.69687501385438111 ) ) ;
#46016=CARTESIAN_POINT ( 'NONE',  ( -95.00000000000002842, 87.33691857156074434, 77.10156250086711793 ) ) ;
#46021=AXIS2_PLACEMENT_3D ( 'NONE', #37168, #2245, #14965 ) ;
#46027=AXIS2_PLACEMENT_3D ( 'NONE', #32768, #61737, #10971 ) ;
#46028=EDGE_CURVE ( 'NONE', #50672, #67440, #62634, .T. ) ;
#46029=CARTESIAN_POINT ( 'NONE',  ( 93.84685191531248449, 91.99731107132950569, 76.99572916753382401 ) ) ;
#46030=CARTESIAN_POINT ( 'NONE',  ( -96.15314808468747287, -208.0026889286704943, 78.26572916753382003 ) ) ;
#46032=ORIENTED_EDGE ( 'NONE', *, *, #28240, .F. ) ;
#46038=CARTESIAN_POINT ( 'NONE',  ( -97.30629616937501680, 90.00000000000004263, 76.46656250086715545 ) ) ;
#46039=CARTESIAN_POINT ( 'NONE',  ( 96.15314808468748708, -208.0026889286704943, 80.54114583420046358 ) ) ;
#46040=ORIENTED_EDGE ( 'NONE', *, *, #58765, .F. ) ;
#46041=ADVANCED_FACE ( 'NONE', ( #21640 ), #33280, .F. ) ;
#46045=CYLINDRICAL_SURFACE ( 'NONE', #21962, 2.649999999999985700 ) ;
#46051=ORIENTED_EDGE ( 'NONE', *, *, #72209, .T. ) ;
#46054=CARTESIAN_POINT ( 'NONE',  ( 93.84685191531248449, 88.00268892867053694, 83.55739583420049144 ) ) ;
#46057=LINE ( 'NONE', #12672, #38052 ) ;
#46059=ORIENTED_EDGE ( 'NONE', *, *, #35051, .T. ) ;
#46063=CARTESIAN_POINT ( 'NONE',  ( -96.32499999999996021, -207.7050326799711968, 85.44916666666665606 ) ) ;
#46066=FACE_BOUND ( 'NONE', #2450, .T. ) ;
#46070=CARTESIAN_POINT ( 'NONE',  ( -92.34999999999999432, -209.9999999999999716, 84.04687500173430692 ) ) ;
#46072=DIRECTION ( 'NONE',  ( -0.000000000000000000, -0.000000000000000000, 1.000000000000000000 ) ) ;
#46074=CARTESIAN_POINT ( 'NONE',  ( 97.64999999999997726, 91.52997821335252127, 80.92479166840098515 ) ) ;
#46075=CARTESIAN_POINT ( 'NONE',  ( -97.65000000000001990, 91.52997821335253548, 80.50145833506765314 ) ) ;
#46078=CARTESIAN_POINT ( 'NONE',  ( 97.30629616937498838, 90.00000000000002842, 79.32406250086715715 ) ) ;
#46082=EDGE_CURVE ( 'NONE', #49121, #29989, #1621, .T. ) ;
#46086=LINE ( 'NONE', #57362, #45971 ) ;
#46098=CARTESIAN_POINT ( 'NONE',  ( -92.69370383062498320, -211.3315407142195852, 76.73114583420048973 ) ) ;
#46103=CARTESIAN_POINT ( 'NONE',  ( -96.67299840329707195, -211.9834083483352174, 74.96344747200149072 ) ) ;
#46104=CARTESIAN_POINT ( 'NONE',  ( 92.34999999999999432, 90.00000000000002842, 75.00000000000000000 ) ) ;
#46105=CARTESIAN_POINT ( 'NONE',  ( 96.48680242707320076, 91.80467564693685745, 74.81083481226639265 ) ) ;
#46107=CARTESIAN_POINT ( 'NONE',  ( 97.64999999981932888, 89.99996905681224746, 78.33187387208513996 ) ) ;
#46114=CARTESIAN_POINT ( 'NONE',  ( 94.99999999999998579, 87.33691857156068750, 86.78531250086713555 ) ) ;
#46119=CARTESIAN_POINT ( 'NONE',  ( -97.30629616937501680, 91.33154071421968467, 79.42989583420047950 ) ) ;
#46120=EDGE_CURVE ( 'NONE', #9070, #50612, #18228, .T. ) ;
#46122=AXIS2_PLACEMENT_3D ( 'NONE', #51878, #44766, #418 ) ;
#46123=CARTESIAN_POINT ( 'NONE',  ( 97.30629616937498838, -208.6684592857803011, 89.37822916753381719 ) ) ;
#46124=EDGE_CURVE ( 'NONE', #57825, #11290, #40777, .T. ) ;
#46127=DIRECTION ( 'NONE',  ( 1.000000000000000000, 0.000000000000000000, 0.000000000000000000 ) ) ;
#46133=VECTOR ( 'NONE', #9762, 1000.000000000000000 ) ;
#46134=CARTESIAN_POINT ( 'NONE',  ( 92.69370383062501162, -211.3315407142195852, 76.51947916753381662 ) ) ;
#46138=CARTESIAN_POINT ( 'NONE',  ( 97.30629616937498838, -209.9999999999999716, 80.59406250086715318 ) ) ;
#46139=CARTESIAN_POINT ( 'NONE',  ( 97.64999999999999147, 90.00000000000002842, 89.68250000000000455 ) ) ;
#46143=CARTESIAN_POINT ( 'NONE',  ( 95.00000000000000000, -213.0599564267049857, 76.82374999999998977 ) ) ;
#46144=DIRECTION ( 'NONE',  ( 0.000000000000000000, 0.000000000000000000, -1.000000000000000000 ) ) ;
#46145=CARTESIAN_POINT ( 'NONE',  ( 97.64999999999997726, -211.5299782133524502, 87.08958333333333712 ) ) ;
#46147=ORIENTED_EDGE ( 'NONE', *, *, #1490, .T. ) ;
#46152=CARTESIAN_POINT ( 'NONE',  ( -92.69370383062502583, 88.66845928578038638, 86.25614583420048120 ) ) ;
#46153=CYLINDRICAL_SURFACE ( 'NONE', #65344, 2.649999999999985700 ) ;
#46155=CARTESIAN_POINT ( 'NONE',  ( 97.64999999999999147, -209.9999999999999716, 77.69687500173431260 ) ) ;
#46156=CARTESIAN_POINT ( 'NONE',  ( 97.64999999999997726, 88.47002178664753558, 77.56458333333333144 ) ) ;
#46159=ORIENTED_EDGE ( 'NONE', *, *, #2678, .T. ) ;
#46161=VECTOR ( 'NONE', #17150, 1000.000000000000000 ) ;
#46163=CARTESIAN_POINT ( 'NONE',  ( 95.00000000000000000, -213.0599564267049857, 88.33312500173431658 ) ) ;
#46164=( BOUNDED_CURVE ( )  B_SPLINE_CURVE ( 2, ( #50248, #37512, #38619, #61554, #4417, #60447, #43537 ),
 .UNSPECIFIED., .F., .F. ) 
 B_SPLINE_CURVE_WITH_KNOTS ( ( 3, 2, 2, 3 ),
 ( 0.3541666666666665741, 0.3611111111111109939, 0.3680555555555554137, 0.3749999999999998335 ),
 .UNSPECIFIED. ) 
 CURVE ( )  GEOMETRIC_REPRESENTATION_ITEM ( )  RATIONAL_B_SPLINE_CURVE ( ( 1.000000000000002220, 0.8660254037844365982, 1.000000000000000000, 0.8660254037844387076, 1.000000000000000000, 0.8660254037844419273, 0.9999999999999967804 ) ) 
 REPRESENTATION_ITEM ( '' )  );
#46165=CARTESIAN_POINT ( 'NONE',  ( -95.00000000000002842, 87.33691857156074434, 81.07031250086716057 ) ) ;
#46166=CARTESIAN_POINT ( 'NONE',  ( 93.84685191531248449, 88.00268892867053694, 89.27239583420049485 ) ) ;
#46170=ADVANCED_FACE ( 'NONE', ( #63365 ), #1360, .F. ) ;
#46174=CARTESIAN_POINT ( 'NONE',  ( -92.69370383062498320, -208.6684592857803011, 78.58322916753381548 ) ) ;
#46186=CARTESIAN_POINT ( 'NONE',  ( -94.99999999999997158, -207.3369185715606307, 76.78406250086712248 ) ) ;
#46192=DIRECTION ( 'NONE',  ( -1.343011723336883198E-16, 1.000000000000000000, 0.000000000000000000 ) ) ;
#46193=ORIENTED_EDGE ( 'NONE', *, *, #48658, .F. ) ;
#46195=VECTOR ( 'NONE', #66377, 1000.000000000000000 ) ;
#46197=CARTESIAN_POINT ( 'NONE',  ( 97.30629616937498838, 90.00000000000002842, 83.61031250086713840 ) ) ;
#46200=AXIS2_PLACEMENT_3D ( 'NONE', #56469, #51920, #73726 ) ;
#46201=CYLINDRICAL_SURFACE ( 'NONE', #61301, 2.649999999999985700 ) ;
#46210=CARTESIAN_POINT ( 'NONE',  ( -97.30629616937501680, 91.33154071421968467, 88.95489583420048518 ) ) ;
#46221=CARTESIAN_POINT ( 'NONE',  ( 97.30629616937498838, -211.3315407142195852, 84.98614583420047097 ) ) ;
#46226=CARTESIAN_POINT ( 'NONE',  ( -94.99999999999997158, -206.9400435732949575, 79.76062500173429726 ) ) ;
#46231=CARTESIAN_POINT ( 'NONE',  ( 92.69370383062501162, -211.3315407142195852, 83.50447916753383026 ) ) ;
#46233=CARTESIAN_POINT ( 'NONE',  ( -97.64999999999996305, -209.9999999999999716, 88.09499999999999886 ) ) ;
#46241=CARTESIAN_POINT ( 'NONE',  ( 92.34999999999999432, 90.00000000000002842, 86.18999999999999773 ) ) ;
#46242=CARTESIAN_POINT ( 'NONE',  ( 97.64999999999999147, -209.9999999999999716, 88.49187500173430010 ) ) ;
#46253=CARTESIAN_POINT ( 'NONE',  ( -97.65000000000001990, 90.00000000000004263, 90.00000000000000000 ) ) ;
#46255=EDGE_LOOP ( 'NONE', ( #228, #57744 ) ) ;
#46260=CARTESIAN_POINT ( 'NONE',  ( -97.65000000000001990, 90.00000000000004263, 86.18999999999999773 ) ) ;
#46263=CARTESIAN_POINT ( 'NONE',  ( -93.67500000000003979, 92.29496732002878900, 86.61333333333332973 ) ) ;
#46266=ORIENTED_EDGE ( 'NONE', *, *, #2890, .T. ) ;
#46267=CARTESIAN_POINT ( 'NONE',  ( -94.99999999999997158, -209.9999999999999716, 75.00000000000000000 ) ) ;
#46268=CARTESIAN_POINT ( 'NONE',  ( -94.99999999999997158, -207.3369185715606307, 86.94406250086714749 ) ) ;
#46271=CARTESIAN_POINT ( 'NONE',  ( -94.99999999999997158, -213.0599564267049857, 79.44312500173430180 ) ) ;
#46274=CARTESIAN_POINT ( 'NONE',  ( -94.99999999999997158, -207.3369185715606307, 74.87906250086713555 ) ) ;
#46283=CARTESIAN_POINT ( 'NONE',  ( -92.69370383062502583, 88.66845928578038638, 79.11239583420046984 ) ) ;
#46287=EDGE_LOOP ( 'NONE', ( #7665, #8624, #66759, #15993 ) ) ;
#46292=DIRECTION ( 'NONE',  ( -0.000000000000000000, -0.000000000000000000, 1.000000000000000000 ) ) ;
#46298=CARTESIAN_POINT ( 'NONE',  ( -97.30629616937495996, -209.9999999999999716, 76.46656250086715545 ) ) ;
#46304=CARTESIAN_POINT ( 'NONE',  ( 92.34999999999998010, -211.5299782133523934, 88.14791666666667425 ) ) ;
#46307=VECTOR ( 'NONE', #39562, 1000.000000000000000 ) ;
#46308=FACE_OUTER_BOUND ( 'NONE', #51756, .T. ) ;
#46313=CARTESIAN_POINT ( 'NONE',  ( 92.69370383062501162, -211.3315407142195852, 85.25072916753379104 ) ) ;
#46319=CARTESIAN_POINT ( 'NONE',  ( 96.32499999999998863, -212.2949673200287179, 85.21104166840096639 ) ) ;
#46321=CARTESIAN_POINT ( 'NONE',  ( -92.69370383062502583, 88.66845928578038638, 79.90614583420048689 ) ) ;
#46328=EDGE_CURVE ( 'NONE', #51512, #5579, #4014, .T. ) ;
#46329=ORIENTED_EDGE ( 'NONE', *, *, #42102, .F. ) ;
#46331=EDGE_LOOP ( 'NONE', ( #12374, #18740, #65450, #63299 ) ) ;
#46337=CARTESIAN_POINT ( 'NONE',  ( 97.30629616937498838, 90.00000000000002842, 84.24531250086714351 ) ) ;
#46340=CARTESIAN_POINT ( 'NONE',  ( 96.15314808468748708, -208.0026889286704943, 83.08114583420048405 ) ) ;
#46349=LINE ( 'NONE', #23056, #60060 ) ;
#46350=CARTESIAN_POINT ( 'NONE',  ( -92.35000000000003695, 90.00000000000004263, 82.69749999999999091 ) ) ;
#46351=CARTESIAN_POINT ( 'NONE',  ( -97.30629616937497417, -208.6684592857803011, 83.23989583420046756 ) ) ;
#46352=CARTESIAN_POINT ( 'NONE',  ( -97.30629616937501680, 90.00000000000004263, 83.45156250086715488 ) ) ;
#46353=ORIENTED_EDGE ( 'NONE', *, *, #43635, .T. ) ;
#46354=CARTESIAN_POINT ( 'NONE',  ( 97.30629616937498838, 90.00000000000002842, 84.24531250086714351 ) ) ;
#46358=ADVANCED_FACE ( 'NONE', ( #47544 ), #53551, .F. ) ;
#46359=CARTESIAN_POINT ( 'NONE',  ( 97.65000000000000568, -211.5299782133524218, 76.37395833506761278 ) ) ;
#46360=CARTESIAN_POINT ( 'NONE',  ( 95.00000000000000000, -209.9999999999999716, 90.00000000000000000 ) ) ;
#46361=CARTESIAN_POINT ( 'NONE',  ( 92.35000000000006537, -208.4700217866474077, 85.50208333333331723 ) ) ;
#46362=CARTESIAN_POINT ( 'NONE',  ( -92.69370383062498320, -211.3315407142195852, 86.09739583420048348 ) ) ;
#46364=CARTESIAN_POINT ( 'NONE',  ( 97.64999999999999147, 90.00000000000002842, 80.15749999999999886 ) ) ;
#46370=CARTESIAN_POINT ( 'NONE',  ( -95.00000000000002842, 93.05995642670501411, 77.14124999999999943 ) ) ;
#46376=( BOUNDED_CURVE ( )  B_SPLINE_CURVE ( 2, ( #22527, #50712, #22153, #52194, #5992, #39074, #68013 ),
 .UNSPECIFIED., .F., .F. ) 
 B_SPLINE_CURVE_WITH_KNOTS ( ( 3, 2, 2, 3 ),
 ( 0.2083333333333331483, 0.2152777777777775681, 0.2222222222222219323, 0.2291666666666663521 ),
 .UNSPECIFIED. ) 
 CURVE ( )  GEOMETRIC_REPRESENTATION_ITEM ( )  RATIONAL_B_SPLINE_CURVE ( ( 1.000000000000003775, 0.8660254037844349329, 1.000000000000000000, 0.8660254037844387076, 1.000000000000000000, 0.8660254037844445918, 0.9999999999999941158 ) ) 
 REPRESENTATION_ITEM ( '' )  );
#46377=CARTESIAN_POINT ( 'NONE',  ( 92.35000000007822507, -209.9999869687480611, 79.28395951162927702 ) ) ;
#46379=CARTESIAN_POINT ( 'NONE',  ( -93.84685191531252713, 88.00268892867056536, 78.42447916753381776 ) ) ;
#46386=CARTESIAN_POINT ( 'NONE',  ( -97.30629616937497417, -211.3315407142195852, 85.40947916753380298 ) ) ;
#46389=CARTESIAN_POINT ( 'NONE',  ( 92.69370383062498320, 88.66845928578035796, 76.51947916753381662 ) ) ;
#46390=CARTESIAN_POINT ( 'NONE',  ( -97.30629616937497417, -208.6684592857803295, 80.85864583420048746 ) ) ;
#46393=DIRECTION ( 'NONE',  ( -3.061616997868382648E-16, -1.000000000000000000, 0.000000000000000000 ) ) ;
#46394=CARTESIAN_POINT ( 'NONE',  ( -93.67499999999998295, -207.7050326799711968, 75.18333333333332291 ) ) ;
#46395=CARTESIAN_POINT ( 'NONE',  ( -97.64999999998390479, 89.99999393654049129, 88.17456390440148084 ) ) ;
#46399=CARTESIAN_POINT ( 'NONE',  ( 97.30629616937498838, -208.6684592857803011, 75.40822916753381833 ) ) ;
#46406=CARTESIAN_POINT ( 'NONE',  ( -92.35000000000003695, 90.00000000000004263, 85.23749999999999716 ) ) ;
#46408=CARTESIAN_POINT ( 'NONE',  ( -96.32500000000001705, 92.29496732002878900, 79.17854166840096752 ) ) ;
#46414=CARTESIAN_POINT ( 'NONE',  ( -92.35000000000003695, -211.5299782133524786, 77.56458333333333144 ) ) ;
#46418=CARTESIAN_POINT ( 'NONE',  ( 97.30629616937498838, 91.33154071421968467, 82.55197916753382970 ) ) ;
#46419=CARTESIAN_POINT ( 'NONE',  ( 95.53230763903961531, -213.2667778271277541, 74.92222617501690252 ) ) ;
#46422=ORIENTED_EDGE ( 'NONE', *, *, #50910, .F. ) ;
#46430=CARTESIAN_POINT ( 'NONE',  ( -93.33864827737279768, 88.39919842643631398, 74.79754476654878204 ) ) ;
#46435=CARTESIAN_POINT ( 'NONE',  ( -92.34999999999999432, -211.5299782133524502, 78.27895833506762813 ) ) ;
#46439=CARTESIAN_POINT ( 'NONE',  ( 97.64999999999997726, 91.52997821335252127, 80.28979166840098003 ) ) ;
#46440=CARTESIAN_POINT ( 'NONE',  ( -97.65000000000001990, 91.52997821335253548, 79.86645833506761960 ) ) ;
#46442=CARTESIAN_POINT ( 'NONE',  ( 92.69370383062498320, 90.00000000000002842, 80.91156250086716284 ) ) ;
#46444=AXIS2_PLACEMENT_3D ( 'NONE', #61257, #32661, #55606 ) ;
#46445=CARTESIAN_POINT ( 'NONE',  ( -92.35000000000000853, -208.4700217866474929, 82.11541666666664696 ) ) ;
#46447=CARTESIAN_POINT ( 'NONE',  ( 92.35000000007822507, -209.9999869687480611, 79.28395951162927702 ) ) ;
#46455=AXIS2_PLACEMENT_3D ( 'NONE', #5159, #39354, #50997 ) ;
#46462=CARTESIAN_POINT ( 'NONE',  ( -92.69370383062498320, -211.3315407142195852, 78.63614583420049087 ) ) ;
#46469=LINE ( 'NONE', #69392, #16443 ) ;
#46477=CARTESIAN_POINT ( 'NONE',  ( 93.84685191531248449, 91.99731107132950569, 88.42572916753381662 ) ) ;
#46482=CARTESIAN_POINT ( 'NONE',  ( -92.69370383062504004, 90.00000000000004263, 79.16531250086714522 ) ) ;
#46483=CARTESIAN_POINT ( 'NONE',  ( 97.30629616937498838, -209.9999999999999716, 87.42031250086714067 ) ) ;
#46484=ADVANCED_FACE ( 'NONE', ( #72668 ), #21546, .F. ) ;
#46486=CARTESIAN_POINT ( 'NONE',  ( 96.32499999999998863, -212.2949673200287179, 80.13104166840095388 ) ) ;
#46498=CARTESIAN_POINT ( 'NONE',  ( 95.00000000000000000, -212.6630814284392557, 81.07031250086716057 ) ) ;
#46499=CARTESIAN_POINT ( 'NONE',  ( 92.34999999999999432, 90.00000000000002842, 90.00000000000000000 ) ) ;
#46503=CARTESIAN_POINT ( 'NONE',  ( 97.64998666484400758, 91.52998591240842075, 83.46479220096851748 ) ) ;
#46504=CARTESIAN_POINT ( 'NONE',  ( 2.499999999999984457, -73.00000000000001421, -201.6999999999999886 ) ) ;
#46505=CARTESIAN_POINT ( 'NONE',  ( 97.64999999999999147, -209.9999999999999716, 84.60249999999999204 ) ) ;
#46508=ORIENTED_EDGE ( 'NONE', *, *, #70230, .T. ) ;
#46509=ORIENTED_EDGE ( 'NONE', *, *, #51683, .F. ) ;
#46514=CARTESIAN_POINT ( 'NONE',  ( -92.69370383062502583, 91.33154071421968467, 88.26697916753381890 ) ) ;
#46517=CARTESIAN_POINT ( 'NONE',  ( 96.32499999999998863, -207.7050326799711968, 75.89770833506763381 ) ) ;
#46518=CARTESIAN_POINT ( 'NONE',  ( 96.32499999999997442, 92.29496732002878900, 77.08833333333332405 ) ) ;
#46520=ORIENTED_EDGE ( 'NONE', *, *, #7831, .T. ) ;
#46521=CARTESIAN_POINT ( 'NONE',  ( -92.34999999999999432, -209.9999999999999716, 88.49187500173430010 ) ) ;
#46526=CARTESIAN_POINT ( 'NONE',  ( -95.00000000000002842, 86.94004357329504273, 88.96812500173430749 ) ) ;
#46527=CARTESIAN_POINT ( 'NONE',  ( -92.69370383062505425, 88.66845928578038638, 80.54114583420049200 ) ) ;
#46528=CARTESIAN_POINT ( 'NONE',  ( 92.69370383062498320, 90.00000000000002842, 75.03781250086713328 ) ) ;
#46529=EDGE_CURVE ( 'NONE', #19930, #60050, #48570, .T. ) ;
#46534=CARTESIAN_POINT ( 'NONE',  ( -92.34999999999999432, -210.0000000198591295, 85.95187500101400246 ) ) ;
#46537=ADVANCED_FACE ( 'NONE', ( #3555 ), #73790, .F. ) ;
#46538=CARTESIAN_POINT ( 'NONE',  ( -92.69370383062498320, -209.9999999999999716, 76.62531250086713897 ) ) ;
#46542=ORIENTED_EDGE ( 'NONE', *, *, #67399, .F. ) ;
#46547=CARTESIAN_POINT ( 'NONE',  ( -93.84685191531248449, -208.0026889286704943, 87.68489583420048916 ) ) ;
#46550=AXIS2_PLACEMENT_3D ( 'NONE', #51403, #10825, #5202 ) ;
#46557=AXIS2_PLACEMENT_3D ( 'NONE', #14639, #67262, #61624 ) ;
#46559=CARTESIAN_POINT ( 'NONE',  ( 92.69370383062498320, 91.33154071421968467, 85.14489583420045449 ) ) ;
#46562=CARTESIAN_POINT ( 'NONE',  ( -97.65000000000001990, 90.00000000000004263, 89.44437500173430067 ) ) ;
#46570=CARTESIAN_POINT ( 'NONE',  ( -97.30629616937501680, 90.00000000000004263, 89.64281250086713726 ) ) ;
#46578=CARTESIAN_POINT ( 'NONE',  ( 97.65000000000000568, -208.4700217866474645, 75.84479166840098685 ) ) ;
#46584=CARTESIAN_POINT ( 'NONE',  ( 97.30629616937498838, -208.6684592857803011, 83.82197916753382572 ) ) ;
#46588=VERTEX_POINT ( 'NONE', #24162 ) ;
#46592=( BOUNDED_CURVE ( )  B_SPLINE_CURVE ( 2, ( #65423, #6782, #1558, #30077, #70287, #18790, #44715, #3384, #49952 ),
 .UNSPECIFIED., .F., .F. ) 
 B_SPLINE_CURVE_WITH_KNOTS ( ( 3, 2, 2, 2, 3 ),
 ( 0.000000000000000000, 0.007055765540882354830, 0.01411153108176470966, 0.02116729662264706449, 0.02116741234826875415 ),
 .UNSPECIFIED. ) 
 CURVE ( )  GEOMETRIC_REPRESENTATION_ITEM ( )  RATIONAL_B_SPLINE_CURVE ( ( 1.000000000000000000, 0.8660254037844387076, 1.000000000000000000, 0.8660254037844387076, 1.000000000000000000, 0.8660254037844387076, 1.000000000000000000, 0.9999978026064856307, 0.9999956052850527133 ) ) 
 REPRESENTATION_ITEM ( '' )  );
#46593=CARTESIAN_POINT ( 'NONE',  ( 95.00000000000000000, -207.3369185715606307, 74.87906250086713555 ) ) ;
#46596=CARTESIAN_POINT ( 'NONE',  ( 97.30629616937498838, -211.3315407142195852, 78.63614583420049087 ) ) ;
#46600=ORIENTED_EDGE ( 'NONE', *, *, #68832, .T. ) ;
#46605=VECTOR ( 'NONE', #14390, 1000.000000000000000 ) ;
#46608=CARTESIAN_POINT ( 'NONE',  ( 92.35000000000000853, -209.9999999999999716, 87.53937500173429953 ) ) ;
#46614=CARTESIAN_POINT ( 'NONE',  ( 93.67499999999999716, 87.70503267997126784, 86.37520833506764006 ) ) ;
#46615=ORIENTED_EDGE ( 'NONE', *, *, #43208, .F. ) ;
#46626=CARTESIAN_POINT ( 'NONE',  ( 94.99999999999998579, 93.05995642670504253, 79.76062500173429726 ) ) ;
#46629=CARTESIAN_POINT ( 'NONE',  ( -95.00000000000002842, 93.05995642670501411, 88.57124999999999204 ) ) ;
#46632=CARTESIAN_POINT ( 'NONE',  ( 93.84685191531248449, 88.00268892867053694, 75.14364583420046984 ) ) ;
#46634=EDGE_LOOP ( 'NONE', ( #31325, #16748, #40121, #3572 ) ) ;
#46636=CARTESIAN_POINT ( 'NONE',  ( -93.84685191531248449, -208.0026889286704943, 81.17614583420048291 ) ) ;
#46639=CARTESIAN_POINT ( 'NONE',  ( 92.59666252161194677, -210.8453944377487232, 74.93511027845777051 ) ) ;
#46641=CARTESIAN_POINT ( 'NONE',  ( -96.15314808468745866, -211.9973110713294489, 77.04864583420047097 ) ) ;
#46643=CARTESIAN_POINT ( 'NONE',  ( 92.34999999999999432, 90.00000000000002842, 83.01499999999998636 ) ) ;
#46645=LINE ( 'NONE', #63950, #57618 ) ;
#46648=CARTESIAN_POINT ( 'NONE',  ( -92.69370383062504004, 90.00000000000004263, 77.26031250086714408 ) ) ;
#46661=CARTESIAN_POINT ( 'NONE',  ( 1.243286885786405054E-17, -120.0000000000000000, 127.5000000000000000 ) ) ;
#46662=CARTESIAN_POINT ( 'NONE',  ( -93.84685191531248449, -208.0026889286704943, 76.88989583420048746 ) ) ;
#46666=CYLINDRICAL_SURFACE ( 'NONE', #14254, 2.649999999999985700 ) ;
#46667=CARTESIAN_POINT ( 'NONE',  ( 2.500000000000029754, 73.00000000000001421, -201.6999999999999886 ) ) ;
#46668=DIRECTION ( 'NONE',  ( -0.000000000000000000, -0.000000000000000000, 1.000000000000000000 ) ) ;
#46673=EDGE_CURVE ( 'NONE', #11821, #32195, #56261, .T. ) ;
#46678=EDGE_CURVE ( 'NONE', #30123, #70981, #46349, .T. ) ;
#46684=CARTESIAN_POINT ( 'NONE',  ( 95.00000000000000000, -212.6630814284392557, 83.45156250086714067 ) ) ;
#46686=ORIENTED_EDGE ( 'NONE', *, *, #64256, .T. ) ;
#46690=CARTESIAN_POINT ( 'NONE',  ( 92.35000000003290666, -209.9999916046337205, 84.99910573348564924 ) ) ;
#46692=CARTESIAN_POINT ( 'NONE',  ( -96.15314808468751551, 88.00268892867056536, 79.11239583420048405 ) ) ;
#46695=ORIENTED_EDGE ( 'NONE', *, *, #11068, .F. ) ;
#46704=CARTESIAN_POINT ( 'NONE',  ( 94.20702885560666573, 87.49569407151196287, 74.98272308147875265 ) ) ;
#46708=VECTOR ( 'NONE', #10132, 1000.000000000000000 ) ;
#46711=CARTESIAN_POINT ( 'NONE',  ( 92.69370383062501162, -209.9999999999999716, 81.38781250086714181 ) ) ;
#46717=CARTESIAN_POINT ( 'NONE',  ( -95.00000000000002842, 86.94004357329504273, 84.44374999999999432 ) ) ;
#46719=AXIS2_PLACEMENT_3D ( 'NONE', #31124, #60463, #64994 ) ;
#46722=CARTESIAN_POINT ( 'NONE',  ( -96.32500000000001705, 87.70503267997129626, 82.48583333333333201 ) ) ;
#46723=CARTESIAN_POINT ( 'NONE',  ( -92.69370383062498320, -208.6684592857803011, 85.56822916753380071 ) ) ;
#46724=CARTESIAN_POINT ( 'NONE',  ( -96.15314808468752972, 91.99731107132950569, 80.80572916753382628 ) ) ;
#46726=CARTESIAN_POINT ( 'NONE',  ( 92.69370383062498320, 88.66845928578037217, 85.88572916753382458 ) ) ;
#46731=CARTESIAN_POINT ( 'NONE',  ( -95.00000000000002842, 90.00000000000004263, 90.00000000000000000 ) ) ;
#46733=CARTESIAN_POINT ( 'NONE',  ( -92.69370383062498320, -209.9999999999999716, 88.05531250086713158 ) ) ;
#46738=CARTESIAN_POINT ( 'NONE',  ( 94.99999999999998579, 93.05995642670504253, 80.31624999999999659 ) ) ;
#46743=AXIS2_PLACEMENT_3D ( 'NONE', #67962, #32620, #45037 ) ;
#46745=CARTESIAN_POINT ( 'NONE',  ( -92.35000000000005116, 88.47002178664754979, 76.92958333333332632 ) ) ;
#46747=CARTESIAN_POINT ( 'NONE',  ( -97.30629616937501680, 91.33154071421968467, 87.04989583420048405 ) ) ;
#46748=CARTESIAN_POINT ( 'NONE',  ( 95.00000000000000000, -206.9400435732949575, 80.95125000000000171 ) ) ;
#46749=CARTESIAN_POINT ( 'NONE',  ( -97.65000000000003411, 90.00000000000004263, 75.00000000000000000 ) ) ;
#46754=CARTESIAN_POINT ( 'NONE',  ( -95.00000000000002842, 87.33691857156074434, 79.00656250086713328 ) ) ;
#46760=CARTESIAN_POINT ( 'NONE',  ( -97.30629616937497417, -211.3315407142195852, 84.77447916753381207 ) ) ;
#46766=CARTESIAN_POINT ( 'NONE',  ( 93.84685191531248449, 88.00268892867053694, 77.20739583420048291 ) ) ;
#46769=CARTESIAN_POINT ( 'NONE',  ( -94.99999999999997158, -212.6630814284392557, 75.99031250086716227 ) ) ;
#46777=CARTESIAN_POINT ( 'NONE',  ( -93.33864827737279768, 88.39919842643631398, 74.79754476654878204 ) ) ;
#46778=CARTESIAN_POINT ( 'NONE',  ( 97.30629616937498838, -208.6684592857803011, 77.94822916753381037 ) ) ;
#46782=EDGE_CURVE ( 'NONE', #27645, #49121, #9697, .T. ) ;
#46785=AXIS2_PLACEMENT_3D ( 'NONE', #8992, #61249, #60872 ) ;
#46799=CARTESIAN_POINT ( 'NONE',  ( 92.69370383062498320, 88.66845928578037217, 82.86947916753382515 ) ) ;
#46800=CARTESIAN_POINT ( 'NONE',  ( -92.35000000000553655, 89.99999459739531460, 81.50687481489494246 ) ) ;
#46804=ORIENTED_EDGE ( 'NONE', *, *, #55860, .T. ) ;
#46815=CARTESIAN_POINT ( 'NONE',  ( -92.34999999999999432, -209.9999999999999716, 77.69687500173431260 ) ) ;
#46819=CARTESIAN_POINT ( 'NONE',  ( 92.34999999999999432, 90.00000000000002842, 79.28437500173430408 ) ) ;
#46820=CARTESIAN_POINT ( 'NONE',  ( -97.65000000000001990, 91.52997821335253548, 77.32645833506762756 ) ) ;
#46821=( BOUNDED_CURVE ( )  B_SPLINE_CURVE ( 2, ( #31622, #30511, #30148, #24513, #36525, #53456, #36896 ),
 .UNSPECIFIED., .F., .F. ) 
 B_SPLINE_CURVE_WITH_KNOTS ( ( 3, 2, 2, 3 ),
 ( 0.2328402629031412763, 0.2398960283911786839, 0.2469517939320956812, 0.2540073681295598185 ),
 .UNSPECIFIED. ) 
 CURVE ( )  GEOMETRIC_REPRESENTATION_ITEM ( )  RATIONAL_B_SPLINE_CURVE ( ( 1.000000000000000000, 0.8660254037844387076, 1.000000000000000000, 0.8660254037844387076, 1.000000000000000000, 0.8660290370063311594, 0.9999927337532719118 ) ) 
 REPRESENTATION_ITEM ( '' )  );
#46822=VECTOR ( 'NONE', #40628, 1000.000000000000000 ) ;
#46824=CARTESIAN_POINT ( 'NONE',  ( 97.30629616937498838, 88.66845928578037217, 79.90614583420048689 ) ) ;
#46826=CARTESIAN_POINT ( 'NONE',  ( 92.35000000003357457, 89.99999234487445676, 78.01464417100922333 ) ) ;
#46828=CARTESIAN_POINT ( 'NONE',  ( 96.32499999999998863, -212.2949673200287179, 79.49604166840096298 ) ) ;
#46834=VERTEX_POINT ( 'NONE', #31629 ) ;
#46840=CARTESIAN_POINT ( 'NONE',  ( -97.30629616937495996, -209.9999999999999716, 77.10156250086714635 ) ) ;
#46847=CARTESIAN_POINT ( 'NONE',  ( 92.35004149090329406, 88.46999783186332422, 85.68729332542760346 ) ) ;
#46854=CARTESIAN_POINT ( 'NONE',  ( 96.32499999999997442, 92.29496732002878900, 86.05770833506763040 ) ) ;
#46859=CARTESIAN_POINT ( 'NONE',  ( 96.15314808468748708, 91.99731107132950569, 87.04989583420048405 ) ) ;
#46861=CARTESIAN_POINT ( 'NONE',  ( -97.30629616937497417, -208.6684592857803295, 85.93864583420051417 ) ) ;
#46862=DIRECTION ( 'NONE',  ( -0.000000000000000000, -0.000000000000000000, 1.000000000000000000 ) ) ;
#46864=CARTESIAN_POINT ( 'NONE',  ( -95.00000000000002842, 93.05995642670504253, 81.58624999999999261 ) ) ;
#46865=CARTESIAN_POINT ( 'NONE',  ( -96.32499999999996021, -212.2949673200287179, 81.85083333333332689 ) ) ;
#46866=CARTESIAN_POINT ( 'NONE',  ( -95.00000000000002842, 87.33691857156074434, 76.46656250086712703 ) ) ;
#46867=CARTESIAN_POINT ( 'NONE',  ( 97.30629616937498838, -211.3315407142195852, 86.09739583420048348 ) ) ;
#46869=CARTESIAN_POINT ( 'NONE',  ( 97.64999999954044085, 90.00004935162768049, 87.22187670868791542 ) ) ;
#46877=EDGE_LOOP ( 'NONE', ( #71530, #39430, #38934, #18249 ) ) ;
#46878=CARTESIAN_POINT ( 'NONE',  ( 92.69370383062501162, -208.6684592857803295, 80.85864583420048746 ) ) ;
#46881=ADVANCED_FACE ( 'NONE', ( #7965 ), #19609, .F. ) ;
#46887=CARTESIAN_POINT ( 'NONE',  ( 97.64999999999997726, -208.4700217866474645, 85.92541666666664923 ) ) ;
#46896=CARTESIAN_POINT ( 'NONE',  ( -96.15314808468751551, 88.00268892867056536, 87.36739583420049371 ) ) ;
#46899=CARTESIAN_POINT ( 'NONE',  ( 96.32499999999998863, -207.7050326799711968, 78.43770833506764006 ) ) ;
#46900=CARTESIAN_POINT ( 'NONE',  ( 96.15314808468750130, -211.9973110713294489, 87.94947916753380923 ) ) ;
#46901=CARTESIAN_POINT ( 'NONE',  ( 92.34999999999999432, 90.00000000000002842, 78.57000000000000739 ) ) ;
#46907=CARTESIAN_POINT ( 'NONE',  ( -92.35000000000005116, 88.47002178664754979, 89.07395833506762983 ) ) ;
#46908=CARTESIAN_POINT ( 'NONE',  ( 94.99999999999998579, 87.33691857156068750, 75.83156250086715033 ) ) ;
#46912=CARTESIAN_POINT ( 'NONE',  ( 92.34999999999999432, 90.00000000000002842, 84.28499999999999659 ) ) ;
#46921=CARTESIAN_POINT ( 'NONE',  ( -93.67500000000003979, 92.29496732002878900, 75.26270833506764291 ) ) ;
#46923=CARTESIAN_POINT ( 'NONE',  ( -92.69370383062498320, -209.9999999999999716, 89.48406250086715374 ) ) ;
#46927=ADVANCED_FACE ( 'NONE', ( #32367 ), #27464, .F. ) ;
#46932=CARTESIAN_POINT ( 'NONE',  ( 96.15314808468748708, 91.99731107132950569, 80.54114583420046358 ) ) ;
#46936=CARTESIAN_POINT ( 'NONE',  ( -93.67500000000003979, 92.29496732002878900, 85.34333333333333371 ) ) ;
#46946=CARTESIAN_POINT ( 'NONE',  ( -96.15314808468751551, 88.00268892867056536, 85.93864583420048575 ) ) ;
#46949=( BOUNDED_CURVE ( )  B_SPLINE_CURVE ( 2, ( #66045, #60404, #31802, #43853, #50582, #56619, #74257 ),
 .UNSPECIFIED., .F., .F. ) 
 B_SPLINE_CURVE_WITH_KNOTS ( ( 3, 2, 2, 3 ),
 ( 0.3598440426548558668, 0.3668998081276851342, 0.3739555736686021037, 0.3810111478283708664 ),
 .UNSPECIFIED. ) 
 CURVE ( )  GEOMETRIC_REPRESENTATION_ITEM ( )  RATIONAL_B_SPLINE_CURVE ( ( 1.000000000000000000, 0.8660254037844387076, 1.000000000000000000, 0.8660254037844387076, 1.000000000000000000, 0.8660290377220891678, 0.9999927323218336106 ) ) 
 REPRESENTATION_ITEM ( '' )  );
#46950=CARTESIAN_POINT ( 'NONE',  ( -94.99999999999997158, -209.9999999999999716, 90.00000000000000000 ) ) ;
#46957=CARTESIAN_POINT ( 'NONE',  ( 92.35000000000000853, 91.52997821335253548, 77.24708333333332178 ) ) ;
#46959=CARTESIAN_POINT ( 'NONE',  ( 93.84685191531251292, -211.9973110713294489, 82.28739583420048120 ) ) ;
#46962=EDGE_CURVE ( 'NONE', #3079, #54593, #20219, .T. ) ;
#46967=CARTESIAN_POINT ( 'NONE',  ( 97.30629616937498838, -211.3315407142195852, 75.30239583420048177 ) ) ;
#46969=CARTESIAN_POINT ( 'NONE',  ( 92.69370383062501162, -211.3315407142195852, 80.32947916753381890 ) ) ;
#46982=CARTESIAN_POINT ( 'NONE',  ( 93.67500000000001137, -207.7050326799711968, 88.06854166840095388 ) ) ;
#46983=CARTESIAN_POINT ( 'NONE',  ( 92.34999999999999432, 91.52997821335252127, 87.40708333333333258 ) ) ;
#46989=ORIENTED_EDGE ( 'NONE', *, *, #2890, .F. ) ;
#46992=CARTESIAN_POINT ( 'NONE',  ( 96.32499999999998863, 87.70503267997126784, 86.48104166840096241 ) ) ;
#46997=CARTESIAN_POINT ( 'NONE',  ( -94.99999999999997158, -206.9400435732949575, 75.23624999999998408 ) ) ;
#46998=VERTEX_POINT ( 'NONE', #33102 ) ;
#47000=ORIENTED_EDGE ( 'NONE', *, *, #4199, .F. ) ;
#47005=CARTESIAN_POINT ( 'NONE',  ( -97.65000000000001990, 91.52997821335253548, 88.04208333333332348 ) ) ;
#47012=CARTESIAN_POINT ( 'NONE',  ( -93.84685191531248449, -208.0026889286704943, 82.44614583420046472 ) ) ;
#47017=CARTESIAN_POINT ( 'NONE',  ( -93.84685191531248449, -208.0026889286704943, 75.46114583420047950 ) ) ;
#47025=CARTESIAN_POINT ( 'NONE',  ( 92.34999999999999432, 89.99996511148934530, 83.09437620840749616 ) ) ;
#47026=CARTESIAN_POINT ( 'NONE',  ( 92.34999999999998010, 90.00002373248486265, 79.91937418090952860 ) ) ;
#47027=CARTESIAN_POINT ( 'NONE',  ( -92.69370383062502583, 91.33154071421968467, 79.85322916753379729 ) ) ;
#47035=CARTESIAN_POINT ( 'NONE',  ( 95.00000000000000000, -209.9999999999999716, 90.00000000000000000 ) ) ;
#47040=CARTESIAN_POINT ( 'NONE',  ( -93.84685191531247028, -211.9973110713294489, 75.40822916753381833 ) ) ;
#47044=( BOUNDED_CURVE ( )  B_SPLINE_CURVE ( 2, ( #7174, #30091, #53036, #9014, #48133, #70667, #71781 ),
 .UNSPECIFIED., .F., .F. ) 
 B_SPLINE_CURVE_WITH_KNOTS ( ( 3, 2, 2, 3 ),
 ( 0.8958333333333331483, 0.9027777777777775681, 0.9097222222222218768, 0.9166666666666662966 ),
 .UNSPECIFIED. ) 
 CURVE ( )  GEOMETRIC_REPRESENTATION_ITEM ( )  RATIONAL_B_SPLINE_CURVE ( ( 1.000000000000004219, 0.8660254037844343777, 1.000000000000000000, 0.8660254037844387076, 1.000000000000000000, 0.8660254037844451469, 0.9999999999999935607 ) ) 
 REPRESENTATION_ITEM ( '' )  );
#47061=ORIENTED_EDGE ( 'NONE', *, *, #43127, .T. ) ;
#47062=CARTESIAN_POINT ( 'NONE',  ( 97.30629616937498838, -211.3315407142195852, 86.09739583420048348 ) ) ;
#47064=VERTEX_POINT ( 'NONE', #28959 ) ;
#47065=CARTESIAN_POINT ( 'NONE',  ( 93.84685191531249870, -208.0026889286704943, 89.69572916753382685 ) ) ;
#47066=EDGE_CURVE ( 'NONE', #36714, #38565, #22218, .T. ) ;
#47070=CARTESIAN_POINT ( 'NONE',  ( -95.00000000000002842, 87.33691857156074434, 79.16531250086715943 ) ) ;
#47076=FACE_OUTER_BOUND ( 'NONE', #57900, .T. ) ;
#47079=ORIENTED_EDGE ( 'NONE', *, *, #57126, .F. ) ;
#47084=VECTOR ( 'NONE', #3382, 1000.000000000000000 ) ;
#47087=CARTESIAN_POINT ( 'NONE',  ( 96.15314808468748708, -208.0026889286704943, 81.81114583420047381 ) ) ;
#47092=CYLINDRICAL_SURFACE ( 'NONE', #72527, 3.299999999999969624 ) ;
#47093=DIRECTION ( 'NONE',  ( -1.000000000000000000, 3.061616997868382648E-16, 0.000000000000000000 ) ) ;
#47096=CARTESIAN_POINT ( 'NONE',  ( -97.30629616937497417, -211.3315407142195852, 84.61572916753380014 ) ) ;
#47097=CARTESIAN_POINT ( 'NONE',  ( -97.30629616937501680, 88.66845928578038638, 83.50447916753383026 ) ) ;
#47100=CARTESIAN_POINT ( 'NONE',  ( 92.69370383062498320, 88.66845928578037217, 82.07572916753380809 ) ) ;
#47107=CARTESIAN_POINT ( 'NONE',  ( -96.15314808468747287, -208.0026889286704943, 86.36197916753381776 ) ) ;
#47115=EDGE_CURVE ( 'NONE', #59848, #43302, #63959, .T. ) ;
#47120=CARTESIAN_POINT ( 'NONE',  ( -94.99999999999997158, -213.0599564267049857, 78.72875000000001933 ) ) ;
#47121=CARTESIAN_POINT ( 'NONE',  ( -93.84685191531252713, 88.00268892867056536, 87.94947916753380923 ) ) ;
#47133=CARTESIAN_POINT ( 'NONE',  ( -97.30629616937497417, -211.3315407142195852, 86.67947916753382742 ) ) ;
#47134=EDGE_CURVE ( 'NONE', #54372, #15642, #39514, .T. ) ;
#47137=CARTESIAN_POINT ( 'NONE',  ( -92.69370383062498320, -208.6684592857803295, 76.83697916753382628 ) ) ;
#47142=CARTESIAN_POINT ( 'NONE',  ( -97.64999999999996305, -209.9999999999999716, 90.00000000000000000 ) ) ;
#47143=EDGE_CURVE ( 'NONE', #18128, #40405, #50539, .T. ) ;
#47146=CARTESIAN_POINT ( 'NONE',  ( -96.15314808468751551, 88.00268892867056536, 75.30239583420048177 ) ) ;
#47147=CARTESIAN_POINT ( 'NONE',  ( 95.00000000000000000, -207.3369185715606307, 77.41906250086714181 ) ) ;
#47148=ORIENTED_EDGE ( 'NONE', *, *, #61882, .T. ) ;
#47150=VERTEX_POINT ( 'NONE', #59388 ) ;
#47151=VECTOR ( 'NONE', #4444, 1000.000000000000000 ) ;
#47153=ORIENTED_EDGE ( 'NONE', *, *, #16728, .F. ) ;
#47162=ORIENTED_EDGE ( 'NONE', *, *, #28162, .T. ) ;
#47163=CARTESIAN_POINT ( 'NONE',  ( 94.99999999999998579, 92.66308142843935514, 78.84781250086714977 ) ) ;
#47164=CARTESIAN_POINT ( 'NONE',  ( 97.64999999999999147, 90.00000000000002842, 76.34749999999999659 ) ) ;
#47166=VERTEX_POINT ( 'NONE', #13873 ) ;
#47168=VERTEX_POINT ( 'NONE', #7516 ) ;
#47170=VERTEX_POINT ( 'NONE', #47369 ) ;
#47177=CARTESIAN_POINT ( 'NONE',  ( -96.32499999999996021, -212.2949673200287179, 78.75520833506763552 ) ) ;
#47179=CARTESIAN_POINT ( 'NONE',  ( 7.103376864691351012E-17, -120.0000000000000000, -80.00000000000000000 ) ) ;
#47181=CARTESIAN_POINT ( 'NONE',  ( 96.32499999999998863, 87.70503267997126784, 80.76604166840097321 ) ) ;
#47182=CARTESIAN_POINT ( 'NONE',  ( -96.32500000000001705, 92.29496732002878900, 75.36854166840096525 ) ) ;
#47184=CARTESIAN_POINT ( 'NONE',  ( 92.69370383062498320, 90.00000000000002842, 79.00656250086716170 ) ) ;
#47191=EDGE_LOOP ( 'NONE', ( #43526, #51484, #5757, #34116 ) ) ;
#47192=CARTESIAN_POINT ( 'NONE',  ( 92.35000000000000853, -209.9999999999999716, 77.29999999999999716 ) ) ;
#47203=CARTESIAN_POINT ( 'NONE',  ( -92.69370383062498320, -209.9999999999999716, 78.05406250086716113 ) ) ;
#47204=EDGE_CURVE ( 'NONE', #47170, #69481, #65409, .T. ) ;
#47209=VECTOR ( 'NONE', #15384, 1000.000000000000000 ) ;
#47211=FACE_OUTER_BOUND ( 'NONE', #10475, .T. ) ;
#47214=DIRECTION ( 'NONE',  ( -0.000000000000000000, -0.000000000000000000, -1.000000000000000000 ) ) ;
#47217=CARTESIAN_POINT ( 'NONE',  ( -97.64999999999996305, -209.9999999999999716, 78.01437500173430806 ) ) ;
#47221=CARTESIAN_POINT ( 'NONE',  ( 97.30629616937498838, 88.66845928578035796, 86.89114583420048632 ) ) ;
#47222=CARTESIAN_POINT ( 'NONE',  ( -92.69370383062498320, -208.6684592857803295, 87.63197916753381378 ) ) ;
#47226=CARTESIAN_POINT ( 'NONE',  ( -94.99999999999997158, -206.9400435732949575, 82.22124999999999773 ) ) ;
#47227=CARTESIAN_POINT ( 'NONE',  ( -93.84685191531252713, 88.00268892867056536, 75.24947916753380639 ) ) ;
#47228=EDGE_CURVE ( 'NONE', #28732, #49041, #54080, .T. ) ;
#47230=CARTESIAN_POINT ( 'NONE',  ( 95.00000000000000000, -207.3369185715606307, 88.21406250086714351 ) ) ;
#47231=ORIENTED_EDGE ( 'NONE', *, *, #55879, .T. ) ;
#47236=DIRECTION ( 'NONE',  ( 0.000000000000000000, 0.000000000000000000, 1.000000000000000000 ) ) ;
#47241=CARTESIAN_POINT ( 'NONE',  ( 93.84685191531249870, -208.0026889286704943, 82.71072916753381321 ) ) ;
#47245=( BOUNDED_SURFACE ( )  B_SPLINE_SURFACE ( 1, 2, ( 
 ( #2473, #31720, #55029, #14805, #43024, #26457, #25719, #59956, #32460, #49391, #59572, #49747, #72671, #20817, #43769, #3192, #26083, #9166, #65587, #8801, #21173, #54304, #48657, #49012, #43411, #25358, #65217, #13690, #71194, #3559, #65965, #20458, #37752, #14054, #36627, #42649, #66689, #60325, #8058, #31353, #72319, #60688, #71573, #20068, #57264, #44508, #67425, #45251, #15554, #22306, #17038, #67799, #28676, #16292, #5769, #15922, #38854, #68167, #38488, #16667, #39975, #61798, #39606, #33200, #62548, #56145, #11028, #56900, #62929, #50869, #27939, #10279, #33953, #4664, #27571, #50499, #5408, #168, #28302, #11387, #34321, #73425, #51239, #74171, #61426, #21934, #44876, #9906, #22685, #45633, #68552, #39233, #27182, #73793, #62162, #10649, #33575, #56532, #51616, #5034, #44123, #67048, #32826, #55776, #4293, #50110, #73045, #21551, #64386, #64756, #30155, #52727, #45989, #24165, #69648, #70362, #23059, #7242, #11743, #47097, #46352, #29403, #7605, #1638, #13241, #6143, #36169, #12495, #18871, #53099, #29048, #6503, #24522, #69281, #51980, #47457, #30518, #35433, #34690, #64020, #12859, #70002, #898, #58743, #57999, #17767, #41809, #59116, #17403, #53466, #68916, #40337, #63284, #58362, #6863, #41443, #23421, #41088, #57644, #12126, #35067, #29774, #1278, #526, #40713, #63657, #52350, #35788, #23784, #18503, #46724, #18142, #24891, #30887, #32000, #2746, #9444, #2001, #20362, #66599, #13607, #43318, #25631, #37300, #48922, #25272, #47820, #53830, #54941, #48565, #32369, #70741, #66238, #71479, #60952, #19979, #15080, #2380, #48197, #3102, #19248, #54576, #49296, #71107, #71845, #65499, #14713, #13965, #25996, #37664, #72220, #8714, #60237, #19613, #60599, #42559, #36910, #59856, #9076, #42198, #3461, #20724, #43680, #8344, #26366, #38021, #65131, #31268, #54216, #36533, #59480, #7969, #42935, #65866, #14350, #31633, #27092, #38764, #61702, #33104, #39889, #67709, #39516, #50775, #73704, #39137, #27847, #10939, #62459, #16570, #22214, #22592, #33862, #10554, #3830, #56437, #27468, #28217, #55312, #56808, #44040, #4949, #4198, #10183, #62838, #5319, #45537, #38397, #68462, #44786, #51147, #74079, #61337, #56054, #16952, #50022, #9816, #11300, #26725, #16199, #66955, #21839, #45156, #68078, #4571, #49655, #15835 ),
 ( #55683, #72949, #72583, #21082, #67335, #15451, #32732, #50405, #73331, #62074, #21452, #33476, #44413, #64660, #40249, #41360, #12040, #58278, #45905, #6772, #23334, #30066, #41719, #47371, #28962, #64300, #17685, #46629, #12771, #69558, #35699, #1183, #63563, #41001, #34233, #57549, #24082, #47005, #57178, #69194, #18058, #40623, #23695, #34981, #28583, #58646, #57916, #24433, #69916, #29685, #7148, #63932, #29320, #11658, #6418, #5682, #52263, #807, #12404, #51524, #80, #17316, #70273, #22974, #46263, #68829, #63197, #34600, #18415, #35353, #52634, #53015, #1548, #18779, #6058, #51897, #438, #36084, #30794, #7518, #14629, #3017, #71388, #13519, #36445, #36814, #37204, #59030, #71023, #13144, #30428, #53377, #19523, #2659, #37574, #1916, #24799, #59391, #7879, #71755, #54482, #42473, #65769, #60148, #8631, #47731, #43228, #48474, #20262, #59763, #31174, #70644, #66150, #19156, #54126, #25909, #13875, #48836, #65412, #42108, #65044, #25538, #53741, #2285, #25177, #48106, #14255, #8246, #19890, #42837, #31539, #67818, #21568, #72337, #3574, #5054, #3943, #26843, #32846, #38504, #10668, #22327, #15936, #56163, #32479, #21950, #49769, #4683, #60707, #9924, #72687, #21190, #45270, #20836, #44896, #67068, #38876, #26478, #61816, #44144, #33593, #14823, #27955, #9560, #16314, #15570, #27197, #39253, #50131, #62181, #27589, #61444, #44525, #37774, #38127, #50516, #73445, #9184, #55796, #73066, #4313, #67444, #10301, #32108, #56552, #33217, #50889, #73812, #55047, #49411, #43790, #66708, #15192, #61067, #55424, #68936, #17424, #6165, #24184, #68191, #51257, #58383, #16689, #5793, #56919, #74194, #22709, #58015, #63300, #63677, #23442, #12515, #914, #39622, #62569, #1295, #11052, #28699, #33970, #5426, #41107, #40733, #39993, #11407, #57659, #29423, #28321, #40356, #45650, #29796, #52751, #51636, #34715, #35451, #6880, #64039, #68571, #17061, #52369, #12144, #187, #545, #17785, #46370, #18164, #23804, #11762, #46745, #23079, #29068, #69666, #6520, #62948, #46007, #35089, #34340, #57280, #51994, #69297, #48587, #18887, #65516, #54595, #30906, #59503, #1658, #3122, #8368, #7620, #41831, #42955, #31284, #41465, #71498, #19997, #2765, #25649, #36551, #65889, #53853, #30174, #35809, #37318, #36191, #59134, #65153, #25290 ) ),
 .UNSPECIFIED., .F., .F., .F. ) 
 B_SPLINE_SURFACE_WITH_KNOTS ( ( 2, 2 ),
 ( 3, 2, 2, 2, 2, 2, 2, 2, 2, 2, 2, 2, 2, 2, 2, 2, 2, 2, 2, 2, 2, 2, 2, 2, 2, 2, 2, 2, 2, 2, 2, 2, 2, 2, 2, 2, 2, 2, 2, 2, 2, 2, 2, 2, 2, 2, 2, 2, 2, 2, 2, 2, 2, 2, 2, 2, 2, 2, 2, 2, 2, 2, 2, 2, 2, 2, 2, 2, 2, 2, 2, 2, 2, 2, 2, 2, 2, 2, 2, 2, 2, 2, 2, 2, 2, 2, 2, 2, 2, 2, 2, 2, 2, 2, 2, 2, 2, 2, 2, 2, 2, 2, 2, 2, 2, 2, 2, 2, 2, 2, 2, 2, 2, 2, 2, 2, 2, 2, 2, 2, 2, 2, 2, 2, 2, 2, 2, 2, 2, 2, 2, 2, 2, 2, 2, 2, 2, 2, 2, 2, 2, 2, 2, 3 ),
 ( 0.000000000000000000, 1.000000000000000000 ),
 ( 0.000000000000000000, 0.006944444444444444059, 0.01388888888888888812, 0.02083333333333333218, 0.02777777777777777624, 0.03472222222222222376, 0.04166666666666666435, 0.04861111111111111188, 0.05555555555555555247, 0.06250000000000000000, 0.06944444444444444753, 0.07638888888888889506, 0.08333333333333332871, 0.09027777777777777624, 0.09722222222222222376, 0.1041666666666666713, 0.1111111111111111049, 0.1180555555555555525, 0.1250000000000000000, 0.1319444444444444475, 0.1388888888888888951, 0.1458333333333333426, 0.1527777777777777901, 0.1597222222222222099, 0.1666666666666666574, 0.1736111111111111049, 0.1805555555555555525, 0.1875000000000000000, 0.1944444444444444475, 0.2013888888888888951, 0.2083333333333333426, 0.2152777777777777901, 0.2222222222222222099, 0.2291666666666666574, 0.2361111111111111049, 0.2430555555555555525, 0.2500000000000000000, 0.2569444444444444198, 0.2638888888888888951, 0.2708333333333333148, 0.2777777777777777901, 0.2847222222222222099, 0.2916666666666666852, 0.2986111111111111049, 0.3055555555555555802, 0.3125000000000000000, 0.3194444444444444198, 0.3263888888888888951, 0.3333333333333333148, 0.3402777777777777901, 0.3472222222222222099, 0.3541666666666666852, 0.3611111111111111049, 0.3680555555555555802, 0.3750000000000000000, 0.3819444444444444198, 0.3888888888888888951, 0.3958333333333333148, 0.4027777777777777901, 0.4097222222222222099, 0.4166666666666666852, 0.4236111111111111049, 0.4305555555555555802, 0.4375000000000000000, 0.4444444444444444198, 0.4513888888888888951, 0.4583333333333333148, 0.4652777777777777901, 0.4722222222222222099, 0.4791666666666666852, 0.4861111111111111049, 0.4930555555555555802, 0.5000000000000000000, 0.5069444444444444198, 0.5138888888888888395, 0.5208333333333333703, 0.5277777777777777901, 0.5347222222222222099, 0.5416666666666666297, 0.5486111111111111605, 0.5555555555555555802, 0.5625000000000000000, 0.5694444444444444198, 0.5763888888888888395, 0.5833333333333333703, 0.5902777777777777901, 0.5972222222222222099, 0.6041666666666666297, 0.6111111111111111605, 0.6180555555555555802, 0.6250000000000000000, 0.6319444444444444198, 0.6388888888888888395, 0.6458333333333333703, 0.6527777777777777901, 0.6597222222222222099, 0.6666666666666666297, 0.6736111111111111605, 0.6805555555555555802, 0.6875000000000000000, 0.6944444444444444198, 0.7013888888888888395, 0.7083333333333333703, 0.7152777777777777901, 0.7222222222222222099, 0.7291666666666666297, 0.7361111111111111605, 0.7430555555555555802, 0.7500000000000000000, 0.7569444444444444198, 0.7638888888888888395, 0.7708333333333333703, 0.7777777777777777901, 0.7847222222222222099, 0.7916666666666666297, 0.7986111111111111605, 0.8055555555555555802, 0.8125000000000000000, 0.8194444444444444198, 0.8263888888888888395, 0.8333333333333333703, 0.8402777777777777901, 0.8472222222222222099, 0.8541666666666666297, 0.8611111111111111605, 0.8680555555555555802, 0.8750000000000000000, 0.8819444444444444198, 0.8888888888888888395, 0.8958333333333333703, 0.9027777777777777901, 0.9097222222222222099, 0.9166666666666666297, 0.9236111111111111605, 0.9305555555555555802, 0.9375000000000000000, 0.9444444444444444198, 0.9513888888888888395, 0.9583333333333333703, 0.9652777777777777901, 0.9722222222222222099, 0.9791666666666666297, 0.9842226772312641092, 0.9940649040035767214 ),
 .UNSPECIFIED. ) 
 GEOMETRIC_REPRESENTATION_ITEM ( )  RATIONAL_B_SPLINE_SURFACE ( (
 ( 1.000000000000000000, 0.8660254037844387076, 1.000000000000000000, 0.8660254037844387076, 1.000000000000000000, 0.8660254037844387076, 1.000000000000000000, 0.8660254037844387076, 1.000000000000000000, 0.8660254037844387076, 1.000000000000000000, 0.8660254037844387076, 1.000000000000000000, 0.8660254037844387076, 1.000000000000000000, 0.8660254037844387076, 1.000000000000000000, 0.8660254037844387076, 1.000000000000000000, 0.8660254037844387076, 1.000000000000000000, 0.8660254037844387076, 1.000000000000000000, 0.8660254037844387076, 1.000000000000000000, 0.8660254037844387076, 1.000000000000000000, 0.8660254037844387076, 1.000000000000000000, 0.8660254037844387076, 1.000000000000000000, 0.8660254037844387076, 1.000000000000000000, 0.8660254037844387076, 1.000000000000000000, 0.8660254037844387076, 1.000000000000000000, 0.8660254037844387076, 1.000000000000000000, 0.8660254037844387076, 1.000000000000000000, 0.8660254037844387076, 1.000000000000000000, 0.8660254037844387076, 1.000000000000000000, 0.8660254037844387076, 1.000000000000000000, 0.8660254037844387076, 1.000000000000000000, 0.8660254037844387076, 1.000000000000000000, 0.8660254037844387076, 1.000000000000000000, 0.8660254037844387076, 1.000000000000000000, 0.8660254037844387076, 1.000000000000000000, 0.8660254037844387076, 1.000000000000000000, 0.8660254037844387076, 1.000000000000000000, 0.8660254037844387076, 1.000000000000000000, 0.8660254037844387076, 1.000000000000000000, 0.8660254037844387076, 1.000000000000000000, 0.8660254037844387076, 1.000000000000000000, 0.8660254037844387076, 1.000000000000000000, 0.8660254037844387076, 1.000000000000000000, 0.8660254037844387076, 1.000000000000000000, 0.8660254037844387076, 1.000000000000000000, 0.8660254037844387076, 1.000000000000000000, 0.8660254037844387076, 1.000000000000000000, 0.8660254037844387076, 1.000000000000000000, 0.8660254037844387076, 1.000000000000000000, 0.8660254037844387076, 1.000000000000000000, 0.8660254037844387076, 1.000000000000000000, 0.8660254037844387076, 1.000000000000000000, 0.8660254037844387076, 1.000000000000000000, 0.8660254037844387076, 1.000000000000000000, 0.8660254037844387076, 1.000000000000000000, 0.8660254037844387076, 1.000000000000000000, 0.8660254037844387076, 1.000000000000000000, 0.8660254037844387076, 1.000000000000000000, 0.8660254037844387076, 1.000000000000000000, 0.8660254037844387076, 1.000000000000000000, 0.8660254037844387076, 1.000000000000000000, 0.8660254037844387076, 1.000000000000000000, 0.8660254037844387076, 1.000000000000000000, 0.8660254037844387076, 1.000000000000000000, 0.8660254037844387076, 1.000000000000000000, 0.8660254037844387076, 1.000000000000000000, 0.8660254037844387076, 1.000000000000000000, 0.8660254037844387076, 1.000000000000000000, 0.8660254037844387076, 1.000000000000000000, 0.8660254037844387076, 1.000000000000000000, 0.8660254037844387076, 1.000000000000000000, 0.8660254037844387076, 1.000000000000000000, 0.8660254037844387076, 1.000000000000000000, 0.8660254037844387076, 1.000000000000000000, 0.8660254037844387076, 1.000000000000000000, 0.8660254037844387076, 1.000000000000000000, 0.8660254037844387076, 1.000000000000000000, 0.8660254037844387076, 1.000000000000000000, 0.8660254037844387076, 1.000000000000000000, 0.8660254037844387076, 1.000000000000000000, 0.8660254037844387076, 1.000000000000000000, 0.8660254037844387076, 1.000000000000000000, 0.8660254037844387076, 1.000000000000000000, 0.8660254037844387076, 1.000000000000000000, 0.8660254037844387076, 1.000000000000000000, 0.8660254037844387076, 1.000000000000000000, 0.8660254037844387076, 1.000000000000000000, 0.8660254037844387076, 1.000000000000000000, 0.8660254037844387076, 1.000000000000000000, 0.8660254037844387076, 1.000000000000000000, 0.8660254037844387076, 1.000000000000000000, 0.8660254037844387076, 1.000000000000000000, 0.8660254037844387076, 1.000000000000000000, 0.8660254037844387076, 1.000000000000000000, 0.8660254037844387076, 1.000000000000000000, 0.8660254037844387076, 1.000000000000000000, 0.8660254037844387076, 1.000000000000000000, 0.8660254037844387076, 1.000000000000000000, 0.8660254037844387076, 1.000000000000000000, 0.8660254037844387076, 1.000000000000000000, 0.8660254037844387076, 1.000000000000000000, 0.8660254037844387076, 1.000000000000000000, 0.8660254037844387076, 1.000000000000000000, 0.8660254037844387076, 1.000000000000000000, 0.8660254037844387076, 1.000000000000000000, 0.8660254037844387076, 1.000000000000000000, 0.8660254037844387076, 1.000000000000000000, 0.8660254037844387076, 1.000000000000000000, 0.8660254037844387076, 1.000000000000000000, 0.8660254037844387076, 1.000000000000000000, 0.8660254037844387076, 1.000000000000000000, 0.8660254037844387076, 1.000000000000000000, 0.8660254037844387076, 1.000000000000000000, 0.8660254037844387076, 1.000000000000000000, 0.8660254037844387076, 1.000000000000000000, 0.8660254037844387076, 1.000000000000000000, 0.8660254037844387076, 1.000000000000000000, 0.8660254037844387076, 1.000000000000000000, 0.8660254037844387076, 1.000000000000000000, 0.8660254037844387076, 1.000000000000000000, 0.8660254037844387076, 1.000000000000000000, 0.8660254037844387076, 1.000000000000000000, 0.8660254037844387076, 1.000000000000000000, 0.8660254037844387076, 1.000000000000000000, 0.8660254037844387076, 1.000000000000000000, 0.8660254037844387076, 1.000000000000000000, 0.8660254037844387076, 1.000000000000000000, 0.8660254037844387076, 1.000000000000000000, 0.8660254037844387076, 1.000000000000000000, 0.8660254037844387076, 1.000000000000000000, 0.8660254037844387076, 1.000000000000000000, 0.8660254037844387076, 1.000000000000000000, 0.8660254037844387076, 1.000000000000000000, 0.8660254037844387076, 1.000000000000000000, 0.8660254037844387076, 1.000000000000000000, 0.8660254037844387076, 1.000000000000000000, 0.8660254037844387076, 1.000000000000000000, 0.8660254037844387076, 1.000000000000000000, 0.8660254037844387076, 1.000000000000000000, 0.8660254037844387076, 1.000000000000000000, 0.8660254037844387076, 1.000000000000000000, 0.8660254037844387076, 1.000000000000000000, 0.8660254037844387076, 1.000000000000000000, 0.8660254037844387076, 1.000000000000000000, 0.8660254037844387076, 1.000000000000000000, 0.8660254037844387076, 1.000000000000000000, 0.8660254037844387076, 1.000000000000000000, 0.8660254037844387076, 1.000000000000000000, 0.9024577157650887083, 0.9469497795711399046, 0.9469497795711399046, 0.9469497795711399046),
 ( 1.000000000000000000, 0.8660254037844387076, 1.000000000000000000, 0.8660254037844387076, 1.000000000000000000, 0.8660254037844387076, 1.000000000000000000, 0.8660254037844387076, 1.000000000000000000, 0.8660254037844387076, 1.000000000000000000, 0.8660254037844387076, 1.000000000000000000, 0.8660254037844387076, 1.000000000000000000, 0.8660254037844387076, 1.000000000000000000, 0.8660254037844387076, 1.000000000000000000, 0.8660254037844387076, 1.000000000000000000, 0.8660254037844387076, 1.000000000000000000, 0.8660254037844387076, 1.000000000000000000, 0.8660254037844387076, 1.000000000000000000, 0.8660254037844387076, 1.000000000000000000, 0.8660254037844387076, 1.000000000000000000, 0.8660254037844387076, 1.000000000000000000, 0.8660254037844387076, 1.000000000000000000, 0.8660254037844387076, 1.000000000000000000, 0.8660254037844387076, 1.000000000000000000, 0.8660254037844387076, 1.000000000000000000, 0.8660254037844387076, 1.000000000000000000, 0.8660254037844387076, 1.000000000000000000, 0.8660254037844387076, 1.000000000000000000, 0.8660254037844387076, 1.000000000000000000, 0.8660254037844387076, 1.000000000000000000, 0.8660254037844387076, 1.000000000000000000, 0.8660254037844387076, 1.000000000000000000, 0.8660254037844387076, 1.000000000000000000, 0.8660254037844387076, 1.000000000000000000, 0.8660254037844387076, 1.000000000000000000, 0.8660254037844387076, 1.000000000000000000, 0.8660254037844387076, 1.000000000000000000, 0.8660254037844387076, 1.000000000000000000, 0.8660254037844387076, 1.000000000000000000, 0.8660254037844387076, 1.000000000000000000, 0.8660254037844387076, 1.000000000000000000, 0.8660254037844387076, 1.000000000000000000, 0.8660254037844387076, 1.000000000000000000, 0.8660254037844387076, 1.000000000000000000, 0.8660254037844387076, 1.000000000000000000, 0.8660254037844387076, 1.000000000000000000, 0.8660254037844387076, 1.000000000000000000, 0.8660254037844387076, 1.000000000000000000, 0.8660254037844387076, 1.000000000000000000, 0.8660254037844387076, 1.000000000000000000, 0.8660254037844387076, 1.000000000000000000, 0.8660254037844387076, 1.000000000000000000, 0.8660254037844387076, 1.000000000000000000, 0.8660254037844387076, 1.000000000000000000, 0.8660254037844387076, 1.000000000000000000, 0.8660254037844387076, 1.000000000000000000, 0.8660254037844387076, 1.000000000000000000, 0.8660254037844387076, 1.000000000000000000, 0.8660254037844387076, 1.000000000000000000, 0.8660254037844387076, 1.000000000000000000, 0.8660254037844387076, 1.000000000000000000, 0.8660254037844387076, 1.000000000000000000, 0.8660254037844387076, 1.000000000000000000, 0.8660254037844387076, 1.000000000000000000, 0.8660254037844387076, 1.000000000000000000, 0.8660254037844387076, 1.000000000000000000, 0.8660254037844387076, 1.000000000000000000, 0.8660254037844387076, 1.000000000000000000, 0.8660254037844387076, 1.000000000000000000, 0.8660254037844387076, 1.000000000000000000, 0.8660254037844387076, 1.000000000000000000, 0.8660254037844387076, 1.000000000000000000, 0.8660254037844387076, 1.000000000000000000, 0.8660254037844387076, 1.000000000000000000, 0.8660254037844387076, 1.000000000000000000, 0.8660254037844387076, 1.000000000000000000, 0.8660254037844387076, 1.000000000000000000, 0.8660254037844387076, 1.000000000000000000, 0.8660254037844387076, 1.000000000000000000, 0.8660254037844387076, 1.000000000000000000, 0.8660254037844387076, 1.000000000000000000, 0.8660254037844387076, 1.000000000000000000, 0.8660254037844387076, 1.000000000000000000, 0.8660254037844387076, 1.000000000000000000, 0.8660254037844387076, 1.000000000000000000, 0.8660254037844387076, 1.000000000000000000, 0.8660254037844387076, 1.000000000000000000, 0.8660254037844387076, 1.000000000000000000, 0.8660254037844387076, 1.000000000000000000, 0.8660254037844387076, 1.000000000000000000, 0.8660254037844387076, 1.000000000000000000, 0.8660254037844387076, 1.000000000000000000, 0.8660254037844387076, 1.000000000000000000, 0.8660254037844387076, 1.000000000000000000, 0.8660254037844387076, 1.000000000000000000, 0.8660254037844387076, 1.000000000000000000, 0.8660254037844387076, 1.000000000000000000, 0.8660254037844387076, 1.000000000000000000, 0.8660254037844387076, 1.000000000000000000, 0.8660254037844387076, 1.000000000000000000, 0.8660254037844387076, 1.000000000000000000, 0.8660254037844387076, 1.000000000000000000, 0.8660254037844387076, 1.000000000000000000, 0.8660254037844387076, 1.000000000000000000, 0.8660254037844387076, 1.000000000000000000, 0.8660254037844387076, 1.000000000000000000, 0.8660254037844387076, 1.000000000000000000, 0.8660254037844387076, 1.000000000000000000, 0.8660254037844387076, 1.000000000000000000, 0.8660254037844387076, 1.000000000000000000, 0.8660254037844387076, 1.000000000000000000, 0.8660254037844387076, 1.000000000000000000, 0.8660254037844387076, 1.000000000000000000, 0.8660254037844387076, 1.000000000000000000, 0.8660254037844387076, 1.000000000000000000, 0.8660254037844387076, 1.000000000000000000, 0.8660254037844387076, 1.000000000000000000, 0.8660254037844387076, 1.000000000000000000, 0.8660254037844387076, 1.000000000000000000, 0.8660254037844387076, 1.000000000000000000, 0.8660254037844387076, 1.000000000000000000, 0.8660254037844387076, 1.000000000000000000, 0.8660254037844387076, 1.000000000000000000, 0.8660254037844387076, 1.000000000000000000, 0.8660254037844387076, 1.000000000000000000, 0.8660254037844387076, 1.000000000000000000, 0.8660254037844387076, 1.000000000000000000, 0.8660254037844387076, 1.000000000000000000, 0.8660254037844387076, 1.000000000000000000, 0.8660254037844387076, 1.000000000000000000, 0.8660254037844387076, 1.000000000000000000, 0.8660254037844387076, 1.000000000000000000, 0.8660254037844387076, 1.000000000000000000, 0.8660254037844387076, 1.000000000000000000, 0.8660254037844387076, 1.000000000000000000, 0.8660254037844387076, 1.000000000000000000, 0.8660254037844387076, 1.000000000000000000, 0.8660254037844387076, 1.000000000000000000, 0.8660254037844387076, 1.000000000000000000, 0.8660254037844387076, 1.000000000000000000, 0.8660254037844387076, 1.000000000000000000, 0.8660254037844387076, 1.000000000000000000, 0.8660254037844387076, 1.000000000000000000, 0.8660254037844387076, 1.000000000000000000, 0.8660254037844387076, 1.000000000000000000, 0.8660254037844387076, 1.000000000000000000, 0.9024577157650887083, 0.9469497795711399046, 0.9469497795711399046, 0.9469497795711399046) ) ) 
 REPRESENTATION_ITEM ( '' )  SURFACE ( )  );
#47246=CARTESIAN_POINT ( 'NONE',  ( 96.32499999999997442, 92.29496732002878900, 82.80333333333332746 ) ) ;
#47250=CARTESIAN_POINT ( 'NONE',  ( 95.00000000000000000, -213.0599564267049857, 86.34874999999999545 ) ) ;
#47261=CARTESIAN_POINT ( 'NONE',  ( -97.30629616937501680, 90.00000000000004263, 87.89656250086714806 ) ) ;
#47265=CARTESIAN_POINT ( 'NONE',  ( 92.69370383062501162, -209.9999999999999716, 88.37281250086715545 ) ) ;
#47266=CARTESIAN_POINT ( 'NONE',  ( 96.32499999999998863, 87.70503267997126784, 78.78166666666666629 ) ) ;
#47267=EDGE_CURVE ( 'NONE', #13854, #66356, #64298, .T. ) ;
#47273=CARTESIAN_POINT ( 'NONE',  ( -97.65000000000001990, 91.52997821335253548, 86.85145833506763324 ) ) ;
#47274=CARTESIAN_POINT ( 'NONE',  ( 97.30629616937498838, 91.33154071421968467, 88.90197916753382401 ) ) ;
#47280=DIRECTION ( 'NONE',  ( -0.000000000000000000, -0.000000000000000000, 1.000000000000000000 ) ) ;
#47281=CARTESIAN_POINT ( 'NONE',  ( -92.34999999999999432, -208.4700217866474645, 86.00479166840096923 ) ) ;
#47285=ORIENTED_EDGE ( 'NONE', *, *, #35315, .F. ) ;
#47286=ORIENTED_EDGE ( 'NONE', *, *, #41239, .F. ) ;
#47292=CARTESIAN_POINT ( 'NONE',  ( -96.15314808468747287, -208.0026889286704943, 86.52072916753382970 ) ) ;
#47302=CARTESIAN_POINT ( 'NONE',  ( 97.30629616937498838, 90.00000000000002842, 81.70531250086713726 ) ) ;
#47305=CARTESIAN_POINT ( 'NONE',  ( -92.35000000000000853, 91.52997821335252127, 85.29041666666665833 ) ) ;
#47307=CARTESIAN_POINT ( 'NONE',  ( 92.35000000000000853, -209.9999999999999716, 80.47499999999999432 ) ) ;
#47310=CARTESIAN_POINT ( 'NONE',  ( 97.64999999999999147, 90.00000000000002842, 83.96750000000000114 ) ) ;
#47311=EDGE_CURVE ( 'NONE', #67765, #55839, #32300, .T. ) ;
#47318=CARTESIAN_POINT ( 'NONE',  ( -93.84685191531254134, 91.99731107132950569, 84.98614583420047097 ) ) ;
#47321=ORIENTED_EDGE ( 'NONE', *, *, #69027, .F. ) ;
#47323=DIRECTION ( 'NONE',  ( -0.000000000000000000, -0.000000000000000000, 1.000000000000000000 ) ) ;
#47324=DIRECTION ( 'NONE',  ( 0.000000000000000000, 0.000000000000000000, 1.000000000000000000 ) ) ;
#47326=CARTESIAN_POINT ( 'NONE',  ( 93.84685191531249870, -208.0026889286704943, 82.71072916753381321 ) ) ;
#47333=CARTESIAN_POINT ( 'NONE',  ( 95.00000000000000000, -212.6630814284392557, 75.19656250086714522 ) ) ;
#47335=CARTESIAN_POINT ( 'NONE',  ( 97.30629616937498838, -211.3315407142195852, 78.00114583420049996 ) ) ;
#47339=ORIENTED_EDGE ( 'NONE', *, *, #33427, .T. ) ;
#47340=CARTESIAN_POINT ( 'NONE',  ( 95.00000000000000000, -206.9400435732949575, 86.74562500173429669 ) ) ;
#47342=( NAMED_UNIT ( * ) PLANE_ANGLE_UNIT ( ) SI_UNIT ( $, .RADIAN. ) );
#47347=CARTESIAN_POINT ( 'NONE',  ( 95.00000000000000000, -213.0599564267049857, 81.98312500173430806 ) ) ;
#47348=CARTESIAN_POINT ( 'NONE',  ( 97.30629616937497417, 89.06968786819601291, 74.84209103131392737 ) ) ;
#47350=VERTEX_POINT ( 'NONE', #45356 ) ;
#47357=CARTESIAN_POINT ( 'NONE',  ( 93.67499999999998295, 92.29496732002878900, 86.79854166840097207 ) ) ;
#47363=CARTESIAN_POINT ( 'NONE',  ( 92.34999999999995168, -211.5299782133524502, 77.98791666666667766 ) ) ;
#47365=CARTESIAN_POINT ( 'NONE',  ( -92.35000000000678710, 90.00000598221780024, 82.14187520865721126 ) ) ;
#47366=VERTEX_POINT ( 'NONE', #56638 ) ;
#47369=CARTESIAN_POINT ( 'NONE',  ( 97.64999999999999147, -209.9999999999999716, 80.15749999999999886 ) ) ;
#47371=CARTESIAN_POINT ( 'NONE',  ( -97.65000000000001990, 88.47002178664754979, 88.78291666666667936 ) ) ;
#47377=CARTESIAN_POINT ( 'NONE',  ( 94.99999999999998579, 90.00000000000002842, 90.00000000000000000 ) ) ;
#47378=CARTESIAN_POINT ( 'NONE',  ( -93.84685191531247028, -211.9973110713294489, 82.86947916753379673 ) ) ;
#47385=AXIS2_PLACEMENT_3D ( 'NONE', #40903, #47280, #65316 ) ;
#47391=CARTESIAN_POINT ( 'NONE',  ( 92.34999999999999432, 90.00000000000002842, 79.91937500173429498 ) ) ;
#47394=CARTESIAN_POINT ( 'NONE',  ( -96.15314808468751551, 88.00268892867056536, 79.58864583420047722 ) ) ;
#47395=DIRECTION ( 'NONE',  ( 1.000000000000000000, 0.000000000000000000, 0.000000000000000000 ) ) ;
#47399=CARTESIAN_POINT ( 'NONE',  ( -97.64999999980585699, -210.0000198431789897, 84.36502761000342332 ) ) ;
#47402=CARTESIAN_POINT ( 'NONE',  ( 96.37670920697046029, 87.70919997534038259, 75.00000000000000000 ) ) ;
#47404=DIRECTION ( 'NONE',  ( 1.000000000000000000, 0.000000000000000000, 0.000000000000000000 ) ) ;
#47405=CARTESIAN_POINT ( 'NONE',  ( -97.30629616937495996, -209.9999999999999716, 75.19656250086714522 ) ) ;
#47407=ORIENTED_EDGE ( 'NONE', *, *, #21888, .T. ) ;
#47414=CARTESIAN_POINT ( 'NONE',  ( -97.64999999950704535, 89.99996796756893502, 85.63541623677065218 ) ) ;
#47420=CARTESIAN_POINT ( 'NONE',  ( 95.00000000000000000, -212.6630814284392557, 86.62656250086713783 ) ) ;
#47421=CARTESIAN_POINT ( 'NONE',  ( 96.15314808468750130, -211.9973110713294489, 87.47322916753381605 ) ) ;
#47426=VERTEX_POINT ( 'NONE', #28406 ) ;
#47428=ORIENTED_EDGE ( 'NONE', *, *, #4015, .F. ) ;
#47429=CARTESIAN_POINT ( 'NONE',  ( -95.00000000000002842, 87.33691857156074434, 82.34031250086714238 ) ) ;
#47433=ORIENTED_EDGE ( 'NONE', *, *, #59319, .F. ) ;
#47434=CARTESIAN_POINT ( 'NONE',  ( -92.34999999999999432, -211.5299782133524218, 87.80395833506766223 ) ) ;
#47442=CARTESIAN_POINT ( 'NONE',  ( 92.79788703567041352, 88.68334238502474420, 74.94590613650809985 ) ) ;
#47445=EDGE_LOOP ( 'NONE', ( #68465, #55678, #58647, #3013 ) ) ;
#47447=CARTESIAN_POINT ( 'NONE',  ( 96.15314808468748708, -208.0026889286704943, 80.54114583420046358 ) ) ;
#47453=FACE_OUTER_BOUND ( 'NONE', #33745, .T. ) ;
#47456=CARTESIAN_POINT ( 'NONE',  ( -93.84685191531248449, -208.0026889286704943, 83.08114583420048405 ) ) ;
#47457=CARTESIAN_POINT ( 'NONE',  ( -95.00000000000002842, 92.66308142843932671, 82.65781250086715204 ) ) ;
#47460=CARTESIAN_POINT ( 'NONE',  ( 92.69370383062498320, 91.33154071421968467, 79.42989583420046529 ) ) ;
#47465=CARTESIAN_POINT ( 'NONE',  ( -92.34999999999999432, -209.9999999999999716, 83.41187500173430180 ) ) ;
#47466=EDGE_CURVE ( 'NONE', #67844, #65764, #52446, .T. ) ;
#47469=CARTESIAN_POINT ( 'NONE',  ( -92.69370383062498320, -208.6684592857803295, 83.02822916753379445 ) ) ;
#47473=EDGE_CURVE ( 'NONE', #32411, #49261, #45745, .T. ) ;
#47475=CARTESIAN_POINT ( 'NONE',  ( 94.99999999999998579, 90.00000000000002842, 90.00000000000000000 ) ) ;
#47481=CARTESIAN_POINT ( 'NONE',  ( -92.69370383062504004, 90.00000000000004263, 88.05531250086713158 ) ) ;
#47486=( BOUNDED_CURVE ( )  B_SPLINE_CURVE ( 2, ( #51407, #56325, #51044, #44296, #68723, #50666, #10831 ),
 .UNSPECIFIED., .F., .F. ) 
 B_SPLINE_CURVE_WITH_KNOTS ( ( 3, 2, 2, 3 ),
 ( 0.1458333333333334536, 0.1527777777777778734, 0.1597222222222222654, 0.1666666666666666852 ),
 .UNSPECIFIED. ) 
 CURVE ( )  GEOMETRIC_REPRESENTATION_ITEM ( )  RATIONAL_B_SPLINE_CURVE ( ( 0.9999999999999978906, 0.8660254037844408170, 1.000000000000000000, 0.8660254037844387076, 1.000000000000000000, 0.8660254037844381525, 1.000000000000000444 ) ) 
 REPRESENTATION_ITEM ( '' )  );
#47496=CARTESIAN_POINT ( 'NONE',  ( -93.84685191531247028, -211.9973110713294489, 86.20322916753382003 ) ) ;
#47500=CARTESIAN_POINT ( 'NONE',  ( -93.84685191531247028, -211.9973110713294489, 77.31322916753381946 ) ) ;
#47502=VERTEX_POINT ( 'NONE', #63758 ) ;
#47503=CARTESIAN_POINT ( 'NONE',  ( -2.499999999999965361, 90.00000000000000000, -90.00000000000000000 ) ) ;
#47505=CARTESIAN_POINT ( 'NONE',  ( -97.64999247309856401, 88.47001744098896836, 88.22729196900364457 ) ) ;
#47506=FACE_OUTER_BOUND ( 'NONE', #36786, .T. ) ;
#47507=CARTESIAN_POINT ( 'NONE',  ( 92.69370383062501162, -208.6684592857803011, 78.15989583420048348 ) ) ;
#47514=VERTEX_POINT ( 'NONE', #18606 ) ;
#47518=ORIENTED_EDGE ( 'NONE', *, *, #15255, .T. ) ;
#47529=CARTESIAN_POINT ( 'NONE',  ( 92.69370383062498320, 88.66845928578037217, 78.42447916753380355 ) ) ;
#47530=LINE ( 'NONE', #18212, #26386 ) ;
#47531=CARTESIAN_POINT ( 'NONE',  ( 96.32499999999998863, -207.7050326799711968, 75.81833333333332803 ) ) ;
#47544=FACE_OUTER_BOUND ( 'NONE', #71480, .T. ) ;
#47546=CARTESIAN_POINT ( 'NONE',  ( 97.65000000000004832, 91.52997821335250705, 77.67041666666666799 ) ) ;
#47547=CARTESIAN_POINT ( 'NONE',  ( -93.67499999999998295, -212.2949673200287179, 78.22604166840096696 ) ) ;
#47549=CARTESIAN_POINT ( 'NONE',  ( 92.34999999999999432, 90.00000000000002842, 74.83937500173429669 ) ) ;
#47550=CARTESIAN_POINT ( 'NONE',  ( -93.67500000000003979, 92.29496732002878900, 75.89770833506763381 ) ) ;
#47551=EDGE_LOOP ( 'NONE', ( #45613, #36002, #47079, #36419 ) ) ;
#47552=CARTESIAN_POINT ( 'NONE',  ( 97.30629616937498838, 91.33154071421968467, 77.47197916753381719 ) ) ;
#47556=CARTESIAN_POINT ( 'NONE',  ( -92.35000000000003695, 89.99999989488615881, 86.58687499784845443 ) ) ;
#47562=CARTESIAN_POINT ( 'NONE',  ( 97.64999999999997726, 90.00000000000002842, 90.00000000000000000 ) ) ;
#47565=CARTESIAN_POINT ( 'NONE',  ( -93.07557990970624928, -211.8218417373838065, 75.00000000000000000 ) ) ;
#47569=CARTESIAN_POINT ( 'NONE',  ( -94.99999999999997158, -207.3369185715606307, 76.94281250086714863 ) ) ;
#47579=CYLINDRICAL_SURFACE ( 'NONE', #20569, 2.649999999999985700 ) ;
#47580=CARTESIAN_POINT ( 'NONE',  ( 92.34999999999999432, 91.52997821335252127, 86.21645833506764234 ) ) ;
#47584=CARTESIAN_POINT ( 'NONE',  ( 96.15314808468748708, 88.00268892867053694, 82.39322916753381776 ) ) ;
#47585=CARTESIAN_POINT ( 'NONE',  ( -97.30629616937495996, -209.9999999999999716, 86.62656250086715204 ) ) ;
#47587=ORIENTED_EDGE ( 'NONE', *, *, #73727, .F. ) ;
#47588=CARTESIAN_POINT ( 'NONE',  ( 97.65000000000000568, -211.5299782133524218, 83.35895833506764063 ) ) ;
#47589=CARTESIAN_POINT ( 'NONE',  ( -92.34999999999999432, -209.9999999999999716, 80.79249999999998977 ) ) ;
#47590=CARTESIAN_POINT ( 'NONE',  ( -93.84685191531252713, 88.00268892867056536, 75.88447916753381151 ) ) ;
#47591=AXIS2_PLACEMENT_3D ( 'NONE', #8202, #9314, #54444 ) ;
#47592=CARTESIAN_POINT ( 'NONE',  ( 93.84685191531251292, -211.9973110713294489, 86.57364583420047666 ) ) ;
#47596=EDGE_CURVE ( 'NONE', #3278, #1800, #17386, .T. ) ;
#47597=CARTESIAN_POINT ( 'NONE',  ( 96.32499999999998863, -212.2949673200287179, 75.60666666666665492 ) ) ;
#47604=CARTESIAN_POINT ( 'NONE',  ( 96.15314808468748708, -208.0026889286704943, 81.33489583420049485 ) ) ;
#47605=CARTESIAN_POINT ( 'NONE',  ( -97.64999999999996305, -209.9999999999999716, 81.10999999999999943 ) ) ;
#47606=CARTESIAN_POINT ( 'NONE',  ( 92.34999999999988063, 91.52997821335246442, 81.05708333333332405 ) ) ;
#47609=EDGE_CURVE ( 'NONE', #55850, #38100, #4904, .T. ) ;
#47612=CARTESIAN_POINT ( 'NONE',  ( 93.67500000000001137, -207.7050326799711968, 85.44916666666665606 ) ) ;
#47614=ORIENTED_EDGE ( 'NONE', *, *, #12632, .F. ) ;
#47618=CARTESIAN_POINT ( 'NONE',  ( -97.64999999999996305, -209.9999999999999716, 90.00000000000000000 ) ) ;
#47620=CARTESIAN_POINT ( 'NONE',  ( -95.00000000000002842, 87.33691857156074434, 88.69031250086716511 ) ) ;
#47624=CARTESIAN_POINT ( 'NONE',  ( 95.00000000000000000, -212.6630814284392557, 87.26156250086714294 ) ) ;
#47625=FACE_OUTER_BOUND ( 'NONE', #3817, .T. ) ;
#47627=ORIENTED_EDGE ( 'NONE', *, *, #13717, .F. ) ;
#47634=CARTESIAN_POINT ( 'NONE',  ( -93.67500000000003979, 87.70503267997129626, 86.48104166840096241 ) ) ;
#47635=CARTESIAN_POINT ( 'NONE',  ( 96.15314808468748708, 88.00268892867053694, 89.37822916753381719 ) ) ;
#47645=CARTESIAN_POINT ( 'NONE',  ( -94.99999999999997158, -212.6630814284392557, 75.83156250086715033 ) ) ;
#47646=ORIENTED_EDGE ( 'NONE', *, *, #28367, .F. ) ;
#47653=CARTESIAN_POINT ( 'NONE',  ( -97.30629616937497417, -211.3315407142195852, 86.67947916753382742 ) ) ;
#47655=CARTESIAN_POINT ( 'NONE',  ( -96.32499999999996021, -212.2949673200287179, 82.48583333333333201 ) ) ;
#47658=CARTESIAN_POINT ( 'NONE',  ( 97.64999999999999147, 89.99999997442942856, 84.04687500080852658 ) ) ;
#47660=CARTESIAN_POINT ( 'NONE',  ( 94.99999999999998579, 92.66308142843932671, 79.95906250086713385 ) ) ;
#47663=CARTESIAN_POINT ( 'NONE',  ( -95.00000000000002842, 93.05995642670504253, 80.95125000000000171 ) ) ;
#47669=CARTESIAN_POINT ( 'NONE',  ( 92.35000000000000853, -210.0000359324574788, 85.63437624451400154 ) ) ;
#47672=ORIENTED_EDGE ( 'NONE', *, *, #23285, .T. ) ;
#47673=CARTESIAN_POINT ( 'NONE',  ( -97.30629616937501680, 90.00000000000004263, 85.83281250086714920 ) ) ;
#47681=( BOUNDED_CURVE ( )  B_SPLINE_CURVE ( 2, ( #55716, #56475, #67743, #54971, #4232, #27509, #21121, #50443, #49687, #73365, #4980 ),
 .UNSPECIFIED., .F., .F. ) 
 B_SPLINE_CURVE_WITH_KNOTS ( ( 3, 2, 2, 2, 2, 3 ),
 ( 0.04233441017594471306, 0.04233459324529428858, 0.04939035878617635544, 0.05644612432705840843, 0.06350188986794047530, 0.06350193517735297499 ),
 .UNSPECIFIED. ) 
 CURVE ( )  GEOMETRIC_REPRESENTATION_ITEM ( )  RATIONAL_B_SPLINE_CURVE ( ( 0.9999930479532868066, 0.9999965238864518824, 1.000000000000000000, 0.8660254037844387076, 1.000000000000000000, 0.8660254037844387076, 1.000000000000000000, 0.8660254037844387076, 1.000000000000000000, 0.9999991396666727539, 0.9999982793443948914 ) ) 
 REPRESENTATION_ITEM ( '' )  );
#47687=CARTESIAN_POINT ( 'NONE',  ( 92.69370383062501162, -211.3315407142195852, 80.96447916753382401 ) ) ;
#47695=CARTESIAN_POINT ( 'NONE',  ( 95.00000000000000000, -207.3369185715606307, 76.14906250086716000 ) ) ;
#47698=CARTESIAN_POINT ( 'NONE',  ( 92.69370383062501162, -211.3315407142195852, 80.96447916753382401 ) ) ;
#47707=CARTESIAN_POINT ( 'NONE',  ( 95.00000000000000000, -213.0599564267049857, 82.61812500173428475 ) ) ;
#47708=CARTESIAN_POINT ( 'NONE',  ( 94.99999999999998579, 93.05995642670504253, 87.93625000000000114 ) ) ;
#47713=LINE ( 'NONE', #31524, #24890 ) ;
#47716=CARTESIAN_POINT ( 'NONE',  ( -93.84685191531254134, 91.99731107132950569, 88.95489583420049939 ) ) ;
#47717=CARTESIAN_POINT ( 'NONE',  ( 92.69370383062498320, 90.00000000000002842, 85.83281250086714920 ) ) ;
#47720=CARTESIAN_POINT ( 'NONE',  ( 96.32499999999997442, 92.29496732002878900, 85.42270833506762528 ) ) ;
#47731=CARTESIAN_POINT ( 'NONE',  ( -95.00000000000002842, 86.94004357329504273, 84.44375000000000853 ) ) ;
#47733=CARTESIAN_POINT ( 'NONE',  ( 92.35000000000000853, 88.47002178664752137, 81.79791666666665151 ) ) ;
#47735=EDGE_LOOP ( 'NONE', ( #71470, #50981 ) ) ;
#47737=CARTESIAN_POINT ( 'NONE',  ( -92.69370383062498320, -208.6684592857803011, 83.02822916753379445 ) ) ;
#47747=CARTESIAN_POINT ( 'NONE',  ( 96.66135172262730180, -211.6008015735635865, 74.79754476654878204 ) ) ;
#47748=CARTESIAN_POINT ( 'NONE',  ( 92.35000000046503033, 89.99996900126896548, 83.09538598081184091 ) ) ;
#47749=DIRECTION ( 'NONE',  ( 0.000000000000000000, -0.000000000000000000, -1.000000000000000000 ) ) ;
#47751=CARTESIAN_POINT ( 'NONE',  ( -95.00000000000002842, 87.33691857156074434, 75.83156250086715033 ) ) ;
#47761=CARTESIAN_POINT ( 'NONE',  ( -96.32499999999996021, -207.7050326799711968, 87.98916666666666231 ) ) ;
#47765=VERTEX_POINT ( 'NONE', #27193 ) ;
#47771=EDGE_CURVE ( 'NONE', #45794, #52132, #72682, .T. ) ;
#47781=CARTESIAN_POINT ( 'NONE',  ( 97.30629616937498838, -211.3315407142195852, 85.46239583420044994 ) ) ;
#47782=CARTESIAN_POINT ( 'NONE',  ( 96.15314808468748708, -208.0026889286704943, 89.58989583420049030 ) ) ;
#47785=CARTESIAN_POINT ( 'NONE',  ( 93.84685191531249870, -208.0026889286704943, 88.42572916753381662 ) ) ;
#47789=CARTESIAN_POINT ( 'NONE',  ( -97.30629616937501680, 91.33154071421968467, 80.22364583420048234 ) ) ;
#47790=VECTOR ( 'NONE', #8122, 1000.000000000000000 ) ;
#47796=ORIENTED_EDGE ( 'NONE', *, *, #53048, .F. ) ;
#47799=AXIS2_PLACEMENT_3D ( 'NONE', #60179, #62300, #9018 ) ;
#47805=CARTESIAN_POINT ( 'NONE',  ( 97.64999999999449187, -210.0000054026048701, 81.50687481489494246 ) ) ;
#47810=CARTESIAN_POINT ( 'NONE',  ( 97.30629616937498838, -209.9999999999999716, 78.53031250086714010 ) ) ;
#47811=CARTESIAN_POINT ( 'NONE',  ( -96.32500000000001705, 92.29496732002878900, 83.54416666666666913 ) ) ;
#47814=CARTESIAN_POINT ( 'NONE',  ( -93.67499999999998295, -212.2949673200287179, 78.86104166840097207 ) ) ;
#47819=CARTESIAN_POINT ( 'NONE',  ( -97.30629616937497417, -211.3315407142195852, 80.17072916753379275 ) ) ;
#47820=CARTESIAN_POINT ( 'NONE',  ( -92.69370383062504004, 90.00000000000004263, 79.95906250086714806 ) ) ;
#47822=CARTESIAN_POINT ( 'NONE',  ( 94.99999999999998579, 92.66308142843935514, 81.86406250086714920 ) ) ;
#47829=CARTESIAN_POINT ( 'NONE',  ( -93.84685191531248449, -208.0026889286704943, 81.81114583420047381 ) ) ;
#47831=VECTOR ( 'NONE', #66367, 1000.000000000000000 ) ;
#47835=ORIENTED_EDGE ( 'NONE', *, *, #69928, .T. ) ;
#47841=CARTESIAN_POINT ( 'NONE',  ( -93.84685191531252713, 88.00268892867056536, 84.13947916753380696 ) ) ;
#47847=CARTESIAN_POINT ( 'NONE',  ( -95.00000000000002842, 92.66308142843932671, 75.51406250086714067 ) ) ;
#47853=CARTESIAN_POINT ( 'NONE',  ( -92.69370383062498320, -211.3315407142195852, 87.52614583420049144 ) ) ;
#47862=CARTESIAN_POINT ( 'NONE',  ( -96.15314808468747287, -208.0026889286704943, 77.63072916753381492 ) ) ;
#47863=CARTESIAN_POINT ( 'NONE',  ( 96.32499999999997442, 92.29496732002878900, 88.51833333333333087 ) ) ;
#47866=CYLINDRICAL_SURFACE ( 'NONE', #66568, 2.649999999999985700 ) ;
#47870=CARTESIAN_POINT ( 'NONE',  ( 92.69370383062501162, -211.3315407142195852, 87.31447916753381833 ) ) ;
#47877=DIRECTION ( 'NONE',  ( -1.000000000000000000, 3.061616997868382648E-16, 0.000000000000000000 ) ) ;
#47892=ORIENTED_EDGE ( 'NONE', *, *, #15688, .F. ) ;
#47893=CARTESIAN_POINT ( 'NONE',  ( 97.30629616937498838, 90.00000000000002842, 79.32406250086715715 ) ) ;
#47894=CARTESIAN_POINT ( 'NONE',  ( -97.65000000000001990, 88.47002178664754979, 81.24229166840096639 ) ) ;
#47906=CARTESIAN_POINT ( 'NONE',  ( -97.45337789172094745, 90.48452257634338025, 74.90854212414870972 ) ) ;
#47913=CARTESIAN_POINT ( 'NONE',  ( -97.64999999999996305, -209.9999999999999716, 79.91937500173429498 ) ) ;
#47915=CARTESIAN_POINT ( 'NONE',  ( 97.64999999999997726, 91.52997821335252127, 77.11479166840095445 ) ) ;
#47916=CARTESIAN_POINT ( 'NONE',  ( -92.35000000000005116, 88.47002178664754979, 77.64395833506762301 ) ) ;
#47918=( BOUNDED_CURVE ( )  B_SPLINE_CURVE ( 2, ( #1299, #24188, #6169, #6524, #46011, #7265, #40359 ),
 .UNSPECIFIED., .F., .F. ) 
 B_SPLINE_CURVE_WITH_KNOTS ( ( 3, 2, 2, 3 ),
 ( 0.8749999999999997780, 0.8819444444444441977, 0.8888888888888886175, 0.8958333333333331483 ),
 .UNSPECIFIED. ) 
 CURVE ( )  GEOMETRIC_REPRESENTATION_ITEM ( )  RATIONAL_B_SPLINE_CURVE ( ( 1.000000000000004219, 0.8660254037844343777, 1.000000000000000000, 0.8660254037844387076, 1.000000000000000000, 0.8660254037844430375, 0.9999999999999956701 ) ) 
 REPRESENTATION_ITEM ( '' )  );
#47919=ORIENTED_EDGE ( 'NONE', *, *, #25572, .T. ) ;
#47920=CARTESIAN_POINT ( 'NONE',  ( 93.84685191531248449, 91.99731107132950569, 75.09072916753380866 ) ) ;
#47922=DIRECTION ( 'NONE',  ( 1.000000000000000000, 0.000000000000000000, 0.000000000000000000 ) ) ;
#47924=CARTESIAN_POINT ( 'NONE',  ( -97.64999999999996305, -209.9999999999999716, 90.00000000000000000 ) ) ;
#47931=VECTOR ( 'NONE', #4568, 1000.000000000000000 ) ;
#47933=CARTESIAN_POINT ( 'NONE',  ( 92.35000000000000853, -208.4700217866474645, 88.12145833506765769 ) ) ;
#47950=DIRECTION ( 'NONE',  ( -0.000000000000000000, -0.000000000000000000, 1.000000000000000000 ) ) ;
#47953=CARTESIAN_POINT ( 'NONE',  ( -97.64999999999996305, -209.9999907079536854, 84.99937468035446386 ) ) ;
#47955=CARTESIAN_POINT ( 'NONE',  ( -97.64999999999996305, -208.4700217866474645, 77.96145833506763267 ) ) ;
#47956=CARTESIAN_POINT ( 'NONE',  ( -92.34999999999999432, -209.9999999999999716, 90.00000000000000000 ) ) ;
#47958=CARTESIAN_POINT ( 'NONE',  ( 97.30629616937498838, 91.33154071421968467, 83.18697916753382060 ) ) ;
#47959=CARTESIAN_POINT ( 'NONE',  ( -94.99999999999997158, -212.6630814284392557, 87.42031250086715488 ) ) ;
#47960=CARTESIAN_POINT ( 'NONE',  ( 94.99999999999998579, 93.05995642670504253, 79.12562500173429214 ) ) ;
#47963=EDGE_CURVE ( 'NONE', #16250, #51073, #12109, .T. ) ;
#47965=CARTESIAN_POINT ( 'NONE',  ( -97.64999999999996305, -209.9999999999999716, 82.37999999999999545 ) ) ;
#47966=CARTESIAN_POINT ( 'NONE',  ( -97.30629616937501680, 90.00000000000004263, 76.94281250086713442 ) ) ;
#47971=CARTESIAN_POINT ( 'NONE',  ( 96.15314808468750130, -211.9973110713294489, 87.94947916753380923 ) ) ;
#47972=VERTEX_POINT ( 'NONE', #17052 ) ;
#47974=VERTEX_POINT ( 'NONE', #46364 ) ;
#47977=CARTESIAN_POINT ( 'NONE',  ( 96.32499999999998863, -207.7050326799711968, 84.07333333333333769 ) ) ;
#47978=ADVANCED_FACE ( 'NONE', ( #39988 ), #18155, .F. ) ;
#47983=CARTESIAN_POINT ( 'NONE',  ( 95.00000000000000000, -212.6630814284392557, 77.26031250086714408 ) ) ;
#47984=DIRECTION ( 'NONE',  ( -0.000000000000000000, -0.000000000000000000, 1.000000000000000000 ) ) ;
#47985=EDGE_CURVE ( 'NONE', #36972, #44773, #17417, .T. ) ;
#47991=CARTESIAN_POINT ( 'NONE',  ( 96.32499999999998863, -207.7050326799711968, 84.07333333333333769 ) ) ;
#48000=CARTESIAN_POINT ( 'NONE',  ( -96.15314808468752972, 91.99731107132950569, 83.34572916753383254 ) ) ;
#48006=ORIENTED_EDGE ( 'NONE', *, *, #19005, .F. ) ;
#48009=CARTESIAN_POINT ( 'NONE',  ( -97.65000000000001990, 91.52997821335253548, 85.58145833506763722 ) ) ;
#48010=CARTESIAN_POINT ( 'NONE',  ( 97.30629616937498838, 88.66845928578037217, 85.62114583420047609 ) ) ;
#48011=LINE ( 'NONE', #66424, #49030 ) ;
#48023=CARTESIAN_POINT ( 'NONE',  ( 94.99999999999998579, 86.94004357329502852, 78.80812500173429669 ) ) ;
#48027=CARTESIAN_POINT ( 'NONE',  ( -96.15314808468745866, -211.9973110713294489, 88.00239583420048461 ) ) ;
#48035=CARTESIAN_POINT ( 'NONE',  ( 97.30629616937498838, 90.00000000000002842, 81.07031250086714635 ) ) ;
#48037=CARTESIAN_POINT ( 'NONE',  ( -92.35000000000003695, 89.99999990163421160, 80.23687499810812085 ) ) ;
#48046=CARTESIAN_POINT ( 'NONE',  ( 92.35000000000000853, -209.9999999999999716, 90.00000000000000000 ) ) ;
#48050=CARTESIAN_POINT ( 'NONE',  ( -97.30629616937501680, 88.66845928578038638, 87.79072916753379729 ) ) ;
#48064=EDGE_CURVE ( 'NONE', #71124, #29550, #43322, .T. ) ;
#48065=CARTESIAN_POINT ( 'NONE',  ( 95.00000000000000000, -207.3369185715606307, 82.02281250086714692 ) ) ;
#48075=CARTESIAN_POINT ( 'NONE',  ( 96.15314808468750130, -211.9973110713294489, 81.12322916753382174 ) ) ;
#48076=ORIENTED_EDGE ( 'NONE', *, *, #47466, .F. ) ;
#48084=LINE ( 'NONE', #31890, #38980 ) ;
#48085=CARTESIAN_POINT ( 'NONE',  ( 96.32499999999998863, -212.2949673200287179, 83.30604166840096525 ) ) ;
#48086=CARTESIAN_POINT ( 'NONE',  ( 97.64999999999997726, 88.47002178664753558, 83.91458333333333997 ) ) ;
#48092=CARTESIAN_POINT ( 'NONE',  ( -93.84685191531252713, 88.00268892867056536, 87.47322916753381605 ) ) ;
#48093=CARTESIAN_POINT ( 'NONE',  ( 96.15314808468748708, 91.99731107132950569, 82.44614583420046472 ) ) ;
#48095=CARTESIAN_POINT ( 'NONE',  ( 97.64999999999997726, 91.52997821335252127, 85.36979166840096411 ) ) ;
#48096=VECTOR ( 'NONE', #65894, 1000.000000000000000 ) ;
#48098=CARTESIAN_POINT ( 'NONE',  ( 97.64999999954044085, -209.9999506483753180, 87.22187670868780174 ) ) ;
#48103=ORIENTED_EDGE ( 'NONE', *, *, #21831, .F. ) ;
#48106=CARTESIAN_POINT ( 'NONE',  ( -92.35000000000005116, 91.52997821335253548, 83.38541666666667140 ) ) ;
#48108=LINE ( 'NONE', #19158, #7109 ) ;
#48112=CARTESIAN_POINT ( 'NONE',  ( -93.84685191531247028, -211.9973110713294489, 83.50447916753381605 ) ) ;
#48114=DIRECTION ( 'NONE',  ( -0.000000000000000000, -0.000000000000000000, -1.000000000000000000 ) ) ;
#48122=AXIS2_PLACEMENT_3D ( 'NONE', #67995, #62754, #4483 ) ;
#48126=CARTESIAN_POINT ( 'NONE',  ( 97.30629616937497417, -209.9999999999998863, 74.79348190356849102 ) ) ;
#48128=DIRECTION ( 'NONE',  ( -0.000000000000000000, -0.000000000000000000, 1.000000000000000000 ) ) ;
#48131=CARTESIAN_POINT ( 'NONE',  ( -97.30629616937501680, 90.00000000000004263, 89.80156250086714920 ) ) ;
#48133=CARTESIAN_POINT ( 'NONE',  ( 93.67499999999999716, 87.70503267997126784, 76.13583333333333769 ) ) ;
#48134=( BOUNDED_CURVE ( )  B_SPLINE_CURVE ( 2, ( #14178, #48765, #64583, #2210, #19081, #13069, #31472 ),
 .UNSPECIFIED., .F., .F. ) 
 B_SPLINE_CURVE_WITH_KNOTS ( ( 3, 2, 2, 3 ),
 ( 0.2083333333333331483, 0.2152777777777775681, 0.2222222222222219323, 0.2291666666666663521 ),
 .UNSPECIFIED. ) 
 CURVE ( )  GEOMETRIC_REPRESENTATION_ITEM ( )  RATIONAL_B_SPLINE_CURVE ( ( 1.000000000000003775, 0.8660254037844349329, 1.000000000000000000, 0.8660254037844387076, 1.000000000000000000, 0.8660254037844445918, 0.9999999999999941158 ) ) 
 REPRESENTATION_ITEM ( '' )  );
#48144=CARTESIAN_POINT ( 'NONE',  ( -94.99999999999997158, -206.9400435732949575, 89.20624999999999716 ) ) ;
#48158=CARTESIAN_POINT ( 'NONE',  ( -97.65000000000001990, 90.00000000000004263, 90.00000000000000000 ) ) ;
#48160=CARTESIAN_POINT ( 'NONE',  ( 92.69370383062501162, -208.6684592857803295, 81.33489583420048064 ) ) ;
#48161=CARTESIAN_POINT ( 'NONE',  ( 93.84685191531251292, -211.9973110713294489, 87.36739583420049371 ) ) ;
#48162=ORIENTED_EDGE ( 'NONE', *, *, #62213, .F. ) ;
#48163=CARTESIAN_POINT ( 'NONE',  ( 95.00000000000000000, -207.3369185715606307, 89.64281250086715147 ) ) ;
#48169=CARTESIAN_POINT ( 'NONE',  ( -96.15314808468751551, 88.00268892867056536, 77.84239583420048803 ) ) ;
#48171=ORIENTED_EDGE ( 'NONE', *, *, #40825, .F. ) ;
#48178=VERTEX_POINT ( 'NONE', #1650 ) ;
#48184=CARTESIAN_POINT ( 'NONE',  ( 93.84685191531251292, -211.9973110713294489, 79.58864583420047722 ) ) ;
#48187=CARTESIAN_POINT ( 'NONE',  ( -92.35000000000003695, 90.00000000000004263, 82.06250000000000000 ) ) ;
#48189=CARTESIAN_POINT ( 'NONE',  ( -92.34999999999998010, -209.9999733970677482, 78.96687592183791082 ) ) ;
#48190=LINE ( 'NONE', #24885, #41375 ) ;
#48195=CARTESIAN_POINT ( 'NONE',  ( -92.69370383062498320, -209.9999999999999716, 79.80031250086713612 ) ) ;
#48197=CARTESIAN_POINT ( 'NONE',  ( -92.69370383062504004, 90.00000000000004263, 79.32406250086715715 ) ) ;
#48198=ORIENTED_EDGE ( 'NONE', *, *, #29535, .F. ) ;
#48199=CARTESIAN_POINT ( 'NONE',  ( 97.30629616937498838, 90.00000000000002842, 81.70531250086713726 ) ) ;
#48201=CARTESIAN_POINT ( 'NONE',  ( 96.32499999999997442, 92.29496732002878900, 78.43770833506764006 ) ) ;
#48203=CARTESIAN_POINT ( 'NONE',  ( -97.64999999953492704, -210.0000309987302956, 83.09538598079114990 ) ) ;
#48206=CARTESIAN_POINT ( 'NONE',  ( -97.30629616937495996, -209.9999999999999716, 83.29281250086714294 ) ) ;
#48221=CARTESIAN_POINT ( 'NONE',  ( -92.69370383062504004, 90.00000000000004263, 86.15031250086714465 ) ) ;
#48224=CARTESIAN_POINT ( 'NONE',  ( -2.499999999999970690, 73.00000000000001421, -204.9999999999999716 ) ) ;
#48227=CARTESIAN_POINT ( 'NONE',  ( -93.84685191531254134, 91.99731107132950569, 75.46114583420047950 ) ) ;
#48228=VECTOR ( 'NONE', #41013, 1000.000000000000000 ) ;
#48235=CARTESIAN_POINT ( 'NONE',  ( -97.30629616937497417, -208.6684592857803011, 82.76364583420048859 ) ) ;
#48237=EDGE_CURVE ( 'NONE', #30123, #69332, #52959, .T. ) ;
#48240=EDGE_CURVE ( 'NONE', #57167, #25433, #21466, .T. ) ;
#48242=CARTESIAN_POINT ( 'NONE',  ( -97.30629616937497417, -208.6684592857803295, 75.77864583420048916 ) ) ;
#48244=VERTEX_POINT ( 'NONE', #32011 ) ;
#48245=DIRECTION ( 'NONE',  ( -0.000000000000000000, -0.000000000000000000, 1.000000000000000000 ) ) ;
#48246=LINE ( 'NONE', #35478, #69480 ) ;
#48247=CARTESIAN_POINT ( 'NONE',  ( 95.00000000000000000, -206.9400435732949575, 79.68124999999999147 ) ) ;
#48249=CARTESIAN_POINT ( 'NONE',  ( 92.69370383062501162, -208.6684592857803011, 74.98489583420048632 ) ) ;
#48266=CARTESIAN_POINT ( 'NONE',  ( 96.15314808468748708, 88.00268892867053694, 79.85322916753381151 ) ) ;
#48269=VERTEX_POINT ( 'NONE', #62089 ) ;
#48275=ORIENTED_EDGE ( 'NONE', *, *, #41680, .F. ) ;
#48281=CARTESIAN_POINT ( 'NONE',  ( -94.99999999999997158, -206.9400435732949575, 84.20562500173429044 ) ) ;
#48285=CARTESIAN_POINT ( 'NONE',  ( -93.67499999999998295, -207.7050326799711968, 74.62770833506762358 ) ) ;
#48288=CARTESIAN_POINT ( 'NONE',  ( 97.64999999999997726, 91.52997821335252127, 75.20979166840096752 ) ) ;
#48289=CARTESIAN_POINT ( 'NONE',  ( -93.67500000000003979, 87.70503267997129626, 75.05104166840095559 ) ) ;
#48291=CARTESIAN_POINT ( 'NONE',  ( 92.69370383062498320, 91.33154071421968467, 75.77864583420048916 ) ) ;
#48295=CARTESIAN_POINT ( 'NONE',  ( 93.67500000000001137, -212.2949673200287179, 77.48520833506763950 ) ) ;
#48302=VERTEX_POINT ( 'NONE', #73343 ) ;
#48304=CARTESIAN_POINT ( 'NONE',  ( 97.65000000000003411, -208.4700217866474929, 82.75041666666666629 ) ) ;
#48311=( GEOMETRIC_REPRESENTATION_CONTEXT ( 3 ) GLOBAL_UNCERTAINTY_ASSIGNED_CONTEXT ( ( #60177 ) ) GLOBAL_UNIT_ASSIGNED_CONTEXT ( ( #35673, #70248, #32250 ) ) REPRESENTATION_CONTEXT ( 'NONE', 'WORKASPACE' ) );
#48320=CARTESIAN_POINT ( 'NONE',  ( 0.000000000000000000, 0.000000000000000000, 0.000000000000000000 ) ) ;
#48326=CARTESIAN_POINT ( 'NONE',  ( 92.69370383062498320, 90.00000000000002842, 84.08656250086716000 ) ) ;
#48327=CARTESIAN_POINT ( 'NONE',  ( -93.84685191531248449, -208.0026889286704943, 86.41489583420049314 ) ) ;
#48328=CARTESIAN_POINT ( 'NONE',  ( 95.00000000000000000, -213.0599564267049857, 83.88812500173429498 ) ) ;
#48331=CARTESIAN_POINT ( 'NONE',  ( -97.64999999999994884, -211.5299782133524502, 81.79791666666666572 ) ) ;
#48332=CARTESIAN_POINT ( 'NONE',  ( -97.30629616937501680, 91.33154071421968467, 77.52489583420046415 ) ) ;
#48335=CARTESIAN_POINT ( 'NONE',  ( 97.30629616937498838, -209.9999999999999716, 84.88031250086713442 ) ) ;
#48338=ORIENTED_EDGE ( 'NONE', *, *, #12080, .F. ) ;
#48340=CARTESIAN_POINT ( 'NONE',  ( 97.64999999999992042, -208.4700217866474361, 84.02041666666666231 ) ) ;
#48343=CARTESIAN_POINT ( 'NONE',  ( 97.30629616937498838, -209.9999999999999716, 79.32406250086715715 ) ) ;
#48348=( BOUNDED_CURVE ( )  B_SPLINE_CURVE ( 2, ( #34914, #40548, #11235, #17985, #6352, #45843, #45092 ),
 .UNSPECIFIED., .F., .F. ) 
 B_SPLINE_CURVE_WITH_KNOTS ( ( 3, 2, 2, 3 ),
 ( 0.9374999999999995559, 0.9444444444444441977, 0.9513888888888889506, 0.9583333333333337034 ),
 .UNSPECIFIED. ) 
 CURVE ( )  GEOMETRIC_REPRESENTATION_ITEM ( )  RATIONAL_B_SPLINE_CURVE ( ( 1.000000000000008660, 0.8660254037844301589, 1.000000000000000000, 0.8660254037844387076, 1.000000000000000000, 0.8660254037844322683, 1.000000000000006439 ) ) 
 REPRESENTATION_ITEM ( '' )  );
#48351=CARTESIAN_POINT ( 'NONE',  ( 95.00000000000000000, -213.0599564267049857, 80.63375000000000625 ) ) ;
#48361=CARTESIAN_POINT ( 'NONE',  ( -97.30629616937501680, 91.33154071421968467, 82.76364583420048859 ) ) ;
#48362=CARTESIAN_POINT ( 'NONE',  ( 94.99999999999998579, 86.94004357329502852, 88.33312500173431658 ) ) ;
#48365=CARTESIAN_POINT ( 'NONE',  ( 92.34999999999999432, 91.52997821335252127, 75.34208333333333485 ) ) ;
#48366=ORIENTED_EDGE ( 'NONE', *, *, #57155, .F. ) ;
#48367=CARTESIAN_POINT ( 'NONE',  ( -93.67499999999998295, -207.7050326799711968, 84.78770833506763438 ) ) ;
#48371=CARTESIAN_POINT ( 'NONE',  ( -92.35000000000003695, 90.00000000000004263, 85.95187500173430806 ) ) ;
#48373=CARTESIAN_POINT ( 'NONE',  ( 94.99999999999998579, 92.66308142843935514, 86.46781250086716852 ) ) ;
#48374=CARTESIAN_POINT ( 'NONE',  ( -92.34999999999999432, -209.9999999999999716, 80.15749999999999886 ) ) ;
#48375=CARTESIAN_POINT ( 'NONE',  ( -92.35000000000003695, 89.99999997442942856, 84.04687500080852658 ) ) ;
#48376=CYLINDRICAL_SURFACE ( 'NONE', #69016, 2.649999999999985700 ) ;
#48383=VERTEX_POINT ( 'NONE', #50787 ) ;
#48385=CARTESIAN_POINT ( 'NONE',  ( 97.64999999999999147, 90.00000000000002842, 78.96687500173429441 ) ) ;
#48389=CARTESIAN_POINT ( 'NONE',  ( -92.69370383062498320, -211.3315407142195852, 83.08114583420048405 ) ) ;
#48391=CARTESIAN_POINT ( 'NONE',  ( -92.35000000000002274, -211.5299782133524786, 82.64458333333332973 ) ) ;
#48392=ADVANCED_FACE ( 'NONE', ( #38777 ), #61714, .F. ) ;
#48398=CARTESIAN_POINT ( 'NONE',  ( 92.69370383062498320, 88.66845928578037217, 88.58447916753382856 ) ) ;
#48400=CARTESIAN_POINT ( 'NONE',  ( 96.15314808468748708, 88.00268892867053694, 81.59947916753381492 ) ) ;
#48402=CARTESIAN_POINT ( 'NONE',  ( -96.32500000000001705, 92.29496732002878900, 80.44854166840097776 ) ) ;
#48406=DIRECTION ( 'NONE',  ( -0.000000000000000000, -0.000000000000000000, 1.000000000000000000 ) ) ;
#48411=EDGE_CURVE ( 'NONE', #22350, #51185, #45554, .T. ) ;
#48415=CARTESIAN_POINT ( 'NONE',  ( -92.69370383062505425, 91.33154071421968467, 86.83822916753381094 ) ) ;
#48422=AXIS2_PLACEMENT_3D ( 'NONE', #1582, #36852, #47404 ) ;
#48426=VECTOR ( 'NONE', #1575, 1000.000000000000000 ) ;
#48428=CARTESIAN_POINT ( 'NONE',  ( 97.30629616937498838, -211.3315407142195852, 80.54114583420049200 ) ) ;
#48436=CARTESIAN_POINT ( 'NONE',  ( 96.15314808468750130, -211.9973110713294489, 76.67822916753381435 ) ) ;
#48437=EDGE_LOOP ( 'NONE', ( #53166, #34603, #67103, #10555 ) ) ;
#48440=VERTEX_POINT ( 'NONE', #12422 ) ;
#48447=CARTESIAN_POINT ( 'NONE',  ( 95.00000000000000000, -206.9400435732949575, 84.20562500173429044 ) ) ;
#48449=CARTESIAN_POINT ( 'NONE',  ( 94.99999999999998579, 93.05995642670504253, 84.76125000000000398 ) ) ;
#48457=CARTESIAN_POINT ( 'NONE',  ( -97.30629616937501680, 91.33154071421968467, 86.57364583420047666 ) ) ;
#48458=CARTESIAN_POINT ( 'NONE',  ( 92.69370383062498320, 90.00000000000002842, 80.11781250086713158 ) ) ;
#48460=CARTESIAN_POINT ( 'NONE',  ( 96.32499999999998863, 87.70503267997126784, 82.67104166840096013 ) ) ;
#48462=FACE_OUTER_BOUND ( 'NONE', #46287, .T. ) ;
#48465=CARTESIAN_POINT ( 'NONE',  ( 97.64999999999999147, -209.9999999999999716, 78.25249999999999773 ) ) ;
#48468=ORIENTED_EDGE ( 'NONE', *, *, #23285, .F. ) ;
#48471=DIRECTION ( 'NONE',  ( 0.000000000000000000, 0.000000000000000000, -1.000000000000000000 ) ) ;
#48474=CARTESIAN_POINT ( 'NONE',  ( -97.65000000000001990, 88.47002178664754979, 84.33791666666667197 ) ) ;
#48479=VERTEX_POINT ( 'NONE', #11313 ) ;
#48480=CARTESIAN_POINT ( 'NONE',  ( 97.64999999999994884, -211.5299782133524786, 85.18458333333332178 ) ) ;
#48481=CARTESIAN_POINT ( 'NONE',  ( -92.69370383062498320, -211.3315407142195852, 79.74739583420047495 ) ) ;
#48488=VECTOR ( 'NONE', #39355, 1000.000000000000000 ) ;
#48496=CARTESIAN_POINT ( 'NONE',  ( -97.64998927488629477, -208.4700155945002393, 86.85145790673762178 ) ) ;
#48497=CARTESIAN_POINT ( 'NONE',  ( -93.84685191531252713, 88.00268892867056536, 75.24947916753380639 ) ) ;
#48506=CARTESIAN_POINT ( 'NONE',  ( 96.32499999999998863, -212.2949673200287179, 78.78166666666666629 ) ) ;
#48508=CARTESIAN_POINT ( 'NONE',  ( -93.67499999999998295, -207.7050326799711968, 86.61333333333332973 ) ) ;
#48511=VERTEX_POINT ( 'NONE', #34245 ) ;
#48512=CARTESIAN_POINT ( 'NONE',  ( 97.64999999999999147, 90.00000000000002842, 84.60249999999999204 ) ) ;
#48514=( NAMED_UNIT ( * ) PLANE_ANGLE_UNIT ( ) SI_UNIT ( $, .RADIAN. ) );
#48515=CARTESIAN_POINT ( 'NONE',  ( -97.64999999999999147, 91.52997821335250705, 84.86708333333332632 ) ) ;
#48518=DIRECTION ( 'NONE',  ( -1.000000000000000000, -0.000000000000000000, -0.000000000000000000 ) ) ;
#48521=CARTESIAN_POINT ( 'NONE',  ( 97.30629616937498838, -208.6684592857803295, 81.12322916753380753 ) ) ;
#48526=CARTESIAN_POINT ( 'NONE',  ( -95.00000000000002842, 93.05995642670504253, 79.68124999999999147 ) ) ;
#48527=ORIENTED_EDGE ( 'NONE', *, *, #4168, .T. ) ;
#48533=CARTESIAN_POINT ( 'NONE',  ( -92.69370383062502583, 91.33154071421968467, 77.47197916753381719 ) ) ;
#48534=ORIENTED_EDGE ( 'NONE', *, *, #3410, .T. ) ;
#48539=CARTESIAN_POINT ( 'NONE',  ( 92.34999999999999432, 91.52997821335252127, 88.12145833506765769 ) ) ;
#48545=ORIENTED_EDGE ( 'NONE', *, *, #21884, .F. ) ;
#48550=ORIENTED_EDGE ( 'NONE', *, *, #45722, .F. ) ;
#48552=CARTESIAN_POINT ( 'NONE',  ( 92.69370383062501162, -208.6684592857803011, 77.52489583420046415 ) ) ;
#48557=ORIENTED_EDGE ( 'NONE', *, *, #31672, .T. ) ;
#48558=CARTESIAN_POINT ( 'NONE',  ( -96.32500000000001705, 87.70503267997129626, 80.58083333333331666 ) ) ;
#48563=CARTESIAN_POINT ( 'NONE',  ( -97.30629616937495996, -209.9999999999999716, 82.65781250086713783 ) ) ;
#48565=CARTESIAN_POINT ( 'NONE',  ( -95.00000000000002842, 87.33691857156074434, 79.80031250086715033 ) ) ;
#48569=CARTESIAN_POINT ( 'NONE',  ( 96.15314808468748708, 91.99731107132950569, 81.17614583420048291 ) ) ;
#48570=( BOUNDED_CURVE ( )  B_SPLINE_CURVE ( 2, ( #32457, #20814, #50866, #60684, #50107, #49386, #4290 ),
 .UNSPECIFIED., .F., .F. ) 
 B_SPLINE_CURVE_WITH_KNOTS ( ( 3, 2, 2, 3 ),
 ( 0.4583333333333335924, 0.4652777777777780122, 0.4722222222222224319, 0.4791666666666668517 ),
 .UNSPECIFIED. ) 
 CURVE ( )  GEOMETRIC_REPRESENTATION_ITEM ( )  RATIONAL_B_SPLINE_CURVE ( ( 0.9999999999999946709, 0.8660254037844440367, 1.000000000000000000, 0.8660254037844387076, 1.000000000000000000, 0.8660254037844354880, 1.000000000000003109 ) ) 
 REPRESENTATION_ITEM ( '' )  );
#48574=CARTESIAN_POINT ( 'NONE',  ( -92.35000000000000853, -209.9999884513869119, 83.41187540116098376 ) ) ;
#48577=CARTESIAN_POINT ( 'NONE',  ( -97.30629616937497417, -208.6684592857803295, 82.60489583420049087 ) ) ;
#48587=CARTESIAN_POINT ( 'NONE',  ( -92.35000000000005116, 88.47002178664754979, 76.29458333333333542 ) ) ;
#48588=DIRECTION ( 'NONE',  ( 1.000000000000000000, 0.000000000000000000, 0.000000000000000000 ) ) ;
#48589=CARTESIAN_POINT ( 'NONE',  ( -92.69370383062502583, 91.33154071421968467, 84.29822916753380468 ) ) ;
#48596=CARTESIAN_POINT ( 'NONE',  ( -92.69370383062502583, 91.33154071421968467, 76.67822916753378593 ) ) ;
#48598=CARTESIAN_POINT ( 'NONE',  ( 90.00000000000000000, 85.00000000000002842, 90.00000000000000000 ) ) ;
#48599=DIRECTION ( 'NONE',  ( 1.000000000000000000, 1.343011723336883198E-16, 0.000000000000000000 ) ) ;
#48600=CARTESIAN_POINT ( 'NONE',  ( 95.00000000000000000, -206.9400435732949575, 84.76125000000000398 ) ) ;
#48602=CARTESIAN_POINT ( 'NONE',  ( -92.69370383062498320, -211.3315407142195852, 83.08114583420048405 ) ) ;
#48605=VECTOR ( 'NONE', #23777, 1000.000000000000000 ) ;
#48606=LINE ( 'NONE', #19651, #62311 ) ;
#48612=CARTESIAN_POINT ( 'NONE',  ( 96.32499999999998863, -207.7050326799711968, 79.62833333333333030 ) ) ;
#48614=DIRECTION ( 'NONE',  ( -0.000000000000000000, -0.000000000000000000, 1.000000000000000000 ) ) ;
#48615=CARTESIAN_POINT ( 'NONE',  ( 96.15314808468748708, -208.0026889286704943, 89.58989583420049030 ) ) ;
#48620=EDGE_LOOP ( 'NONE', ( #619, #72483, #24422, #58746 ) ) ;
#48634=ORIENTED_EDGE ( 'NONE', *, *, #51424, .F. ) ;
#48635=CARTESIAN_POINT ( 'NONE',  ( 97.30629616937498838, 88.66845928578037217, 80.54114583420049200 ) ) ;
#48641=ORIENTED_EDGE ( 'NONE', *, *, #56601, .F. ) ;
#48650=CARTESIAN_POINT ( 'NONE',  ( 92.34999999999998010, 89.99999071025125374, 78.01437532303467037 ) ) ;
#48655=CARTESIAN_POINT ( 'NONE',  ( -92.34999999999999432, -209.9999999999999716, 76.42687500173430237 ) ) ;
#48657=CARTESIAN_POINT ( 'NONE',  ( -96.15314808468751551, 88.00268892867056536, 88.63739583420048973 ) ) ;
#48658=EDGE_CURVE ( 'NONE', #49261, #4256, #9257, .T. ) ;
#48659=CARTESIAN_POINT ( 'NONE',  ( 97.64999999999997726, 88.47002178664753558, 75.10395833506764518 ) ) ;
#48660=CARTESIAN_POINT ( 'NONE',  ( -92.69370383062502583, 88.66845928578038638, 88.00239583420047040 ) ) ;
#48662=CARTESIAN_POINT ( 'NONE',  ( 97.30629616937498838, 88.66845928578037217, 76.09614583420048461 ) ) ;
#48666=CARTESIAN_POINT ( 'NONE',  ( -93.67500000000003979, 92.29496732002878900, 78.43770833506764006 ) ) ;
#48670=FACE_BOUND ( 'NONE', #46255, .T. ) ;
#48675=CARTESIAN_POINT ( 'NONE',  ( -93.67500000000003979, 92.29496732002878900, 86.05770833506763040 ) ) ;
#48677=CARTESIAN_POINT ( 'NONE',  ( -93.67500000000003979, 87.70503267997129626, 76.32104166840096582 ) ) ;
#48683=CARTESIAN_POINT ( 'NONE',  ( -92.35000000000003695, 90.00000000000004263, 78.88750000000000284 ) ) ;
#48690=CARTESIAN_POINT ( 'NONE',  ( 94.99999999999998579, 92.66308142843932671, 85.19781250086714408 ) ) ;
#48691=CARTESIAN_POINT ( 'NONE',  ( -97.30629616937497417, -208.6684592857803295, 82.76364583420048859 ) ) ;
#48695=CARTESIAN_POINT ( 'NONE',  ( -92.34999999999999432, -208.4700217866474645, 79.57541666666665492 ) ) ;
#48697=AXIS2_PLACEMENT_3D ( 'NONE', #11825, #18223, #40411 ) ;
#48699=CARTESIAN_POINT ( 'NONE',  ( 92.69370383062501162, -211.3315407142195852, 85.25072916753379104 ) ) ;
#48703=FACE_OUTER_BOUND ( 'NONE', #5655, .T. ) ;
#48713=CARTESIAN_POINT ( 'NONE',  ( 95.00000000000000000, -212.6630814284392557, 77.89531250086714920 ) ) ;
#48720=CARTESIAN_POINT ( 'NONE',  ( 92.35000000000002274, -208.4700217866474645, 79.78708333333332803 ) ) ;
#48723=EDGE_LOOP ( 'NONE', ( #9433, #25164, #51591, #28878, #41065, #36686, #73428, #40315, #17952, #9461, #25780, #62832, #70202, #7514, #53683, #56973 ) ) ;
#48727=CARTESIAN_POINT ( 'NONE',  ( -93.84685191531252713, 88.00268892867056536, 82.39322916753381776 ) ) ;
#48730=CYLINDRICAL_SURFACE ( 'NONE', #9474, 2.649999999999999467 ) ;
#48733=CARTESIAN_POINT ( 'NONE',  ( -96.32499999999996021, -207.7050326799711968, 86.16354166840096696 ) ) ;
#48738=CARTESIAN_POINT ( 'NONE',  ( -92.35000000000005116, 91.52997821335253548, 87.90979166840095615 ) ) ;
#48739=VERTEX_POINT ( 'NONE', #52499 ) ;
#48741=CARTESIAN_POINT ( 'NONE',  ( 92.69370383062498320, 90.00000000000002842, 85.99156250086716113 ) ) ;
#48744=CARTESIAN_POINT ( 'NONE',  ( -96.32500000000001705, 87.70503267997129626, 83.83520833506763381 ) ) ;
#48753=VECTOR ( 'NONE', #61455, 1000.000000000000000 ) ;
#48754=CARTESIAN_POINT ( 'NONE',  ( 97.65000000000000568, 88.47002178664752137, 78.91395833506763324 ) ) ;
#48760=CARTESIAN_POINT ( 'NONE',  ( -93.84685191531247028, -211.9973110713294489, 84.93322916753382401 ) ) ;
#48763=ORIENTED_EDGE ( 'NONE', *, *, #57459, .T. ) ;
#48765=CARTESIAN_POINT ( 'NONE',  ( 92.34999999999995168, 91.52997821335250705, 86.77208333333334167 ) ) ;
#48767=CARTESIAN_POINT ( 'NONE',  ( -93.67499999999998295, -212.2949673200287179, 76.32104166840096582 ) ) ;
#48768=CARTESIAN_POINT ( 'NONE',  ( 92.69370383062498320, 91.33154071421968467, 78.15989583420048348 ) ) ;
#48777=CARTESIAN_POINT ( 'NONE',  ( 96.32499999999997442, 92.29496732002878900, 89.15333333333333599 ) ) ;
#48779=CARTESIAN_POINT ( 'NONE',  ( -97.30629616937501680, 88.66845928578038638, 82.07572916753382231 ) ) ;
#48780=CARTESIAN_POINT ( 'NONE',  ( -2.499999999999970690, 73.00000000000001421, -255.0000000000000000 ) ) ;
#48785=( BOUNDED_CURVE ( )  B_SPLINE_CURVE ( 2, ( #6420, #18060, #34983, #29322, #62461, #10556, #11303 ),
 .UNSPECIFIED., .F., .F. ) 
 B_SPLINE_CURVE_WITH_KNOTS ( ( 3, 2, 2, 3 ),
 ( 0.000000000000000000, 0.006944444444444406762, 0.01388888888888881352, 0.02083333333333322115 ),
 .UNSPECIFIED. ) 
 CURVE ( )  GEOMETRIC_REPRESENTATION_ITEM ( )  RATIONAL_B_SPLINE_CURVE ( ( 1.000000000000000000, 0.8660254037844387076, 1.000000000000000000, 0.8660254037844387076, 1.000000000000000000, 0.8660254037844408170, 0.9999999999999978906 ) ) 
 REPRESENTATION_ITEM ( '' )  );
#48791=CARTESIAN_POINT ( 'NONE',  ( 96.15314808468750130, -211.9973110713294489, 79.21822916753382060 ) ) ;
#48792=AXIS2_PLACEMENT_3D ( 'NONE', #69997, #47093, #69642 ) ;
#48797=AXIS2_PLACEMENT_3D ( 'NONE', #13896, #47749, #59412 ) ;
#48798=EDGE_CURVE ( 'NONE', #55390, #26258, #25070, .T. ) ;
#48799=CARTESIAN_POINT ( 'NONE',  ( -2.499999999999970690, 73.00000000000001421, -204.9999999999999716 ) ) ;
#48804=CARTESIAN_POINT ( 'NONE',  ( 93.84685191531251292, -211.9973110713294489, 75.30239583420048177 ) ) ;
#48809=ORIENTED_EDGE ( 'NONE', *, *, #39201, .T. ) ;
#48810=CARTESIAN_POINT ( 'NONE',  ( -97.64996285368241047, -208.4700003402110156, 82.40645685155115530 ) ) ;
#48812=CARTESIAN_POINT ( 'NONE',  ( -93.67500000000003979, 92.29496732002878900, 89.23270833506762756 ) ) ;
#48815=CARTESIAN_POINT ( 'NONE',  ( 96.32499999999998863, -207.7050326799711968, 82.88270833506763324 ) ) ;
#48816=CARTESIAN_POINT ( 'NONE',  ( 92.34999999999999432, 91.52997821335252127, 86.13708333333332234 ) ) ;
#48822=ORIENTED_EDGE ( 'NONE', *, *, #74092, .F. ) ;
#48823=CARTESIAN_POINT ( 'NONE',  ( -96.15314808468752972, 91.99731107132950569, 89.06072916753382174 ) ) ;
#48824=CARTESIAN_POINT ( 'NONE',  ( 94.99999999999998579, 92.66308142843935514, 81.86406250086714920 ) ) ;
#48826=CARTESIAN_POINT ( 'NONE',  ( 93.67499999999998295, 92.29496732002878900, 81.08354166840096866 ) ) ;
#48834=CARTESIAN_POINT ( 'NONE',  ( -95.00000000000002842, 86.94004357329504273, 82.61812500173428475 ) ) ;
#48836=CARTESIAN_POINT ( 'NONE',  ( -95.00000000000002842, 86.94004357329504273, 83.80875000000000341 ) ) ;
#48839=CARTESIAN_POINT ( 'NONE',  ( 97.64999999999997726, 91.52997821335252127, 88.54479166840097548 ) ) ;
#48841=DIRECTION ( 'NONE',  ( -0.000000000000000000, -0.000000000000000000, 1.000000000000000000 ) ) ;
#48842=CARTESIAN_POINT ( 'NONE',  ( -92.69370383062498320, -208.6684592857803011, 77.94822916753381037 ) ) ;
#48843=ORIENTED_EDGE ( 'NONE', *, *, #3587, .F. ) ;
#48852=CARTESIAN_POINT ( 'NONE',  ( 92.69370383062498320, 91.33154071421968467, 89.58989583420047609 ) ) ;
#48855=CARTESIAN_POINT ( 'NONE',  ( -94.99999999999997158, -206.9400435732949575, 86.74562500173429669 ) ) ;
#48856=CARTESIAN_POINT ( 'NONE',  ( -95.00000000000002842, 92.66308142843932671, 76.14906250086716000 ) ) ;
#48857=CYLINDRICAL_SURFACE ( 'NONE', #52665, 2.649999999999999467 ) ;
#48862=DIRECTION ( 'NONE',  ( -0.000000000000000000, -0.000000000000000000, 1.000000000000000000 ) ) ;
#48863=EDGE_CURVE ( 'NONE', #28639, #73949, #12553, .T. ) ;
#48865=UNCERTAINTY_MEASURE_WITH_UNIT (LENGTH_MEASURE( 1.000000000000000082E-05 ), #23668, 'distance_accuracy_value', 'NONE');
#48868=CARTESIAN_POINT ( 'NONE',  ( 96.66734480923263106, 87.91120745868266795, 75.00000000000000000 ) ) ;
#48872=CARTESIAN_POINT ( 'NONE',  ( -97.64999999999994884, -211.5299782133524502, 87.51291666666666913 ) ) ;
#48878=CARTESIAN_POINT ( 'NONE',  ( -97.30629616937495996, -209.9999999999999716, 89.80156250086714920 ) ) ;
#48886=CARTESIAN_POINT ( 'NONE',  ( 92.69370383062501162, -209.9999999999999716, 83.29281250086714294 ) ) ;
#48888=CARTESIAN_POINT ( 'NONE',  ( 97.30629616937498838, -211.3315407142195852, 87.52614583420049144 ) ) ;
#48890=CARTESIAN_POINT ( 'NONE',  ( -93.67499999999998295, -212.2949673200287179, 80.68666666666665321 ) ) ;
#48894=CARTESIAN_POINT ( 'NONE',  ( -95.00000000000002842, 92.66308142843932671, 78.84781250086714977 ) ) ;
#48906=ORIENTED_EDGE ( 'NONE', *, *, #51009, .T. ) ;
#48908=ORIENTED_EDGE ( 'NONE', *, *, #35488, .T. ) ;
#48911=CARTESIAN_POINT ( 'NONE',  ( 93.84685191531251292, -211.9973110713294489, 78.95364583420047211 ) ) ;
#48914=CARTESIAN_POINT ( 'NONE',  ( -95.00000000000002842, 90.00000000000004263, 90.00000000000000000 ) ) ;
#48922=CARTESIAN_POINT ( 'NONE',  ( -93.84685191531254134, 91.99731107132950569, 80.06489583420048461 ) ) ;
#48924=CARTESIAN_POINT ( 'NONE',  ( 97.30629616937498838, 88.66845928578037217, 77.20739583420046870 ) ) ;
#48927=CARTESIAN_POINT ( 'NONE',  ( -96.15314808468745866, -211.9973110713294489, 88.47864583420047779 ) ) ;
#48931=CARTESIAN_POINT ( 'NONE',  ( -96.15314808468745866, -211.9973110713294489, 83.39864583420047950 ) ) ;
#48940=CARTESIAN_POINT ( 'NONE',  ( -92.69370383062502583, 88.66845928578038638, 86.09739583420048348 ) ) ;
#48947=DIRECTION ( 'NONE',  ( 1.000000000000000000, 0.000000000000000000, 0.000000000000000000 ) ) ;
#48950=ADVANCED_FACE ( 'NONE', ( #19402 ), #42350, .F. ) ;
#48953=CARTESIAN_POINT ( 'NONE',  ( 97.64999999999999147, 90.00000000000002842, 86.50750000000000739 ) ) ;
#48954=CARTESIAN_POINT ( 'NONE',  ( -93.84685191531248449, -208.0026889286704943, 81.96989583420048575 ) ) ;
#48964=CARTESIAN_POINT ( 'NONE',  ( -97.64999999999996305, -211.5299782133524218, 81.87729166840097150 ) ) ;
#48969=CARTESIAN_POINT ( 'NONE',  ( -95.00000000000002842, 90.00000000000004263, 90.00000000000000000 ) ) ;
#48972=AXIS2_PLACEMENT_3D ( 'NONE', #33609, #73827, #22339 ) ;
#48976=EDGE_LOOP ( 'NONE', ( #40054, #16948, #31499, #36507 ) ) ;
#48987=VERTEX_POINT ( 'NONE', #14461 ) ;
#48991=( BOUNDED_CURVE ( )  B_SPLINE_CURVE ( 2, ( #41901, #14050, #30602, #55025, #25715, #48281, #13323, #3554, #18955 ),
 .UNSPECIFIED., .F., .F. ) 
 B_SPLINE_CURVE_WITH_KNOTS ( ( 3, 2, 2, 2, 3 ),
 ( 0.3386766260354857061, 0.3386767459640170341, 0.3457325115049341147, 0.3527882770458510842, 0.3598440426548558668 ),
 .UNSPECIFIED. ) 
 CURVE ( )  GEOMETRIC_REPRESENTATION_ITEM ( )  RATIONAL_B_SPLINE_CURVE ( ( 0.9999954456810212777, 0.9999977228018045450, 1.000000000000000000, 0.8660254037844387076, 1.000000000000000000, 0.8660254037844387076, 1.000000000000000000, 0.8660254037844387076, 1.000000000000000000 ) ) 
 REPRESENTATION_ITEM ( '' )  );
#48992=CARTESIAN_POINT ( 'NONE',  ( 92.69370383062498320, 88.66845928578037217, 75.88447916753382572 ) ) ;
#48994=CARTESIAN_POINT ( 'NONE',  ( -97.65000000000000568, 89.99999348150292633, 88.17437522718661569 ) ) ;
#48999=DIRECTION ( 'NONE',  ( -0.000000000000000000, -0.000000000000000000, 1.000000000000000000 ) ) ;
#49001=CARTESIAN_POINT ( 'NONE',  ( 95.00000000000000000, -207.3369185715606307, 89.48406250086713953 ) ) ;
#49011=CARTESIAN_POINT ( 'NONE',  ( -92.34999999999999432, -209.9999999999999716, 75.15687500173430635 ) ) ;
#49012=CARTESIAN_POINT ( 'NONE',  ( -97.30629616937501680, 88.66845928578038638, 88.58447916753382856 ) ) ;
#49015=CARTESIAN_POINT ( 'NONE',  ( 92.34999999999999432, 90.00000000000002842, 76.74437500173429783 ) ) ;
#49016=CARTESIAN_POINT ( 'NONE',  ( -96.15314808468751551, 88.00268892867056536, 87.84364583420047268 ) ) ;
#49018=CARTESIAN_POINT ( 'NONE',  ( 94.99999999999998579, 87.33691857156068750, 75.99031250086716227 ) ) ;
#49022=CARTESIAN_POINT ( 'NONE',  ( -97.64998056384376923, 91.52998943482256777, 78.59645755884378104 ) ) ;
#49023=CARTESIAN_POINT ( 'NONE',  ( -97.65000000000007674, 91.52997821335250705, 89.31208333333333371 ) ) ;
#49025=CARTESIAN_POINT ( 'NONE',  ( -94.99999999999997158, -213.0599564267049857, 87.61874999999999147 ) ) ;
#49028=AXIS2_PLACEMENT_3D ( 'NONE', #19591, #59462, #70718 ) ;
#49029=ORIENTED_EDGE ( 'NONE', *, *, #9985, .T. ) ;
#49030=VECTOR ( 'NONE', #65676, 1000.000000000000000 ) ;
#49033=CARTESIAN_POINT ( 'NONE',  ( -97.64999999969889188, -209.9999754409357422, 87.53856274002470172 ) ) ;
#49037=DIRECTION ( 'NONE',  ( -1.000000000000000000, 3.061616997868382648E-16, 0.000000000000000000 ) ) ;
#49041=VERTEX_POINT ( 'NONE', #70473 ) ;
#49043=CARTESIAN_POINT ( 'NONE',  ( -93.84685191531254134, 91.99731107132950569, 82.44614583420046472 ) ) ;
#49058=CARTESIAN_POINT ( 'NONE',  ( 92.69370383062498320, 91.33154071421968467, 82.76364583420048859 ) ) ;
#49060=CARTESIAN_POINT ( 'NONE',  ( -97.30629616937497417, -208.6684592857803295, 83.39864583420049371 ) ) ;
#49064=CARTESIAN_POINT ( 'NONE',  ( -93.67499999999998295, -207.7050326799711968, 77.08833333333332405 ) ) ;
#49066=AXIS2_PLACEMENT_3D ( 'NONE', #45561, #29343, #34621 ) ;
#49068=CARTESIAN_POINT ( 'NONE',  ( 95.00000000000000000, -207.3369185715606307, 82.49906250086714010 ) ) ;
#49082=CARTESIAN_POINT ( 'NONE',  ( 97.30629616937498838, -208.6684592857803295, 76.83697916753382628 ) ) ;
#49089=CARTESIAN_POINT ( 'NONE',  ( 97.64999999999997726, -208.4700217866474645, 80.84541666666666515 ) ) ;
#49096=CARTESIAN_POINT ( 'NONE',  ( -92.69370383062502583, 88.66845928578038638, 84.35114583420049428 ) ) ;
#49097=CARTESIAN_POINT ( 'NONE',  ( -92.35000000000678710, 90.00000598221780024, 82.14187520865721126 ) ) ;
#49099=CARTESIAN_POINT ( 'NONE',  ( 93.67499999999998295, 92.29496732002878900, 75.28916666666665947 ) ) ;
#49103=CARTESIAN_POINT ( 'NONE',  ( -94.99999999999997158, -206.9400435732949575, 86.11062500173430578 ) ) ;
#49107=CARTESIAN_POINT ( 'NONE',  ( -95.00000000000002842, 86.94004357329504273, 83.88812500173429498 ) ) ;
#49110=CARTESIAN_POINT ( 'NONE',  ( 97.30629616937498838, 88.66845928578037217, 88.16114583420048234 ) ) ;
#49113=EDGE_CURVE ( 'NONE', #39397, #6687, #43569, .T. ) ;
#49121=VERTEX_POINT ( 'NONE', #59218 ) ;
#49129=CARTESIAN_POINT ( 'NONE',  ( -94.99999999999997158, -212.6630814284392557, 84.88031250086714863 ) ) ;
#49138=VECTOR ( 'NONE', #42747, 1000.000000000000000 ) ;
#49140=CARTESIAN_POINT ( 'NONE',  ( -97.64999999999996305, -209.9999999999999716, 76.10937500173430692 ) ) ;
#49141=CARTESIAN_POINT ( 'NONE',  ( 97.30629616937498838, 90.00000000000002842, 79.16531250086714522 ) ) ;
#49146=CARTESIAN_POINT ( 'NONE',  ( 93.09104985768151153, 91.56137061862943938, 74.88237134757152091 ) ) ;
#49152=CARTESIAN_POINT ( 'NONE',  ( 97.64999999999990621, 91.52997821335254969, 89.10041666666667481 ) ) ;
#49154=CARTESIAN_POINT ( 'NONE',  ( -96.15314808468751551, 88.00268892867056536, 81.49364583420047836 ) ) ;
#49158=EDGE_CURVE ( 'NONE', #48440, #7925, #27202, .T. ) ;
#49162=EDGE_CURVE ( 'NONE', #15980, #70981, #16955, .T. ) ;
#49163=CARTESIAN_POINT ( 'NONE',  ( 97.65000000000003411, 91.52997821335250705, 85.29041666666665833 ) ) ;
#49167=CARTESIAN_POINT ( 'NONE',  ( 92.69370383062501162, -208.6684592857803011, 78.95364583420048632 ) ) ;
#49175=CARTESIAN_POINT ( 'NONE',  ( 92.69370383062501162, -211.3315407142195852, 77.15447916753382174 ) ) ;
#49182=AXIS2_PLACEMENT_3D ( 'NONE', #64104, #11471, #11829 ) ;
#49186=EDGE_LOOP ( 'NONE', ( #587, #19320, #73413, #15445 ) ) ;
#49188=CARTESIAN_POINT ( 'NONE',  ( 95.00000000000000000, -213.0599564267049857, 78.80812500173429669 ) ) ;
#49189=CARTESIAN_POINT ( 'NONE',  ( 97.64999999999999147, 90.00000000000002842, 85.23749999999999716 ) ) ;
#49192=DIRECTION ( 'NONE',  ( -0.000000000000000000, -0.000000000000000000, -1.000000000000000000 ) ) ;
#49193=ORIENTED_EDGE ( 'NONE', *, *, #59971, .F. ) ;
#49194=CARTESIAN_POINT ( 'NONE',  ( -92.69370383062505425, 88.66845928578038638, 88.16114583420048234 ) ) ;
#49195=CARTESIAN_POINT ( 'NONE',  ( 97.30629616937498838, 90.00000000000002842, 82.34031250086714238 ) ) ;
#49203=ORIENTED_EDGE ( 'NONE', *, *, #9829, .T. ) ;
#49208=( BOUNDED_CURVE ( )  B_SPLINE_CURVE ( 2, ( #9950, #32872, #55821, #44552, #52392, #69320, #40761, #13282, #63328, #64430, #35111 ),
 .UNSPECIFIED., .F., .F. ) 
 B_SPLINE_CURVE_WITH_KNOTS ( ( 3, 2, 2, 2, 2, 3 ),
 ( 0.4233457466685772164, 0.4233459324529421641, 0.4304016979938243836, 0.4374574635347066587, 0.4445132290755888782, 0.4445132602971387792 ),
 .UNSPECIFIED. ) 
 CURVE ( )  GEOMETRIC_REPRESENTATION_ITEM ( )  RATIONAL_B_SPLINE_CURVE ( ( 0.9999929448534692344, 0.9999964723338481409, 1.000000000000000000, 0.8660254037844387076, 1.000000000000000000, 0.8660254037844387076, 1.000000000000000000, 0.8660254037844387076, 1.000000000000000000, 0.9999994071664494166, 0.9999988143381453032 ) ) 
 REPRESENTATION_ITEM ( '' )  );
#49212=CARTESIAN_POINT ( 'NONE',  ( -97.30629616937497417, -208.6684592857803011, 78.79489583420047438 ) ) ;
#49213=ORIENTED_EDGE ( 'NONE', *, *, #49716, .T. ) ;
#49224=CARTESIAN_POINT ( 'NONE',  ( 92.69370383062498320, 88.66845928578035796, 87.79072916753379729 ) ) ;
#49225=FACE_OUTER_BOUND ( 'NONE', #7422, .T. ) ;
#49227=CARTESIAN_POINT ( 'NONE',  ( 95.73997229764715655, -212.5681771730651235, 75.00000000000000000 ) ) ;
#49231=EDGE_CURVE ( 'NONE', #14688, #66971, #55816, .T. ) ;
#49238=CARTESIAN_POINT ( 'NONE',  ( 92.69370383062498320, 88.66845928578035796, 89.21947916753381946 ) ) ;
#49240=FACE_OUTER_BOUND ( 'NONE', #58425, .T. ) ;
#49242=CARTESIAN_POINT ( 'NONE',  ( -97.64999999999994884, -208.4700217866474645, 87.40708333333333258 ) ) ;
#49259=CARTESIAN_POINT ( 'NONE',  ( 93.84685191531249870, -208.0026889286704943, 81.91697916753381037 ) ) ;
#49260=CARTESIAN_POINT ( 'NONE',  ( 97.30629616937498838, -209.9999999999999716, 83.76906250086716454 ) ) ;
#49261=VERTEX_POINT ( 'NONE', #67074 ) ;
#49263=CARTESIAN_POINT ( 'NONE',  ( 95.00000000000000000, -212.6630814284392557, 88.05531250086716000 ) ) ;
#49269=CARTESIAN_POINT ( 'NONE',  ( -97.30629616937501680, 88.66845928578038638, 76.51947916753381662 ) ) ;
#49285=CARTESIAN_POINT ( 'NONE',  ( 93.84685191531251292, -211.9973110713294489, 77.68364583420047609 ) ) ;
#49296=CARTESIAN_POINT ( 'NONE',  ( -96.15314808468751551, 88.00268892867056536, 79.11239583420048405 ) ) ;
#49298=CARTESIAN_POINT ( 'NONE',  ( 92.69370383062498320, 90.00000000000002842, 78.21281250086714465 ) ) ;
#49300=CYLINDRICAL_SURFACE ( 'NONE', #74335, 2.649999999999985700 ) ;
#49301=CARTESIAN_POINT ( 'NONE',  ( -97.30629616937495996, -209.9999999999999716, 89.64281250086713726 ) ) ;
#49303=FACE_BOUND ( 'NONE', #46331, .T. ) ;
#49305=CARTESIAN_POINT ( 'NONE',  ( -92.69370383062498320, -209.9999999999999716, 79.80031250086713612 ) ) ;
#49314=CARTESIAN_POINT ( 'NONE',  ( -95.00000000000002842, 86.94004357329504273, 84.52312500173428589 ) ) ;
#49315=CARTESIAN_POINT ( 'NONE',  ( -97.30629616937501680, 91.33154071421968467, 86.41489583420047893 ) ) ;
#49319=ORIENTED_EDGE ( 'NONE', *, *, #65258, .T. ) ;
#49324=AXIS2_PLACEMENT_3D ( 'NONE', #50138, #67450, #15942 ) ;
#49331=CARTESIAN_POINT ( 'NONE',  ( -95.00000000000002842, 93.05995642670504253, 87.30124999999999602 ) ) ;
#49332=CARTESIAN_POINT ( 'NONE',  ( -96.15314808468745866, -211.9973110713294489, 83.55739583420049144 ) ) ;
#49334=EDGE_CURVE ( 'NONE', #15908, #39621, #42126, .T. ) ;
#49340=EDGE_CURVE ( 'NONE', #17937, #71124, #63513, .T. ) ;
#49347=( BOUNDED_CURVE ( )  B_SPLINE_CURVE ( 2, ( #56053, #73703, #16567, #51522, #9815, #4197, #44411 ),
 .UNSPECIFIED., .F., .F. ) 
 B_SPLINE_CURVE_WITH_KNOTS ( ( 3, 2, 2, 3 ),
 ( 0.08333333333333288462, 0.09027777777777759582, 0.09722222222222230703, 0.1041666666666670182 ),
 .UNSPECIFIED. ) 
 CURVE ( )  GEOMETRIC_REPRESENTATION_ITEM ( )  RATIONAL_B_SPLINE_CURVE ( ( 1.000000000000008660, 0.8660254037844301589, 1.000000000000000000, 0.8660254037844387076, 1.000000000000000000, 0.8660254037844320463, 1.000000000000006661 ) ) 
 REPRESENTATION_ITEM ( '' )  );
#49354=CARTESIAN_POINT ( 'NONE',  ( -92.35002849301773153, -208.4700053361959817, 87.27479280632964276 ) ) ;
#49357=ORIENTED_EDGE ( 'NONE', *, *, #61870, .F. ) ;
#49360=EDGE_LOOP ( 'NONE', ( #33642, #18209, #67328, #45197 ) ) ;
#49367=CARTESIAN_POINT ( 'NONE',  ( 93.84685191531248449, 91.99731107132950569, 77.63072916753381492 ) ) ;
#49368=DIRECTION ( 'NONE',  ( 1.000000000000000000, 0.000000000000000000, 0.000000000000000000 ) ) ;
#49370=ORIENTED_EDGE ( 'NONE', *, *, #10291, .F. ) ;
#49373=EDGE_CURVE ( 'NONE', #49572, #53174, #17855, .T. ) ;
#49375=CARTESIAN_POINT ( 'NONE',  ( 92.69370383062498320, 88.66845928578037217, 87.15572916753380639 ) ) ;
#49378=CARTESIAN_POINT ( 'NONE',  ( 93.84685191531249870, -208.0026889286704943, 89.53697916753381492 ) ) ;
#49380=LINE ( 'NONE', #67792, #8978 ) ;
#49382=VECTOR ( 'NONE', #53491, 1000.000000000000000 ) ;
#49386=CARTESIAN_POINT ( 'NONE',  ( -92.34999999999995168, -208.4700217866474929, 82.75041666666666629 ) ) ;
#49390=CARTESIAN_POINT ( 'NONE',  ( -92.34999999999999432, -208.4700217866474645, 77.11479166840095445 ) ) ;
#49391=CARTESIAN_POINT ( 'NONE',  ( -95.00000000000002842, 87.33691857156074434, 89.32531250086715602 ) ) ;
#49395=CARTESIAN_POINT ( 'NONE',  ( 93.84685191531248449, 88.00268892867053694, 89.11364583420048291 ) ) ;
#49396=CARTESIAN_POINT ( 'NONE',  ( -96.15314808468752972, 91.99731107132950569, 86.99697916753380866 ) ) ;
#49397=ORIENTED_EDGE ( 'NONE', *, *, #33768, .T. ) ;
#49400=CARTESIAN_POINT ( 'NONE',  ( -94.99999999999997158, -209.9999999999999716, 90.00000000000000000 ) ) ;
#49411=CARTESIAN_POINT ( 'NONE',  ( -95.00000000000002842, 86.94004357329504273, 79.99874999999998693 ) ) ;
#49416=CARTESIAN_POINT ( 'NONE',  ( -97.65000000000003411, 90.00001272927832474, 76.10937456147250657 ) ) ;
#49419=CARTESIAN_POINT ( 'NONE',  ( -97.30629616937501680, 88.66845928578038638, 82.07572916753380809 ) ) ;
#49423=DIRECTION ( 'NONE',  ( 1.000000000000000000, 0.000000000000000000, 0.000000000000000000 ) ) ;
#49427=CARTESIAN_POINT ( 'NONE',  ( 97.65000000000000568, -208.4700217866474645, 80.28979166840095161 ) ) ;
#49430=CARTESIAN_POINT ( 'NONE',  ( 92.69370383062498320, 88.66845928578035796, 79.05947916753382287 ) ) ;
#49431=CARTESIAN_POINT ( 'NONE',  ( -93.84685191531248449, -208.0026889286704943, 83.87489583420048689 ) ) ;
#49435=CARTESIAN_POINT ( 'NONE',  ( 0.000000000000000000, 0.000000000000000000, -80.00000000000000000 ) ) ;
#49437=CARTESIAN_POINT ( 'NONE',  ( -92.34999999999999432, -209.9999999999999716, 76.98250000000000171 ) ) ;
#49440=CARTESIAN_POINT ( 'NONE',  ( 96.15314808468750130, -211.9973110713294489, 84.77447916753381207 ) ) ;
#49442=AXIS2_PLACEMENT_3D ( 'NONE', #59042, #36827, #71035 ) ;
#49446=( BOUNDED_CURVE ( )  B_SPLINE_CURVE ( 2, ( #44674, #33357, #9321, #55193, #20974, #56317, #3717 ),
 .UNSPECIFIED., .F., .F. ) 
 B_SPLINE_CURVE_WITH_KNOTS ( ( 3, 2, 2, 3 ),
 ( 0.1250000000000002220, 0.1319444444444446418, 0.1388888888888890338, 0.1458333333333334536 ),
 .UNSPECIFIED. ) 
 CURVE ( )  GEOMETRIC_REPRESENTATION_ITEM ( )  RATIONAL_B_SPLINE_CURVE ( ( 0.9999999999999956701, 0.8660254037844430375, 1.000000000000000000, 0.8660254037844387076, 1.000000000000000000, 0.8660254037844365982, 1.000000000000002220 ) ) 
 REPRESENTATION_ITEM ( '' )  );
#49448=VERTEX_POINT ( 'NONE', #57663 ) ;
#49453=CARTESIAN_POINT ( 'NONE',  ( 92.69370383062501162, -208.6684592857803295, 77.04864583420048518 ) ) ;
#49454=CARTESIAN_POINT ( 'NONE',  ( -94.99999999999997158, -209.9999999999999716, 90.00000000000000000 ) ) ;
#49457=CARTESIAN_POINT ( 'NONE',  ( 96.15314808468748708, 88.00268892867053694, 87.47322916753381605 ) ) ;
#49458=CARTESIAN_POINT ( 'NONE',  ( -97.64999999960629395, 90.00002930740643592, 76.74344264317980446 ) ) ;
#49459=CARTESIAN_POINT ( 'NONE',  ( 96.32499999999998863, -207.7050326799711968, 82.80333333333332746 ) ) ;
#49461=ORIENTED_EDGE ( 'NONE', *, *, #35209, .F. ) ;
#49467=CARTESIAN_POINT ( 'NONE',  ( -92.69370383062504004, 90.00000000000004263, 83.76906250086716454 ) ) ;
#49469=CARTESIAN_POINT ( 'NONE',  ( -92.35000000000005116, 88.47002178664754979, 82.08895833506764461 ) ) ;
#49475=CARTESIAN_POINT ( 'NONE',  ( -94.99999999999997158, -206.9400435732949575, 87.38062500173430180 ) ) ;
#49479=CARTESIAN_POINT ( 'NONE',  ( -95.00000000000002842, 93.05995642670501411, 82.30062500173428930 ) ) ;
#49482=CARTESIAN_POINT ( 'NONE',  ( 93.84685191531248449, 88.00268892867053694, 87.36739583420049371 ) ) ;
#49491=VERTEX_POINT ( 'NONE', #49590 ) ;
#49500=CARTESIAN_POINT ( 'NONE',  ( -97.30629616937497417, -208.6684592857803011, 85.93864583420048575 ) ) ;
#49504=CARTESIAN_POINT ( 'NONE',  ( -97.64999999999996305, -209.9999999999999716, 90.00000000000000000 ) ) ;
#49510=CARTESIAN_POINT ( 'NONE',  ( 94.99999999999998579, 87.33691857156068750, 79.00656250086714749 ) ) ;
#49512=DIRECTION ( 'NONE',  ( -0.000000000000000000, -0.000000000000000000, -1.000000000000000000 ) ) ;
#49514=DIRECTION ( 'NONE',  ( -0.000000000000000000, -0.000000000000000000, 1.000000000000000000 ) ) ;
#49516=CARTESIAN_POINT ( 'NONE',  ( -92.34999999999996589, -211.5299782133523934, 87.08958333333333712 ) ) ;
#49520=CARTESIAN_POINT ( 'NONE',  ( -97.30629616937501680, 88.66845928578038638, 83.98072916753380923 ) ) ;
#49530=CARTESIAN_POINT ( 'NONE',  ( 97.30629616937498838, -209.9999999999999716, 77.41906250086715602 ) ) ;
#49534=VERTEX_POINT ( 'NONE', #66171 ) ;
#49543=CARTESIAN_POINT ( 'NONE',  ( 92.69370383062501162, -209.9999999999999716, 76.46656250086715545 ) ) ;
#49545=ORIENTED_EDGE ( 'NONE', *, *, #42010, .T. ) ;
#49548=VECTOR ( 'NONE', #38881, 1000.000000000000000 ) ;
#49550=CARTESIAN_POINT ( 'NONE',  ( -97.64999999960633659, -209.9999706968024782, 82.45844277047601167 ) ) ;
#49551=VECTOR ( 'NONE', #826, 1000.000000000000000 ) ;
#49552=CARTESIAN_POINT ( 'NONE',  ( -92.35000000000003695, 90.00000000000004263, 89.12687500173430521 ) ) ;
#49555=CARTESIAN_POINT ( 'NONE',  ( 96.32499999999998863, -212.2949673200287179, 81.40104166840096411 ) ) ;
#49556=CARTESIAN_POINT ( 'NONE',  ( 93.67499999999998295, 92.29496732002878900, 86.71916666666666629 ) ) ;
#49559=CARTESIAN_POINT ( 'NONE',  ( -92.75110981005065014, -210.5903413996856273, 74.79348190356849102 ) ) ;
#49562=CARTESIAN_POINT ( 'NONE',  ( -96.15314808468752972, 91.99731107132950569, 83.98072916753382344 ) ) ;
#49563=EDGE_CURVE ( 'NONE', #53104, #64725, #58670, .T. ) ;
#49564=CARTESIAN_POINT ( 'NONE',  ( 97.30629616937498838, 88.66845928578037217, 81.01739583420048518 ) ) ;
#49572=VERTEX_POINT ( 'NONE', #26290 ) ;
#49573=ADVANCED_FACE ( 'NONE', ( #49225 ), #72153, .F. ) ;
#49574=CARTESIAN_POINT ( 'NONE',  ( -93.67499999999998295, -207.7050326799711968, 80.97770833506763211 ) ) ;
#49575=CARTESIAN_POINT ( 'NONE',  ( 97.64999999999997726, 88.47002178664753558, 89.07395833506762983 ) ) ;
#49577=CARTESIAN_POINT ( 'NONE',  ( 95.00000000000000000, -209.9999999999999716, 90.00000000000000000 ) ) ;
#49578=CARTESIAN_POINT ( 'NONE',  ( -96.15314808468747287, -208.0026889286704943, 78.10697916753380809 ) ) ;
#49580=EDGE_CURVE ( 'NONE', #38969, #69628, #40447, .T. ) ;
#49582=CYLINDRICAL_SURFACE ( 'NONE', #46444, 26.50000000000000355 ) ;
#49589=CARTESIAN_POINT ( 'NONE',  ( 94.99999999999998579, 87.33691857156068750, 89.16656250086712987 ) ) ;
#49590=CARTESIAN_POINT ( 'NONE',  ( -2.500000000000015543, -73.00000000000001421, -258.2999999999999545 ) ) ;
#49592=CARTESIAN_POINT ( 'NONE',  ( -92.35000000000003695, 90.00000000000004263, 87.14249999999999829 ) ) ;
#49601=AXIS2_PLACEMENT_3D ( 'NONE', #45186, #68107, #106 ) ;
#49604=CARTESIAN_POINT ( 'NONE',  ( -94.99999999999997158, -213.0599564267049857, 83.17374999999999829 ) ) ;
#49611=EDGE_CURVE ( 'NONE', #36383, #30790, #16886, .T. ) ;
#49613=DIRECTION ( 'NONE',  ( -1.000000000000000000, -0.000000000000000000, -0.000000000000000000 ) ) ;
#49618=CARTESIAN_POINT ( 'NONE',  ( 92.69370383062501162, -208.6684592857803295, 80.69989583420046131 ) ) ;
#49619=CARTESIAN_POINT ( 'NONE',  ( 97.30629616937498838, -208.6684592857803295, 84.45697916753383083 ) ) ;
#49621=CARTESIAN_POINT ( 'NONE',  ( 96.15314808468750130, -211.9973110713294489, 84.93322916753382401 ) ) ;
#49625=ORIENTED_EDGE ( 'NONE', *, *, #34310, .F. ) ;
#49628=CARTESIAN_POINT ( 'NONE',  ( -95.00000000000002842, 92.66308142843932671, 78.21281250086717307 ) ) ;
#49634=CARTESIAN_POINT ( 'NONE',  ( 97.64999999999997726, -208.4700217866474645, 89.17979166840096639 ) ) ;
#49636=CARTESIAN_POINT ( 'NONE',  ( 94.99999999999998579, 90.00000000000002842, 90.00000000000000000 ) ) ;
#49639=( BOUNDED_CURVE ( )  B_SPLINE_CURVE ( 2, ( #15654, #32921, #21653, #68274, #16390, #67523, #44608, #61894, #62267 ),
 .UNSPECIFIED., .F., .F. ) 
 B_SPLINE_CURVE_WITH_KNOTS ( ( 3, 2, 2, 2, 3 ),
 ( 0.4445132602993024373, 0.4515689946186892123, 0.4586247601596063483, 0.4656805257005234844, 0.4656806970079900854 ),
 .UNSPECIFIED. ) 
 CURVE ( )  GEOMETRIC_REPRESENTATION_ITEM ( )  RATIONAL_B_SPLINE_CURVE ( ( 0.9999988143388863771, 0.8660259966176188096, 1.000000000000000000, 0.8660254037844387076, 1.000000000000000000, 0.8660254037844387076, 1.000000000000000000, 0.9999967472206192642, 0.9999934945991874047 ) ) 
 REPRESENTATION_ITEM ( '' )  );
#49643=ORIENTED_EDGE ( 'NONE', *, *, #13291, .F. ) ;
#49644=ORIENTED_EDGE ( 'NONE', *, *, #2417, .T. ) ;
#49647=CARTESIAN_POINT ( 'NONE',  ( 95.00000000000000000, -207.3369185715606307, 76.14906250086716000 ) ) ;
#49649=CARTESIAN_POINT ( 'NONE',  ( -2.499999999999965361, 90.00000000000000000, -310.0000000000000000 ) ) ;
#49650=ORIENTED_EDGE ( 'NONE', *, *, #45722, .T. ) ;
#49651=ORIENTED_EDGE ( 'NONE', *, *, #54481, .T. ) ;
#49652=ORIENTED_EDGE ( 'NONE', *, *, #55174, .T. ) ;
#49654=LINE ( 'NONE', #9074, #68330 ) ;
#49655=CARTESIAN_POINT ( 'NONE',  ( -94.53673242685063371, 87.15692181550789996, 74.72378867588408013 ) ) ;
#49660=CARTESIAN_POINT ( 'NONE',  ( 94.99999999999998579, 87.33691857156068750, 79.00656250086713328 ) ) ;
#49667=CARTESIAN_POINT ( 'NONE',  ( -96.15314808468745866, -211.9973110713294489, 78.95364583420047211 ) ) ;
#49670=CARTESIAN_POINT ( 'NONE',  ( 2.500000000000015987, -65.00000000000000000, -90.00000000000000000 ) ) ;
#49672=ORIENTED_EDGE ( 'NONE', *, *, #62121, .F. ) ;
#49673=ORIENTED_EDGE ( 'NONE', *, *, #19113, .T. ) ;
#49675=CARTESIAN_POINT ( 'NONE',  ( -93.67499999999998295, -212.2949673200287179, 88.94166666666666288 ) ) ;
#49677=CARTESIAN_POINT ( 'NONE',  ( -97.30629616937501680, 88.66845928578038638, 81.44072916753381719 ) ) ;
#49687=CARTESIAN_POINT ( 'NONE',  ( 97.64999999999999147, -209.9999999999999716, 88.49187500173430010 ) ) ;
#49688=CARTESIAN_POINT ( 'NONE',  ( -92.69370383062498320, -209.9999999999999716, 84.40406250086715545 ) ) ;
#49710=B_SPLINE_CURVE_WITH_KNOTS ( 'NONE', 3,
 ( #67183, #55534, #42773, #65706, #55902, #14186, #60443, #37139, #60083, #21296, #66813, #20194, #66090, #9288, #9666, #8561, #49146, #2950, #10031, #25841, #72071, #15682, #38616, #44254 ),
 .UNSPECIFIED., .F., .F.,
 ( 4, 2, 2, 2, 2, 2, 2, 2, 2, 2, 2, 4 ),
 ( -0.009991285186810239943, -0.009254074022779373160, -0.008516862858748506376, -0.007779651694717638725, -0.007411046112702206201, -0.007042440530686772809, -0.006673834948671339418, -0.006305229366655907761, -0.005568018202625041845, -0.004830807038594175928, -0.004462201456578743404, -0.004093595874563310012 ),
 .UNSPECIFIED. ) ;
#49716=EDGE_CURVE ( 'NONE', #71746, #48302, #65925, .T. ) ;
#49726=ORIENTED_EDGE ( 'NONE', *, *, #9534, .F. ) ;
#49727=CARTESIAN_POINT ( 'NONE',  ( 93.84685191531248449, 88.00268892867053694, 75.30239583420048177 ) ) ;
#49734=CARTESIAN_POINT ( 'NONE',  ( 96.15314808468748708, 88.00268892867053694, 88.58447916753381435 ) ) ;
#49737=CARTESIAN_POINT ( 'NONE',  ( 95.00000000000000000, -207.3369185715606307, 86.94406250086714749 ) ) ;
#49743=CARTESIAN_POINT ( 'NONE',  ( 97.64999999989933599, 90.00002309722570715, 83.41187580057898288 ) ) ;
#49746=CARTESIAN_POINT ( 'NONE',  ( -97.64999999999994884, -211.5299782133524502, 77.43229166840096411 ) ) ;
#49747=CARTESIAN_POINT ( 'NONE',  ( -97.30629616937501680, 88.66845928578038638, 89.21947916753381946 ) ) ;
#49749=ORIENTED_EDGE ( 'NONE', *, *, #22081, .T. ) ;
#49750=CARTESIAN_POINT ( 'NONE',  ( 97.30629616937498838, 90.00000000000002842, 88.69031250086715090 ) ) ;
#49751=CARTESIAN_POINT ( 'NONE',  ( -95.00000000000002842, 92.66308142843932671, 89.48406250086713953 ) ) ;
#49759=CARTESIAN_POINT ( 'NONE',  ( -96.15314808468747287, -208.0026889286704943, 89.53697916753381492 ) ) ;
#49769=CARTESIAN_POINT ( 'NONE',  ( -96.32500000000001705, 92.29496732002878900, 82.27416666666665890 ) ) ;
#49778=CARTESIAN_POINT ( 'NONE',  ( -92.69370383062502583, 91.33154071421968467, 81.75822916753381264 ) ) ;
#49784=CARTESIAN_POINT ( 'NONE',  ( -2.499999999999973355, 65.00000000000000000, -290.0000000000000568 ) ) ;
#49785=CARTESIAN_POINT ( 'NONE',  ( 93.67500000000001137, -207.7050326799711968, 80.44854166840097776 ) ) ;
#49786=DIRECTION ( 'NONE',  ( -0.000000000000000000, -0.000000000000000000, 1.000000000000000000 ) ) ;
#49789=CARTESIAN_POINT ( 'NONE',  ( 93.84685191531248449, 91.99731107132950569, 82.07572916753382231 ) ) ;
#49790=CARTESIAN_POINT ( 'NONE',  ( -92.69370383062498320, -209.9999999999999716, 81.86406250086714920 ) ) ;
#49794=CARTESIAN_POINT ( 'NONE',  ( -96.32499999999996021, -207.7050326799711968, 77.82916666666665151 ) ) ;
#49800=CARTESIAN_POINT ( 'NONE',  ( -93.84685191531252713, 88.00268892867056536, 76.67822916753381435 ) ) ;
#49801=CARTESIAN_POINT ( 'NONE',  ( 97.30629616937498838, -211.3315407142195852, 85.46239583420047836 ) ) ;
#49803=CARTESIAN_POINT ( 'NONE',  ( 97.01450244679210755, 88.86758821614978388, 74.79348190356853365 ) ) ;
#49809=CARTESIAN_POINT ( 'NONE',  ( 100.0010000000000190, -115.9999999999999716, -40.00000000000002132 ) ) ;
#49815=CARTESIAN_POINT ( 'NONE',  ( 97.30629616937498838, -209.9999999999999716, 75.51406250086715488 ) ) ;
#49818=CYLINDRICAL_SURFACE ( 'NONE', #61673, 2.649999999999985700 ) ;
#49819=CARTESIAN_POINT ( 'NONE',  ( 97.30629616937498838, 91.33154071421968467, 88.26697916753381890 ) ) ;
#49821=CARTESIAN_POINT ( 'NONE',  ( 93.67500000000001137, -212.2949673200287179, 80.58083333333331666 ) ) ;
#49822=VECTOR ( 'NONE', #66060, 1000.000000000000000 ) ;
#49833=CARTESIAN_POINT ( 'NONE',  ( -94.99999999999997158, -206.9400435732949575, 77.14124999999999943 ) ) ;
#49838=CARTESIAN_POINT ( 'NONE',  ( -94.99999999999997158, -206.9400435732949575, 85.47562500173431488 ) ) ;
#49844=CARTESIAN_POINT ( 'NONE',  ( -95.00000000000002842, 86.94004357329504273, 81.34812500173430294 ) ) ;
#49846=CARTESIAN_POINT ( 'NONE',  ( 92.69370383062498320, 91.33154071421968467, 82.12864583420048348 ) ) ;
#49847=DIRECTION ( 'NONE',  ( -0.000000000000000000, -0.000000000000000000, 1.000000000000000000 ) ) ;
#49860=CARTESIAN_POINT ( 'NONE',  ( -93.84685191531248449, -208.0026889286704943, 83.87489583420048689 ) ) ;
#49867=CARTESIAN_POINT ( 'NONE',  ( 92.34999999999998010, 90.00001272874952463, 81.82437456149077093 ) ) ;
#49868=CARTESIAN_POINT ( 'NONE',  ( 97.64999999997404245, -210.0000117261773198, 82.77687459617033028 ) ) ;
#49869=CARTESIAN_POINT ( 'NONE',  ( 93.84685191531248449, 88.00268892867053694, 78.95364583420047211 ) ) ;
#49871=CARTESIAN_POINT ( 'NONE',  ( 97.64999999999999147, 89.99999997928482287, 80.87187500099604165 ) ) ;
#49877=( BOUNDED_CURVE ( )  B_SPLINE_CURVE ( 2, ( #69104, #61983, #351, #710, #51426, #57821, #28872 ),
 .UNSPECIFIED., .F., .F. ) 
 B_SPLINE_CURVE_WITH_KNOTS ( ( 3, 2, 2, 3 ),
 ( 0.2708333333333337034, 0.2777777777777781232, 0.2847222222222224874, 0.2916666666666669072 ),
 .UNSPECIFIED. ) 
 CURVE ( )  GEOMETRIC_REPRESENTATION_ITEM ( )  RATIONAL_B_SPLINE_CURVE ( ( 0.9999999999999924505, 0.8660254037844462571, 1.000000000000000000, 0.8660254037844387076, 1.000000000000000000, 0.8660254037844343777, 1.000000000000004219 ) ) 
 REPRESENTATION_ITEM ( '' )  );
#49879=VECTOR ( 'NONE', #5783, 1000.000000000000000 ) ;
#49880=CARTESIAN_POINT ( 'NONE',  ( 93.67500000000001137, -212.2949673200287179, 78.67583333333332973 ) ) ;
#49881=CARTESIAN_POINT ( 'NONE',  ( -92.35000000000177067, -209.9999969335172807, 75.79187510780353421 ) ) ;
#49884=CARTESIAN_POINT ( 'NONE',  ( -93.84685191531254134, 91.99731107132950569, 84.35114583420048007 ) ) ;
#49892=DIRECTION ( 'NONE',  ( -0.000000000000000000, -0.000000000000000000, 1.000000000000000000 ) ) ;
#49897=CARTESIAN_POINT ( 'NONE',  ( 93.84685191531249870, -208.0026889286704943, 79.53572916753381605 ) ) ;
#49900=EDGE_CURVE ( 'NONE', #33622, #49572, #66087, .T. ) ;
#49902=CARTESIAN_POINT ( 'NONE',  ( -96.32499999999996021, -207.7050326799711968, 81.71854166840095957 ) ) ;
#49908=CARTESIAN_POINT ( 'NONE',  ( 92.69370383062501162, -208.6684592857803011, 75.14364583420049826 ) ) ;
#49919=CARTESIAN_POINT ( 'NONE',  ( -97.65000000000001990, 90.00000000000004263, 89.44437500173430067 ) ) ;
#49922=CARTESIAN_POINT ( 'NONE',  ( 92.35000000000002274, -211.5299782133524502, 78.70229166840096013 ) ) ;
#49923=CARTESIAN_POINT ( 'NONE',  ( 96.32499999999997442, 92.29496732002878900, 80.26333333333332121 ) ) ;
#49926=ORIENTED_EDGE ( 'NONE', *, *, #21617, .T. ) ;
#49927=CARTESIAN_POINT ( 'NONE',  ( -93.23660927304928236, -211.4937631030103944, 74.79348190356849102 ) ) ;
#49932=CARTESIAN_POINT ( 'NONE',  ( -96.15314808468752972, 91.99731107132950569, 85.88572916753381037 ) ) ;
#49933=CARTESIAN_POINT ( 'NONE',  ( 92.69370383062498320, 90.00000000000002842, 78.84781250086714977 ) ) ;
#49939=CARTESIAN_POINT ( 'NONE',  ( -96.15314808468747287, -208.0026889286704943, 81.91697916753381037 ) ) ;
#49941=AXIS2_PLACEMENT_3D ( 'NONE', #60913, #2705, #9404 ) ;
#49946=FACE_OUTER_BOUND ( 'NONE', #12696, .T. ) ;
#49948=CARTESIAN_POINT ( 'NONE',  ( -96.15314808468745866, -211.9973110713294489, 78.31864583420048120 ) ) ;
#49952=CARTESIAN_POINT ( 'NONE',  ( 97.64999999964362587, 89.99995654222556141, 89.12687334326064104 ) ) ;
#49955=CARTESIAN_POINT ( 'NONE',  ( -92.35000000000003695, 90.00000000000004263, 89.68250000000000455 ) ) ;
#49958=CARTESIAN_POINT ( 'NONE',  ( -94.99999999999997158, -213.0599564267049857, 85.71374999999999034 ) ) ;
#49965=CARTESIAN_POINT ( 'NONE',  ( -97.65000000000001990, 90.00000000000004263, 76.03000000000000114 ) ) ;
#49970=CARTESIAN_POINT ( 'NONE',  ( 97.64999999999999147, 90.00000000000002842, 75.00000000000000000 ) ) ;
#49973=CARTESIAN_POINT ( 'NONE',  ( -94.99999999999997158, -213.0599564267049857, 86.34874999999999545 ) ) ;
#49975=CARTESIAN_POINT ( 'NONE',  ( -94.99999999999997158, -209.9999999999999716, 90.00000000000000000 ) ) ;
#49983=CARTESIAN_POINT ( 'NONE',  ( 92.69370383062501162, -211.3315407142195852, 75.09072916753382287 ) ) ;
#49984=VECTOR ( 'NONE', #34560, 1000.000000000000000 ) ;
#49992=CARTESIAN_POINT ( 'NONE',  ( 95.00000000000000000, -212.6630814284392557, 77.10156250086711793 ) ) ;
#49993=CARTESIAN_POINT ( 'NONE',  ( 92.69370383062501162, -211.3315407142195852, 85.40947916753381719 ) ) ;
#49994=EDGE_LOOP ( 'NONE', ( #659, #59719, #22278, #9995, #47428 ) ) ;
#49995=CARTESIAN_POINT ( 'NONE',  ( 97.30629616937498838, -208.6684592857803011, 85.09197916753380753 ) ) ;
#49998=ORIENTED_EDGE ( 'NONE', *, *, #1333, .F. ) ;
#50004=CARTESIAN_POINT ( 'NONE',  ( 97.64999999999999147, -209.9999999999999716, 89.12687500173430521 ) ) ;
#50013=CARTESIAN_POINT ( 'NONE',  ( 96.15314808468748708, -208.0026889286704943, 74.82614583420047438 ) ) ;
#50022=CARTESIAN_POINT ( 'NONE',  ( -97.30629616937501680, 88.66845928578038638, 75.24947916753383481 ) ) ;
#50026=CARTESIAN_POINT ( 'NONE',  ( 97.30629616937498838, 88.66845928578037217, 76.57239583420046358 ) ) ;
#50029=CARTESIAN_POINT ( 'NONE',  ( -94.99999999999997158, -207.3369185715606307, 88.21406250086714351 ) ) ;
#50030=ORIENTED_EDGE ( 'NONE', *, *, #37215, .F. ) ;
#50034=CARTESIAN_POINT ( 'NONE',  ( -97.30629616937495996, -209.9999999999999716, 80.11781250086713158 ) ) ;
#50046=CARTESIAN_POINT ( 'NONE',  ( 93.55421244156880789, -208.0396902886532757, 74.86947676125079454 ) ) ;
#50047=CARTESIAN_POINT ( 'NONE',  ( -95.00000000000002842, 87.33691857156074434, 82.18156250086714465 ) ) ;
#50054=CARTESIAN_POINT ( 'NONE',  ( -97.64999999999996305, -209.9999999999999716, 89.44437500173430067 ) ) ;
#50057=CARTESIAN_POINT ( 'NONE',  ( -97.65000000000003411, 91.52997821335256390, 87.40708333333333258 ) ) ;
#50058=CARTESIAN_POINT ( 'NONE',  ( -94.99999999999997158, -212.6630814284392557, 79.16531250086715943 ) ) ;
#50059=CARTESIAN_POINT ( 'NONE',  ( -94.99999999999997158, -213.0599564267049857, 87.06312500173429214 ) ) ;
#50064=CARTESIAN_POINT ( 'NONE',  ( -95.00000000000002842, 86.94004357329504273, 80.71312500173429783 ) ) ;
#50066=VECTOR ( 'NONE', #12764, 1000.000000000000000 ) ;
#50072=DIRECTION ( 'NONE',  ( -0.000000000000000000, -0.000000000000000000, 1.000000000000000000 ) ) ;
#50078=( BOUNDED_CURVE ( )  B_SPLINE_CURVE ( 2, ( #66764, #15256, #46063, #12580, #17484, #23868, #603 ),
 .UNSPECIFIED., .F., .F. ) 
 B_SPLINE_CURVE_WITH_KNOTS ( ( 3, 2, 2, 3 ),
 ( 0.2916666666666669072, 0.2986111111111113270, 0.3055555555555557468, 0.3125000000000001665 ),
 .UNSPECIFIED. ) 
 CURVE ( )  GEOMETRIC_REPRESENTATION_ITEM ( )  RATIONAL_B_SPLINE_CURVE ( ( 0.9999999999999956701, 0.8660254037844430375, 1.000000000000000000, 0.8660254037844387076, 1.000000000000000000, 0.8660254037844354880, 1.000000000000003109 ) ) 
 REPRESENTATION_ITEM ( '' )  );
#50080=CARTESIAN_POINT ( 'NONE',  ( -93.67499999999998295, -207.7050326799711968, 87.32770833506762642 ) ) ;
#50094=CARTESIAN_POINT ( 'NONE',  ( 94.99999999999998579, 92.66308142843935514, 76.30781250086715772 ) ) ;
#50100=CARTESIAN_POINT ( 'NONE',  ( 92.69370383062498320, 88.66845928578037217, 89.06072916753379332 ) ) ;
#50102=CARTESIAN_POINT ( 'NONE',  ( 97.30629616937498838, -208.6684592857803011, 86.20322916753382003 ) ) ;
#50103=CARTESIAN_POINT ( 'NONE',  ( 94.99999999999998579, 90.00000000000002842, 90.00000000000000000 ) ) ;
#50107=CARTESIAN_POINT ( 'NONE',  ( -93.67499999999998295, -207.7050326799711968, 82.80333333333332746 ) ) ;
#50109=CARTESIAN_POINT ( 'NONE',  ( -97.30629616937497417, -211.3315407142195852, 88.42572916753380241 ) ) ;
#50110=CARTESIAN_POINT ( 'NONE',  ( -95.00000000000002842, 87.33691857156074434, 84.24531250086715772 ) ) ;
#50112=CARTESIAN_POINT ( 'NONE',  ( 97.30629616937498838, 88.66845928578037217, 86.73239583420047438 ) ) ;
#50113=CARTESIAN_POINT ( 'NONE',  ( -96.15314808468752972, 91.99731107132950569, 88.26697916753380468 ) ) ;
#50120=CARTESIAN_POINT ( 'NONE',  ( -92.69370383062498320, -208.6684592857803295, 89.37822916753378877 ) ) ;
#50126=ORIENTED_EDGE ( 'NONE', *, *, #41680, .T. ) ;
#50128=ORIENTED_EDGE ( 'NONE', *, *, #56665, .T. ) ;
#50131=CARTESIAN_POINT ( 'NONE',  ( -97.65000000000001990, 90.00000000000004263, 81.10999999999999943 ) ) ;
#50132=EDGE_CURVE ( 'NONE', #36714, #428, #50998, .T. ) ;
#50134=CARTESIAN_POINT ( 'NONE',  ( 97.65000000000000568, -211.5299782133524218, 75.73895833506765030 ) ) ;
#50138=CARTESIAN_POINT ( 'NONE',  ( -94.99999999999997158, -209.9999999999999716, 90.00000000000000000 ) ) ;
#50140=ORIENTED_EDGE ( 'NONE', *, *, #57784, .T. ) ;
#50141=CARTESIAN_POINT ( 'NONE',  ( -95.00000000000002842, 87.33691857156074434, 82.81656250086713555 ) ) ;
#50150=CARTESIAN_POINT ( 'NONE',  ( -94.99999999999997158, -207.3369185715606307, 88.37281250086715545 ) ) ;
#50157=CARTESIAN_POINT ( 'NONE',  ( 94.99999999999998579, 92.66308142843932671, 78.84781250086714977 ) ) ;
#50158=CARTESIAN_POINT ( 'NONE',  ( -94.99999999999997158, -212.6630814284392557, 82.97531250086714749 ) ) ;
#50161=CARTESIAN_POINT ( 'NONE',  ( 92.35000000052950497, -209.9999663481461027, 81.18829462297289012 ) ) ;
#50162=CARTESIAN_POINT ( 'NONE',  ( -97.64999999999994884, -208.4700217866474645, 76.61208333333333087 ) ) ;
#50164=CARTESIAN_POINT ( 'NONE',  ( -92.69370383062505425, 88.66845928578038638, 79.90614583420048689 ) ) ;
#50165=CARTESIAN_POINT ( 'NONE',  ( 96.15314808468748708, -208.0026889286704943, 81.81114583420047381 ) ) ;
#50169=VERTEX_POINT ( 'NONE', #57020 ) ;
#50181=CARTESIAN_POINT ( 'NONE',  ( 96.15314808468750130, -211.9973110713294489, 76.67822916753381435 ) ) ;
#50185=CARTESIAN_POINT ( 'NONE',  ( 94.99999999999998579, 87.33691857156068750, 86.78531250086716398 ) ) ;
#50187=CARTESIAN_POINT ( 'NONE',  ( 92.35000000000002274, -211.5299782133524502, 76.71791666666666742 ) ) ;
#50198=CARTESIAN_POINT ( 'NONE',  ( 2.500000000000015987, 65.00000000000000000, -290.0000000000000568 ) ) ;
#50200=FACE_OUTER_BOUND ( 'NONE', #70234, .T. ) ;
#50203=CARTESIAN_POINT ( 'NONE',  ( -96.32499999999996021, -212.2949673200287179, 83.20020833506764291 ) ) ;
#50205=CARTESIAN_POINT ( 'NONE',  ( -97.30629616937501680, 90.00000000000004263, 89.64281250086713726 ) ) ;
#50207=CARTESIAN_POINT ( 'NONE',  ( 96.32499999999998863, 87.70503267997126784, 81.40104166840096411 ) ) ;
#50208=CARTESIAN_POINT ( 'NONE',  ( -92.35000000000005116, 91.52997821335253548, 81.55979166840097605 ) ) ;
#50210=ORIENTED_EDGE ( 'NONE', *, *, #43581, .F. ) ;
#50211=CARTESIAN_POINT ( 'NONE',  ( 92.69370383062498320, 90.00000000000002842, 84.08656250086716000 ) ) ;
#50213=CARTESIAN_POINT ( 'NONE',  ( -97.64995850909681963, 88.46999783186339528, 85.68729332542761767 ) ) ;
#50224=VERTEX_POINT ( 'NONE', #10403 ) ;
#50228=CARTESIAN_POINT ( 'NONE',  ( -97.64999999978466860, 90.00002100773832581, 79.91868729552945183 ) ) ;
#50231=CARTESIAN_POINT ( 'NONE',  ( -96.15314808468747287, -208.0026889286704943, 79.53572916753381605 ) ) ;
#50232=VERTEX_POINT ( 'NONE', #18262 ) ;
#50234=CARTESIAN_POINT ( 'NONE',  ( 96.32499999999998863, -212.2949673200287179, 81.32166666666667254 ) ) ;
#50239=CARTESIAN_POINT ( 'NONE',  ( -92.34999999999999432, -211.5299782133524218, 77.64395833506762301 ) ) ;
#50241=CARTESIAN_POINT ( 'NONE',  ( 93.84685191531248449, 91.99731107132950569, 77.47197916753380298 ) ) ;
#50248=CARTESIAN_POINT ( 'NONE',  ( 97.64999999999999147, -209.9999999999999716, 84.60249999999999204 ) ) ;
#50249=CARTESIAN_POINT ( 'NONE',  ( 96.32499999999998863, -212.2949673200287179, 83.22666666666665947 ) ) ;
#50252=CARTESIAN_POINT ( 'NONE',  ( -97.64999999960633659, -209.9999706968024782, 82.45844277047601167 ) ) ;
#50254=VERTEX_POINT ( 'NONE', #52854 ) ;
#50255=CARTESIAN_POINT ( 'NONE',  ( -96.15314808468752972, 91.99731107132950569, 82.55197916753380127 ) ) ;
#50257=EDGE_CURVE ( 'NONE', #11086, #20441, #41562, .T. ) ;
#50270=CARTESIAN_POINT ( 'NONE',  ( 92.69370383062501162, -209.9999999999999716, 77.10156250086714635 ) ) ;
#50272=ORIENTED_EDGE ( 'NONE', *, *, #12235, .T. ) ;
#50274=CARTESIAN_POINT ( 'NONE',  ( 96.92110976540175216, -208.6943671794273030, 74.79348190356853365 ) ) ;
#50276=CARTESIAN_POINT ( 'NONE',  ( -97.64999999947052345, 90.00003365185393989, 81.18829462297244959 ) ) ;
#50278=VECTOR ( 'NONE', #26071, 1000.000000000000000 ) ;
#50280=CARTESIAN_POINT ( 'NONE',  ( 97.64999999999997726, -208.4700217866474645, 89.73541666666666572 ) ) ;
#50282=AXIS2_PLACEMENT_3D ( 'NONE', #62406, #27038, #31942 ) ;
#50293=CARTESIAN_POINT ( 'NONE',  ( 93.67500000000001137, -207.7050326799711968, 78.54354166840096241 ) ) ;
#50294=CARTESIAN_POINT ( 'NONE',  ( 97.64999999999997726, 91.52997821335252127, 82.75041666666665208 ) ) ;
#50297=ORIENTED_EDGE ( 'NONE', *, *, #48237, .T. ) ;
#50300=CARTESIAN_POINT ( 'NONE',  ( -93.84685191531252713, 88.00268892867056536, 85.56822916753381492 ) ) ;
#50301=CARTESIAN_POINT ( 'NONE',  ( 93.84685191531248449, 91.99731107132950569, 79.37697916753380412 ) ) ;
#50313=CARTESIAN_POINT ( 'NONE',  ( -94.99999999999997158, -212.6630814284392557, 80.91156250086714863 ) ) ;
#50324=CARTESIAN_POINT ( 'NONE',  ( 92.34999999999999432, 90.00000000000002842, 88.17437500173430465 ) ) ;
#50326=( BOUNDED_CURVE ( )  B_SPLINE_CURVE ( 2, ( #2542, #55097, #59636, #14121, #24677, #70900, #25426 ),
 .UNSPECIFIED., .F., .F. ) 
 B_SPLINE_CURVE_WITH_KNOTS ( ( 3, 2, 2, 3 ),
 ( 0.6041666666666670737, 0.6111111111111116045, 0.6180555555555559133, 0.6250000000000003331 ),
 .UNSPECIFIED. ) 
 CURVE ( )  GEOMETRIC_REPRESENTATION_ITEM ( )  RATIONAL_B_SPLINE_CURVE ( ( 0.9999999999999914513, 0.8660254037844472563, 1.000000000000000000, 0.8660254037844387076, 1.000000000000000000, 0.8660254037844322683, 1.000000000000006439 ) ) 
 REPRESENTATION_ITEM ( '' )  );
#50327=CARTESIAN_POINT ( 'NONE',  ( -97.30629616937497417, -211.3315407142195852, 75.09072916753382287 ) ) ;
#50331=DIRECTION ( 'NONE',  ( 1.000000000000000000, 0.000000000000000000, 0.000000000000000000 ) ) ;
#50337=CARTESIAN_POINT ( 'NONE',  ( 94.99999999999998579, 86.94004357329502852, 81.34812500173430294 ) ) ;
#50342=CARTESIAN_POINT ( 'NONE',  ( 93.67499999999999716, 87.70503267997126784, 77.40583333333331950 ) ) ;
#50347=AXIS2_PLACEMENT_3D ( 'NONE', #70968, #71704, #59336 ) ;
#50354=CARTESIAN_POINT ( 'NONE',  ( -92.34999999999999432, -209.9999999999999716, 84.60249999999999204 ) ) ;
#50364=CARTESIAN_POINT ( 'NONE',  ( 93.84685191531251292, -211.9973110713294489, 88.63739583420048973 ) ) ;
#50365=ORIENTED_EDGE ( 'NONE', *, *, #23544, .T. ) ;
#50369=DIRECTION ( 'NONE',  ( -0.000000000000000000, -0.000000000000000000, -1.000000000000000000 ) ) ;
#50372=CARTESIAN_POINT ( 'NONE',  ( 96.15314808468748708, -208.0026889286704943, 77.36614583420046642 ) ) ;
#50373=ORIENTED_EDGE ( 'NONE', *, *, #47963, .F. ) ;
#50374=CARTESIAN_POINT ( 'NONE',  ( 95.00000000000000000, -212.6630814284392557, 83.61031250086716682 ) ) ;
#50377=CARTESIAN_POINT ( 'NONE',  ( 2.500000000000034639, 90.00000000000000000, -90.00000000000000000 ) ) ;
#50382=CARTESIAN_POINT ( 'NONE',  ( 95.00000000000000000, -206.9400435732949575, 88.65062500173431204 ) ) ;
#50385=ORIENTED_EDGE ( 'NONE', *, *, #2441, .T. ) ;
#50387=CONICAL_SURFACE ( 'NONE', #26352, 2.649999999999999467, 1.029744258676654312 ) ;
#50394=ORIENTED_EDGE ( 'NONE', *, *, #43127, .F. ) ;
#50395=CARTESIAN_POINT ( 'NONE',  ( 92.69370383062501162, -211.3315407142195852, 76.36072916753381890 ) ) ;
#50404=ADVANCED_FACE ( 'NONE', ( #51740 ), #40456, .F. ) ;
#50405=CARTESIAN_POINT ( 'NONE',  ( -92.35000000000005116, 88.47002178664754979, 89.62958333333332916 ) ) ;
#50407=CARTESIAN_POINT ( 'NONE',  ( 92.69370383062498320, 91.33154071421968467, 78.15989583420048348 ) ) ;
#50410=CARTESIAN_POINT ( 'NONE',  ( -94.99999999999997158, -207.3369185715606307, 88.84906250086713442 ) ) ;
#50415=FACE_OUTER_BOUND ( 'NONE', #67776, .T. ) ;
#50416=CARTESIAN_POINT ( 'NONE',  ( -92.69370383062498320, -208.6684592857803295, 78.58322916753381548 ) ) ;
#50433=CARTESIAN_POINT ( 'NONE',  ( -95.00000000000002842, 87.33691857156074434, 80.27656250086714351 ) ) ;
#50443=CARTESIAN_POINT ( 'NONE',  ( 97.65000000000000568, -208.4700217866474645, 88.54479166840097548 ) ) ;
#50444=CARTESIAN_POINT ( 'NONE',  ( -93.84685191531247028, -211.9973110713294489, 77.94822916753382458 ) ) ;
#50462=CARTESIAN_POINT ( 'NONE',  ( 95.00000000000000000, -207.3369185715606307, 87.57906250086713840 ) ) ;
#50463=CARTESIAN_POINT ( 'NONE',  ( 92.34999999999992326, -208.4700217866474929, 86.13708333333332234 ) ) ;
#50472=FACE_OUTER_BOUND ( 'NONE', #73873, .T. ) ;
#50477=ORIENTED_EDGE ( 'NONE', *, *, #32771, .F. ) ;
#50480=ORIENTED_EDGE ( 'NONE', *, *, #9020, .T. ) ;
#50482=CARTESIAN_POINT ( 'NONE',  ( 97.30629616937498838, 88.66845928578037217, 77.36614583420048064 ) ) ;
#50486=ADVANCED_FACE ( 'NONE', ( #13359 ), #60721, .F. ) ;
#50489=CARTESIAN_POINT ( 'NONE',  ( 93.84685191531248449, 88.00268892867053694, 87.84364583420047268 ) ) ;
#50491=CARTESIAN_POINT ( 'NONE',  ( 97.30629616937498838, -209.9999999999999716, 84.88031250086713442 ) ) ;
#50498=CARTESIAN_POINT ( 'NONE',  ( -92.69370383062498320, -208.6684592857803011, 87.47322916753381605 ) ) ;
#50499=CARTESIAN_POINT ( 'NONE',  ( -95.00000000000002842, 92.66308142843932671, 85.83281250086714920 ) ) ;
#50501=CARTESIAN_POINT ( 'NONE',  ( 92.69370383062498320, 88.66845928578037217, 86.52072916753381548 ) ) ;
#50502=CARTESIAN_POINT ( 'NONE',  ( -93.84685191531252713, 88.00268892867056536, 85.40947916753380298 ) ) ;
#50506=CARTESIAN_POINT ( 'NONE',  ( -97.64999999999996305, -211.5299782133524218, 80.60729166840097548 ) ) ;
#50510=CARTESIAN_POINT ( 'NONE',  ( 92.35000000000000853, -208.4700217866474645, 82.32708333333334849 ) ) ;
#50513=CIRCLE ( 'NONE', #49324, 2.649999999999985700 ) ;
#50516=CARTESIAN_POINT ( 'NONE',  ( -92.35000000000005116, 88.47002178664754979, 80.73958333333332860 ) ) ;
#50518=DIRECTION ( 'NONE',  ( 0.000000000000000000, 0.000000000000000000, -1.000000000000000000 ) ) ;
#50520=CARTESIAN_POINT ( 'NONE',  ( -93.67500000000003979, 87.70503267997129626, 78.78166666666666629 ) ) ;
#50524=LINE ( 'NONE', #27961, #8497 ) ;
#50528=ORIENTED_EDGE ( 'NONE', *, *, #21034, .F. ) ;
#50529=CARTESIAN_POINT ( 'NONE',  ( -97.30629616937501680, 88.66845928578038638, 83.34572916753380412 ) ) ;
#50532=CARTESIAN_POINT ( 'NONE',  ( 95.00000000000000000, -209.9999999999999716, 90.00000000000000000 ) ) ;
#50536=CARTESIAN_POINT ( 'NONE',  ( 92.35000000000000853, -209.9999999999999716, 90.00000000000000000 ) ) ;
#50539=( BOUNDED_CURVE ( )  B_SPLINE_CURVE ( 2, ( #46260, #41717, #24430, #7876, #37202, #42471, #25535 ),
 .UNSPECIFIED., .F., .F. ) 
 B_SPLINE_CURVE_WITH_KNOTS ( ( 3, 2, 2, 3 ),
 ( 0.2499999999999995837, 0.2569444444444442532, 0.2638888888888890061, 0.2708333333333337034 ),
 .UNSPECIFIED. ) 
 CURVE ( )  GEOMETRIC_REPRESENTATION_ITEM ( )  RATIONAL_B_SPLINE_CURVE ( ( 1.000000000000007994, 0.8660254037844307140, 1.000000000000000000, 0.8660254037844387076, 1.000000000000000000, 0.8660254037844311581, 1.000000000000007550 ) ) 
 REPRESENTATION_ITEM ( '' )  );
#50540=CARTESIAN_POINT ( 'NONE',  ( 92.69370383062498320, 90.00000000000002842, 81.54656250086715374 ) ) ;
#50541=CARTESIAN_POINT ( 'NONE',  ( -92.69370383062498320, -209.9999999999999716, 81.22906250086715829 ) ) ;
#50542=CARTESIAN_POINT ( 'NONE',  ( -92.35000000000005116, 91.52997821335253548, 84.73479166840094479 ) ) ;
#50546=CARTESIAN_POINT ( 'NONE',  ( 92.34999999999999432, 90.00000000000002842, 85.63437500173431260 ) ) ;
#50547=CARTESIAN_POINT ( 'NONE',  ( -95.00000000000002842, 87.33691857156074434, 79.16531250086715943 ) ) ;
#50548=CARTESIAN_POINT ( 'NONE',  ( 95.00000000000000000, -207.3369185715606307, 80.59406250086715318 ) ) ;
#50549=ORIENTED_EDGE ( 'NONE', *, *, #30732, .F. ) ;
#50551=ORIENTED_EDGE ( 'NONE', *, *, #33273, .F. ) ;
#50559=EDGE_LOOP ( 'NONE', ( #27902, #29310, #73853, #33267 ) ) ;
#50566=CARTESIAN_POINT ( 'NONE',  ( 94.99999999999998579, 87.33691857156068750, 85.51531250086713953 ) ) ;
#50568=CARTESIAN_POINT ( 'NONE',  ( 92.35000000000000853, -209.9999999999999716, 77.93499999999998806 ) ) ;
#50571=ORIENTED_EDGE ( 'NONE', *, *, #70274, .F. ) ;
#50574=DIRECTION ( 'NONE',  ( 1.000000000000000000, 0.000000000000000000, 0.000000000000000000 ) ) ;
#50578=CYLINDRICAL_SURFACE ( 'NONE', #55625, 2.649999999999985700 ) ;
#50580=CARTESIAN_POINT ( 'NONE',  ( 95.00000000000000000, -209.9999999999999716, 90.00000000000000000 ) ) ;
#50581=CARTESIAN_POINT ( 'NONE',  ( 94.99999999999998579, 90.00000000000002842, 90.00000000000000000 ) ) ;
#50582=CARTESIAN_POINT ( 'NONE',  ( -96.32499999999996021, -212.2949673200287179, 83.83520833506763381 ) ) ;
#50584=CARTESIAN_POINT ( 'NONE',  ( -94.99999999999997158, -206.9400435732949575, 83.57062500173429953 ) ) ;
#50588=CARTESIAN_POINT ( 'NONE',  ( 97.64999999999999147, 90.00000000000002842, 83.41187500173430180 ) ) ;
#50589=CARTESIAN_POINT ( 'NONE',  ( -97.65000000000001990, 91.52997821335253548, 83.67645833506762187 ) ) ;
#50592=CARTESIAN_POINT ( 'NONE',  ( 97.30629616937498838, 88.66845928578037217, 82.44614583420049314 ) ) ;
#50593=EDGE_CURVE ( 'NONE', #9802, #14986, #40013, .T. ) ;
#50597=CARTESIAN_POINT ( 'NONE',  ( 92.34999999999999432, 90.00000000000002842, 88.09499999999999886 ) ) ;
#50600=CARTESIAN_POINT ( 'NONE',  ( -93.67500000000003979, 87.70503267997129626, 82.67104166840096013 ) ) ;
#50601=LINE ( 'NONE', #34804, #43200 ) ;
#50608=CARTESIAN_POINT ( 'NONE',  ( -92.35000000000003695, 89.99999990163421160, 80.23687499810812085 ) ) ;
#50609=CARTESIAN_POINT ( 'NONE',  ( -93.84685191531247028, -211.9973110713294489, 81.12322916753382174 ) ) ;
#50611=CARTESIAN_POINT ( 'NONE',  ( -95.00000000000002842, 87.33691857156074434, 88.53156250086713897 ) ) ;
#50612=VERTEX_POINT ( 'NONE', #56571 ) ;
#50626=CARTESIAN_POINT ( 'NONE',  ( 92.35001655588493463, -208.4700122281028598, 79.23145767387347860 ) ) ;
#50627=DIRECTION ( 'NONE',  ( 0.000000000000000000, 0.000000000000000000, -1.000000000000000000 ) ) ;
#50629=DIRECTION ( 'NONE',  ( -1.000000000000000000, -0.000000000000000000, -0.000000000000000000 ) ) ;
#50630=ORIENTED_EDGE ( 'NONE', *, *, #26377, .F. ) ;
#50632=CARTESIAN_POINT ( 'NONE',  ( -96.15314808468752972, 91.99731107132950569, 79.37697916753380412 ) ) ;
#50643=CARTESIAN_POINT ( 'NONE',  ( -96.32499999999996021, -207.7050326799711968, 84.81416666666666515 ) ) ;
#50644=CARTESIAN_POINT ( 'NONE',  ( 95.00000000000000000, -212.6630814284392557, 75.99031250086716227 ) ) ;
#50647=EDGE_CURVE ( 'NONE', #769, #56779, #61833, .T. ) ;
#50652=CARTESIAN_POINT ( 'NONE',  ( -93.67499999999998295, -207.7050326799711968, 85.42270833506762528 ) ) ;
#50655=CARTESIAN_POINT ( 'NONE',  ( 96.32499999999998863, -212.2949673200287179, 87.03666666666666174 ) ) ;
#50656=EDGE_CURVE ( 'NONE', #32383, #64543, #21965, .T. ) ;
#50665=VERTEX_POINT ( 'NONE', #44915 ) ;
#50666=CARTESIAN_POINT ( 'NONE',  ( 92.34999999999999432, 88.47002178664753558, 87.51291666666666913 ) ) ;
#50667=CARTESIAN_POINT ( 'NONE',  ( 96.32499999999998863, -207.7050326799711968, 80.97770833506763211 ) ) ;
#50668=CARTESIAN_POINT ( 'NONE',  ( 97.64999999999999147, 90.00000000000002842, 81.42749999999999488 ) ) ;
#50669=ORIENTED_EDGE ( 'NONE', *, *, #29840, .F. ) ;
#50672=VERTEX_POINT ( 'NONE', #73459 ) ;
#50676=CARTESIAN_POINT ( 'NONE',  ( 92.34999999999999432, 89.99997747860817299, 84.36437578067153709 ) ) ;
#50678=CARTESIAN_POINT ( 'NONE',  ( -93.84685191531252713, 88.00268892867056536, 83.66322916753382799 ) ) ;
#50679=CARTESIAN_POINT ( 'NONE',  ( 92.69370383062498320, 88.66845928578037217, 78.26572916753380582 ) ) ;
#50683=CARTESIAN_POINT ( 'NONE',  ( -94.99999999999997158, -209.9999999999999716, 90.00000000000000000 ) ) ;
#50684=CARTESIAN_POINT ( 'NONE',  ( 93.67499999999999716, 87.70503267997126784, 88.91520833506763211 ) ) ;
#50685=FACE_OUTER_BOUND ( 'NONE', #31429, .T. ) ;
#50691=CARTESIAN_POINT ( 'NONE',  ( -92.69370383062498320, -208.6684592857803011, 76.67822916753378593 ) ) ;
#50694=PLANE ( 'NONE',  #67329 ) ;
#50698=CARTESIAN_POINT ( 'NONE',  ( -97.65000000000003411, -211.5299782133524502, 77.98791666666667766 ) ) ;
#50700=CARTESIAN_POINT ( 'NONE',  ( -93.33922900947476364, -211.6002630214759961, 74.64190534806809296 ) ) ;
#50702=CARTESIAN_POINT ( 'NONE',  ( 96.32499999999997442, 92.29496732002878900, 88.59770833506763665 ) ) ;
#50704=LINE ( 'NONE', #5241, #44141 ) ;
#50708=CARTESIAN_POINT ( 'NONE',  ( 93.67500000000001137, -207.7050326799711968, 86.16354166840096696 ) ) ;
#50709=CARTESIAN_POINT ( 'NONE',  ( 97.30629616937498838, 88.66845928578035796, 83.55739583420047722 ) ) ;
#50712=CARTESIAN_POINT ( 'NONE',  ( 92.34999999999998010, -208.4700217866475498, 86.77208333333334167 ) ) ;
#50715=CARTESIAN_POINT ( 'NONE',  ( -97.65000000000001990, 90.00000000000004263, 84.36437500173430237 ) ) ;
#50720=CARTESIAN_POINT ( 'NONE',  ( -92.69370383062505425, 91.33154071421968467, 88.74322916753382628 ) ) ;
#50722=AXIS2_PLACEMENT_3D ( 'NONE', #30946, #47877, #23842 ) ;
#50723=CARTESIAN_POINT ( 'NONE',  ( -92.34999999999999432, -208.4700217866474645, 85.92541666666664923 ) ) ;
#50734=CARTESIAN_POINT ( 'NONE',  ( 96.15314808468748708, -208.0026889286704943, 85.77989583420048803 ) ) ;
#50735=EDGE_CURVE ( 'NONE', #41314, #36799, #68783, .T. ) ;
#50743=CARTESIAN_POINT ( 'NONE',  ( 96.15314808468750130, -211.9973110713294489, 77.15447916753380753 ) ) ;
#50745=CARTESIAN_POINT ( 'NONE',  ( 92.69370383062501162, -208.6684592857803011, 83.39864583420050792 ) ) ;
#50746=VERTEX_POINT ( 'NONE', #30190 ) ;
#50750=CARTESIAN_POINT ( 'NONE',  ( -95.00000000000002842, 92.66308142843932671, 75.03781250086714749 ) ) ;
#50752=LINE ( 'NONE', #16931, #11242 ) ;
#50759=ORIENTED_EDGE ( 'NONE', *, *, #56807, .T. ) ;
#50760=( BOUNDED_CURVE ( )  B_SPLINE_CURVE ( 2, ( #66076, #31462, #14545, #66797, #72056, #2576, #20177 ),
 .UNSPECIFIED., .F., .F. ) 
 B_SPLINE_CURVE_WITH_KNOTS ( ( 3, 2, 2, 3 ),
 ( 0.4374999999999994449, 0.4444444444444441422, 0.4513888888888888951, 0.4583333333333335924 ),
 .UNSPECIFIED. ) 
 CURVE ( )  GEOMETRIC_REPRESENTATION_ITEM ( )  RATIONAL_B_SPLINE_CURVE ( ( 1.000000000000010658, 0.8660254037844280495, 1.000000000000000000, 0.8660254037844387076, 1.000000000000000000, 0.8660254037844333785, 1.000000000000005329 ) ) 
 REPRESENTATION_ITEM ( '' )  );
#50764=ORIENTED_EDGE ( 'NONE', *, *, #44469, .T. ) ;
#50765=ORIENTED_EDGE ( 'NONE', *, *, #46028, .F. ) ;
#50766=CARTESIAN_POINT ( 'NONE',  ( 92.69370383062501162, -209.9999999999999716, 76.30781250086714351 ) ) ;
#50775=CARTESIAN_POINT ( 'NONE',  ( -95.00000000000002842, 92.66308142843932671, 76.94281250086714863 ) ) ;
#50781=CARTESIAN_POINT ( 'NONE',  ( -97.30629616937495996, -209.9999999999999716, 87.73781250086713612 ) ) ;
#50783=CARTESIAN_POINT ( 'NONE',  ( -92.34999999999999432, -209.9999999999999716, 75.71250000000000568 ) ) ;
#50786=CARTESIAN_POINT ( 'NONE',  ( -94.99999999999997158, -207.3369185715606307, 78.05406250086714692 ) ) ;
#50787=CARTESIAN_POINT ( 'NONE',  ( 97.64999999999690772, -210.0000040461968638, 77.06187486178042434 ) ) ;
#50794=CARTESIAN_POINT ( 'NONE',  ( -95.00000000000002842, 93.05995642670504253, 76.50624999999999432 ) ) ;
#50795=CARTESIAN_POINT ( 'NONE',  ( 92.80789733908686401, -208.8322938842642031, 74.89296886168679634 ) ) ;
#50796=CARTESIAN_POINT ( 'NONE',  ( -93.84685191531252713, 88.00268892867056536, 82.23447916753380582 ) ) ;
#50806=CARTESIAN_POINT ( 'NONE',  ( -94.99999999999997158, -212.6630814284392557, 77.89531250086714920 ) ) ;
#50807=CARTESIAN_POINT ( 'NONE',  ( -92.35000000000003695, 90.00000000000004263, 81.42749999999999488 ) ) ;
#50811=DIRECTION ( 'NONE',  ( -0.000000000000000000, -0.000000000000000000, 1.000000000000000000 ) ) ;
#50812=CARTESIAN_POINT ( 'NONE',  ( -97.65000000000001990, 88.47002178664754979, 80.60729166840097548 ) ) ;
#50814=ORIENTED_EDGE ( 'NONE', *, *, #72549, .T. ) ;
#50816=CARTESIAN_POINT ( 'NONE',  ( 97.65000000000000568, 91.52997821335252127, 77.11479166840095445 ) ) ;
#50817=CYLINDRICAL_SURFACE ( 'NONE', #40276, 2.649999999999999467 ) ;
#50825=DIRECTION ( 'NONE',  ( -0.000000000000000000, -0.000000000000000000, 1.000000000000000000 ) ) ;
#50826=ORIENTED_EDGE ( 'NONE', *, *, #12207, .T. ) ;
#50827=VECTOR ( 'NONE', #43097, 1000.000000000000000 ) ;
#50838=AXIS2_PLACEMENT_3D ( 'NONE', #54878, #48862, #66900 ) ;
#50842=ORIENTED_EDGE ( 'NONE', *, *, #51256, .F. ) ;
#50849=CARTESIAN_POINT ( 'NONE',  ( 96.32499999999997442, 92.29496732002878900, 87.24833333333333485 ) ) ;
#50856=CARTESIAN_POINT ( 'NONE',  ( 96.15314808468748708, 91.99731107132950569, 89.43114583420047836 ) ) ;
#50858=CARTESIAN_POINT ( 'NONE',  ( 97.30629616937498838, -209.9999999999999716, 86.78531250086714977 ) ) ;
#50862=DIRECTION ( 'NONE',  ( -0.000000000000000000, -0.000000000000000000, 1.000000000000000000 ) ) ;
#50866=CARTESIAN_POINT ( 'NONE',  ( -96.32499999999996021, -207.7050326799711968, 82.90916666666666401 ) ) ;
#50868=CARTESIAN_POINT ( 'NONE',  ( -97.30629616937495996, -209.9999999999999716, 86.46781250086714010 ) ) ;
#50869=CARTESIAN_POINT ( 'NONE',  ( -95.00000000000002842, 87.33691857156074434, 86.15031250086714465 ) ) ;
#50872=CARTESIAN_POINT ( 'NONE',  ( 97.30629616937498838, 91.33154071421968467, 84.29822916753380468 ) ) ;
#50873=CARTESIAN_POINT ( 'NONE',  ( -96.15314808468751551, 88.00268892867056536, 85.93864583420048575 ) ) ;
#50876=CYLINDRICAL_SURFACE ( 'NONE', #38547, 2.649999999999985700 ) ;
#50877=CYLINDRICAL_SURFACE ( 'NONE', #5566, 2.649999999999985700 ) ;
#50879=CARTESIAN_POINT ( 'NONE',  ( -97.30629616937497417, -208.6684592857803295, 89.58989583420047609 ) ) ;
#50880=AXIS2_PLACEMENT_3D ( 'NONE', #25669, #71517, #53136 ) ;
#50883=CARTESIAN_POINT ( 'NONE',  ( -97.65000000000001990, 90.00000000000004263, 90.00000000000000000 ) ) ;
#50886=VERTEX_POINT ( 'NONE', #2414 ) ;
#50889=CARTESIAN_POINT ( 'NONE',  ( -92.35000000000003695, 90.00000000000004263, 80.15749999999999886 ) ) ;
#50899=CARTESIAN_POINT ( 'NONE',  ( -97.30629616937501680, 91.33154071421968467, 78.79489583420047438 ) ) ;
#50900=CARTESIAN_POINT ( 'NONE',  ( 97.64999999999999147, 90.00000000000002842, 90.00000000000000000 ) ) ;
#50907=CARTESIAN_POINT ( 'NONE',  ( -94.99999999999997158, -212.6630814284392557, 88.69031250086716511 ) ) ;
#50910=EDGE_CURVE ( 'NONE', #51295, #45415, #32736, .T. ) ;
#50911=CARTESIAN_POINT ( 'NONE',  ( 94.99999999999998579, 87.33691857156068750, 78.53031250086715431 ) ) ;
#50914=CARTESIAN_POINT ( 'NONE',  ( -93.84685191531248449, -208.0026889286704943, 81.33489583420049485 ) ) ;
#50921=CARTESIAN_POINT ( 'NONE',  ( -95.00000000000002842, 92.66308142843932671, 78.21281250086717307 ) ) ;
#50922=CARTESIAN_POINT ( 'NONE',  ( 92.69370383062501162, -209.9999999999999716, 80.11781250086713158 ) ) ;
#50926=ORIENTED_EDGE ( 'NONE', *, *, #29715, .F. ) ;
#50927=ADVANCED_FACE ( 'NONE', ( #2778 ), #14002, .F. ) ;
#50937=EDGE_CURVE ( 'NONE', #22009, #17976, #19790, .T. ) ;
#50942=CARTESIAN_POINT ( 'NONE',  ( 92.35000000003290666, -209.9999916046337205, 84.99910573348564924 ) ) ;
#50943=CARTESIAN_POINT ( 'NONE',  ( 94.99999999999998579, 92.66308142843935514, 85.19781250086714408 ) ) ;
#50946=CARTESIAN_POINT ( 'NONE',  ( 97.64999999999997726, -208.4700217866474645, 78.30541666666668732 ) ) ;
#50949=ORIENTED_EDGE ( 'NONE', *, *, #34143, .F. ) ;
#50950=VECTOR ( 'NONE', #57210, 1000.000000000000000 ) ;
#50951=ORIENTED_EDGE ( 'NONE', *, *, #43256, .T. ) ;
#50960=CYLINDRICAL_SURFACE ( 'NONE', #29570, 2.649999999999985700 ) ;
#50962=CARTESIAN_POINT ( 'NONE',  ( -97.64999999999994884, -211.5299782133524502, 82.51229166840094820 ) ) ;
#50963=VERTEX_POINT ( 'NONE', #1671 ) ;
#50967=CARTESIAN_POINT ( 'NONE',  ( 92.34999999999999432, 90.00000000000002842, 81.82437500173429612 ) ) ;
#50968=CARTESIAN_POINT ( 'NONE',  ( -97.65000000000001990, 90.00000000000004263, 78.01437500173430806 ) ) ;
#50970=CARTESIAN_POINT ( 'NONE',  ( 92.69370383062498320, 88.66845928578037217, 84.13947916753383538 ) ) ;
#50971=CARTESIAN_POINT ( 'NONE',  ( 92.34999999999999432, 90.00000000000002842, 83.65000000000000568 ) ) ;
#50979=CARTESIAN_POINT ( 'NONE',  ( -97.65000000000001990, 88.47002178664754979, 82.51229166840094820 ) ) ;
#50981=ORIENTED_EDGE ( 'NONE', *, *, #65899, .F. ) ;
#50983=DIRECTION ( 'NONE',  ( 1.000000000000000000, -3.061616997868383141E-16, 0.000000000000000000 ) ) ;
#50988=( BOUNDED_CURVE ( )  B_SPLINE_CURVE ( 2, ( #52613, #1165, #41700, #41339, #12754, #35680, #58622 ),
 .UNSPECIFIED., .F., .F. ) 
 B_SPLINE_CURVE_WITH_KNOTS ( ( 3, 2, 2, 3 ),
 ( 0.2963422021981248489, 0.3033979182579413236, 0.3104536837988239872, 0.3175094496506953301 ),
 .UNSPECIFIED. ) 
 CURVE ( )  GEOMETRIC_REPRESENTATION_ITEM ( )  RATIONAL_B_SPLINE_CURVE ( ( 0.9999981209241337599, 0.8660263433289606683, 1.000000000000000000, 0.8660254037844387076, 1.000000000000000000, 0.8660254037844387076, 1.000000000000000000 ) ) 
 REPRESENTATION_ITEM ( '' )  );
#50989=CARTESIAN_POINT ( 'NONE',  ( -97.30629616937495996, -209.9999999999999716, 80.27656250086714351 ) ) ;
#50991=CARTESIAN_POINT ( 'NONE',  ( -92.69370383062502583, 88.66845928578038638, 88.63739583420047552 ) ) ;
#50995=CARTESIAN_POINT ( 'NONE',  ( -97.28022634950859526, -211.1627451397946231, 74.94226573542150049 ) ) ;
#50997=DIRECTION ( 'NONE',  ( 1.000000000000000000, 0.000000000000000000, 0.000000000000000000 ) ) ;
#50998=LINE ( 'NONE', #4412, #48488 ) ;
#51002=LINE ( 'NONE', #73924, #23226 ) ;
#51003=CARTESIAN_POINT ( 'NONE',  ( 97.64999999999999147, 90.00000000000002842, 90.00000000000000000 ) ) ;
#51008=CARTESIAN_POINT ( 'NONE',  ( 92.69370383062498320, 91.33154071421968467, 89.74864583420048803 ) ) ;
#51009=EDGE_CURVE ( 'NONE', #55876, #65477, #27472, .T. ) ;
#51010=CARTESIAN_POINT ( 'NONE',  ( -97.30629616937495996, -209.9999999999999716, 89.16656250086715829 ) ) ;
#51015=CARTESIAN_POINT ( 'NONE',  ( -95.00000000000002842, 87.33691857156074434, 78.37156250086714238 ) ) ;
#51020=CARTESIAN_POINT ( 'NONE',  ( 97.64999999999999147, 89.99999998014077107, 85.95187500101400246 ) ) ;
#51025=CARTESIAN_POINT ( 'NONE',  ( 93.84685191531249870, -208.0026889286704943, 75.09072916753380866 ) ) ;
#51028=ADVANCED_FACE ( 'NONE', ( #9477 ), #21874, .F. ) ;
#51034=CARTESIAN_POINT ( 'NONE',  ( 2.500000000000031530, 80.00000000000000000, -310.0000000000000000 ) ) ;
#51035=CARTESIAN_POINT ( 'NONE',  ( 92.35000000000000853, -209.9999999999999716, 86.82500000000000284 ) ) ;
#51037=ORIENTED_EDGE ( 'NONE', *, *, #16640, .F. ) ;
#51044=CARTESIAN_POINT ( 'NONE',  ( 96.32499999999998863, 87.70503267997126784, 87.67166666666666686 ) ) ;
#51045=CARTESIAN_POINT ( 'NONE',  ( 92.35000000000000853, -209.9999999999999716, 78.01437500173430806 ) ) ;
#51046=CARTESIAN_POINT ( 'NONE',  ( 97.64999999999999147, 90.00000000000002842, 80.79249999999998977 ) ) ;
#51048=CARTESIAN_POINT ( 'NONE',  ( 97.64999999999999147, -209.9999999999999716, 90.00000000000000000 ) ) ;
#51052=CARTESIAN_POINT ( 'NONE',  ( -96.32500000000001705, 92.29496732002878900, 89.33854166840096411 ) ) ;
#51053=CARTESIAN_POINT ( 'NONE',  ( -97.30629616937501680, 91.33154071421968467, 80.85864583420048746 ) ) ;
#51054=CARTESIAN_POINT ( 'NONE',  ( 94.99999999999998579, 87.33691857156068750, 77.73656250086713726 ) ) ;
#51060=DIRECTION ( 'NONE',  ( -0.000000000000000000, -0.000000000000000000, 1.000000000000000000 ) ) ;
#51064=CARTESIAN_POINT ( 'NONE',  ( -97.30629616937495996, -209.9999999999999716, 78.21281250086714465 ) ) ;
#51065=ORIENTED_EDGE ( 'NONE', *, *, #32057, .F. ) ;
#51069=ORIENTED_EDGE ( 'NONE', *, *, #20864, .T. ) ;
#51071=EDGE_CURVE ( 'NONE', #44773, #3345, #47681, .T. ) ;
#51073=VERTEX_POINT ( 'NONE', #66635 ) ;
#51074=CARTESIAN_POINT ( 'NONE',  ( -94.99999999999997158, -207.3369185715606307, 89.64281250086715147 ) ) ;
#51076=CARTESIAN_POINT ( 'NONE',  ( -97.64999999999997726, 88.47002178664750716, 76.71791666666666742 ) ) ;
#51083=AXIS2_PLACEMENT_3D ( 'NONE', #60349, #54696, #49423 ) ;
#51085=CARTESIAN_POINT ( 'NONE',  ( 96.15314808468748708, 91.99731107132950569, 83.71614583420047495 ) ) ;
#51092=CARTESIAN_POINT ( 'NONE',  ( -97.65000000000001990, 91.52997821335253548, 84.31145833506762699 ) ) ;
#51097=CARTESIAN_POINT ( 'NONE',  ( 92.35000000046409241, -210.0000309672231253, 77.38038495127494798 ) ) ;
#51100=CARTESIAN_POINT ( 'NONE',  ( -94.99999999999997158, -213.0599564267049857, 85.71374999999997613 ) ) ;
#51101=CARTESIAN_POINT ( 'NONE',  ( -92.35000000000005116, 88.47002178664753558, 80.10458333333330927 ) ) ;
#51103=CARTESIAN_POINT ( 'NONE',  ( -97.65000000000001990, 90.00000000000004263, 77.29999999999999716 ) ) ;
#51104=EDGE_CURVE ( 'NONE', #66094, #46998, #35178, .T. ) ;
#51105=VECTOR ( 'NONE', #28399, 1000.000000000000000 ) ;
#51111=CARTESIAN_POINT ( 'NONE',  ( 96.15314808468750130, -211.9973110713294489, 86.83822916753382515 ) ) ;
#51118=ORIENTED_EDGE ( 'NONE', *, *, #47143, .T. ) ;
#51120=CARTESIAN_POINT ( 'NONE',  ( 97.30629616937498838, -208.6684592857803295, 78.58322916753381548 ) ) ;
#51122=CARTESIAN_POINT ( 'NONE',  ( 96.15314808468748708, -208.0026889286704943, 84.50989583420049200 ) ) ;
#51132=CARTESIAN_POINT ( 'NONE',  ( 96.32499999999998863, -212.2949673200287179, 86.48104166840096241 ) ) ;
#51140=CARTESIAN_POINT ( 'NONE',  ( 95.00000000000000000, -212.6630814284392557, 75.83156250086715033 ) ) ;
#51147=CARTESIAN_POINT ( 'NONE',  ( -92.69370383062504004, 90.00000000000004263, 75.51406250086715488 ) ) ;
#51152=CARTESIAN_POINT ( 'NONE',  ( -93.84685191531247028, -211.9973110713294489, 86.67947916753381321 ) ) ;
#51155=CARTESIAN_POINT ( 'NONE',  ( 92.48104893696870477, -210.1706338775360337, 74.92125785461004739 ) ) ;
#51157=CARTESIAN_POINT ( 'NONE',  ( -92.69370383062498320, -209.9999999999999716, 77.89531250086714920 ) ) ;
#51167=CARTESIAN_POINT ( 'NONE',  ( -92.35000000000003695, 90.00000000000004263, 76.34749999999999659 ) ) ;
#51169=CARTESIAN_POINT ( 'NONE',  ( -95.00000000000002842, 92.66308142843932671, 81.86406250086714920 ) ) ;
#51174=ADVANCED_FACE ( 'NONE', ( #34262 ), #23725, .F. ) ;
#51177=CARTESIAN_POINT ( 'NONE',  ( 97.64999999964365429, -210.0000434577794408, 89.12687334326047051 ) ) ;
#51182=CARTESIAN_POINT ( 'NONE',  ( -97.65000000000001990, 90.00000000000004263, 85.63437500173431260 ) ) ;
#51183=CARTESIAN_POINT ( 'NONE',  ( -97.30629616937495996, -209.9999999999999716, 80.91156250086716284 ) ) ;
#51185=VERTEX_POINT ( 'NONE', #28618 ) ;
#51188=CARTESIAN_POINT ( 'NONE',  ( 94.99999999999998579, 93.05995642670504253, 76.58562500173430010 ) ) ;
#51192=EDGE_CURVE ( 'NONE', #52450, #48511, #45570, .T. ) ;
#51199=DIRECTION ( 'NONE',  ( -0.000000000000000000, -0.000000000000000000, 1.000000000000000000 ) ) ;
#51201=( BOUNDED_CURVE ( )  B_SPLINE_CURVE ( 2, ( #68820, #429, #69551, #35690, #58633, #23324, #5672 ),
 .UNSPECIFIED., .F., .F. ) 
 B_SPLINE_CURVE_WITH_KNOTS ( ( 3, 2, 2, 3 ),
 ( 0.7408554641904511184, 0.7479111473372028751, 0.7549669128781208993, 0.7620226289501886852 ),
 .UNSPECIFIED. ) 
 CURVE ( )  GEOMETRIC_REPRESENTATION_ITEM ( )  RATIONAL_B_SPLINE_CURVE ( ( 0.9999968710422149076, 0.8660269682816007508, 1.000000000000000000, 0.8660254037844387076, 1.000000000000000000, 0.8660263430970057685, 0.9999981213880371200 ) ) 
 REPRESENTATION_ITEM ( '' )  );
#51202=CARTESIAN_POINT ( 'NONE',  ( 97.30629616937498838, -209.9999999999999716, 86.78531250086714977 ) ) ;
#51206=CARTESIAN_POINT ( 'NONE',  ( 97.64999999999999147, -209.9999999999999716, 89.68250000000000455 ) ) ;
#51207=VERTEX_POINT ( 'NONE', #35015 ) ;
#51208=CARTESIAN_POINT ( 'NONE',  ( -92.34999999999999432, -208.4700217866474645, 84.73479166840094479 ) ) ;
#51210=CARTESIAN_POINT ( 'NONE',  ( -96.32499999999996021, -212.2949673200287179, 80.02520833506763154 ) ) ;
#51214=ORIENTED_EDGE ( 'NONE', *, *, #2824, .F. ) ;
#51216=ORIENTED_EDGE ( 'NONE', *, *, #49231, .T. ) ;
#51222=CARTESIAN_POINT ( 'NONE',  ( 95.46326757314949418, 87.15692181550788575, 74.72378867588406592 ) ) ;
#51228=CARTESIAN_POINT ( 'NONE',  ( 94.99999999999998579, 92.66308142843935514, 83.76906250086713612 ) ) ;
#51230=CARTESIAN_POINT ( 'NONE',  ( 95.00000000000000000, -212.6630814284392557, 84.72156250086713669 ) ) ;
#51231=CARTESIAN_POINT ( 'NONE',  ( -97.64999999999996305, -209.9999999999999716, 81.18937500173430521 ) ) ;
#51235=DIRECTION ( 'NONE',  ( -0.000000000000000000, -0.000000000000000000, 1.000000000000000000 ) ) ;
#51238=CARTESIAN_POINT ( 'NONE',  ( -92.69370383062498320, -211.3315407142195852, 86.73239583420047438 ) ) ;
#51239=CARTESIAN_POINT ( 'NONE',  ( -96.15314808468751551, 88.00268892867056536, 85.46239583420047836 ) ) ;
#51241=CARTESIAN_POINT ( 'NONE',  ( 93.84685191531248449, 88.00268892867053694, 82.76364583420047438 ) ) ;
#51242=CARTESIAN_POINT ( 'NONE',  ( -92.69370383062502583, 91.33154071421968467, 84.29822916753380468 ) ) ;
#51256=EDGE_CURVE ( 'NONE', #38048, #14970, #27919, .T. ) ;
#51257=CARTESIAN_POINT ( 'NONE',  ( -93.67500000000003979, 87.70503267997129626, 79.41666666666665719 ) ) ;
#51260=CARTESIAN_POINT ( 'NONE',  ( -97.64999999999994884, -209.9999678257240703, 76.74437388893710477 ) ) ;
#51262=CARTESIAN_POINT ( 'NONE',  ( -92.34999999999999432, -210.0000001167898631, 84.68187499741277691 ) ) ;
#51264=EDGE_CURVE ( 'NONE', #31708, #23659, #35606, .T. ) ;
#51267=CARTESIAN_POINT ( 'NONE',  ( -92.69370383062502583, 88.66845928578038638, 77.84239583420045960 ) ) ;
#51275=CARTESIAN_POINT ( 'NONE',  ( -93.84685191531248449, -208.0026889286704943, 88.31989583420048007 ) ) ;
#51280=CARTESIAN_POINT ( 'NONE',  ( 97.30629616937498838, 88.66845928578035796, 77.36614583420048064 ) ) ;
#51281=CARTESIAN_POINT ( 'NONE',  ( -92.69370383062498320, -208.6684592857803295, 80.64697916753382856 ) ) ;
#51290=CARTESIAN_POINT ( 'NONE',  ( -92.69370383062505425, 88.66845928578038638, 77.36614583420048064 ) ) ;
#51291=CARTESIAN_POINT ( 'NONE',  ( 96.15314808468750130, -211.9973110713294489, 81.59947916753381492 ) ) ;
#51295=VERTEX_POINT ( 'NONE', #25575 ) ;
#51301=EDGE_LOOP ( 'NONE', ( #53652, #62366, #46266, #52505 ) ) ;
#51305=CARTESIAN_POINT ( 'NONE',  ( 93.67500000000001137, -207.7050326799711968, 84.89354166840095672 ) ) ;
#51306=CARTESIAN_POINT ( 'NONE',  ( 97.30629616937498838, 90.00000000000002842, 82.49906250086715431 ) ) ;
#51308=CARTESIAN_POINT ( 'NONE',  ( 97.64999999999997726, -208.4700217866474645, 77.67041666666665378 ) ) ;
#51311=VERTEX_POINT ( 'NONE', #65806 ) ;
#51323=EDGE_LOOP ( 'NONE', ( #41156, #1302, #42085, #2937 ) ) ;
#51324=CARTESIAN_POINT ( 'NONE',  ( -97.64999999999996305, -209.9999999999999716, 83.09437500173430635 ) ) ;
#51329=CARTESIAN_POINT ( 'NONE',  ( 97.64999999999999147, 90.00000000000002842, 78.33187500173430351 ) ) ;
#51330=CARTESIAN_POINT ( 'NONE',  ( -92.35000000000005116, 91.52997821335253548, 80.28979166840098003 ) ) ;
#51332=CARTESIAN_POINT ( 'NONE',  ( 97.30629616937498838, 90.00000000000002842, 85.03906250086714635 ) ) ;
#51343=EDGE_LOOP ( 'NONE', ( #23219, #21341, #25343, #7357 ) ) ;
#51346=CARTESIAN_POINT ( 'NONE',  ( -92.34999999999999432, -211.5299782133524218, 75.10395833506764518 ) ) ;
#51350=CARTESIAN_POINT ( 'NONE',  ( 96.66135172262730180, -211.6008015735635865, 74.79754476654878204 ) ) ;
#51352=CARTESIAN_POINT ( 'NONE',  ( -96.15314808468745866, -211.9973110713294489, 81.01739583420049939 ) ) ;
#51357=CARTESIAN_POINT ( 'NONE',  ( 7.103376864691351012E-17, -120.0000000000000000, -64.00000000000000000 ) ) ;
#51361=CARTESIAN_POINT ( 'NONE',  ( 96.32499999999998863, 87.70503267997126784, 78.22604166840096696 ) ) ;
#51365=EDGE_CURVE ( 'NONE', #51185, #44202, #7298, .T. ) ;
#51369=CARTESIAN_POINT ( 'NONE',  ( 94.99999999999998579, 92.66308142843932671, 86.46781250086714010 ) ) ;
#51371=CARTESIAN_POINT ( 'NONE',  ( -92.69370383062498320, -211.3315407142195852, 88.79614583420048746 ) ) ;
#51372=CARTESIAN_POINT ( 'NONE',  ( 97.64999999999999147, 90.00000000000002842, 82.69749999999999091 ) ) ;
#51375=CARTESIAN_POINT ( 'NONE',  ( -96.15314808468751551, 88.00268892867056536, 80.85864583420047325 ) ) ;
#51380=CARTESIAN_POINT ( 'NONE',  ( 92.35000000021534561, -209.9999789922616458, 79.91868729553134187 ) ) ;
#51383=CARTESIAN_POINT ( 'NONE',  ( -97.64999999999993463, -208.4700217866474361, 84.86708333333332632 ) ) ;
#51384=CARTESIAN_POINT ( 'NONE',  ( 96.15314808468750130, -211.9973110713294489, 75.40822916753381833 ) ) ;
#51390=CARTESIAN_POINT ( 'NONE',  ( 95.00000000000000000, -207.3369185715606307, 85.83281250086717762 ) ) ;
#51395=CARTESIAN_POINT ( 'NONE',  ( 93.67500000000001137, -212.2949673200287179, 76.77083333333332860 ) ) ;
#51397=CARTESIAN_POINT ( 'NONE',  ( 97.64999999999999147, -209.9999999999999716, 88.41249999999999432 ) ) ;
#51403=CARTESIAN_POINT ( 'NONE',  ( 95.00000000000000000, -209.9999999999999716, 90.00000000000000000 ) ) ;
#51406=ADVANCED_FACE ( 'NONE', ( #30097 ), #7913, .F. ) ;
#51407=CARTESIAN_POINT ( 'NONE',  ( 97.64999999999999147, 90.00000000000002842, 87.77749999999998920 ) ) ;
#51408=CARTESIAN_POINT ( 'NONE',  ( 96.32499999999998863, -207.7050326799711968, 78.43770833506764006 ) ) ;
#51409=CARTESIAN_POINT ( 'NONE',  ( 97.64999999999997726, 91.52997821335252127, 82.11541666666666117 ) ) ;
#51417=( BOUNDED_CURVE ( )  B_SPLINE_CURVE ( 2, ( #43263, #25213, #7549, #59798, #24831, #30829, #2316 ),
 .UNSPECIFIED., .F., .F. ) 
 B_SPLINE_CURVE_WITH_KNOTS ( ( 3, 2, 2, 3 ),
 ( 0.8125000000000002220, 0.8194444444444446418, 0.8263888888888889506, 0.8333333333333334814 ),
 .UNSPECIFIED. ) 
 CURVE ( )  GEOMETRIC_REPRESENTATION_ITEM ( )  RATIONAL_B_SPLINE_CURVE ( ( 0.9999999999999956701, 0.8660254037844430375, 1.000000000000000000, 0.8660254037844387076, 1.000000000000000000, 0.8660254037844365982, 1.000000000000002220 ) ) 
 REPRESENTATION_ITEM ( '' )  );
#51418=CARTESIAN_POINT ( 'NONE',  ( -93.84685191531252713, 88.00268892867056536, 82.39322916753381776 ) ) ;
#51419=CARTESIAN_POINT ( 'NONE',  ( 94.99999999999998579, 87.33691857156068750, 77.10156250086711793 ) ) ;
#51424=EDGE_CURVE ( 'NONE', #44177, #60576, #30831, .T. ) ;
#51426=CARTESIAN_POINT ( 'NONE',  ( 93.67500000000001137, -212.2949673200287179, 85.66083333333332916 ) ) ;
#51428=ORIENTED_EDGE ( 'NONE', *, *, #43732, .F. ) ;
#51430=CARTESIAN_POINT ( 'NONE',  ( -97.30629616937495996, -209.9999999999999716, 77.57781250086713953 ) ) ;
#51431=ORIENTED_EDGE ( 'NONE', *, *, #20955, .T. ) ;
#51439=CARTESIAN_POINT ( 'NONE',  ( -94.99999999999997158, -212.6630814284392557, 75.83156250086715033 ) ) ;
#51446=CIRCLE ( 'NONE', #1107, 12.74999999999999822 ) ;
#51450=CARTESIAN_POINT ( 'NONE',  ( 92.69370383062498320, 88.66845928578035796, 83.98072916753380923 ) ) ;
#51456=VECTOR ( 'NONE', #50627, 1000.000000000000000 ) ;
#51467=CARTESIAN_POINT ( 'NONE',  ( -97.30629616937501680, 91.33154071421968467, 89.58989583420047609 ) ) ;
#51470=CARTESIAN_POINT ( 'NONE',  ( -96.32500000000001705, 87.70503267997129626, 79.94583333333332575 ) ) ;
#51478=CARTESIAN_POINT ( 'NONE',  ( 96.15314808468748708, -208.0026889286704943, 85.14489583420048291 ) ) ;
#51483=CARTESIAN_POINT ( 'NONE',  ( -97.64999999999996305, -209.9999999999999716, 87.45999999999999375 ) ) ;
#51484=ORIENTED_EDGE ( 'NONE', *, *, #42193, .F. ) ;
#51486=CARTESIAN_POINT ( 'NONE',  ( 97.30629616937498838, -208.6684592857803295, 77.94822916753381037 ) ) ;
#51488=CARTESIAN_POINT ( 'NONE',  ( 93.84685191531249870, -208.0026889286704943, 81.44072916753381719 ) ) ;
#51496=CARTESIAN_POINT ( 'NONE',  ( -93.84685191531252713, 88.00268892867056536, 75.40822916753381833 ) ) ;
#51504=CARTESIAN_POINT ( 'NONE',  ( 92.35000000000002274, -208.4700217866474645, 86.85145833506763324 ) ) ;
#51507=ORIENTED_EDGE ( 'NONE', *, *, #26233, .T. ) ;
#51512=VERTEX_POINT ( 'NONE', #23191 ) ;
#51518=ORIENTED_EDGE ( 'NONE', *, *, #19096, .T. ) ;
#51522=CARTESIAN_POINT ( 'NONE',  ( -94.99999999999997158, -206.9400435732949575, 88.57124999999999204 ) ) ;
#51524=CARTESIAN_POINT ( 'NONE',  ( -97.65000000000001990, 88.47002178664754979, 86.87791666666664980 ) ) ;
#51529=CARTESIAN_POINT ( 'NONE',  ( -97.30629616937497417, -211.3315407142195852, 85.88572916753382458 ) ) ;
#51536=CARTESIAN_POINT ( 'NONE',  ( -92.69370383062498320, -211.3315407142195852, 75.30239583420048177 ) ) ;
#51540=DIRECTION ( 'NONE',  ( -0.000000000000000000, -0.000000000000000000, 1.000000000000000000 ) ) ;
#51545=CARTESIAN_POINT ( 'NONE',  ( 94.99999999999998579, 86.94004357329502852, 80.07812500173429271 ) ) ;
#51547=CARTESIAN_POINT ( 'NONE',  ( -92.69370383062504004, 90.00000000000004263, 79.80031250086713612 ) ) ;
#51551=ORIENTED_EDGE ( 'NONE', *, *, #72943, .F. ) ;
#51556=CARTESIAN_POINT ( 'NONE',  ( 92.35000000019411459, -210.0000198427945861, 86.27002759516706476 ) ) ;
#51561=CARTESIAN_POINT ( 'NONE',  ( -96.15314808468747287, -208.0026889286704943, 80.80572916753382628 ) ) ;
#51567=CARTESIAN_POINT ( 'NONE',  ( -92.35000000000003695, 90.00000000000004263, 90.00000000000000000 ) ) ;
#51568=CARTESIAN_POINT ( 'NONE',  ( 97.64999999999999147, -209.9999999999999716, 81.42749999999999488 ) ) ;
#51575=CARTESIAN_POINT ( 'NONE',  ( 93.84685191531251292, -211.9973110713294489, 89.11364583420048291 ) ) ;
#51584=CARTESIAN_POINT ( 'NONE',  ( -97.64999999999996305, -211.5299782133524218, 79.97229166840095615 ) ) ;
#51585=ADVANCED_FACE ( 'NONE', ( #20673 ), #43626, .F. ) ;
#51591=ORIENTED_EDGE ( 'NONE', *, *, #66295, .T. ) ;
#51592=CARTESIAN_POINT ( 'NONE',  ( -94.99999999999997158, -209.9999999999999716, 90.00000000000000000 ) ) ;
#51595=CARTESIAN_POINT ( 'NONE',  ( 94.87443773336545405, 87.35320520944273426, 74.99648857272264024 ) ) ;
#51597=ORIENTED_EDGE ( 'NONE', *, *, #19947, .F. ) ;
#51601=CARTESIAN_POINT ( 'NONE',  ( 94.99999999999998579, 87.33691857156068750, 86.62656250086715204 ) ) ;
#51604=CARTESIAN_POINT ( 'NONE',  ( 96.15314808468750130, -211.9973110713294489, 80.32947916753380468 ) ) ;
#51608=CARTESIAN_POINT ( 'NONE',  ( -93.67499999999998295, -212.2949673200287179, 81.40104166840096411 ) ) ;
#51610=FACE_OUTER_BOUND ( 'NONE', #69954, .T. ) ;
#51613=CARTESIAN_POINT ( 'NONE',  ( 96.32499999999998863, 87.70503267997126784, 85.21104166840096639 ) ) ;
#51615=CARTESIAN_POINT ( 'NONE',  ( -97.30629616937497417, -208.6684592857803011, 85.14489583420048291 ) ) ;
#51616=CARTESIAN_POINT ( 'NONE',  ( -96.15314808468752972, 91.99731107132950569, 84.61572916753381435 ) ) ;
#51617=VERTEX_POINT ( 'NONE', #68314 ) ;
#51619=CARTESIAN_POINT ( 'NONE',  ( 96.15314808468748708, 91.99731107132950569, 83.71614583420047495 ) ) ;
#51620=CARTESIAN_POINT ( 'NONE',  ( -92.69370383062502583, 91.33154071421968467, 86.20322916753382003 ) ) ;
#51621=VERTEX_POINT ( 'NONE', #29915 ) ;
#51627=CARTESIAN_POINT ( 'NONE',  ( -94.99999999999997158, -212.6630814284392557, 87.26156250086714294 ) ) ;
#51636=CARTESIAN_POINT ( 'NONE',  ( -95.00000000000002842, 93.05995642670501411, 77.77624999999999034 ) ) ;
#51639=CARTESIAN_POINT ( 'NONE',  ( 95.00000000000000000, -209.9999999999999716, 90.00000000000000000 ) ) ;
#51640=CARTESIAN_POINT ( 'NONE',  ( -92.35000000000003695, 90.00000015433754186, 79.60187500750917877 ) ) ;
#51643=( BOUNDED_CURVE ( )  B_SPLINE_CURVE ( 2, ( #41293, #35280, #53675, #47663, #7073, #13074, #70209 ),
 .UNSPECIFIED., .F., .F. ) 
 B_SPLINE_CURVE_WITH_KNOTS ( ( 3, 2, 2, 3 ),
 ( 0.5833333333333329263, 0.5902777777777776791, 0.5972222222222223209, 0.6041666666666670737 ),
 .UNSPECIFIED. ) 
 CURVE ( )  GEOMETRIC_REPRESENTATION_ITEM ( )  RATIONAL_B_SPLINE_CURVE ( ( 1.000000000000008660, 0.8660254037844301589, 1.000000000000000000, 0.8660254037844387076, 1.000000000000000000, 0.8660254037844301589, 1.000000000000008660 ) ) 
 REPRESENTATION_ITEM ( '' )  );
#51647=CARTESIAN_POINT ( 'NONE',  ( -96.15314808468751551, 88.00268892867056536, 78.31864583420048120 ) ) ;
#51657=CARTESIAN_POINT ( 'NONE',  ( -92.69370383062498320, -209.9999999999999716, 88.84906250086716284 ) ) ;
#51658=CARTESIAN_POINT ( 'NONE',  ( 97.30629616937498838, 91.33154071421968467, 78.74197916753381321 ) ) ;
#51659=CARTESIAN_POINT ( 'NONE',  ( -97.30629616937495996, -209.9999999999999716, 80.91156250086716284 ) ) ;
#51662=ORIENTED_EDGE ( 'NONE', *, *, #59268, .F. ) ;
#51664=CARTESIAN_POINT ( 'NONE',  ( -92.34999999999999432, -211.5299782133524502, 75.65958333333333030 ) ) ;
#51669=CARTESIAN_POINT ( 'NONE',  ( -97.30629616937501680, 91.33154071421968467, 76.41364583420049428 ) ) ;
#51670=CARTESIAN_POINT ( 'NONE',  ( 95.00000000000000000, -212.6630814284392557, 80.27656250086714351 ) ) ;
#51674=FACE_OUTER_BOUND ( 'NONE', #3074, .T. ) ;
#51679=EDGE_CURVE ( 'NONE', #6029, #1787, #14964, .T. ) ;
#51683=EDGE_CURVE ( 'NONE', #24878, #71079, #22661, .T. ) ;
#51688=CARTESIAN_POINT ( 'NONE',  ( 93.84685191531248449, 91.99731107132950569, 83.98072916753382344 ) ) ;
#51691=ORIENTED_EDGE ( 'NONE', *, *, #10435, .T. ) ;
#51698=CARTESIAN_POINT ( 'NONE',  ( 92.34999999999999432, 90.00000000000002842, 84.28499999999999659 ) ) ;
#51708=CARTESIAN_POINT ( 'NONE',  ( -96.32499999999996021, -207.7050326799711968, 82.98854166840096980 ) ) ;
#51712=CARTESIAN_POINT ( 'NONE',  ( 97.64999999999999147, 90.00000000000002842, 77.69687500173431260 ) ) ;
#51713=CARTESIAN_POINT ( 'NONE',  ( -96.32500000000001705, 92.29496732002878900, 77.90854166840097150 ) ) ;
#51715=CARTESIAN_POINT ( 'NONE',  ( 97.30629616937498838, 88.66845928578037217, 78.63614583420049087 ) ) ;
#51716=DIRECTION ( 'NONE',  ( 4.476705744456278560E-17, -1.000000000000000000, 8.723836835350694626E-17 ) ) ;
#51733=DIRECTION ( 'NONE',  ( -0.000000000000000000, -0.000000000000000000, 1.000000000000000000 ) ) ;
#51734=CARTESIAN_POINT ( 'NONE',  ( -94.99999999999997158, -212.6630814284392557, 82.34031250086714238 ) ) ;
#51738=DIRECTION ( 'NONE',  ( 1.000000000000000000, 0.000000000000000000, -0.000000000000000000 ) ) ;
#51739=CARTESIAN_POINT ( 'NONE',  ( 92.69370383062498320, 90.00000000000002842, 76.30781250086714351 ) ) ;
#51740=FACE_OUTER_BOUND ( 'NONE', #22049, .T. ) ;
#51746=CARTESIAN_POINT ( 'NONE',  ( 97.30629616937498838, 88.66845928578035796, 87.52614583420049144 ) ) ;
#51748=CARTESIAN_POINT ( 'NONE',  ( 97.64999999999994884, 88.47002178664752137, 82.64458333333332973 ) ) ;
#51753=CARTESIAN_POINT ( 'NONE',  ( -93.84685191531254134, 91.99731107132950569, 78.00114583420048575 ) ) ;
#51756=EDGE_LOOP ( 'NONE', ( #28421, #17374, #47000, #22894 ) ) ;
#51772=CARTESIAN_POINT ( 'NONE',  ( 93.84685191531251292, -211.9973110713294489, 82.92239583420048632 ) ) ;
#51773=CARTESIAN_POINT ( 'NONE',  ( -96.32499999999996021, -207.7050326799711968, 81.00416666666666288 ) ) ;
#51775=VECTOR ( 'NONE', #21036, 1000.000000000000000 ) ;
#51777=EDGE_CURVE ( 'NONE', #38565, #4451, #32509, .T. ) ;
#51779=CARTESIAN_POINT ( 'NONE',  ( 95.00000000000000000, -206.9400435732949575, 89.84125000000000227 ) ) ;
#51784=CARTESIAN_POINT ( 'NONE',  ( -93.84685191531252713, 88.00268892867056536, 86.83822916753382515 ) ) ;
#51786=CARTESIAN_POINT ( 'NONE',  ( -97.65000000000001990, 90.00000000000004263, 83.65000000000000568 ) ) ;
#51787=CARTESIAN_POINT ( 'NONE',  ( 97.64999999999997726, -211.5299782133524502, 75.73895833506765030 ) ) ;
#51788=CARTESIAN_POINT ( 'NONE',  ( 97.64999999999997726, 88.47002178664753558, 80.10458333333332348 ) ) ;
#51792=ORIENTED_EDGE ( 'NONE', *, *, #68582, .T. ) ;
#51794=CARTESIAN_POINT ( 'NONE',  ( -93.67499999999998295, -207.7050326799711968, 82.88270833506763324 ) ) ;
#51797=CARTESIAN_POINT ( 'NONE',  ( -93.84685191531254134, 91.99731107132950569, 81.96989583420048575 ) ) ;
#51798=CARTESIAN_POINT ( 'NONE',  ( 94.99999999999998579, 92.66308142843935514, 75.51406250086714067 ) ) ;
#51804=DIRECTION ( 'NONE',  ( 1.000000000000000000, 0.000000000000000000, 0.000000000000000000 ) ) ;
#51806=FACE_OUTER_BOUND ( 'NONE', #38551, .T. ) ;
#51810=CARTESIAN_POINT ( 'NONE',  ( -92.69370383062498320, -208.6684592857803011, 79.21822916753380639 ) ) ;
#51818=ORIENTED_EDGE ( 'NONE', *, *, #7778, .F. ) ;
#51819=CARTESIAN_POINT ( 'NONE',  ( -93.84685191531248449, -208.0026889286704943, 75.46114583420047950 ) ) ;
#51828=CARTESIAN_POINT ( 'NONE',  ( 96.15314808468748708, 88.00268892867053694, 83.50447916753381605 ) ) ;
#51832=FACE_OUTER_BOUND ( 'NONE', #48620, .T. ) ;
#51837=CARTESIAN_POINT ( 'NONE',  ( 97.65000000000000568, 88.47002178664753558, 78.83458333333334167 ) ) ;
#51838=EDGE_CURVE ( 'NONE', #19675, #56878, #38024, .T. ) ;
#51840=CARTESIAN_POINT ( 'NONE',  ( -95.00000000000002842, 92.66308142843932671, 88.21406250086712930 ) ) ;
#51843=ADVANCED_FACE ( 'NONE', ( #8483, #71989 ), #71618, .T. ) ;
#51853=CARTESIAN_POINT ( 'NONE',  ( 2.500000000000034639, 89.99999999999998579, -279.9999999999999432 ) ) ;
#51854=CARTESIAN_POINT ( 'NONE',  ( 92.69370383062501162, -209.9999999999999716, 85.99156250086716113 ) ) ;
#51862=( BOUNDED_CURVE ( )  B_SPLINE_CURVE ( 2, ( #1272, #893, #35782, #164, #23055, #6499, #28297 ),
 .UNSPECIFIED., .F., .F. ) 
 B_SPLINE_CURVE_WITH_KNOTS ( ( 3, 2, 2, 3 ),
 ( 0.04166666666666644231, 0.04861111111111085514, 0.05555555555555525410, 0.06249999999999966693 ),
 .UNSPECIFIED. ) 
 CURVE ( )  GEOMETRIC_REPRESENTATION_ITEM ( )  RATIONAL_B_SPLINE_CURVE ( ( 1.000000000000004219, 0.8660254037844343777, 1.000000000000000000, 0.8660254037844387076, 1.000000000000000000, 0.8660254037844451469, 0.9999999999999935607 ) ) 
 REPRESENTATION_ITEM ( '' )  );
#51867=CARTESIAN_POINT ( 'NONE',  ( 97.30629616937498838, -208.6684592857803011, 84.45697916753383083 ) ) ;
#51870=ORIENTED_EDGE ( 'NONE', *, *, #31783, .F. ) ;
#51876=DIRECTION ( 'NONE',  ( -0.000000000000000000, -0.000000000000000000, 1.000000000000000000 ) ) ;
#51878=CARTESIAN_POINT ( 'NONE',  ( 95.00000000000000000, -209.9999999999999716, 90.00000000000000000 ) ) ;
#51879=CARTESIAN_POINT ( 'NONE',  ( 96.32499999999998863, -207.7050326799711968, 88.59770833506763665 ) ) ;
#51884=ORIENTED_EDGE ( 'NONE', *, *, #57459, .F. ) ;
#51886=EDGE_CURVE ( 'NONE', #29642, #51953, #53403, .T. ) ;
#51897=CARTESIAN_POINT ( 'NONE',  ( -95.00000000000002842, 93.05995642670501411, 86.03125000000000000 ) ) ;
#51902=CARTESIAN_POINT ( 'NONE',  ( -96.15314808468745866, -211.9973110713294489, 87.84364583420047268 ) ) ;
#51903=VERTEX_POINT ( 'NONE', #39279 ) ;
#51904=CARTESIAN_POINT ( 'NONE',  ( -92.34999999999999432, -211.5299782133524218, 79.54895833506762415 ) ) ;
#51906=CARTESIAN_POINT ( 'NONE',  ( 93.67499999999999716, 87.70503267997126784, 81.21583333333333599 ) ) ;
#51907=CARTESIAN_POINT ( 'NONE',  ( -96.15314808468745866, -211.9973110713294489, 76.41364583420048007 ) ) ;
#51915=CARTESIAN_POINT ( 'NONE',  ( -97.30629616937501680, 88.66845928578038638, 76.99572916753380980 ) ) ;
#51920=DIRECTION ( 'NONE',  ( -0.000000000000000000, -0.000000000000000000, -1.000000000000000000 ) ) ;
#51921=FACE_OUTER_BOUND ( 'NONE', #16937, .T. ) ;
#51926=CARTESIAN_POINT ( 'NONE',  ( -92.35000000000012221, 90.00000071509187194, 85.31687502647973531 ) ) ;
#51927=CARTESIAN_POINT ( 'NONE',  ( -96.15314808468747287, -208.0026889286704943, 75.09072916753380866 ) ) ;
#51930=CARTESIAN_POINT ( 'NONE',  ( -97.64999999999996305, -209.9999999999999716, 79.83999999999998920 ) ) ;
#51941=CARTESIAN_POINT ( 'NONE',  ( -97.64999999996642543, 89.99999234487438571, 78.01464417100932280 ) ) ;
#51943=CARTESIAN_POINT ( 'NONE',  ( 92.69370383062501162, -211.3315407142195852, 87.79072916753379729 ) ) ;
#51948=ORIENTED_EDGE ( 'NONE', *, *, #29262, .F. ) ;
#51951=CARTESIAN_POINT ( 'NONE',  ( -96.15314808468752972, 91.99731107132950569, 82.07572916753382231 ) ) ;
#51952=VECTOR ( 'NONE', #18560, 1000.000000000000000 ) ;
#51953=VERTEX_POINT ( 'NONE', #3968 ) ;
#51959=EDGE_CURVE ( 'NONE', #14970, #52132, #52075, .T. ) ;
#51967=CARTESIAN_POINT ( 'NONE',  ( 97.30629616937498838, 91.33154071421968467, 84.29822916753380468 ) ) ;
#51970=CARTESIAN_POINT ( 'NONE',  ( 93.84685191531251292, -211.9973110713294489, 80.22364583420046813 ) ) ;
#51973=CARTESIAN_POINT ( 'NONE',  ( -92.34999999999999432, -209.9999999999999716, 76.34749999999999659 ) ) ;
#51979=CARTESIAN_POINT ( 'NONE',  ( -94.99999999999997158, -212.6630814284392557, 84.08656250086713158 ) ) ;
#51980=CARTESIAN_POINT ( 'NONE',  ( -96.15314808468752972, 91.99731107132950569, 82.71072916753381321 ) ) ;
#51982=CARTESIAN_POINT ( 'NONE',  ( 92.69370383062498320, 90.00000000000002842, 84.56281250086713897 ) ) ;
#51985=CARTESIAN_POINT ( 'NONE',  ( 97.64999999999999147, 89.99999988321010846, 84.68187499741277691 ) ) ;
#51987=CARTESIAN_POINT ( 'NONE',  ( -94.99999999999997158, -207.3369185715606307, 86.94406250086714749 ) ) ;
#51991=DIRECTION ( 'NONE',  ( -0.000000000000000000, -0.000000000000000000, 1.000000000000000000 ) ) ;
#51994=CARTESIAN_POINT ( 'NONE',  ( -92.35000000000005116, 91.52997821335253548, 76.40041666666667197 ) ) ;
#51996=CARTESIAN_POINT ( 'NONE',  ( -94.94576887096259554, -207.6112450486804164, 74.83591575723764322 ) ) ;
#51998=VECTOR ( 'NONE', #57387, 1000.000000000000000 ) ;
#52001=CARTESIAN_POINT ( 'NONE',  ( -97.65000000000003411, -208.4700217866474929, 78.51708333333334622 ) ) ;
#52003=CARTESIAN_POINT ( 'NONE',  ( -96.15314808468752972, 91.99731107132950569, 78.74197916753381321 ) ) ;
#52004=EDGE_CURVE ( 'NONE', #10456, #67765, #49208, .T. ) ;
#52012=CARTESIAN_POINT ( 'NONE',  ( -96.32500000000001705, 87.70503267997129626, 75.58020833506763836 ) ) ;
#52013=CARTESIAN_POINT ( 'NONE',  ( -92.69370383062498320, -209.9999999999999716, 85.03906250086714635 ) ) ;
#52018=CARTESIAN_POINT ( 'NONE',  ( 93.84685191531248449, 91.99731107132950569, 75.72572916753382799 ) ) ;
#52019=CARTESIAN_POINT ( 'NONE',  ( -97.30629616937497417, -208.6684592857803295, 78.95364583420045790 ) ) ;
#52030=CARTESIAN_POINT ( 'NONE',  ( 93.84685191531251292, -211.9973110713294489, 76.41364583420048007 ) ) ;
#52042=EDGE_LOOP ( 'NONE', ( #58077, #58075, #68539, #63486 ) ) ;
#52048=CARTESIAN_POINT ( 'NONE',  ( 92.69370383062498320, 88.66845928578037217, 83.50447916753383026 ) ) ;
#52053=EDGE_CURVE ( 'NONE', #27169, #20441, #28724, .T. ) ;
#52068=CARTESIAN_POINT ( 'NONE',  ( -96.32499999999996021, -207.7050326799711968, 80.44854166840097776 ) ) ;
#52072=CARTESIAN_POINT ( 'NONE',  ( 97.64999999999999147, 90.00000000000002842, 79.60187500173429953 ) ) ;
#52073=CARTESIAN_POINT ( 'NONE',  ( -97.65000000000001990, 90.00000000000004263, 79.28437500173430408 ) ) ;
#52075=( BOUNDED_CURVE ( )  B_SPLINE_CURVE ( 2, ( #21598, #16714, #39652, #26867, #38903, #10697, #33623, #56580, #5080, #72714, #28348 ),
 .UNSPECIFIED., .F., .F. ) 
 B_SPLINE_CURVE_WITH_KNOTS ( ( 3, 2, 2, 2, 2, 3 ),
 ( 0.1481709449575320525, 0.1481710763585296908, 0.1552268418994117993, 0.1622826074402939078, 0.1693383729811760163, 0.1693384224419976214 ),
 .UNSPECIFIED. ) 
 CURVE ( )  GEOMETRIC_REPRESENTATION_ITEM ( )  RATIONAL_B_SPLINE_CURVE ( ( 0.9999950100190690971, 0.9999975049630689394, 1.000000000000000000, 0.8660254037844387076, 1.000000000000000000, 0.8660254037844387076, 1.000000000000000000, 0.8660254037844387076, 1.000000000000000000, 0.9999990608398812153, 0.9999981216929294536 ) ) 
 REPRESENTATION_ITEM ( '' )  );
#52076=ORIENTED_EDGE ( 'NONE', *, *, #32239, .T. ) ;
#52077=CARTESIAN_POINT ( 'NONE',  ( 97.30629616937498838, 90.00000000000002842, 79.95906250086714806 ) ) ;
#52094=CARTESIAN_POINT ( 'NONE',  ( -92.69370383062498320, -209.9999999999999716, 77.41906250086715602 ) ) ;
#52095=( BOUNDED_CURVE ( )  B_SPLINE_CURVE ( 2, ( #73553, #50626, #29442, #67936, #17804, #16425, #935 ),
 .UNSPECIFIED., .F., .F. ) 
 B_SPLINE_CURVE_WITH_KNOTS ( ( 3, 2, 2, 3 ),
 ( 0.6773535682752289677, 0.6844092574655884498, 0.6914650230064715020, 0.6985206468843491168 ),
 .UNSPECIFIED. ) 
 CURVE ( )  GEOMETRIC_REPRESENTATION_ITEM ( )  RATIONAL_B_SPLINE_CURVE ( ( 0.9999971005499468379, 0.8660268535251529620, 1.000000000000000000, 0.8660254037844387076, 1.000000000000000000, 0.8660280936759657822, 0.9999946203249591159 ) ) 
 REPRESENTATION_ITEM ( '' )  );
#52103=CARTESIAN_POINT ( 'NONE',  ( 96.15314808468748708, 88.00268892867053694, 75.24947916753380639 ) ) ;
#52107=DIRECTION ( 'NONE',  ( 1.000000000000000000, 0.000000000000000000, 0.000000000000000000 ) ) ;
#52111=VECTOR ( 'NONE', #62666, 1000.000000000000000 ) ;
#52113=CARTESIAN_POINT ( 'NONE',  ( 96.15314808468748708, 91.99731107132950569, 88.95489583420049939 ) ) ;
#52118=CARTESIAN_POINT ( 'NONE',  ( -93.84685191531252713, 88.00268892867056536, 79.69447916753379957 ) ) ;
#52120=CARTESIAN_POINT ( 'NONE',  ( 93.84685191531249870, -208.0026889286704943, 86.99697916753380866 ) ) ;
#52123=CARTESIAN_POINT ( 'NONE',  ( -97.65000000000001990, 90.00000000000004263, 90.00000000000000000 ) ) ;
#52128=EDGE_CURVE ( 'NONE', #74057, #15980, #23741, .T. ) ;
#52132=VERTEX_POINT ( 'NONE', #8391 ) ;
#52134=CARTESIAN_POINT ( 'NONE',  ( 92.69370383062501162, -211.3315407142195852, 82.23447916753383424 ) ) ;
#52136=EDGE_CURVE ( 'NONE', #66421, #59589, #43362, .T. ) ;
#52141=CARTESIAN_POINT ( 'NONE',  ( 93.67500000000001137, -207.7050326799711968, 84.17916666666666003 ) ) ;
#52144=VERTEX_POINT ( 'NONE', #42243 ) ;
#52148=CARTESIAN_POINT ( 'NONE',  ( -95.00000000000002842, 92.66308142843932671, 86.46781250086716852 ) ) ;
#52151=CARTESIAN_POINT ( 'NONE',  ( 93.67500000000001137, -207.7050326799711968, 75.36854166840096525 ) ) ;
#52152=CARTESIAN_POINT ( 'NONE',  ( 94.99999999999998579, 86.94004357329500010, 78.72875000000001933 ) ) ;
#52153=ORIENTED_EDGE ( 'NONE', *, *, #30644, .T. ) ;
#52154=CARTESIAN_POINT ( 'NONE',  ( -94.99999999999997158, -206.9400435732949575, 89.28562500173430294 ) ) ;
#52156=CARTESIAN_POINT ( 'NONE',  ( -97.64999999953492704, -210.0000309987302956, 83.09538598079114990 ) ) ;
#52159=CARTESIAN_POINT ( 'NONE',  ( 96.32499999999998863, 87.70503267997126784, 84.57604166840096127 ) ) ;
#52160=CARTESIAN_POINT ( 'NONE',  ( -95.00000000000002842, 92.66308142843932671, 81.38781250086715602 ) ) ;
#52161=CARTESIAN_POINT ( 'NONE',  ( 93.84685191531248449, 88.00268892867053694, 75.14364583420046984 ) ) ;
#52169=CARTESIAN_POINT ( 'NONE',  ( -96.15314808468745866, -211.9973110713294489, 77.04864583420047097 ) ) ;
#52178=CARTESIAN_POINT ( 'NONE',  ( -97.30629616937495996, -209.9999999999999716, 89.16656250086715829 ) ) ;
#52184=VERTEX_POINT ( 'NONE', #7647 ) ;
#52187=CARTESIAN_POINT ( 'NONE',  ( -97.65000000000001990, 89.99996406046686559, 83.72937624475873974 ) ) ;
#52188=VECTOR ( 'NONE', #33152, 1000.000000000000000 ) ;
#52191=CARTESIAN_POINT ( 'NONE',  ( 92.69370383062498320, 90.00000000000002842, 85.83281250086714920 ) ) ;
#52194=CARTESIAN_POINT ( 'NONE',  ( 95.00000000000000000, -206.9400435732949575, 86.66624999999999091 ) ) ;
#52198=CARTESIAN_POINT ( 'NONE',  ( 97.64999999999999147, -210.0000000334413244, 87.85687500050293863 ) ) ;
#52205=ADVANCED_FACE ( 'NONE', ( #25315 ), #47866, .F. ) ;
#52216=CARTESIAN_POINT ( 'NONE',  ( -92.35000000000003695, 90.00000000000004263, 90.00000000000000000 ) ) ;
#52217=EDGE_CURVE ( 'NONE', #44776, #24481, #65047, .T. ) ;
#52218=ADVANCED_FACE ( 'NONE', ( #65174 ), #14012, .F. ) ;
#52220=CARTESIAN_POINT ( 'NONE',  ( 92.69370383062501162, -208.6684592857803011, 84.03364583420049883 ) ) ;
#52226=CARTESIAN_POINT ( 'NONE',  ( 97.30629616937498838, -209.9999999999999716, 75.99031250086714806 ) ) ;
#52230=CARTESIAN_POINT ( 'NONE',  ( 97.30629616937498838, -208.6684592857803011, 79.37697916753381833 ) ) ;
#52240=EDGE_LOOP ( 'NONE', ( #35273, #47162, #15345, #25709 ) ) ;
#52242=CARTESIAN_POINT ( 'NONE',  ( 93.67500000000001137, -212.2949673200287179, 87.01020833506763097 ) ) ;
#52250=CARTESIAN_POINT ( 'NONE',  ( 92.34999999999999432, 88.47002178664753558, 85.68729166840097378 ) ) ;
#52263=CARTESIAN_POINT ( 'NONE',  ( -93.67500000000003979, 87.70503267997129626, 87.03666666666666174 ) ) ;
#52269=CYLINDRICAL_SURFACE ( 'NONE', #11911, 12.74999999999999822 ) ;
#52270=CARTESIAN_POINT ( 'NONE',  ( -93.84685191531247028, -211.9973110713294489, 85.40947916753380298 ) ) ;
#52272=CARTESIAN_POINT ( 'NONE',  ( -97.64999999999997726, -209.9999856621396930, 79.28437450583719226 ) ) ;
#52275=CARTESIAN_POINT ( 'NONE',  ( -96.15314808468745866, -211.9973110713294489, 77.68364583420047609 ) ) ;
#52285=CARTESIAN_POINT ( 'NONE',  ( -95.00000000000002842, 92.66308142843932671, 79.32406250086714294 ) ) ;
#52298=CARTESIAN_POINT ( 'NONE',  ( -93.84685191531247028, -211.9973110713294489, 76.67822916753381435 ) ) ;
#52302=VECTOR ( 'NONE', #38409, 1000.000000000000000 ) ;
#52303=( BOUNDED_CURVE ( )  B_SPLINE_CURVE ( 2, ( #54299, #48650, #70827, #13685, #38104, #3553, #32083, #14800, #8436 ),
 .UNSPECIFIED., .F., .F. ) 
 B_SPLINE_CURVE_WITH_KNOTS ( ( 3, 2, 2, 2, 3 ),
 ( 0.7620226289464456793, 0.7620226784152968058, 0.7690784439561787478, 0.7761342094970608008, 0.7831899741065913023 ),
 .UNSPECIFIED. ) 
 CURVE ( )  GEOMETRIC_REPRESENTATION_ITEM ( )  RATIONAL_B_SPLINE_CURVE ( ( 0.9999981213880071440, 0.9999990606874179511, 1.000000000000000000, 0.8660254037844387076, 1.000000000000000000, 0.8660254037844387076, 1.000000000000000000, 0.8660254037844387076, 1.000000000000000000 ) ) 
 REPRESENTATION_ITEM ( '' )  );
#52315=CARTESIAN_POINT ( 'NONE',  ( 96.15314808468750130, -211.9973110713294489, 84.13947916753380696 ) ) ;
#52322=CARTESIAN_POINT ( 'NONE',  ( -96.15314808468751551, 88.00268892867056536, 82.28739583420048120 ) ) ;
#52327=EDGE_CURVE ( 'NONE', #68050, #34509, #26146, .T. ) ;
#52337=CARTESIAN_POINT ( 'NONE',  ( 92.69370383062501162, -211.3315407142195852, 82.71072916753379900 ) ) ;
#52341=AXIS2_PLACEMENT_3D ( 'NONE', #9307, #36125, #41765 ) ;
#52345=AXIS2_PLACEMENT_3D ( 'NONE', #61270, #3400, #9015 ) ;
#52347=CARTESIAN_POINT ( 'NONE',  ( 95.00000000000000000, -206.9400435732949575, 76.50624999999999432 ) ) ;
#52348=CARTESIAN_POINT ( 'NONE',  ( -94.99999999999997158, -207.3369185715606307, 85.67406250086715147 ) ) ;
#52350=CARTESIAN_POINT ( 'NONE',  ( -96.15314808468751551, 88.00268892867056536, 81.01739583420049939 ) ) ;
#52351=ORIENTED_EDGE ( 'NONE', *, *, #35542, .T. ) ;
#52353=CARTESIAN_POINT ( 'NONE',  ( 92.69370383062498320, 88.66845928578037217, 83.34572916753380412 ) ) ;
#52356=CARTESIAN_POINT ( 'NONE',  ( -92.35000000000005116, 88.47002178664754979, 78.91395833506763324 ) ) ;
#52359=CARTESIAN_POINT ( 'NONE',  ( 93.67500000000001137, -207.7050326799711968, 85.44916666666665606 ) ) ;
#52360=CARTESIAN_POINT ( 'NONE',  ( -92.69370383062498320, -209.9999999999999716, 85.51531250086713953 ) ) ;
#52368=ORIENTED_EDGE ( 'NONE', *, *, #32664, .F. ) ;
#52369=CARTESIAN_POINT ( 'NONE',  ( -96.32500000000001705, 87.70503267997129626, 77.40583333333331950 ) ) ;
#52370=CARTESIAN_POINT ( 'NONE',  ( -97.64999999999996305, -209.9999999999999716, 78.57000000000000739 ) ) ;
#52371=CARTESIAN_POINT ( 'NONE',  ( -95.31113939543058677, -207.6265741463517998, 74.84415580543367241 ) ) ;
#52374=CARTESIAN_POINT ( 'NONE',  ( 97.64999999946594755, -209.9999467985095976, 78.96687695417307395 ) ) ;
#52377=CARTESIAN_POINT ( 'NONE',  ( -95.00000000000002842, 87.33691857156074434, 79.64156250086713840 ) ) ;
#52383=CARTESIAN_POINT ( 'NONE',  ( -96.15314808468747287, -208.0026889286704943, 85.88572916753381037 ) ) ;
#52388=CARTESIAN_POINT ( 'NONE',  ( 94.99999999999998579, 92.66308142843932671, 76.94281250086714863 ) ) ;
#52389=CARTESIAN_POINT ( 'NONE',  ( -94.99999999999997158, -212.6630814284392557, 75.35531250086715715 ) ) ;
#52392=CARTESIAN_POINT ( 'NONE',  ( -96.32500000000001705, 92.29496732002878900, 82.98854166840096980 ) ) ;
#52398=CARTESIAN_POINT ( 'NONE',  ( 97.30629616937498838, -209.9999999999999716, 75.35531250086714294 ) ) ;
#52402=ORIENTED_EDGE ( 'NONE', *, *, #22798, .T. ) ;
#52403=CARTESIAN_POINT ( 'NONE',  ( -92.34999999999999432, -209.9999999999999716, 90.00000000000000000 ) ) ;
#52406=VERTEX_POINT ( 'NONE', #28256 ) ;
#52412=CARTESIAN_POINT ( 'NONE',  ( 97.30629616937498838, 90.00000000000002842, 85.03906250086714635 ) ) ;
#52415=ORIENTED_EDGE ( 'NONE', *, *, #57164, .T. ) ;
#52416=ORIENTED_EDGE ( 'NONE', *, *, #69928, .F. ) ;
#52422=CARTESIAN_POINT ( 'NONE',  ( -92.35000000000005116, 88.47002178664753558, 87.72458333333332803 ) ) ;
#52429=EDGE_LOOP ( 'NONE', ( #10943, #541, #73661, #41881 ) ) ;
#52430=CARTESIAN_POINT ( 'NONE',  ( -97.64999999999994884, -211.5299782133524502, 78.06729166840096923 ) ) ;
#52433=LINE ( 'NONE', #30607, #66323 ) ;
#52435=CARTESIAN_POINT ( 'NONE',  ( 96.32499999999998863, 87.70503267997126784, 78.86104166840097207 ) ) ;
#52436=CARTESIAN_POINT ( 'NONE',  ( -96.32500000000001705, 92.29496732002878900, 79.81354166840095843 ) ) ;
#52438=CARTESIAN_POINT ( 'NONE',  ( 93.84685191531248449, 88.00268892867053694, 80.38239583420048007 ) ) ;
#52446=LINE ( 'NONE', #63031, #40942 ) ;
#52449=VECTOR ( 'NONE', #62939, 1000.000000000000000 ) ;
#52450=VERTEX_POINT ( 'NONE', #64342 ) ;
#52452=LINE ( 'NONE', #71866, #56499 ) ;
#52457=CARTESIAN_POINT ( 'NONE',  ( -97.30629616937495996, -209.9999999999999716, 79.00656250086716170 ) ) ;
#52460=AXIS2_PLACEMENT_3D ( 'NONE', #44358, #10134, #56000 ) ;
#52462=CYLINDRICAL_SURFACE ( 'NONE', #42697, 2.649999999999985700 ) ;
#52470=CARTESIAN_POINT ( 'NONE',  ( 94.99999999999998579, 90.00000000000002842, 90.00000000000000000 ) ) ;
#52476=CARTESIAN_POINT ( 'NONE',  ( 92.69370383062498320, 90.00000000000002842, 88.53156250086716739 ) ) ;
#52477=CARTESIAN_POINT ( 'NONE',  ( -97.30629616937497417, -211.3315407142195852, 87.31447916753381833 ) ) ;
#52478=CARTESIAN_POINT ( 'NONE',  ( 97.64996928176852009, 91.52999594853174870, 79.01979289519825045 ) ) ;
#52479=VERTEX_POINT ( 'NONE', #29727 ) ;
#52481=CARTESIAN_POINT ( 'NONE',  ( -92.34999999999999432, -209.9999999999999716, 82.69749999999999091 ) ) ;
#52482=CARTESIAN_POINT ( 'NONE',  ( -93.84685191531254134, 91.99731107132950569, 74.82614583420047438 ) ) ;
#52483=CARTESIAN_POINT ( 'NONE',  ( 97.30629616937498838, -208.6684592857803011, 86.83822916753381094 ) ) ;
#52486=VECTOR ( 'NONE', #44624, 1000.000000000000000 ) ;
#52494=CARTESIAN_POINT ( 'NONE',  ( 96.15314808468750130, -211.9973110713294489, 81.12322916753382174 ) ) ;
#52497=( BOUNDED_CURVE ( )  B_SPLINE_CURVE ( 2, ( #36486, #48515, #20310, #66189, #25582, #71428, #65084 ),
 .UNSPECIFIED., .F., .F. ) 
 B_SPLINE_CURVE_WITH_KNOTS ( ( 3, 2, 2, 3 ),
 ( 0.3333333333333333703, 0.3402777777777777901, 0.3472222222222221544, 0.3541666666666665741 ),
 .UNSPECIFIED. ) 
 CURVE ( )  GEOMETRIC_REPRESENTATION_ITEM ( )  RATIONAL_B_SPLINE_CURVE ( ( 0.9999999999999988898, 0.8660254037844398178, 1.000000000000000000, 0.8660254037844387076, 1.000000000000000000, 0.8660254037844408170, 0.9999999999999978906 ) ) 
 REPRESENTATION_ITEM ( '' )  );
#52499=CARTESIAN_POINT ( 'NONE',  ( -92.35000000000003695, 89.99999998014077107, 85.95187500101400246 ) ) ;
#52501=CARTESIAN_POINT ( 'NONE',  ( 96.32499999999998863, -207.7050326799711968, 84.70833333333332860 ) ) ;
#52505=ORIENTED_EDGE ( 'NONE', *, *, #134, .F. ) ;
#52510=CARTESIAN_POINT ( 'NONE',  ( -95.00000000000002842, 87.33691857156074434, 86.78531250086716398 ) ) ;
#52514=CARTESIAN_POINT ( 'NONE',  ( 95.00000000000000000, -206.9400435732949575, 76.58562500173430010 ) ) ;
#52516=CARTESIAN_POINT ( 'NONE',  ( 93.67499999999999716, 87.70503267997126784, 78.67583333333332973 ) ) ;
#52519=CARTESIAN_POINT ( 'NONE',  ( 92.34999999999999432, 90.00000000000002842, 79.83999999999998920 ) ) ;
#52525=CARTESIAN_POINT ( 'NONE',  ( -93.84685191531252713, 88.00268892867056536, 80.48822916753381662 ) ) ;
#52526=CARTESIAN_POINT ( 'NONE',  ( 96.15314808468748708, 88.00268892867053694, 76.51947916753380241 ) ) ;
#52535=CARTESIAN_POINT ( 'NONE',  ( -93.84685191531247028, -211.9973110713294489, 75.24947916753380639 ) ) ;
#52536=ORIENTED_EDGE ( 'NONE', *, *, #44729, .F. ) ;
#52539=ORIENTED_EDGE ( 'NONE', *, *, #32311, .T. ) ;
#52543=CARTESIAN_POINT ( 'NONE',  ( -97.30629616937497417, -208.6684592857803011, 87.84364583420048689 ) ) ;
#52545=CARTESIAN_POINT ( 'NONE',  ( 97.65000000000000568, 91.52997821335252127, 88.54479166840097548 ) ) ;
#52558=CARTESIAN_POINT ( 'NONE',  ( 93.84685191531248449, 91.99731107132950569, 81.91697916753381037 ) ) ;
#52568=FACE_OUTER_BOUND ( 'NONE', #33667, .T. ) ;
#52571=CARTESIAN_POINT ( 'NONE',  ( -92.69370383062505425, 91.33154071421968467, 85.56822916753380071 ) ) ;
#52583=CARTESIAN_POINT ( 'NONE',  ( 96.15314808468750130, -211.9973110713294489, 80.48822916753381662 ) ) ;
#52589=CARTESIAN_POINT ( 'NONE',  ( 96.73972734126404305, -208.4859488783623362, 74.79348190356850523 ) ) ;
#52592=CARTESIAN_POINT ( 'NONE',  ( 92.69370383062501162, -208.6684592857803011, 78.95364583420048632 ) ) ;
#52597=CARTESIAN_POINT ( 'NONE',  ( 96.32499999999997442, 92.29496732002878900, 80.34270833506762699 ) ) ;
#52608=CARTESIAN_POINT ( 'NONE',  ( 95.00000000000000000, -213.0599564267049857, 86.42812500173430124 ) ) ;
#52610=CARTESIAN_POINT ( 'NONE',  ( 97.64999999999997726, 88.47002178664753558, 87.72458333333332803 ) ) ;
#52613=CARTESIAN_POINT ( 'NONE',  ( 92.35000000003287823, 90.00000839536618003, 84.99910573348789455 ) ) ;
#52615=ORIENTED_EDGE ( 'NONE', *, *, #6983, .F. ) ;
#52618=CARTESIAN_POINT ( 'NONE',  ( 96.32499999999997442, 92.29496732002878900, 86.69270833506763552 ) ) ;
#52634=CARTESIAN_POINT ( 'NONE',  ( -96.32500000000001705, 87.70503267997129626, 86.29583333333333428 ) ) ;
#52636=CARTESIAN_POINT ( 'NONE',  ( 92.34999999999999432, 90.00000000000002842, 81.74500000000000455 ) ) ;
#52641=CARTESIAN_POINT ( 'NONE',  ( -97.30629616937497417, -211.3315407142195852, 81.44072916753381719 ) ) ;
#52644=CARTESIAN_POINT ( 'NONE',  ( 92.49271422325850267, -210.3406226724007979, 74.92458348457969919 ) ) ;
#52646=CARTESIAN_POINT ( 'NONE',  ( -97.30629616937495996, -209.9999999999999716, 76.94281250086713442 ) ) ;
#52653=CARTESIAN_POINT ( 'NONE',  ( 97.64999999999992042, 88.47002178664749295, 88.35958333333334735 ) ) ;
#52654=CARTESIAN_POINT ( 'NONE',  ( -93.84685191531254134, 91.99731107132950569, 78.63614583420047666 ) ) ;
#52657=VECTOR ( 'NONE', #48999, 1000.000000000000000 ) ;
#52662=CARTESIAN_POINT ( 'NONE',  ( 92.35000000005783249, -210.0000112241611703, 75.47473230081648410 ) ) ;
#52664=CARTESIAN_POINT ( 'NONE',  ( -94.99999999999997158, -209.9999999999999716, 90.00000000000000000 ) ) ;
#52665=AXIS2_PLACEMENT_3D ( 'NONE', #30453, #30090, #47395 ) ;
#52667=CARTESIAN_POINT ( 'NONE',  ( -92.35000000000003695, 90.00000000000004263, 90.00000000000000000 ) ) ;
#52668=CARTESIAN_POINT ( 'NONE',  ( -96.15314808468745866, -211.9973110713294489, 77.20739583420048291 ) ) ;
#52670=DIRECTION ( 'NONE',  ( -0.000000000000000000, -0.000000000000000000, 1.000000000000000000 ) ) ;
#52688=CARTESIAN_POINT ( 'NONE',  ( 96.15314808468750130, -211.9973110713294489, 86.67947916753381321 ) ) ;
#52692=EDGE_CURVE ( 'NONE', #57437, #32439, #52497, .T. ) ;
#52693=CARTESIAN_POINT ( 'NONE',  ( 95.00000000000000000, -212.6630814284392557, 89.32531250086715602 ) ) ;
#52697=CARTESIAN_POINT ( 'NONE',  ( -97.30629616937501680, 91.33154071421968467, 82.12864583420048348 ) ) ;
#52698=ORIENTED_EDGE ( 'NONE', *, *, #16325, .F. ) ;
#52707=DIRECTION ( 'NONE',  ( 1.000000000000000000, 0.000000000000000000, 0.000000000000000000 ) ) ;
#52709=CARTESIAN_POINT ( 'NONE',  ( 94.37155072198197558, 87.44368763736524386, 74.98613922222769190 ) ) ;
#52711=AXIS2_PLACEMENT_3D ( 'NONE', #58747, #64760, #42202 ) ;
#52716=CARTESIAN_POINT ( 'NONE',  ( 93.84685191531251292, -211.9973110713294489, 80.85864583420047325 ) ) ;
#52718=CARTESIAN_POINT ( 'NONE',  ( -97.64999999999996305, -209.9999999999999716, 76.66499999999999204 ) ) ;
#52724=CARTESIAN_POINT ( 'NONE',  ( -92.35000000000009379, 88.47002178664753558, 82.64458333333332973 ) ) ;
#52725=CARTESIAN_POINT ( 'NONE',  ( -96.15314808468745866, -211.9973110713294489, 83.39864583420047950 ) ) ;
#52727=CARTESIAN_POINT ( 'NONE',  ( -95.00000000000002842, 92.66308142843932671, 83.92781250086716227 ) ) ;
#52730=CARTESIAN_POINT ( 'NONE',  ( 94.99999999999998579, 92.66308142843935514, 79.95906250086713385 ) ) ;
#52738=CARTESIAN_POINT ( 'NONE',  ( -96.15314808468745866, -211.9973110713294489, 87.84364583420047268 ) ) ;
#52751=CARTESIAN_POINT ( 'NONE',  ( -96.32500000000001705, 92.29496732002878900, 77.82916666666665151 ) ) ;
#52754=DIRECTION ( 'NONE',  ( -0.000000000000000000, -0.000000000000000000, 1.000000000000000000 ) ) ;
#52759=( BOUNDED_CURVE ( )  B_SPLINE_CURVE ( 2, ( #12490, #13234, #35428, #23415, #18865, #58356, #6856 ),
 .UNSPECIFIED., .F., .F. ) 
 B_SPLINE_CURVE_WITH_KNOTS ( ( 3, 2, 2, 3 ),
 ( 0.3125000000000001665, 0.3194444444444445308, 0.3263888888888890061, 0.3333333333333333703 ),
 .UNSPECIFIED. ) 
 CURVE ( )  GEOMETRIC_REPRESENTATION_ITEM ( )  RATIONAL_B_SPLINE_CURVE ( ( 0.9999999999999967804, 0.8660254037844419273, 1.000000000000000000, 0.8660254037844387076, 1.000000000000000000, 0.8660254037844375974, 1.000000000000001110 ) ) 
 REPRESENTATION_ITEM ( '' )  );
#52761=CARTESIAN_POINT ( 'NONE',  ( -96.15314808468752972, 91.99731107132950569, 75.56697916753381605 ) ) ;
#52766=CARTESIAN_POINT ( 'NONE',  ( -93.67500000000003979, 87.70503267997129626, 75.68604166840097491 ) ) ;
#52767=CARTESIAN_POINT ( 'NONE',  ( -94.99999999999997158, -207.3369185715606307, 84.56281250086716739 ) ) ;
#52774=CARTESIAN_POINT ( 'NONE',  ( -93.84685191531247028, -211.9973110713294489, 76.67822916753381435 ) ) ;
#52780=CARTESIAN_POINT ( 'NONE',  ( -92.35000982492222477, 88.47001611422608391, 88.43895794268867405 ) ) ;
#52783=CARTESIAN_POINT ( 'NONE',  ( -92.69370383062505425, 88.66845928578038638, 76.09614583420048461 ) ) ;
#52784=CARTESIAN_POINT ( 'NONE',  ( 92.69370383062501162, -208.6684592857803011, 76.88989583420047325 ) ) ;
#52796=ORIENTED_EDGE ( 'NONE', *, *, #7906, .T. ) ;
#52802=CARTESIAN_POINT ( 'NONE',  ( 94.99999999999998579, 87.33691857156068750, 84.88031250086714863 ) ) ;
#52805=DIRECTION ( 'NONE',  ( -0.000000000000000000, -0.000000000000000000, 1.000000000000000000 ) ) ;
#52806=VERTEX_POINT ( 'NONE', #4526 ) ;
#52810=VERTEX_POINT ( 'NONE', #20682 ) ;
#52812=CARTESIAN_POINT ( 'NONE',  ( -94.99999999999997158, -206.9400435732949575, 75.31562500173430408 ) ) ;
#52813=CARTESIAN_POINT ( 'NONE',  ( 92.34999999999999432, 90.00000000000002842, 83.65000000000000568 ) ) ;
#52818=CARTESIAN_POINT ( 'NONE',  ( -93.67499999999998295, -212.2949673200287179, 78.86104166840097207 ) ) ;
#52821=LINE ( 'NONE', #36260, #9851 ) ;
#52824=CARTESIAN_POINT ( 'NONE',  ( 93.67499999999999716, 87.70503267997126784, 78.75520833506763552 ) ) ;
#52825=CARTESIAN_POINT ( 'NONE',  ( -96.32500000000001705, 87.70503267997129626, 75.58020833506763836 ) ) ;
#52827=VERTEX_POINT ( 'NONE', #73287 ) ;
#52829=CARTESIAN_POINT ( 'NONE',  ( 92.69370383062498320, 91.33154071421968467, 79.58864583420047722 ) ) ;
#52845=CARTESIAN_POINT ( 'NONE',  ( -92.69370383062498320, -208.6684592857803011, 78.74197916753382742 ) ) ;
#52847=AXIS2_PLACEMENT_3D ( 'NONE', #62277, #4781, #55885 ) ;
#52852=CYLINDRICAL_SURFACE ( 'NONE', #72628, 2.649999999999985700 ) ;
#52853=CARTESIAN_POINT ( 'NONE',  ( -92.35000000000003695, 90.00000000000004263, 83.96750000000000114 ) ) ;
#52854=CARTESIAN_POINT ( 'NONE',  ( -99.99999999999997158, -214.9999999999999716, -90.00000000000000000 ) ) ;
#52855=DIRECTION ( 'NONE',  ( -1.000000000000000000, -0.000000000000000000, -0.000000000000000000 ) ) ;
#52860=CARTESIAN_POINT ( 'NONE',  ( -89.99999999999998579, -124.0000000000000142, 39.99999999999996447 ) ) ;
#52862=CARTESIAN_POINT ( 'NONE',  ( 94.99999999999998579, 92.66308142843932671, 87.10281250086715943 ) ) ;
#52863=CARTESIAN_POINT ( 'NONE',  ( -97.30629616937495996, -209.9999999999999716, 85.99156250086716113 ) ) ;
#52867=CARTESIAN_POINT ( 'NONE',  ( 97.64999999999999147, -209.9999999999999716, 83.41187500173430180 ) ) ;
#52868=CARTESIAN_POINT ( 'NONE',  ( -94.99999999999997158, -206.9400435732949575, 79.68124999999999147 ) ) ;
#52869=CARTESIAN_POINT ( 'NONE',  ( -95.00000000000002842, 92.66308142843932671, 76.78406250086712248 ) ) ;
#52871=CARTESIAN_POINT ( 'NONE',  ( 92.69370383062501162, -208.6684592857803011, 86.41489583420047893 ) ) ;
#52883=CARTESIAN_POINT ( 'NONE',  ( 92.69370383062501162, -208.6684592857803295, 83.39864583420049371 ) ) ;
#52885=CARTESIAN_POINT ( 'NONE',  ( 100.0010000000000190, -123.9999999999999858, -40.00000000000002132 ) ) ;
#52886=CARTESIAN_POINT ( 'NONE',  ( 97.64999999999999147, 90.00000000000002842, 82.69749999999999091 ) ) ;
#52890=CARTESIAN_POINT ( 'NONE',  ( 95.00000000000000000, -206.9400435732949575, 85.39624999999998067 ) ) ;
#52899=CARTESIAN_POINT ( 'NONE',  ( -97.30629616937501680, 91.33154071421968467, 87.84364583420048689 ) ) ;
#52903=CARTESIAN_POINT ( 'NONE',  ( 97.30629616937498838, -208.6684592857803011, 88.74322916753379786 ) ) ;
#52904=CARTESIAN_POINT ( 'NONE',  ( 96.32499999999997442, 92.29496732002878900, 78.35833333333333428 ) ) ;
#52908=EDGE_CURVE ( 'NONE', #48244, #54357, #5643, .T. ) ;
#52909=CARTESIAN_POINT ( 'NONE',  ( 93.67500000000001137, -212.2949673200287179, 79.94583333333332575 ) ) ;
#52912=CARTESIAN_POINT ( 'NONE',  ( -96.32500000000001705, 87.70503267997129626, 87.01020833506763097 ) ) ;
#52913=CARTESIAN_POINT ( 'NONE',  ( 97.30629616937498838, 90.00000000000002842, 89.48406250086715374 ) ) ;
#52916=CARTESIAN_POINT ( 'NONE',  ( -2.500000000000020428, -90.00000000000000000, -90.00000000000000000 ) ) ;
#52917=DIRECTION ( 'NONE',  ( 1.000000000000000000, 0.000000000000000000, 0.000000000000000000 ) ) ;
#52919=ORIENTED_EDGE ( 'NONE', *, *, #41692, .T. ) ;
#52920=CARTESIAN_POINT ( 'NONE',  ( -92.35000000000003695, 90.00000000000004263, 89.04749999999999943 ) ) ;
#52921=CARTESIAN_POINT ( 'NONE',  ( -97.30629616937497417, -208.6684592857803011, 75.61989583420047722 ) ) ;
#52927=ORIENTED_EDGE ( 'NONE', *, *, #12080, .T. ) ;
#52928=CARTESIAN_POINT ( 'NONE',  ( -92.69370383062498320, -208.6684592857803011, 87.63197916753382799 ) ) ;
#52935=CARTESIAN_POINT ( 'NONE',  ( -97.65000000000001990, 91.52997821335253548, 83.67645833506763609 ) ) ;
#52938=CARTESIAN_POINT ( 'NONE',  ( 96.15314808468748708, 88.00268892867053694, 82.23447916753380582 ) ) ;
#52951=CARTESIAN_POINT ( 'NONE',  ( -97.30629616937501680, 91.33154071421968467, 87.04989583420046984 ) ) ;
#52959=( BOUNDED_CURVE ( )  B_SPLINE_CURVE ( 2, ( #19624, #42570, #8358, #31278, #39150, #54951, #15465 ),
 .UNSPECIFIED., .F., .F. ) 
 B_SPLINE_CURVE_WITH_KNOTS ( ( 3, 2, 2, 3 ),
 ( 0.1874999999999999167, 0.1944444444444443365, 0.2013888888888887285, 0.2083333333333331483 ),
 .UNSPECIFIED. ) 
 CURVE ( )  GEOMETRIC_REPRESENTATION_ITEM ( )  RATIONAL_B_SPLINE_CURVE ( ( 1.000000000000001554, 0.8660254037844371533, 1.000000000000000000, 0.8660254037844387076, 1.000000000000000000, 0.8660254037844424824, 0.9999999999999962252 ) ) 
 REPRESENTATION_ITEM ( '' )  );
#52965=CARTESIAN_POINT ( 'NONE',  ( 93.84685191531249870, -208.0026889286704943, 83.34572916753383254 ) ) ;
#52968=CYLINDRICAL_SURFACE ( 'NONE', #5646, 12.74999999999999822 ) ;
#52971=CARTESIAN_POINT ( 'NONE',  ( 92.34999999999993747, -208.4700217866474929, 88.67708333333332860 ) ) ;
#52972=CARTESIAN_POINT ( 'NONE',  ( 96.15314808468748708, -208.0026889286704943, 74.82614583420047438 ) ) ;
#52975=CARTESIAN_POINT ( 'NONE',  ( 92.69370383062501162, -209.9999999999999716, 78.37156250086715659 ) ) ;
#52977=AXIS2_PLACEMENT_3D ( 'NONE', #24261, #41541, #63749 ) ;
#52979=LINE ( 'NONE', #43195, #37138 ) ;
#52986=FILL_AREA_STYLE_COLOUR ( '', #38710 ) ;
#52990=CARTESIAN_POINT ( 'NONE',  ( 93.67500000000001137, -207.7050326799711968, 84.89354166840095672 ) ) ;
#52991=CARTESIAN_POINT ( 'NONE',  ( 92.34999999999999432, 91.52997821335252127, 88.04208333333332348 ) ) ;
#52995=EDGE_CURVE ( 'NONE', #69189, #35387, #57792, .T. ) ;
#53001=CARTESIAN_POINT ( 'NONE',  ( 94.99999999999998579, 93.05995642670504253, 87.38062500173430180 ) ) ;
#53007=VECTOR ( 'NONE', #58376, 1000.000000000000000 ) ;
#53008=CARTESIAN_POINT ( 'NONE',  ( -92.34999999999999432, -209.9999999999999716, 75.07749999999998636 ) ) ;
#53015=CARTESIAN_POINT ( 'NONE',  ( -97.65000000000001990, 88.47002178664754979, 86.24291666666665890 ) ) ;
#53016=ORIENTED_EDGE ( 'NONE', *, *, #35414, .F. ) ;
#53022=CARTESIAN_POINT ( 'NONE',  ( -94.99999999999997158, -207.3369185715606307, 83.76906250086713612 ) ) ;
#53032=CARTESIAN_POINT ( 'NONE',  ( 97.64999999999999147, 90.00000000000002842, 82.77687500173431090 ) ) ;
#53034=CARTESIAN_POINT ( 'NONE',  ( -97.30629616937501680, 90.00000000000004263, 78.21281250086714465 ) ) ;
#53036=CARTESIAN_POINT ( 'NONE',  ( 96.32499999999998863, 87.70503267997126784, 76.24166666666666003 ) ) ;
#53046=CARTESIAN_POINT ( 'NONE',  ( -92.69370383062498320, -209.9999999999999716, 76.78406250086715090 ) ) ;
#53048=EDGE_CURVE ( 'NONE', #32074, #44409, #56052, .T. ) ;
#53052=ORIENTED_EDGE ( 'NONE', *, *, #27655, .T. ) ;
#53059=CARTESIAN_POINT ( 'NONE',  ( 96.32499999999998863, 87.70503267997126784, 83.30604166840096525 ) ) ;
#53061=EDGE_LOOP ( 'NONE', ( #28021, #8638 ) ) ;
#53062=CARTESIAN_POINT ( 'NONE',  ( -92.35000000000003695, 90.00000000000004263, 90.00000000000000000 ) ) ;
#53065=CARTESIAN_POINT ( 'NONE',  ( 95.00000000000000000, -207.3369185715606307, 84.40406250086714124 ) ) ;
#53066=CARTESIAN_POINT ( 'NONE',  ( 93.84685191531251292, -211.9973110713294489, 88.00239583420048461 ) ) ;
#53074=CARTESIAN_POINT ( 'NONE',  ( -95.00000000000002842, 92.66308142843932671, 80.11781250086714579 ) ) ;
#53078=ORIENTED_EDGE ( 'NONE', *, *, #72236, .F. ) ;
#53082=VERTEX_POINT ( 'NONE', #22044 ) ;
#53088=CARTESIAN_POINT ( 'NONE',  ( 97.30629616937498838, -209.9999999999999716, 82.97531250086714749 ) ) ;
#53095=CARTESIAN_POINT ( 'NONE',  ( -93.67499999999998295, -212.2949673200287179, 75.60666666666665492 ) ) ;
#53096=CARTESIAN_POINT ( 'NONE',  ( -97.64999999954989107, -210.0000310946949753, 88.81037122969127040 ) ) ;
#53098=CARTESIAN_POINT ( 'NONE',  ( -94.99999999999997158, -207.3369185715606307, 83.13406250086714522 ) ) ;
#53099=CARTESIAN_POINT ( 'NONE',  ( -95.00000000000002842, 87.33691857156074434, 82.97531250086716170 ) ) ;
#53102=CARTESIAN_POINT ( 'NONE',  ( 92.69370383062498320, 88.66845928578037217, 81.44072916753381719 ) ) ;
#53104=VERTEX_POINT ( 'NONE', #44987 ) ;
#53110=CARTESIAN_POINT ( 'NONE',  ( -92.69370383062498320, -211.3315407142195852, 84.82739583420048746 ) ) ;
#53112=CARTESIAN_POINT ( 'NONE',  ( -96.32499999999996021, -212.2949673200287179, 89.47083333333333144 ) ) ;
#53115=CARTESIAN_POINT ( 'NONE',  ( 96.32499999999997442, 92.29496732002878900, 80.26333333333332121 ) ) ;
#53116=ORIENTED_EDGE ( 'NONE', *, *, #73234, .T. ) ;
#53121=CARTESIAN_POINT ( 'NONE',  ( -97.30629616937501680, 88.66845928578038638, 89.06072916753379332 ) ) ;
#53127=CARTESIAN_POINT ( 'NONE',  ( -93.84685191531252713, 88.00268892867056536, 75.88447916753381151 ) ) ;
#53134=CARTESIAN_POINT ( 'NONE',  ( -93.84685191531248449, -208.0026889286704943, 87.04989583420048405 ) ) ;
#53135=EDGE_CURVE ( 'NONE', #29022, #70651, #59766, .T. ) ;
#53136=DIRECTION ( 'NONE',  ( -2.628368902995175337E-16, -1.000000000000000000, 0.000000000000000000 ) ) ;
#53138=CARTESIAN_POINT ( 'NONE',  ( 96.15314808468748708, 91.99731107132950569, 74.98489583420048632 ) ) ;
#53139=CARTESIAN_POINT ( 'NONE',  ( -93.33920801875063944, -211.6002412367801071, 74.80065669543250806 ) ) ;
#53141=VERTEX_POINT ( 'NONE', #68288 ) ;
#53145=CARTESIAN_POINT ( 'NONE',  ( -96.32500000000001705, 87.70503267997129626, 88.28020833506764120 ) ) ;
#53148=CARTESIAN_POINT ( 'NONE',  ( -97.30629616937501680, 90.00000000000004263, 75.83156250086716454 ) ) ;
#53149=CARTESIAN_POINT ( 'NONE',  ( 93.84685191531251292, -211.9973110713294489, 77.68364583420047609 ) ) ;
#53151=EDGE_LOOP ( 'NONE', ( #19663, #54577, #61009, #62985, #65752, #10057, #29827, #47231 ) ) ;
#53152=AXIS2_PLACEMENT_3D ( 'NONE', #66884, #15004, #60882 ) ;
#53158=EDGE_LOOP ( 'NONE', ( #40473, #23130, #69422, #13765 ) ) ;
#53165=ORIENTED_EDGE ( 'NONE', *, *, #41126, .T. ) ;
#53166=ORIENTED_EDGE ( 'NONE', *, *, #63704, .F. ) ;
#53168=ORIENTED_EDGE ( 'NONE', *, *, #33153, .T. ) ;
#53170=CARTESIAN_POINT ( 'NONE',  ( 93.84685191531248449, 88.00268892867053694, 78.47739583420049314 ) ) ;
#53172=CARTESIAN_POINT ( 'NONE',  ( 92.35000000000002274, -211.5299782133524502, 75.44791666666667140 ) ) ;
#53174=VERTEX_POINT ( 'NONE', #51350 ) ;
#53179=CARTESIAN_POINT ( 'NONE',  ( -97.65000000000000568, 88.47002178664756400, 87.51291666666666913 ) ) ;
#53180=CARTESIAN_POINT ( 'NONE',  ( -95.43397055421762332, 92.35870626171013953, 74.84690984288799598 ) ) ;
#53184=CARTESIAN_POINT ( 'NONE',  ( 93.67499999999998295, 92.29496732002878900, 77.82916666666665151 ) ) ;
#53185=CARTESIAN_POINT ( 'NONE',  ( -92.34999999999999432, -209.9999999999999716, 78.33187500173430351 ) ) ;
#53188=CARTESIAN_POINT ( 'NONE',  ( 97.64999999999999147, 90.00000000000002842, 74.52187500173430124 ) ) ;
#53189=CARTESIAN_POINT ( 'NONE',  ( -92.35000000000005116, 91.52997821335253548, 75.84479166840098685 ) ) ;
#53190=( BOUNDED_CURVE ( )  B_SPLINE_CURVE ( 2, ( #33222, #70388, #18892, #11767, #58021, #29429, #41470, #922, #46013 ),
 .UNSPECIFIED., .F., .F. ) 
 B_SPLINE_CURVE_WITH_KNOTS ( ( 3, 2, 2, 2, 3 ),
 ( 0.7620226289464459013, 0.7620226784152965838, 0.7690784439561786368, 0.7761342094970606897, 0.7831899741065915244 ),
 .UNSPECIFIED. ) 
 CURVE ( )  GEOMETRIC_REPRESENTATION_ITEM ( )  RATIONAL_B_SPLINE_CURVE ( ( 0.9999981213880242414, 0.9999990606874264998, 1.000000000000000000, 0.8660254037844387076, 1.000000000000000000, 0.8660254037844387076, 1.000000000000000000, 0.8660254037844387076, 1.000000000000000000 ) ) 
 REPRESENTATION_ITEM ( '' )  );
#53191=ORIENTED_EDGE ( 'NONE', *, *, #67931, .F. ) ;
#53192=CARTESIAN_POINT ( 'NONE',  ( 97.30629616937498838, 88.66845928578037217, 80.54114583420049200 ) ) ;
#53194=LINE ( 'NONE', #28779, #70299 ) ;
#53205=ADVANCED_FACE ( 'NONE', ( #636 ), #1383, .F. ) ;
#53212=CARTESIAN_POINT ( 'NONE',  ( -92.69370383062498320, -211.3315407142195852, 78.00114583420049996 ) ) ;
#53215=EDGE_CURVE ( 'NONE', #9807, #51953, #29516, .T. ) ;
#53226=CARTESIAN_POINT ( 'NONE',  ( 97.65000000000000568, 91.52997821335252127, 86.00479166840096923 ) ) ;
#53230=CARTESIAN_POINT ( 'NONE',  ( 97.30629616937498838, 88.66845928578035796, 82.44614583420049314 ) ) ;
#53231=CARTESIAN_POINT ( 'NONE',  ( -92.69370383062498320, -209.9999999999999716, 85.67406250086715147 ) ) ;
#53232=CARTESIAN_POINT ( 'NONE',  ( 97.64999999946594755, 90.00005320149050192, 78.96687695417308817 ) ) ;
#53235=CARTESIAN_POINT ( 'NONE',  ( -92.34999999999999432, -208.4700217866474645, 82.11541666666666117 ) ) ;
#53236=CARTESIAN_POINT ( 'NONE',  ( -95.00000000000002842, 92.66308142843932671, 77.41906250086714181 ) ) ;
#53237=CARTESIAN_POINT ( 'NONE',  ( 92.69370383062501162, -209.9999999999999716, 87.10281250086714522 ) ) ;
#53245=CARTESIAN_POINT ( 'NONE',  ( 93.67500000000001137, -212.2949673200287179, 75.50083333333331836 ) ) ;
#53251=CARTESIAN_POINT ( 'NONE',  ( 92.69370383062501162, -209.9999999999999716, 82.18156250086715886 ) ) ;
#53252=FACE_OUTER_BOUND ( 'NONE', #32429, .T. ) ;
#53258=CARTESIAN_POINT ( 'NONE',  ( 92.35000000000002274, -208.4700217866474645, 86.13708333333332234 ) ) ;
#53261=EDGE_LOOP ( 'NONE', ( #34988, #2180, #71833, #40497 ) ) ;
#53262=VECTOR ( 'NONE', #65337, 1000.000000000000000 ) ;
#53266=CARTESIAN_POINT ( 'NONE',  ( -95.00000000000002842, 92.66308142843932671, 89.00781250086716057 ) ) ;
#53267=DIRECTION ( 'NONE',  ( 1.000000000000000000, 0.000000000000000000, 0.000000000000000000 ) ) ;
#53269=CARTESIAN_POINT ( 'NONE',  ( 92.35000000000002274, -211.5299782133524502, 74.89229166840097207 ) ) ;
#53270=CARTESIAN_POINT ( 'NONE',  ( 97.64999999999999147, 90.00000000000002842, 76.98250000000000171 ) ) ;
#53272=CARTESIAN_POINT ( 'NONE',  ( -93.67499999999998295, -212.2949673200287179, 87.75104166840095843 ) ) ;
#53277=CARTESIAN_POINT ( 'NONE',  ( -92.35000000000003695, 90.00000000000004263, 86.58687500173429896 ) ) ;
#53278=CARTESIAN_POINT ( 'NONE',  ( 96.15314808468748708, 88.00268892867053694, 75.88447916753381151 ) ) ;
#53281=CARTESIAN_POINT ( 'NONE',  ( 2.500000000000031530, 80.00000000000000000, -90.00000000000000000 ) ) ;
#53282=CARTESIAN_POINT ( 'NONE',  ( -92.35000000018064270, -210.0000309433161476, 78.33187387208045038 ) ) ;
#53286=CARTESIAN_POINT ( 'NONE',  ( -97.65000000000001990, 90.00000000000004263, 79.83999999999998920 ) ) ;
#53295=CARTESIAN_POINT ( 'NONE',  ( -92.69370383062498320, -209.9999999999999716, 88.21406250086714351 ) ) ;
#53297=CARTESIAN_POINT ( 'NONE',  ( -94.99999999999997158, -213.0599564267049857, 82.53874999999999318 ) ) ;
#53306=CARTESIAN_POINT ( 'NONE',  ( 92.69370383062498320, 88.66845928578035796, 80.17072916753380696 ) ) ;
#53309=CARTESIAN_POINT ( 'NONE',  ( -97.65000000000001990, 90.00000000000004263, 85.55499999999999261 ) ) ;
#53312=CARTESIAN_POINT ( 'NONE',  ( 95.00000000000000000, -209.9999999999999716, 90.00000000000000000 ) ) ;
#53318=CARTESIAN_POINT ( 'NONE',  ( 97.64999999999999147, -209.9999999999999716, 86.50750000000000739 ) ) ;
#53320=CARTESIAN_POINT ( 'NONE',  ( -93.84685191531252713, 88.00268892867056536, 87.31447916753380412 ) ) ;
#53321=AXIS2_PLACEMENT_3D ( 'NONE', #47035, #63963, #6801 ) ;
#53332=CARTESIAN_POINT ( 'NONE',  ( 92.69370383062501162, -209.9999999999999716, 82.81656250086714977 ) ) ;
#53339=CARTESIAN_POINT ( 'NONE',  ( 93.84685191531251292, -211.9973110713294489, 76.41364583420048007 ) ) ;
#53341=CARTESIAN_POINT ( 'NONE',  ( 97.30629616937498838, -209.9999999999999716, 79.32406250086715715 ) ) ;
#53343=DIRECTION ( 'NONE',  ( -0.000000000000000000, -0.000000000000000000, 1.000000000000000000 ) ) ;
#53346=CARTESIAN_POINT ( 'NONE',  ( 96.32499999999998863, -207.7050326799711968, 86.69270833506763552 ) ) ;
#53351=CARTESIAN_POINT ( 'NONE',  ( 93.67500000000001137, -212.2949673200287179, 84.47020833506762472 ) ) ;
#53352=CARTESIAN_POINT ( 'NONE',  ( 96.32499999999997442, 92.29496732002878900, 89.78833333333332689 ) ) ;
#53353=ORIENTED_EDGE ( 'NONE', *, *, #13477, .F. ) ;
#53357=ORIENTED_EDGE ( 'NONE', *, *, #60046, .F. ) ;
#53359=CARTESIAN_POINT ( 'NONE',  ( -93.84685191531252713, 88.00268892867056536, 86.83822916753382515 ) ) ;
#53361=CARTESIAN_POINT ( 'NONE',  ( 93.84685191531248449, 91.99731107132950569, 86.36197916753381776 ) ) ;
#53363=CARTESIAN_POINT ( 'NONE',  ( 96.32499999999997442, 92.29496732002878900, 86.05770833506763040 ) ) ;
#53373=CARTESIAN_POINT ( 'NONE',  ( -92.35000000000002274, 90.00000000000004263, 75.00000000000000000 ) ) ;
#53374=EDGE_CURVE ( 'NONE', #19936, #44954, #29928, .T. ) ;
#53377=CARTESIAN_POINT ( 'NONE',  ( -92.35000000000005116, 88.47002178664754979, 85.18458333333332178 ) ) ;
#53379=ORIENTED_EDGE ( 'NONE', *, *, #26845, .F. ) ;
#53381=CIRCLE ( 'NONE', #42539, 3.299999999999997158 ) ;
#53382=CARTESIAN_POINT ( 'NONE',  ( 95.00000000000000000, -209.9999999999999716, 90.00000000000000000 ) ) ;
#53385=CARTESIAN_POINT ( 'NONE',  ( -96.15314808468747287, -208.0026889286704943, 81.91697916753381037 ) ) ;
#53399=CARTESIAN_POINT ( 'NONE',  ( -92.69370383062502583, 91.33154071421968467, 75.40822916753381833 ) ) ;
#53403=( BOUNDED_CURVE ( )  B_SPLINE_CURVE ( 2, ( #50161, #61840, #10323, #56193, #62974, #16337, #62595 ),
 .UNSPECIFIED., .F., .F. ) 
 B_SPLINE_CURVE_WITH_KNOTS ( ( 3, 2, 2, 3 ),
 ( 0.5503499107226622611, 0.5574054777297072771, 0.5644612432705896632, 0.5715170088666295944 ),
 .UNSPECIFIED. ) 
 CURVE ( )  GEOMETRIC_REPRESENTATION_ITEM ( )  RATIONAL_B_SPLINE_CURVE ( ( 0.9999924607068835236, 0.8660291735370695410, 1.000000000000000000, 0.8660254037844387076, 1.000000000000000000, 0.8660254037844387076, 1.000000000000000000 ) ) 
 REPRESENTATION_ITEM ( '' )  );
#53412=CARTESIAN_POINT ( 'NONE',  ( -94.99999999999997158, -207.3369185715606307, 76.94281250086714863 ) ) ;
#53413=CYLINDRICAL_SURFACE ( 'NONE', #72206, 3.299999999999969624 ) ;
#53416=VECTOR ( 'NONE', #32, 1000.000000000000114 ) ;
#53427=ORIENTED_EDGE ( 'NONE', *, *, #16114, .F. ) ;
#53428=CARTESIAN_POINT ( 'NONE',  ( 96.15314808468750130, -211.9973110713294489, 84.77447916753381207 ) ) ;
#53433=ORIENTED_EDGE ( 'NONE', *, *, #35414, .T. ) ;
#53436=CARTESIAN_POINT ( 'NONE',  ( -93.84685191531252713, 88.00268892867056536, 79.21822916753382060 ) ) ;
#53439=ORIENTED_EDGE ( 'NONE', *, *, #68628, .T. ) ;
#53441=ORIENTED_EDGE ( 'NONE', *, *, #29877, .F. ) ;
#53448=ORIENTED_EDGE ( 'NONE', *, *, #31911, .F. ) ;
#53452=CARTESIAN_POINT ( 'NONE',  ( 95.00000000000000000, -212.6630814284392557, 77.10156250086711793 ) ) ;
#53456=CARTESIAN_POINT ( 'NONE',  ( -97.64995850909662067, -211.5300021681366047, 85.68729332542763188 ) ) ;
#53465=CARTESIAN_POINT ( 'NONE',  ( -93.84685191531247028, -211.9973110713294489, 80.32947916753380468 ) ) ;
#53466=CARTESIAN_POINT ( 'NONE',  ( -92.69370383062502583, 91.33154071421968467, 81.91697916753381037 ) ) ;
#53468=CARTESIAN_POINT ( 'NONE',  ( 96.15314808468748708, 91.99731107132950569, 82.44614583420046472 ) ) ;
#53477=CARTESIAN_POINT ( 'NONE',  ( -2.500000000000012879, -65.00000000000000000, -90.00000000000000000 ) ) ;
#53478=CARTESIAN_POINT ( 'NONE',  ( -94.99999999999997158, -212.6630814284392557, 82.18156250086715886 ) ) ;
#53480=CARTESIAN_POINT ( 'NONE',  ( -92.34999999999996589, -211.5299782133524502, 89.62958333333334338 ) ) ;
#53483=DIRECTION ( 'NONE',  ( -0.000000000000000000, -0.000000000000000000, 1.000000000000000000 ) ) ;
#53487=LINE ( 'NONE', #14371, #25472 ) ;
#53489=CARTESIAN_POINT ( 'NONE',  ( -92.69370383062502583, 88.66845928578038638, 84.19239583420046813 ) ) ;
#53491=DIRECTION ( 'NONE',  ( -0.000000000000000000, -0.000000000000000000, -1.000000000000000000 ) ) ;
#53496=CARTESIAN_POINT ( 'NONE',  ( -93.84685191531254134, 91.99731107132950569, 74.82614583420047438 ) ) ;
#53501=DIRECTION ( 'NONE',  ( -0.000000000000000000, -0.000000000000000000, -1.000000000000000000 ) ) ;
#53505=CARTESIAN_POINT ( 'NONE',  ( -96.15314808468745866, -211.9973110713294489, 85.46239583420047836 ) ) ;
#53509=CARTESIAN_POINT ( 'NONE',  ( -92.69370383062498320, -209.9999999999999716, 76.78406250086715090 ) ) ;
#53512=CARTESIAN_POINT ( 'NONE',  ( -94.99999999999997158, -213.0599564267049857, 81.98312500173430806 ) ) ;
#53516=CARTESIAN_POINT ( 'NONE',  ( 95.00000000000000000, -212.6630814284392557, 77.10156250086711793 ) ) ;
#53531=DIRECTION ( 'NONE',  ( 0.000000000000000000, 0.000000000000000000, 1.000000000000000000 ) ) ;
#53533=VECTOR ( 'NONE', #34716, 1000.000000000000000 ) ;
#53536=CARTESIAN_POINT ( 'NONE',  ( 92.69370383062498320, 91.33154071421968467, 80.22364583420048234 ) ) ;
#53537=CARTESIAN_POINT ( 'NONE',  ( -96.32500000000001705, 87.70503267997129626, 81.29520833506762756 ) ) ;
#53541=ORIENTED_EDGE ( 'NONE', *, *, #10382, .T. ) ;
#53548=CARTESIAN_POINT ( 'NONE',  ( -94.00680085345865677, 92.13398380010822564, 74.81432998548486069 ) ) ;
#53551=CYLINDRICAL_SURFACE ( 'NONE', #43260, 2.649999999999985700 ) ;
#53554=CARTESIAN_POINT ( 'NONE',  ( -92.34999999999999432, -211.5299782133524502, 79.54895833506762415 ) ) ;
#53555=DIRECTION ( 'NONE',  ( -0.000000000000000000, -0.000000000000000000, 1.000000000000000000 ) ) ;
#53556=CARTESIAN_POINT ( 'NONE',  ( 93.67499999999998295, 92.29496732002878900, 76.00354166840097037 ) ) ;
#53557=CARTESIAN_POINT ( 'NONE',  ( -92.35000000000005116, 88.47002178664754979, 76.37395833506761278 ) ) ;
#53559=CARTESIAN_POINT ( 'NONE',  ( 97.30629616937498838, 91.33154071421968467, 75.56697916753383026 ) ) ;
#53573=CARTESIAN_POINT ( 'NONE',  ( 97.64999999999993463, -208.4700217866474077, 81.48041666666665606 ) ) ;
#53575=CARTESIAN_POINT ( 'NONE',  ( -0.0004442498525516064278, 0.001194404164626844313, -64.00000000000000000 ) ) ;
#53576=CARTESIAN_POINT ( 'NONE',  ( -92.69370383062498320, -208.6684592857803011, 76.83697916753382628 ) ) ;
#53579=DIRECTION ( 'NONE',  ( -0.000000000000000000, -0.000000000000000000, 1.000000000000000000 ) ) ;
#53591=DIRECTION ( 'NONE',  ( -1.000000000000000000, 3.061616997868383141E-16, -0.000000000000000000 ) ) ;
#53594=CARTESIAN_POINT ( 'NONE',  ( 94.99999999999998579, 92.66308142843932671, 84.56281250086716739 ) ) ;
#53595=CARTESIAN_POINT ( 'NONE',  ( -92.69370383062498320, -209.9999999999999716, 85.03906250086714635 ) ) ;
#53599=CARTESIAN_POINT ( 'NONE',  ( -93.67499999999998295, -207.7050326799711968, 80.26333333333332121 ) ) ;
#53600=CARTESIAN_POINT ( 'NONE',  ( -97.30629616937501680, 90.00000000000004263, 75.67281250086713840 ) ) ;
#53601=CARTESIAN_POINT ( 'NONE',  ( 97.30629616937498838, -209.9999999999999716, 86.15031250086714465 ) ) ;
#53612=CARTESIAN_POINT ( 'NONE',  ( 92.69370383062501162, -209.9999999999999716, 79.00656250086716170 ) ) ;
#53613=CARTESIAN_POINT ( 'NONE',  ( -94.99999999999997158, -206.9400435732949575, 80.95125000000000171 ) ) ;
#53616=( BOUNDED_CURVE ( )  B_SPLINE_CURVE ( 2, ( #58206, #36750, #48402, #18346, #6708, #41648, #48037 ),
 .UNSPECIFIED., .F., .F. ) 
 B_SPLINE_CURVE_WITH_KNOTS ( ( 3, 2, 2, 3 ),
 ( 0.5926843883797354717, 0.5997400709749998171, 0.6067958365158829803, 0.6138516023186938453 ),
 .UNSPECIFIED. ) 
 CURVE ( )  GEOMETRIC_REPRESENTATION_ITEM ( )  RATIONAL_B_SPLINE_CURVE ( ( 0.9999968501007930888, 0.8660269787525570750, 1.000000000000000000, 0.8660254037844387076, 1.000000000000000000, 0.8660254037844387076, 1.000000000000000000 ) ) 
 REPRESENTATION_ITEM ( '' )  );
#53620=CARTESIAN_POINT ( 'NONE',  ( 93.67500000000001137, -207.7050326799711968, 84.81416666666666515 ) ) ;
#53628=CARTESIAN_POINT ( 'NONE',  ( -92.35000000000000853, -210.0000001051137701, 86.58687499784845443 ) ) ;
#53630=CARTESIAN_POINT ( 'NONE',  ( -97.30629616937501680, 88.66845928578038638, 83.50447916753383026 ) ) ;
#53631=VECTOR ( 'NONE', #41455, 1000.000000000000000 ) ;
#53636=CARTESIAN_POINT ( 'NONE',  ( 97.30629616937498838, -208.6684592857803011, 87.47322916753381605 ) ) ;
#53637=CARTESIAN_POINT ( 'NONE',  ( 93.67499999999998295, 92.29496732002878900, 76.55916666666666970 ) ) ;
#53639=ORIENTED_EDGE ( 'NONE', *, *, #32771, .T. ) ;
#53642=CARTESIAN_POINT ( 'NONE',  ( -92.35000000000002274, -211.5299782133524786, 85.18458333333332178 ) ) ;
#53644=VERTEX_POINT ( 'NONE', #22647 ) ;
#53645=CARTESIAN_POINT ( 'NONE',  ( -97.65000000000001990, 90.00000000000004263, 86.26937500173430351 ) ) ;
#53647=CARTESIAN_POINT ( 'NONE',  ( 96.15314808468748708, 91.99731107132950569, 85.77989583420048803 ) ) ;
#53650=CARTESIAN_POINT ( 'NONE',  ( -92.34999999999999432, -209.9999999999999716, 78.33187500173430351 ) ) ;
#53652=ORIENTED_EDGE ( 'NONE', *, *, #32179, .F. ) ;
#53653=DIRECTION ( 'NONE',  ( -0.000000000000000000, -0.000000000000000000, 1.000000000000000000 ) ) ;
#53657=ORIENTED_EDGE ( 'NONE', *, *, #6785, .T. ) ;
#53663=CARTESIAN_POINT ( 'NONE',  ( -97.64999999994218172, 89.99998877583867340, 75.47473230081648410 ) ) ;
#53664=CARTESIAN_POINT ( 'NONE',  ( -96.15314808468745866, -211.9973110713294489, 88.63739583420048973 ) ) ;
#53665=ORIENTED_EDGE ( 'NONE', *, *, #15302, .F. ) ;
#53667=VERTEX_POINT ( 'NONE', #63249 ) ;
#53672=CARTESIAN_POINT ( 'NONE',  ( 96.15314808468748708, 91.99731107132950569, 82.44614583420046472 ) ) ;
#53675=CARTESIAN_POINT ( 'NONE',  ( -96.32500000000001705, 92.29496732002878900, 81.00416666666666288 ) ) ;
#53678=CARTESIAN_POINT ( 'NONE',  ( 2.499999999999983569, -80.00000000000000000, -90.00000000000000000 ) ) ;
#53683=ORIENTED_EDGE ( 'NONE', *, *, #1325, .F. ) ;
#53684=CARTESIAN_POINT ( 'NONE',  ( -96.15314808468752972, 91.99731107132950569, 86.99697916753380866 ) ) ;
#53687=AXIS2_PLACEMENT_3D ( 'NONE', #61459, #9941, #54698 ) ;
#53688=CARTESIAN_POINT ( 'NONE',  ( 97.64999999999999147, 90.00000000000002842, 90.00000000000000000 ) ) ;
#53693=CARTESIAN_POINT ( 'NONE',  ( 92.35000000000000853, -209.9999999999999716, 77.93499999999998806 ) ) ;
#53696=CARTESIAN_POINT ( 'NONE',  ( 95.00000000000000000, -207.3369185715606307, 81.38781250086715602 ) ) ;
#53708=CARTESIAN_POINT ( 'NONE',  ( 97.30629616937498838, -211.3315407142195852, 80.54114583420049200 ) ) ;
#53709=EDGE_CURVE ( 'NONE', #48987, #41411, #29012, .T. ) ;
#53717=LINE ( 'NONE', #13120, #5345 ) ;
#53718=CARTESIAN_POINT ( 'NONE',  ( 93.67500000000001137, -212.2949673200287179, 83.83520833506763381 ) ) ;
#53719=CARTESIAN_POINT ( 'NONE',  ( 93.67499999999998295, 92.29496732002878900, 84.17916666666666003 ) ) ;
#53725=CARTESIAN_POINT ( 'NONE',  ( -97.30629616937501680, 90.00000000000004263, 87.89656250086714806 ) ) ;
#53728=CARTESIAN_POINT ( 'NONE',  ( 97.30629616937498838, 88.66845928578037217, 85.46239583420047836 ) ) ;
#53731=CARTESIAN_POINT ( 'NONE',  ( 92.34999999999999432, 91.52997821335252127, 87.48645833506763836 ) ) ;
#53741=CARTESIAN_POINT ( 'NONE',  ( -96.32500000000001705, 92.29496732002878900, 83.54416666666666913 ) ) ;
#53742=ADVANCED_FACE ( 'NONE', ( #57230 ), #16629, .F. ) ;
#53745=CARTESIAN_POINT ( 'NONE',  ( 96.92110976540138267, 91.30563282057313756, 74.79348190356853365 ) ) ;
#53746=FACE_OUTER_BOUND ( 'NONE', #44369, .T. ) ;
#53749=CARTESIAN_POINT ( 'NONE',  ( -94.99999999999997158, -212.6630814284392557, 83.45156250086714067 ) ) ;
#53760=CARTESIAN_POINT ( 'NONE',  ( -94.99999999999997158, -206.9400435732949575, 89.84125000000000227 ) ) ;
#53764=CARTESIAN_POINT ( 'NONE',  ( -95.00000000000002842, 87.33691857156074434, 75.19656250086714522 ) ) ;
#53773=CARTESIAN_POINT ( 'NONE',  ( -96.32499999999996021, -207.7050326799711968, 86.71916666666666629 ) ) ;
#53778=CARTESIAN_POINT ( 'NONE',  ( 93.67500000000001137, -212.2949673200287179, 78.12020833506763040 ) ) ;
#53786=EDGE_CURVE ( 'NONE', #40782, #11821, #34735, .T. ) ;
#53792=CARTESIAN_POINT ( 'NONE',  ( 96.15314808468750130, -211.9973110713294489, 86.04447916753380809 ) ) ;
#53793=CARTESIAN_POINT ( 'NONE',  ( 96.15314808468750130, -211.9973110713294489, 88.10822916753382117 ) ) ;
#53800=CARTESIAN_POINT ( 'NONE',  ( -95.00000000000002842, 87.33691857156074434, 78.53031250086715431 ) ) ;
#53811=CYLINDRICAL_SURFACE ( 'NONE', #49028, 2.649999999999999467 ) ;
#53819=CARTESIAN_POINT ( 'NONE',  ( 97.30629616937498838, -211.3315407142195852, 77.84239583420045960 ) ) ;
#53820=CARTESIAN_POINT ( 'NONE',  ( -99.99999999999997158, -214.9999999999999716, 90.00000000000000000 ) ) ;
#53822=LINE ( 'NONE', #41802, #10152 ) ;
#53829=CARTESIAN_POINT ( 'NONE',  ( -92.69370383062498320, -211.3315407142195852, 81.01739583420048518 ) ) ;
#53830=CARTESIAN_POINT ( 'NONE',  ( -92.69370383062502583, 88.66845928578038638, 79.90614583420048689 ) ) ;
#53834=CARTESIAN_POINT ( 'NONE',  ( 92.69370383062498320, 91.33154071421968467, 80.69989583420048973 ) ) ;
#53835=( BOUNDED_CURVE ( )  B_SPLINE_CURVE ( 2, ( #29652, #53, #17285, #18381, #22944, #23305, #46233 ),
 .UNSPECIFIED., .F., .F. ) 
 B_SPLINE_CURVE_WITH_KNOTS ( ( 3, 2, 2, 3 ),
 ( 0.1041666666666670182, 0.1111111111111114103, 0.1180555555555558161, 0.1250000000000002220 ),
 .UNSPECIFIED. ) 
 CURVE ( )  GEOMETRIC_REPRESENTATION_ITEM ( )  RATIONAL_B_SPLINE_CURVE ( ( 0.9999999999999933387, 0.8660254037844453689, 1.000000000000000000, 0.8660254037844387076, 1.000000000000000000, 0.8660254037844343777, 1.000000000000004219 ) ) 
 REPRESENTATION_ITEM ( '' )  );
#53842=CARTESIAN_POINT ( 'NONE',  ( -97.30629616937497417, -211.3315407142195852, 83.34572916753381833 ) ) ;
#53844=VECTOR ( 'NONE', #1399, 1000.000000000000000 ) ;
#53853=CARTESIAN_POINT ( 'NONE',  ( -95.00000000000002842, 93.05995642670501411, 75.23624999999999829 ) ) ;
#53855=CARTESIAN_POINT ( 'NONE',  ( -97.30629616937501680, 90.00000000000004263, 83.92781250086714806 ) ) ;
#53860=CARTESIAN_POINT ( 'NONE',  ( -97.30629616937501680, 88.66845928578038638, 75.09072916753382287 ) ) ;
#53868=CARTESIAN_POINT ( 'NONE',  ( -96.15314808468747287, -208.0026889286704943, 83.34572916753383254 ) ) ;
#53873=ADVANCED_FACE ( 'NONE', ( #12462 ), #34281, .F. ) ;
#53875=CARTESIAN_POINT ( 'NONE',  ( 2.500000000000004441, -90.00000000000000000, -279.9999999999999432 ) ) ;
#53877=CARTESIAN_POINT ( 'NONE',  ( -93.84685191531248449, -208.0026889286704943, 76.25489583420049655 ) ) ;
#53886=CARTESIAN_POINT ( 'NONE',  ( 93.84685191531249870, -208.0026889286704943, 89.06072916753382174 ) ) ;
#53899=PLANE ( 'NONE',  #29816 ) ;
#53905=DIRECTION ( 'NONE',  ( 1.000000000000000000, 0.000000000000000000, 0.000000000000000000 ) ) ;
#53909=CARTESIAN_POINT ( 'NONE',  ( 93.84685191531248449, 88.00268892867053694, 80.38239583420048007 ) ) ;
#53910=FACE_OUTER_BOUND ( 'NONE', #5601, .T. ) ;
#53911=EDGE_CURVE ( 'NONE', #55837, #5520, #70073, .T. ) ;
#53916=ORIENTED_EDGE ( 'NONE', *, *, #34135, .F. ) ;
#53921=ADVANCED_FACE ( 'NONE', ( #18577 ), #40790, .F. ) ;
#53922=VECTOR ( 'NONE', #1596, 1000.000000000000000 ) ;
#53933=CARTESIAN_POINT ( 'NONE',  ( -92.34999999999999432, -209.9999999999999716, 74.52187500173430124 ) ) ;
#53936=CARTESIAN_POINT ( 'NONE',  ( 96.32499999999998863, 87.70503267997126784, 76.95604166840095672 ) ) ;
#53937=CARTESIAN_POINT ( 'NONE',  ( -95.00000000000002842, 93.05995642670501411, 76.58562500173430010 ) ) ;
#53940=CARTESIAN_POINT ( 'NONE',  ( 96.15314808468748708, 88.00268892867053694, 76.67822916753381435 ) ) ;
#53941=CARTESIAN_POINT ( 'NONE',  ( 92.34999999999999432, 91.52997821335252127, 82.32708333333334849 ) ) ;
#53951=EDGE_LOOP ( 'NONE', ( #52076, #30507, #47892, #40567 ) ) ;
#53954=CARTESIAN_POINT ( 'NONE',  ( 92.35000000000000853, -209.9999999999999716, 83.01499999999998636 ) ) ;
#53958=CARTESIAN_POINT ( 'NONE',  ( -97.30629616937497417, -208.6684592857803011, 75.14364583420049826 ) ) ;
#53961=VECTOR ( 'NONE', #27248, 1000.000000000000000 ) ;
#53967=CARTESIAN_POINT ( 'NONE',  ( -92.35000000000000853, -210.0000001051137701, 86.58687499784845443 ) ) ;
#53973=CARTESIAN_POINT ( 'NONE',  ( 96.15314808468748708, 88.00268892867053694, 84.29822916753381890 ) ) ;
#53974=CARTESIAN_POINT ( 'NONE',  ( -97.30629616937497417, -211.3315407142195852, 87.94947916753382344 ) ) ;
#53979=CARTESIAN_POINT ( 'NONE',  ( -92.34999999999999432, -211.5299782133524502, 82.00958333333332462 ) ) ;
#53981=CARTESIAN_POINT ( 'NONE',  ( -93.84685191531252713, 88.00268892867056536, 76.51947916753380241 ) ) ;
#53987=AXIS2_PLACEMENT_3D ( 'NONE', #33728, #22453, #40475 ) ;
#53988=EDGE_CURVE ( 'NONE', #23400, #57437, #67451, .T. ) ;
#53989=CARTESIAN_POINT ( 'NONE',  ( 93.84685191531249870, -208.0026889286704943, 85.09197916753380753 ) ) ;
#53995=EDGE_CURVE ( 'NONE', #22794, #58538, #31861, .T. ) ;
#53996=ORIENTED_EDGE ( 'NONE', *, *, #1091, .F. ) ;
#53999=CARTESIAN_POINT ( 'NONE',  ( 92.69370383062501162, -209.9999999999999716, 79.64156250086715261 ) ) ;
#54004=CYLINDRICAL_SURFACE ( 'NONE', #67000, 2.649999999999985700 ) ;
#54005=CARTESIAN_POINT ( 'NONE',  ( 97.64999999999999147, -209.9999999999999716, 80.15749999999999886 ) ) ;
#54013=EDGE_CURVE ( 'NONE', #13090, #9512, #43392, .T. ) ;
#54015=CARTESIAN_POINT ( 'NONE',  ( -97.30629616937501680, 90.00000000000004263, 84.08656250086716000 ) ) ;
#54016=CARTESIAN_POINT ( 'NONE',  ( -97.64999999999996305, -209.9999999999999716, 77.29999999999999716 ) ) ;
#54019=CARTESIAN_POINT ( 'NONE',  ( 93.67499999999998295, 92.29496732002878900, 75.92416666666666458 ) ) ;
#54021=CARTESIAN_POINT ( 'NONE',  ( -97.64999999999996305, -209.9999999999999716, 84.99937500173429328 ) ) ;
#54025=CARTESIAN_POINT ( 'NONE',  ( -93.67500000000003979, 92.29496732002878900, 87.32770833506762642 ) ) ;
#54026=CARTESIAN_POINT ( 'NONE',  ( 97.30629616937498838, 90.00000000000002842, 86.30906250086715659 ) ) ;
#54035=AXIS2_PLACEMENT_3D ( 'NONE', #44119, #27179, #38485 ) ;
#54040=PLANE ( 'NONE',  #62583 ) ;
#54043=CARTESIAN_POINT ( 'NONE',  ( -94.99999999999997158, -209.9999999999999716, 90.00000000000000000 ) ) ;
#54044=CARTESIAN_POINT ( 'NONE',  ( -92.69370383062498320, -208.6684592857803011, 83.82197916753382572 ) ) ;
#54049=DIRECTION ( 'NONE',  ( -0.000000000000000000, -0.000000000000000000, 1.000000000000000000 ) ) ;
#54050=CARTESIAN_POINT ( 'NONE',  ( 96.15314808468748708, 88.00268892867053694, 88.74322916753382628 ) ) ;
#54052=CARTESIAN_POINT ( 'NONE',  ( 93.84685191531248449, 88.00268892867053694, 82.76364583420047438 ) ) ;
#54066=CARTESIAN_POINT ( 'NONE',  ( -93.84685191531254134, 91.99731107132950569, 86.25614583420048120 ) ) ;
#54080=CIRCLE ( 'NONE', #21661, 12.74999999999999822 ) ;
#54081=CARTESIAN_POINT ( 'NONE',  ( 93.84685191531249870, -208.0026889286704943, 80.80572916753382628 ) ) ;
#54094=CARTESIAN_POINT ( 'NONE',  ( 97.30629616937498838, -211.3315407142195852, 75.46114583420049371 ) ) ;
#54102=CARTESIAN_POINT ( 'NONE',  ( -92.35000000000003695, 90.00000000000004263, 82.69749999999999091 ) ) ;
#54105=CARTESIAN_POINT ( 'NONE',  ( 92.35000000000002274, -208.4700217866474645, 84.31145833506762699 ) ) ;
#54106=CARTESIAN_POINT ( 'NONE',  ( 92.34999999999999432, 88.47002178664753558, 83.70291666666668107 ) ) ;
#54112=CARTESIAN_POINT ( 'NONE',  ( -95.00000000000002842, 87.33691857156074434, 86.78531250086713555 ) ) ;
#54113=CARTESIAN_POINT ( 'NONE',  ( 92.69370383062498320, 91.33154071421968467, 80.69989583420048973 ) ) ;
#54115=CARTESIAN_POINT ( 'NONE',  ( 96.32499999999997442, 92.29496732002878900, 82.88270833506763324 ) ) ;
#54122=ORIENTED_EDGE ( 'NONE', *, *, #39482, .T. ) ;
#54123=ORIENTED_EDGE ( 'NONE', *, *, #30213, .T. ) ;
#54124=DIRECTION ( 'NONE',  ( -1.000000000000000000, 0.000000000000000000, 0.000000000000000000 ) ) ;
#54126=CARTESIAN_POINT ( 'NONE',  ( -92.35000000000003695, 90.00000000000004263, 83.96750000000000114 ) ) ;
#54128=CARTESIAN_POINT ( 'NONE',  ( 97.64999999999999147, 90.00000000000002842, 82.06250000000000000 ) ) ;
#54132=CARTESIAN_POINT ( 'NONE',  ( -94.99999999999997158, -207.3369185715606307, 81.22906250086715829 ) ) ;
#54139=CARTESIAN_POINT ( 'NONE',  ( 92.35000000000000853, -209.9999999999999716, 83.72937500173429726 ) ) ;
#54146=CARTESIAN_POINT ( 'NONE',  ( 97.64999999999999147, 89.99999413691126904, 82.77687479895028844 ) ) ;
#54148=CARTESIAN_POINT ( 'NONE',  ( -93.84685191531254134, 91.99731107132950569, 76.73114583420047552 ) ) ;
#54151=ADVANCED_FACE ( 'NONE', ( #68152 ), #68538, .F. ) ;
#54154=CARTESIAN_POINT ( 'NONE',  ( 92.35000000000000853, -209.9999999999999716, 90.00000000000000000 ) ) ;
#54162=CARTESIAN_POINT ( 'NONE',  ( -97.64999999999994884, -211.5299782133524502, 88.78291666666667936 ) ) ;
#54174=ORIENTED_EDGE ( 'NONE', *, *, #21571, .F. ) ;
#54180=CARTESIAN_POINT ( 'NONE',  ( 92.69370383062501162, -211.3315407142195852, 80.80572916753379786 ) ) ;
#54188=CARTESIAN_POINT ( 'NONE',  ( -97.30629616937501680, 88.66845928578038638, 75.88447916753382572 ) ) ;
#54196=CARTESIAN_POINT ( 'NONE',  ( 92.35000000003287823, -209.9999916080746516, 86.90410584365268676 ) ) ;
#54198=CARTESIAN_POINT ( 'NONE',  ( 0.000000000000000000, 0.000000000000000000, -310.0000000000000000 ) ) ;
#54204=CARTESIAN_POINT ( 'NONE',  ( 93.84685191531251292, -211.9973110713294489, 78.31864583420048120 ) ) ;
#54207=CARTESIAN_POINT ( 'NONE',  ( -97.65000000000001990, 90.00000000000004263, 88.09499999999999886 ) ) ;
#54209=LINE ( 'NONE', #13601, #37675 ) ;
#54213=CARTESIAN_POINT ( 'NONE',  ( -97.64999999999996305, -208.4700217866474645, 88.75645833506762017 ) ) ;
#54215=CARTESIAN_POINT ( 'NONE',  ( -94.99999999999997158, -212.6630814284392557, 82.18156250086714465 ) ) ;
#54216=CARTESIAN_POINT ( 'NONE',  ( -97.30629616937501680, 90.00000000000004263, 77.73656250086715147 ) ) ;
#54219=CARTESIAN_POINT ( 'NONE',  ( 94.99999999999998579, 87.33691857156068750, 82.18156250086714465 ) ) ;
#54223=CARTESIAN_POINT ( 'NONE',  ( -93.67499999999998295, -212.2949673200287179, 76.87666666666666515 ) ) ;
#54226=CARTESIAN_POINT ( 'NONE',  ( -94.99999999999997158, -212.6630814284392557, 82.81656250086712134 ) ) ;
#54240=CARTESIAN_POINT ( 'NONE',  ( -95.00000000000002842, 92.66308142843932671, 83.76906250086713612 ) ) ;
#54241=CARTESIAN_POINT ( 'NONE',  ( -96.01774234934295293, -207.8046129959941197, 74.85985921673513133 ) ) ;
#54245=CARTESIAN_POINT ( 'NONE',  ( -92.69370383062502583, 91.33154071421968467, 74.77322916753379900 ) ) ;
#54252=CARTESIAN_POINT ( 'NONE',  ( 93.67500000000001137, -207.7050326799711968, 84.81416666666666515 ) ) ;
#54254=CARTESIAN_POINT ( 'NONE',  ( -97.30629616937495996, -209.9999999999999716, 82.18156250086715886 ) ) ;
#54265=CARTESIAN_POINT ( 'NONE',  ( 97.30629616937498838, -211.3315407142195852, 89.43114583420049257 ) ) ;
#54276=FACE_OUTER_BOUND ( 'NONE', #48723, .T. ) ;
#54278=ORIENTED_EDGE ( 'NONE', *, *, #49162, .T. ) ;
#54285=( BOUNDED_CURVE ( )  B_SPLINE_CURVE ( 2, ( #67189, #73190, #67563, #37884, #26211, #60814, #15686 ),
 .UNSPECIFIED., .F., .F. ) 
 B_SPLINE_CURVE_WITH_KNOTS ( ( 3, 2, 2, 3 ),
 ( 0.7408554641864648627, 0.7479111473335299243, 0.7549669128744133095, 0.7620226289464454572 ),
 .UNSPECIFIED. ) 
 CURVE ( )  GEOMETRIC_REPRESENTATION_ITEM ( )  RATIONAL_B_SPLINE_CURVE ( ( 0.9999968710554256734, 0.8660269682749952569, 1.000000000000000000, 0.8660254037844387076, 1.000000000000000000, 0.8660263430970250864, 0.9999981213879984843 ) ) 
 REPRESENTATION_ITEM ( '' )  );
#54286=CARTESIAN_POINT ( 'NONE',  ( 92.69370383062498320, 90.00000000000002842, 80.91156250086716284 ) ) ;
#54287=FACE_BOUND ( 'NONE', #42158, .T. ) ;
#54291=VERTEX_POINT ( 'NONE', #1533 ) ;
#54299=CARTESIAN_POINT ( 'NONE',  ( 92.35000000003357457, 89.99999234487445676, 78.01464417100922333 ) ) ;
#54301=CARTESIAN_POINT ( 'NONE',  ( -96.32500000000001705, 87.70503267997129626, 78.04083333333333883 ) ) ;
#54303=CARTESIAN_POINT ( 'NONE',  ( -97.64999999999994884, -211.5299782133524502, 75.52729166840099140 ) ) ;
#54304=CARTESIAN_POINT ( 'NONE',  ( -95.00000000000002842, 87.33691857156074434, 88.69031250086716511 ) ) ;
#54306=CARTESIAN_POINT ( 'NONE',  ( 93.67499999999999716, 87.70503267997126784, 75.58020833506763836 ) ) ;
#54307=CARTESIAN_POINT ( 'NONE',  ( -93.67500000000003979, 92.29496732002878900, 77.80270833506763495 ) ) ;
#54309=CARTESIAN_POINT ( 'NONE',  ( 97.30629616937498838, 90.00000000000002842, 76.14906250086716000 ) ) ;
#54314=EDGE_LOOP ( 'NONE', ( #55141, #59983, #10924, #38476 ) ) ;
#54316=CARTESIAN_POINT ( 'NONE',  ( 92.35000000000000853, -209.9999999999999716, 89.36499999999999488 ) ) ;
#54318=EDGE_CURVE ( 'NONE', #5972, #37629, #31424, .T. ) ;
#54326=CARTESIAN_POINT ( 'NONE',  ( -94.99999999999997158, -207.3369185715606307, 75.67281250086716682 ) ) ;
#54335=CARTESIAN_POINT ( 'NONE',  ( 95.00000000000000000, -206.9400435732949575, 80.39562500173430237 ) ) ;
#54337=LINE ( 'NONE', #26118, #22996 ) ;
#54341=EDGE_CURVE ( 'NONE', #69810, #44748, #24063, .T. ) ;
#54344=CARTESIAN_POINT ( 'NONE',  ( 93.84685191531248449, 91.99731107132950569, 84.61572916753381435 ) ) ;
#54345=CARTESIAN_POINT ( 'NONE',  ( -97.30629616937497417, -211.3315407142195852, 83.50447916753383026 ) ) ;
#54349=CARTESIAN_POINT ( 'NONE',  ( -97.64999999999996305, -209.9999999999999716, 77.29999999999999716 ) ) ;
#54353=CARTESIAN_POINT ( 'NONE',  ( 97.30629616937498838, -209.9999999999999716, 82.97531250086714749 ) ) ;
#54355=EDGE_CURVE ( 'NONE', #7925, #15992, #47713, .T. ) ;
#54357=VERTEX_POINT ( 'NONE', #9333 ) ;
#54362=CARTESIAN_POINT ( 'NONE',  ( 92.69370383062501162, -211.3315407142195852, 78.42447916753380355 ) ) ;
#54368=CARTESIAN_POINT ( 'NONE',  ( 96.32499999999998863, -207.7050326799711968, 82.16833333333332234 ) ) ;
#54372=VERTEX_POINT ( 'NONE', #33004 ) ;
#54373=CARTESIAN_POINT ( 'NONE',  ( -96.32499999999996021, -212.2949673200287179, 86.37520833506764006 ) ) ;
#54375=CARTESIAN_POINT ( 'NONE',  ( -92.69370383062502583, 91.33154071421968467, 82.55197916753382970 ) ) ;
#54376=DIRECTION ( 'NONE',  ( 0.000000000000000000, 0.000000000000000000, 1.000000000000000000 ) ) ;
#54381=CARTESIAN_POINT ( 'NONE',  ( -92.34999999999999432, -209.9999999999999716, 84.68187500173429783 ) ) ;
#54385=CARTESIAN_POINT ( 'NONE',  ( -92.35000000000003695, 90.00000000000004263, 87.85687500173429498 ) ) ;
#54386=AXIS2_PLACEMENT_3D ( 'NONE', #34054, #63381, #17505 ) ;
#54387=EDGE_LOOP ( 'NONE', ( #59618, #32198, #34878, #41556 ) ) ;
#54388=CARTESIAN_POINT ( 'NONE',  ( 93.84685191531248449, 91.99731107132950569, 87.15572916753382060 ) ) ;
#54391=CARTESIAN_POINT ( 'NONE',  ( 92.34999999999999432, 90.00000000000002842, 88.73000000000000398 ) ) ;
#54399=EDGE_CURVE ( 'NONE', #26840, #8961, #70278, .T. ) ;
#54401=CARTESIAN_POINT ( 'NONE',  ( 92.35000000010803944, 90.00001510551041406, 78.64888723592453346 ) ) ;
#54402=EDGE_CURVE ( 'NONE', #65764, #42628, #26286, .T. ) ;
#54406=CARTESIAN_POINT ( 'NONE',  ( -92.69370383062498320, -211.3315407142195852, 83.71614583420050337 ) ) ;
#54407=ORIENTED_EDGE ( 'NONE', *, *, #66902, .T. ) ;
#54413=CARTESIAN_POINT ( 'NONE',  ( 94.99999999999998579, 87.33691857156068750, 77.10156250086711793 ) ) ;
#54426=CARTESIAN_POINT ( 'NONE',  ( -92.69370383062505425, 91.33154071421968467, 84.29822916753380468 ) ) ;
#54429=CYLINDRICAL_SURFACE ( 'NONE', #50347, 2.649999999999985700 ) ;
#54433=ORIENTED_EDGE ( 'NONE', *, *, #49716, .F. ) ;
#54441=CARTESIAN_POINT ( 'NONE',  ( 96.15314808468748708, -208.0026889286704943, 79.42989583420049371 ) ) ;
#54444=DIRECTION ( 'NONE',  ( 1.000000000000000000, 0.000000000000000000, 0.000000000000000000 ) ) ;
#54449=CARTESIAN_POINT ( 'NONE',  ( 93.84685191531249870, -208.0026889286704943, 77.63072916753381492 ) ) ;
#54450=AXIS2_PLACEMENT_3D ( 'NONE', #50683, #27757, #57448 ) ;
#54451=ORIENTED_EDGE ( 'NONE', *, *, #18591, .T. ) ;
#54455=DIRECTION ( 'NONE',  ( -0.000000000000000000, -0.000000000000000000, 1.000000000000000000 ) ) ;
#54458=CARTESIAN_POINT ( 'NONE',  ( 97.64999999999997726, -211.5299782133524502, 82.08895833506764461 ) ) ;
#54459=CARTESIAN_POINT ( 'NONE',  ( 94.99999999999998579, 86.94004357329500010, 84.44375000000000853 ) ) ;
#54461=CARTESIAN_POINT ( 'NONE',  ( 96.73972734126401463, 91.51405112163766375, 74.79348190356853365 ) ) ;
#54466=CARTESIAN_POINT ( 'NONE',  ( -95.00000000000002842, 87.33691857156074434, 89.32531250086715602 ) ) ;
#54467=CARTESIAN_POINT ( 'NONE',  ( 96.15314808468748708, 88.00268892867053694, 82.86947916753379673 ) ) ;
#54469=CARTESIAN_POINT ( 'NONE',  ( 92.34999999999999432, 88.47002178664753558, 81.24229166840098060 ) ) ;
#54470=CARTESIAN_POINT ( 'NONE',  ( 92.34999999999999432, 90.00000000000002842, 80.47499999999999432 ) ) ;
#54481=EDGE_CURVE ( 'NONE', #31307, #27645, #3581, .T. ) ;
#54482=CARTESIAN_POINT ( 'NONE',  ( -93.67500000000003979, 92.29496732002878900, 84.70833333333332860 ) ) ;
#54486=( BOUNDED_CURVE ( )  B_SPLINE_CURVE ( 2, ( #4020, #30059, #38206, #46997, #59022, #35691, #53008 ),
 .UNSPECIFIED., .F., .T. ) 
 B_SPLINE_CURVE_WITH_KNOTS ( ( 3, 2, 2, 3 ),
 ( 0.9583333333333337034, 0.9652777777777781232, 0.9722222222222225430, 0.9791666666666669627 ),
 .UNSPECIFIED. ) 
 CURVE ( )  GEOMETRIC_REPRESENTATION_ITEM ( )  RATIONAL_B_SPLINE_CURVE ( ( 0.9999999999999935607, 0.8660254037844451469, 1.000000000000000000, 0.8660254037844387076, 1.000000000000000000, 0.8660254037844322683, 1.000000000000006439 ) ) 
 REPRESENTATION_ITEM ( '' )  );
#54488=VERTEX_POINT ( 'NONE', #8973 ) ;
#54490=CARTESIAN_POINT ( 'NONE',  ( -97.30629616937497417, -211.3315407142195852, 78.90072916753381094 ) ) ;
#54498=EDGE_CURVE ( 'NONE', #72643, #50746, #72693, .T. ) ;
#54509=CARTESIAN_POINT ( 'NONE',  ( -97.30629616937501680, 90.00000000000004263, 75.03781250086713328 ) ) ;
#54512=( BOUNDED_CURVE ( )  B_SPLINE_CURVE ( 2, ( #38956, #68273, #67898, #26917, #44607, #67149, #73520 ),
 .UNSPECIFIED., .F., .F. ) 
 B_SPLINE_CURVE_WITH_KNOTS ( ( 3, 2, 2, 3 ),
 ( 0.8958333333333331483, 0.9027777777777775681, 0.9097222222222218768, 0.9166666666666662966 ),
 .UNSPECIFIED. ) 
 CURVE ( )  GEOMETRIC_REPRESENTATION_ITEM ( )  RATIONAL_B_SPLINE_CURVE ( ( 1.000000000000004219, 0.8660254037844343777, 1.000000000000000000, 0.8660254037844387076, 1.000000000000000000, 0.8660254037844451469, 0.9999999999999935607 ) ) 
 REPRESENTATION_ITEM ( '' )  );
#54514=FACE_OUTER_BOUND ( 'NONE', #63222, .T. ) ;
#54522=CARTESIAN_POINT ( 'NONE',  ( -96.32499999999996021, -207.7050326799711968, 89.25916666666667254 ) ) ;
#54524=EDGE_LOOP ( 'NONE', ( #13492, #69169, #64665, #20732 ) ) ;
#54527=CARTESIAN_POINT ( 'NONE',  ( 95.00000000000000000, -206.9400435732949575, 81.66562500173431260 ) ) ;
#54529=AXIS2_PLACEMENT_3D ( 'NONE', #20334, #14691, #54918 ) ;
#54531=CARTESIAN_POINT ( 'NONE',  ( -97.65000000000001990, 90.00000000000004263, 81.10999999999999943 ) ) ;
#54535=CARTESIAN_POINT ( 'NONE',  ( 96.15314808468750130, -211.9973110713294489, 81.59947916753381492 ) ) ;
#54536=CARTESIAN_POINT ( 'NONE',  ( 95.00000000000000000, -212.6630814284392557, 89.32531250086715602 ) ) ;
#54539=CARTESIAN_POINT ( 'NONE',  ( 95.00000000000000000, -207.3369185715606307, 87.10281250086715943 ) ) ;
#54545=CARTESIAN_POINT ( 'NONE',  ( -97.30629616937501680, 88.66845928578038638, 77.78947916753381264 ) ) ;
#54563=ORIENTED_EDGE ( 'NONE', *, *, #63957, .T. ) ;
#54564=CARTESIAN_POINT ( 'NONE',  ( 93.84685191531249870, -208.0026889286704943, 80.01197916753380923 ) ) ;
#54575=ADVANCED_FACE ( 'NONE', ( #48462 ), #5955, .F. ) ;
#54576=CARTESIAN_POINT ( 'NONE',  ( -95.00000000000002842, 87.33691857156074434, 79.16531250086715943 ) ) ;
#54577=ORIENTED_EDGE ( 'NONE', *, *, #35333, .F. ) ;
#54578=CARTESIAN_POINT ( 'NONE',  ( 93.84685191531248449, 88.00268892867053694, 78.95364583420047211 ) ) ;
#54587=CARTESIAN_POINT ( 'NONE',  ( -92.69370383062498320, -208.6684592857803295, 84.29822916753380468 ) ) ;
#54593=VERTEX_POINT ( 'NONE', #28863 ) ;
#54595=CARTESIAN_POINT ( 'NONE',  ( -96.32500000000001705, 87.70503267997129626, 76.13583333333333769 ) ) ;
#54597=CARTESIAN_POINT ( 'NONE',  ( -97.64999999980591383, 89.99998015682162134, 84.36502760998403971 ) ) ;
#54599=CARTESIAN_POINT ( 'NONE',  ( -95.00000000000002842, 87.33691857156074434, 84.72156250086713669 ) ) ;
#54602=CYLINDRICAL_SURFACE ( 'NONE', #73201, 3.299999999999969624 ) ;
#54607=LINE ( 'NONE', #62490, #27341 ) ;
#54611=CARTESIAN_POINT ( 'NONE',  ( 96.32499999999998863, 87.70503267997126784, 86.40166666666667084 ) ) ;
#54612=CARTESIAN_POINT ( 'NONE',  ( -94.99999999999997158, -212.6630814284392557, 83.61031250086716682 ) ) ;
#54621=CARTESIAN_POINT ( 'NONE',  ( -92.35000000000003695, 90.00000000000004263, 78.25249999999999773 ) ) ;
#54623=( BOUNDED_CURVE ( )  B_SPLINE_CURVE ( 2, ( #49965, #33417, #33047, #55988, #5624, #68020, #72886 ),
 .UNSPECIFIED., .F., .F. ) 
 B_SPLINE_CURVE_WITH_KNOTS ( ( 3, 2, 2, 3 ),
 ( 0.9166666666666662966, 0.9236111111111108274, 0.9305555555555551361, 0.9374999999999995559 ),
 .UNSPECIFIED. ) 
 CURVE ( )  GEOMETRIC_REPRESENTATION_ITEM ( )  RATIONAL_B_SPLINE_CURVE ( ( 1.000000000000006439, 0.8660254037844322683, 1.000000000000000000, 0.8660254037844387076, 1.000000000000000000, 0.8660254037844472563, 0.9999999999999914513 ) ) 
 REPRESENTATION_ITEM ( '' )  );
#54631=EDGE_CURVE ( 'NONE', #42391, #68050, #45430, .T. ) ;
#54643=CARTESIAN_POINT ( 'NONE',  ( 97.30629616937498838, 90.00000000000002842, 81.22906250086715829 ) ) ;
#54649=EDGE_CURVE ( 'NONE', #1126, #2080, #60220, .T. ) ;
#54650=ORIENTED_EDGE ( 'NONE', *, *, #19748, .T. ) ;
#54652=LINE ( 'NONE', #24966, #52657 ) ;
#54653=ORIENTED_EDGE ( 'NONE', *, *, #35702, .T. ) ;
#54663=CARTESIAN_POINT ( 'NONE',  ( -96.15314808468747287, -208.0026889286704943, 89.53697916753381492 ) ) ;
#54667=CARTESIAN_POINT ( 'NONE',  ( 96.32499999999997442, 92.29496732002878900, 75.89770833506763381 ) ) ;
#54668=CARTESIAN_POINT ( 'NONE',  ( -97.30629616937501680, 88.66845928578038638, 87.79072916753381151 ) ) ;
#54670=CARTESIAN_POINT ( 'NONE',  ( 92.69370383062498320, 90.00000000000002842, 75.19656250086714522 ) ) ;
#54673=CARTESIAN_POINT ( 'NONE',  ( 96.32499999999998863, -212.2949673200287179, 87.67166666666666686 ) ) ;
#54675=AXIS2_PLACEMENT_3D ( 'NONE', #16679, #39616, #27581 ) ;
#54676=CARTESIAN_POINT ( 'NONE',  ( -92.35000000000005116, 91.52997821335253548, 78.38479166840096468 ) ) ;
#54679=FACE_OUTER_BOUND ( 'NONE', #40694, .T. ) ;
#54693=CARTESIAN_POINT ( 'NONE',  ( -96.15314808468752972, 91.99731107132950569, 83.18697916753382060 ) ) ;
#54695=CIRCLE ( 'NONE', #25858, 15.69999999999999929 ) ;
#54696=DIRECTION ( 'NONE',  ( -0.000000000000000000, -0.000000000000000000, 1.000000000000000000 ) ) ;
#54698=DIRECTION ( 'NONE',  ( 0.000000000000000000, 0.000000000000000000, -1.000000000000000000 ) ) ;
#54704=CARTESIAN_POINT ( 'NONE',  ( 92.69370383062498320, 90.00000000000002842, 82.81656250086714977 ) ) ;
#54705=CARTESIAN_POINT ( 'NONE',  ( -97.30629616937497417, -211.3315407142195852, 81.59947916753382913 ) ) ;
#54707=EDGE_LOOP ( 'NONE', ( #50669, #25682, #31171, #43319 ) ) ;
#54708=CARTESIAN_POINT ( 'NONE',  ( -93.67499999999998295, -212.2949673200287179, 81.32166666666667254 ) ) ;
#54709=CARTESIAN_POINT ( 'NONE',  ( -92.34999999999999432, -209.9999999999999716, 77.61749999999999261 ) ) ;
#54712=AXIS2_PLACEMENT_3D ( 'NONE', #39728, #73916, #15291 ) ;
#54713=CARTESIAN_POINT ( 'NONE',  ( 96.15314808468748708, -208.0026889286704943, 83.71614583420047495 ) ) ;
#54719=( BOUNDED_CURVE ( )  B_SPLINE_CURVE ( 2, ( #14533, #8899, #61154, #60781, #42742, #60417, #54391 ),
 .UNSPECIFIED., .F., .F. ) 
 B_SPLINE_CURVE_WITH_KNOTS ( ( 3, 2, 2, 3 ),
 ( 0.06249999999999966693, 0.06944444444444407283, 0.07638888888888849260, 0.08333333333333288462 ),
 .UNSPECIFIED. ) 
 CURVE ( )  GEOMETRIC_REPRESENTATION_ITEM ( )  RATIONAL_B_SPLINE_CURVE ( ( 1.000000000000006439, 0.8660254037844322683, 1.000000000000000000, 0.8660254037844387076, 1.000000000000000000, 0.8660254037844472563, 0.9999999999999914513 ) ) 
 REPRESENTATION_ITEM ( '' )  );
#54720=CARTESIAN_POINT ( 'NONE',  ( -92.34999999999999432, -208.4700217866474645, 75.84479166840098685 ) ) ;
#54723=DIRECTION ( 'NONE',  ( 1.000000000000000000, 0.000000000000000000, 0.000000000000000000 ) ) ;
#54727=CARTESIAN_POINT ( 'NONE',  ( 93.84685191531251292, -211.9973110713294489, 79.11239583420048405 ) ) ;
#54730=CARTESIAN_POINT ( 'NONE',  ( -97.64996284860750109, 91.52999966271900689, 76.69145685134847668 ) ) ;
#54733=DIRECTION ( 'NONE',  ( -0.000000000000000000, -0.000000000000000000, 1.000000000000000000 ) ) ;
#54734=CARTESIAN_POINT ( 'NONE',  ( 92.35000000000002274, -208.4700217866474645, 81.69208333333332916 ) ) ;
#54740=CARTESIAN_POINT ( 'NONE',  ( -94.99999999999997158, -213.0599564267049857, 86.42812500173430124 ) ) ;
#54742=CARTESIAN_POINT ( 'NONE',  ( -97.30629616937501680, 88.66845928578038638, 84.13947916753383538 ) ) ;
#54743=CARTESIAN_POINT ( 'NONE',  ( 93.67499999999999716, 87.70503267997126784, 88.28020833506764120 ) ) ;
#54745=CARTESIAN_POINT ( 'NONE',  ( 94.99999999999998579, 93.05995642670504253, 76.50624999999999432 ) ) ;
#54748=CARTESIAN_POINT ( 'NONE',  ( -92.34999999999999432, -209.9999999999999716, 85.31687500173428873 ) ) ;
#54753=CARTESIAN_POINT ( 'NONE',  ( -97.65000000000001990, 88.47002178664754979, 84.41729166840097776 ) ) ;
#54755=CARTESIAN_POINT ( 'NONE',  ( 92.69370383062498320, 91.33154071421968467, 88.47864583420047779 ) ) ;
#54756=EDGE_CURVE ( 'NONE', #47170, #37739, #36695, .T. ) ;
#54760=CARTESIAN_POINT ( 'NONE',  ( -93.23660927304929658, 88.50623689698963403, 74.79348190356844839 ) ) ;
#54767=VERTEX_POINT ( 'NONE', #7417 ) ;
#54768=VECTOR ( 'NONE', #59226, 1000.000000000000000 ) ;
#54777=CARTESIAN_POINT ( 'NONE',  ( -97.30629616937497417, -211.3315407142195852, 86.04447916753382231 ) ) ;
#54780=EDGE_LOOP ( 'NONE', ( #22070, #16636, #25905, #39950, #11283 ) ) ;
#54783=CARTESIAN_POINT ( 'NONE',  ( -97.64999999999996305, -209.9999872707217037, 76.10937456147250657 ) ) ;
#54784=CARTESIAN_POINT ( 'NONE',  ( 92.69370383062498320, 90.00000000000002842, 77.57781250086713953 ) ) ;
#54786=CARTESIAN_POINT ( 'NONE',  ( -97.65000000000001990, 90.00000000000004263, 89.36499999999999488 ) ) ;
#54794=CARTESIAN_POINT ( 'NONE',  ( -93.84685191531254134, 91.99731107132950569, 82.44614583420046472 ) ) ;
#54806=CARTESIAN_POINT ( 'NONE',  ( 97.30629616937498838, -209.9999999999999716, 78.05406250086716113 ) ) ;
#54820=CARTESIAN_POINT ( 'NONE',  ( 92.69370383062501162, -209.9999999999999716, 75.83156250086716454 ) ) ;
#54822=ORIENTED_EDGE ( 'NONE', *, *, #67370, .T. ) ;
#54825=ORIENTED_EDGE ( 'NONE', *, *, #29444, .T. ) ;
#54826=CARTESIAN_POINT ( 'NONE',  ( -92.34999999999999432, -208.4700217866474645, 82.19479166840095274 ) ) ;
#54831=CARTESIAN_POINT ( 'NONE',  ( 95.00000000000000000, -206.9400435732949575, 79.12562500173429214 ) ) ;
#54832=CARTESIAN_POINT ( 'NONE',  ( 93.67499999999998295, 92.29496732002878900, 84.81416666666666515 ) ) ;
#54835=CARTESIAN_POINT ( 'NONE',  ( -92.69370383062501162, -210.2956651733040303, 74.79348190356850523 ) ) ;
#54839=CARTESIAN_POINT ( 'NONE',  ( -96.15314808468752972, 91.99731107132950569, 87.79072916753381151 ) ) ;
#54840=CARTESIAN_POINT ( 'NONE',  ( 93.84685191531248449, 91.99731107132950569, 81.28197916753380525 ) ) ;
#54841=EDGE_CURVE ( 'NONE', #72954, #67569, #55117, .T. ) ;
#54855=CARTESIAN_POINT ( 'NONE',  ( 97.64999999999999147, 90.00000000000002842, 89.12687500173430521 ) ) ;
#54857=CARTESIAN_POINT ( 'NONE',  ( -92.34999999999999432, -210.0000000024460576, 75.15687493084206494 ) ) ;
#54858=CARTESIAN_POINT ( 'NONE',  ( -96.15314808468745866, -211.9973110713294489, 78.95364583420047211 ) ) ;
#54863=CARTESIAN_POINT ( 'NONE',  ( 94.99999999999998579, 90.00000000000002842, 90.00000000000000000 ) ) ;
#54868=LINE ( 'NONE', #25923, #63754 ) ;
#54869=CARTESIAN_POINT ( 'NONE',  ( 96.15314808468748708, 91.99731107132950569, 88.16114583420046813 ) ) ;
#54870=CARTESIAN_POINT ( 'NONE',  ( -93.67499999999998295, -212.2949673200287179, 85.76666666666665151 ) ) ;
#54871=CARTESIAN_POINT ( 'NONE',  ( 97.65000000000000568, 88.47002178664752137, 81.45395833506763950 ) ) ;
#54876=AXIS2_PLACEMENT_3D ( 'NONE', #65078, #36480, #1223 ) ;
#54878=CARTESIAN_POINT ( 'NONE',  ( -95.00000000000002842, 90.00000000000004263, 90.00000000000000000 ) ) ;
#54879=VECTOR ( 'NONE', #21398, 1000.000000000000000 ) ;
#54885=CARTESIAN_POINT ( 'NONE',  ( -96.32499999999996021, -212.2949673200287179, 88.20083333333332121 ) ) ;
#54890=CARTESIAN_POINT ( 'NONE',  ( 96.32499999999998863, -212.2949673200287179, 78.22604166840096696 ) ) ;
#54902=CARTESIAN_POINT ( 'NONE',  ( 93.84685191531249870, -208.0026889286704943, 80.01197916753380923 ) ) ;
#54903=CARTESIAN_POINT ( 'NONE',  ( 97.30629616937498838, -209.9999999999999716, 86.30906250086715659 ) ) ;
#54906=CARTESIAN_POINT ( 'NONE',  ( 96.15314808468750130, -211.9973110713294489, 87.47322916753381605 ) ) ;
#54910=ORIENTED_EDGE ( 'NONE', *, *, #48237, .F. ) ;
#54911=CARTESIAN_POINT ( 'NONE',  ( -97.30629616937501680, 88.66845928578038638, 78.42447916753380355 ) ) ;
#54918=DIRECTION ( 'NONE',  ( 0.000000000000000000, 0.000000000000000000, 1.000000000000000000 ) ) ;
#54920=ADVANCED_FACE ( 'NONE', ( #17126 ), #68633, .F. ) ;
#54924=( BOUNDED_CURVE ( )  B_SPLINE_CURVE ( 2, ( #52718, #41078, #62922, #40327, #12488, #5762, #51973 ),
 .UNSPECIFIED., .F., .F. ) 
 B_SPLINE_CURVE_WITH_KNOTS ( ( 3, 2, 2, 3 ),
 ( 0.8749999999999997780, 0.8819444444444441977, 0.8888888888888886175, 0.8958333333333331483 ),
 .UNSPECIFIED. ) 
 CURVE ( )  GEOMETRIC_REPRESENTATION_ITEM ( )  RATIONAL_B_SPLINE_CURVE ( ( 1.000000000000004219, 0.8660254037844343777, 1.000000000000000000, 0.8660254037844387076, 1.000000000000000000, 0.8660254037844430375, 0.9999999999999956701 ) ) 
 REPRESENTATION_ITEM ( '' )  );
#54929=CARTESIAN_POINT ( 'NONE',  ( 96.15314808468750130, -211.9973110713294489, 79.05947916753380866 ) ) ;
#54936=ORIENTED_EDGE ( 'NONE', *, *, #65104, .F. ) ;
#54941=CARTESIAN_POINT ( 'NONE',  ( -93.84685191531252713, 88.00268892867056536, 79.85322916753381151 ) ) ;
#54943=CARTESIAN_POINT ( 'NONE',  ( 94.99999999999998579, 92.66308142843935514, 76.14906250086716000 ) ) ;
#54947=CARTESIAN_POINT ( 'NONE',  ( -97.64999999999990621, -211.5299782133524786, 76.71791666666666742 ) ) ;
#54950=CARTESIAN_POINT ( 'NONE',  ( -96.15314808468747287, -208.0026889286704943, 80.01197916753380923 ) ) ;
#54951=CARTESIAN_POINT ( 'NONE',  ( 92.35000000000002274, 88.47002178664750716, 86.87791666666664980 ) ) ;
#54956=CARTESIAN_POINT ( 'NONE',  ( -95.00000000000002842, 90.00000000000004263, 90.00000000000000000 ) ) ;
#54959=CARTESIAN_POINT ( 'NONE',  ( -92.69370383062502583, 91.33154071421968467, 85.56822916753380071 ) ) ;
#54963=ORIENTED_EDGE ( 'NONE', *, *, #20030, .F. ) ;
#54967=LINE ( 'NONE', #3490, #56186 ) ;
#54971=CARTESIAN_POINT ( 'NONE',  ( 92.35000000000000853, -208.4700217866474645, 88.75645833506762017 ) ) ;
#54972=CARTESIAN_POINT ( 'NONE',  ( -92.69370383062498320, -209.9999999999999716, 83.13406250086715943 ) ) ;
#54985=CARTESIAN_POINT ( 'NONE',  ( -94.99999999999997158, -209.9999999999999716, 90.00000000000000000 ) ) ;
#54997=DIRECTION ( 'NONE',  ( 1.000000000000000000, 0.000000000000000000, 0.000000000000000000 ) ) ;
#55000=VERTEX_POINT ( 'NONE', #50205 ) ;
#55007=CARTESIAN_POINT ( 'NONE',  ( 94.99999999999998579, 92.66308142843935514, 75.03781250086714749 ) ) ;
#55008=FACE_OUTER_BOUND ( 'NONE', #68319, .T. ) ;
#55015=CARTESIAN_POINT ( 'NONE',  ( 93.84685191531248449, 91.99731107132950569, 88.26697916753380468 ) ) ;
#55017=CARTESIAN_POINT ( 'NONE',  ( 97.30629616937498838, -211.3315407142195852, 89.27239583420048064 ) ) ;
#55025=CARTESIAN_POINT ( 'NONE',  ( -97.64999999999996305, -208.4700217866474645, 84.31145833506762699 ) ) ;
#55027=DIRECTION ( 'NONE',  ( -0.000000000000000000, -0.000000000000000000, 1.000000000000000000 ) ) ;
#55028=CARTESIAN_POINT ( 'NONE',  ( -97.64999999999996305, -209.9999999999999716, 77.37937500173428873 ) ) ;
#55029=CARTESIAN_POINT ( 'NONE',  ( -96.15314808468752972, 91.99731107132950569, 89.69572916753382685 ) ) ;
#55032=CARTESIAN_POINT ( 'NONE',  ( 97.30629616937498838, 91.33154071421968467, 86.20322916753382003 ) ) ;
#55033=CARTESIAN_POINT ( 'NONE',  ( -96.15314808468751551, 88.00268892867056536, 87.20864583420046756 ) ) ;
#55035=CARTESIAN_POINT ( 'NONE',  ( 94.99999999999998579, 92.66308142843935514, 78.21281250086717307 ) ) ;
#55040=CARTESIAN_POINT ( 'NONE',  ( -96.32500000000001705, 92.29496732002878900, 89.25916666666667254 ) ) ;
#55042=DIRECTION ( 'NONE',  ( 1.000000000000000000, 0.000000000000000000, 0.000000000000000000 ) ) ;
#55047=CARTESIAN_POINT ( 'NONE',  ( -93.67500000000003979, 87.70503267997129626, 80.05166666666666231 ) ) ;
#55048=LINE ( 'NONE', #19354, #59101 ) ;
#55056=CARTESIAN_POINT ( 'NONE',  ( -97.30629616937501680, 88.66845928578038638, 80.80572916753382628 ) ) ;
#55058=CARTESIAN_POINT ( 'NONE',  ( 94.99999999999998579, 86.94004357329502852, 82.61812500173428475 ) ) ;
#55065=LINE ( 'NONE', #31015, #8553 ) ;
#55066=CARTESIAN_POINT ( 'NONE',  ( 97.64999999999999147, -209.9999999999999716, 90.00000000000000000 ) ) ;
#55068=CARTESIAN_POINT ( 'NONE',  ( 92.69370383062498320, 90.00000000000002842, 79.64156250086715261 ) ) ;
#55069=VECTOR ( 'NONE', #53501, 1000.000000000000000 ) ;
#55072=CARTESIAN_POINT ( 'NONE',  ( -96.15314808468747287, -208.0026889286704943, 82.71072916753381321 ) ) ;
#55075=DIRECTION ( 'NONE',  ( -0.000000000000000000, 0.000000000000000000, 1.000000000000000000 ) ) ;
#55076=CARTESIAN_POINT ( 'NONE',  ( -94.99999999999997158, -206.9400435732949575, 79.04625000000000057 ) ) ;
#55079=CARTESIAN_POINT ( 'NONE',  ( 95.00000000000000000, -212.6630814284392557, 84.08656250086713158 ) ) ;
#55084=CARTESIAN_POINT ( 'NONE',  ( -94.99999999999997158, -206.9400435732949575, 75.95062500173428077 ) ) ;
#55088=FACE_OUTER_BOUND ( 'NONE', #9892, .T. ) ;
#55091=CARTESIAN_POINT ( 'NONE',  ( 97.30629616937498838, -209.9999999999999716, 78.05406250086716113 ) ) ;
#55096=CIRCLE ( 'NONE', #35887, 2.649999999999985700 ) ;
#55097=CARTESIAN_POINT ( 'NONE',  ( 97.64999999999989200, -211.5299782133525071, 80.73958333333335702 ) ) ;
#55098=CARTESIAN_POINT ( 'NONE',  ( 93.84685191531248449, 88.00268892867053694, 85.46239583420047836 ) ) ;
#55101=CARTESIAN_POINT ( 'NONE',  ( 95.00000000000000000, -206.9400435732949575, 82.22124999999999773 ) ) ;
#55104=ORIENTED_EDGE ( 'NONE', *, *, #54355, .F. ) ;
#55108=CARTESIAN_POINT ( 'NONE',  ( -97.30629616937501680, 90.00000000000004263, 85.35656250086715602 ) ) ;
#55109=CARTESIAN_POINT ( 'NONE',  ( 92.35000752690139336, 88.47001744098895415, 88.22729196900363036 ) ) ;
#55111=CARTESIAN_POINT ( 'NONE',  ( 93.67499999999999716, 87.70503267997126784, 76.13583333333333769 ) ) ;
#55113=ORIENTED_EDGE ( 'NONE', *, *, #59094, .T. ) ;
#55115=CARTESIAN_POINT ( 'NONE',  ( -97.64999999999994884, -208.4700217866474645, 85.58145833506763722 ) ) ;
#55117=LINE ( 'NONE', #61511, #19393 ) ;
#55119=CARTESIAN_POINT ( 'NONE',  ( -92.35000000000003695, 90.00000000000004263, 83.41187500173430180 ) ) ;
#55122=CARTESIAN_POINT ( 'NONE',  ( 96.15314808468748708, 88.00268892867053694, 88.10822916753382117 ) ) ;
#55124=VECTOR ( 'NONE', #42264, 1000.000000000000000 ) ;
#55140=CARTESIAN_POINT ( 'NONE',  ( -92.69370383062498320, -208.6684592857803011, 84.45697916753383083 ) ) ;
#55141=ORIENTED_EDGE ( 'NONE', *, *, #15688, .T. ) ;
#55148=CARTESIAN_POINT ( 'NONE',  ( 92.34999999999999432, 88.47002178664752137, 81.87729166840097150 ) ) ;
#55149=CARTESIAN_POINT ( 'NONE',  ( 97.65000000000000568, -208.4700217866474645, 82.82979166840095786 ) ) ;
#55150=CARTESIAN_POINT ( 'NONE',  ( 92.69370383062498320, 88.66845928578035796, 77.63072916753380071 ) ) ;
#55151=CARTESIAN_POINT ( 'NONE',  ( 97.65000000000000568, -209.9999999999999716, 75.00000000000000000 ) ) ;
#55153=EDGE_CURVE ( 'NONE', #36890, #70455, #52433, .T. ) ;
#55156=FACE_OUTER_BOUND ( 'NONE', #61018, .T. ) ;
#55161=( BOUNDED_CURVE ( )  B_SPLINE_CURVE ( 2, ( #64945, #25077, #30704, #13783, #13422, #25447, #53650, #42377, #53282 ),
 .UNSPECIFIED., .F., .F. ) 
 B_SPLINE_CURVE_WITH_KNOTS ( ( 3, 2, 2, 2, 3 ),
 ( 0.7196881748069930973, 0.7267438507144522442, 0.7337996162553684920, 0.7408553817962847399, 0.7408554641904511184 ),
 .UNSPECIFIED. ) 
 CURVE ( )  GEOMETRIC_REPRESENTATION_ITEM ( )  RATIONAL_B_SPLINE_CURVE ( ( 0.9999965961301877648, 0.8660271057409657525, 1.000000000000000000, 0.8660254037844387076, 1.000000000000000000, 0.8660254037844387076, 1.000000000000000000, 0.9999984355028379568, 0.9999968710422149076 ) ) 
 REPRESENTATION_ITEM ( '' )  );
#55167=CARTESIAN_POINT ( 'NONE',  ( -93.84685191531252713, 88.00268892867056536, 81.59947916753381492 ) ) ;
#55174=EDGE_CURVE ( 'NONE', #70250, #65477, #52821, .T. ) ;
#55179=CARTESIAN_POINT ( 'NONE',  ( 95.00000000000000000, -207.3369185715606307, 77.57781250086715374 ) ) ;
#55187=PLANE ( 'NONE',  #14950 ) ;
#55190=CARTESIAN_POINT ( 'NONE',  ( 95.00000000000000000, -207.3369185715606307, 76.30781250086715772 ) ) ;
#55192=ORIENTED_EDGE ( 'NONE', *, *, #8831, .F. ) ;
#55193=CARTESIAN_POINT ( 'NONE',  ( -94.99999999999997158, -206.9400435732949575, 87.93624999999998693 ) ) ;
#55197=VECTOR ( 'NONE', #10360, 1000.000000000000000 ) ;
#55203=CARTESIAN_POINT ( 'NONE',  ( 97.64999999999999147, -209.9999999999999716, 80.23687500173429044 ) ) ;
#55204=CARTESIAN_POINT ( 'NONE',  ( 93.67499999999999716, 87.70503267997126784, 85.66083333333332916 ) ) ;
#55206=ORIENTED_EDGE ( 'NONE', *, *, #41692, .F. ) ;
#55211=CARTESIAN_POINT ( 'NONE',  ( -93.84685191531254134, 91.99731107132950569, 84.50989583420049200 ) ) ;
#55212=CARTESIAN_POINT ( 'NONE',  ( 97.30629616937498838, 88.66845928578037217, 81.65239583420049030 ) ) ;
#55214=FACE_OUTER_BOUND ( 'NONE', #43650, .T. ) ;
#55222=EDGE_CURVE ( 'NONE', #63128, #24873, #43528, .T. ) ;
#55223=CARTESIAN_POINT ( 'NONE',  ( 93.67499999999998295, 92.29496732002878900, 88.70354166840097321 ) ) ;
#55224=EDGE_LOOP ( 'NONE', ( #21343, #23504, #40122, #786 ) ) ;
#55226=CARTESIAN_POINT ( 'NONE',  ( -97.30629616937497417, -211.3315407142195852, 79.53572916753380184 ) ) ;
#55238=DIRECTION ( 'NONE',  ( -0.000000000000000000, -0.000000000000000000, 1.000000000000000000 ) ) ;
#55240=CARTESIAN_POINT ( 'NONE',  ( 97.30629616937498838, 91.33154071421968467, 86.83822916753381094 ) ) ;
#55244=CARTESIAN_POINT ( 'NONE',  ( -97.64999999999997726, 88.47002178664752137, 86.87791666666664980 ) ) ;
#55247=CARTESIAN_POINT ( 'NONE',  ( 97.64999999999999147, 90.00000000000002842, 77.61749999999999261 ) ) ;
#55248=CARTESIAN_POINT ( 'NONE',  ( 95.00000000000000000, -206.9400435732949575, 75.23624999999998408 ) ) ;
#55258=CARTESIAN_POINT ( 'NONE',  ( -92.34999999999999432, -208.4700217866474645, 89.73541666666666572 ) ) ;
#55265=PLANE ( 'NONE',  #45494 ) ;
#55269=ADVANCED_FACE ( 'NONE', ( #19700 ), #47245, .F. ) ;
#55276=CARTESIAN_POINT ( 'NONE',  ( 92.69370383062501162, -209.9999999999999716, 82.65781250086713783 ) ) ;
#55277=CARTESIAN_POINT ( 'NONE',  ( 97.30629616937498838, -209.9999999999999716, 84.40406250086715545 ) ) ;
#55279=CARTESIAN_POINT ( 'NONE',  ( 95.00000000000000000, -212.6630814284392557, 85.51531250086713953 ) ) ;
#55280=EDGE_CURVE ( 'NONE', #35608, #60230, #53487, .T. ) ;
#55286=CARTESIAN_POINT ( 'NONE',  ( -97.30629616937501680, 91.33154071421968467, 78.95364583420048632 ) ) ;
#55288=ORIENTED_EDGE ( 'NONE', *, *, #33327, .F. ) ;
#55293=CARTESIAN_POINT ( 'NONE',  ( 95.00000000000000000, -206.9400435732949575, 89.28562500173430294 ) ) ;
#55296=ORIENTED_EDGE ( 'NONE', *, *, #62659, .F. ) ;
#55300=EDGE_LOOP ( 'NONE', ( #51691, #69911, #46329, #5007 ) ) ;
#55302=CARTESIAN_POINT ( 'NONE',  ( 95.00000000000000000, -212.6630814284392557, 75.19656250086714522 ) ) ;
#55305=FACE_BOUND ( 'NONE', #45577, .T. ) ;
#55312=CARTESIAN_POINT ( 'NONE',  ( -92.69370383062504004, 90.00000000000004263, 76.14906250086716000 ) ) ;
#55314=CARTESIAN_POINT ( 'NONE',  ( 93.84685191531248449, 88.00268892867053694, 76.41364583420048007 ) ) ;
#55317=CARTESIAN_POINT ( 'NONE',  ( -92.69370383062498320, -208.6684592857803011, 88.10822916753380696 ) ) ;
#55321=CARTESIAN_POINT ( 'NONE',  ( -97.30629616937495996, -209.9999999999999716, 80.75281250086715090 ) ) ;
#55326=VERTEX_POINT ( 'NONE', #18523 ) ;
#55329=DIRECTION ( 'NONE',  ( 1.000000000000000000, 0.000000000000000000, 0.000000000000000000 ) ) ;
#55332=FACE_OUTER_BOUND ( 'NONE', #45499, .T. ) ;
#55333=CARTESIAN_POINT ( 'NONE',  ( -92.69370383062504004, 90.00000000000004263, 82.97531250086714749 ) ) ;
#55342=LINE ( 'NONE', #3863, #15321 ) ;
#55343=DIRECTION ( 'NONE',  ( 1.000000000000000000, 0.000000000000000000, 0.000000000000000000 ) ) ;
#55345=CARTESIAN_POINT ( 'NONE',  ( -97.30629616937495996, -209.9999999999999716, 82.81656250086714977 ) ) ;
#55352=CONICAL_SURFACE ( 'NONE', #22961, 2.649999999999999467, 1.029744258676654312 ) ;
#55368=( BOUNDED_CURVE ( )  B_SPLINE_CURVE ( 2, ( #52519, #12300, #7777, #13775, #18674, #35239, #18313 ),
 .UNSPECIFIED., .F., .F. ) 
 B_SPLINE_CURVE_WITH_KNOTS ( ( 3, 2, 2, 3 ),
 ( 0.6666666666666667407, 0.6736111111111112715, 0.6805555555555555802, 0.6875000000000000000 ),
 .UNSPECIFIED. ) 
 CURVE ( )  GEOMETRIC_REPRESENTATION_ITEM ( )  RATIONAL_B_SPLINE_CURVE ( ( 0.9999999999999978906, 0.8660254037844408170, 1.000000000000000000, 0.8660254037844387076, 1.000000000000000000, 0.8660254037844387076, 1.000000000000000000 ) ) 
 REPRESENTATION_ITEM ( '' )  );
#55371=ORIENTED_EDGE ( 'NONE', *, *, #2343, .F. ) ;
#55382=EDGE_LOOP ( 'NONE', ( #70943, #42914, #10512, #48634 ) ) ;
#55383=CARTESIAN_POINT ( 'NONE',  ( 92.69370383062498320, 88.66845928578037217, 77.78947916753381264 ) ) ;
#55384=DIRECTION ( 'NONE',  ( -0.000000000000000000, -0.000000000000000000, 1.000000000000000000 ) ) ;
#55386=ORIENTED_EDGE ( 'NONE', *, *, #25137, .T. ) ;
#55389=VECTOR ( 'NONE', #57270, 1000.000000000000000 ) ;
#55390=VERTEX_POINT ( 'NONE', #42218 ) ;
#55391=CARTESIAN_POINT ( 'NONE',  ( 93.84685191531248449, 91.99731107132950569, 89.53697916753381492 ) ) ;
#55393=CARTESIAN_POINT ( 'NONE',  ( 97.30629616937498838, -208.6684592857803011, 86.83822916753381094 ) ) ;
#55396=FACE_OUTER_BOUND ( 'NONE', #38400, .T. ) ;
#55398=CARTESIAN_POINT ( 'NONE',  ( -0.0004442498525516064278, 0.001194404164626844313, -85.60000000000000853 ) ) ;
#55401=CARTESIAN_POINT ( 'NONE',  ( -96.32499999999996021, -212.2949673200287179, 74.94520833506761903 ) ) ;
#55405=CARTESIAN_POINT ( 'NONE',  ( 92.69370383062498320, 88.66845928578037217, 87.79072916753381151 ) ) ;
#55406=CARTESIAN_POINT ( 'NONE',  ( -92.35000000000003695, 88.93103996628917685, 74.48490336299447279 ) ) ;
#55410=FACE_OUTER_BOUND ( 'NONE', #62340, .T. ) ;
#55414=EDGE_CURVE ( 'NONE', #15281, #44177, #11243, .T. ) ;
#55424=CARTESIAN_POINT ( 'NONE',  ( -96.32500000000001705, 92.29496732002878900, 79.73416666666666686 ) ) ;
#55430=CARTESIAN_POINT ( 'NONE',  ( -93.84685191531247028, -211.9973110713294489, 75.40822916753381833 ) ) ;
#55433=CARTESIAN_POINT ( 'NONE',  ( -95.00000000000002842, 87.33691857156074434, 83.45156250086714067 ) ) ;
#55436=CARTESIAN_POINT ( 'NONE',  ( -93.67500000000003979, 87.70503267997129626, 85.76666666666665151 ) ) ;
#55440=CARTESIAN_POINT ( 'NONE',  ( 92.35001798596596245, -208.4700114024452375, 80.50145761676020584 ) ) ;
#55445=CARTESIAN_POINT ( 'NONE',  ( 93.84685191531248449, 88.00268892867053694, 81.01739583420049939 ) ) ;
#55446=CARTESIAN_POINT ( 'NONE',  ( -92.69370383062498320, -209.9999999999999716, 82.49906250086715431 ) ) ;
#55452=CARTESIAN_POINT ( 'NONE',  ( -93.67499999999998295, -212.2949673200287179, 76.24166666666666003 ) ) ;
#55457=CARTESIAN_POINT ( 'NONE',  ( -92.69370383062505425, 91.33154071421968467, 78.74197916753381321 ) ) ;
#55458=CARTESIAN_POINT ( 'NONE',  ( 93.84685191531251292, -211.9973110713294489, 82.12864583420046927 ) ) ;
#55459=ORIENTED_EDGE ( 'NONE', *, *, #58037, .T. ) ;
#55464=CARTESIAN_POINT ( 'NONE',  ( 97.64999999981932888, 89.99996905681224746, 78.33187387208513996 ) ) ;
#55467=CARTESIAN_POINT ( 'NONE',  ( 93.67500000000001137, -207.7050326799711968, 84.17916666666666003 ) ) ;
#55476=CARTESIAN_POINT ( 'NONE',  ( 92.69370383062498320, 91.33154071421968467, 87.84364583420048689 ) ) ;
#55477=CARTESIAN_POINT ( 'NONE',  ( -92.35000000000003695, 90.00000000000004263, 83.41187500173430180 ) ) ;
#55478=CARTESIAN_POINT ( 'NONE',  ( 92.35000000000000853, -209.9999999999999716, 81.10999999999999943 ) ) ;
#55486=CARTESIAN_POINT ( 'NONE',  ( -96.32499999999996021, -207.7050326799711968, 77.19416666666666060 ) ) ;
#55493=CARTESIAN_POINT ( 'NONE',  ( -96.32499999999996021, -212.2949673200287179, 86.37520833506764006 ) ) ;
#55498=CARTESIAN_POINT ( 'NONE',  ( -96.32500000000001705, 92.29496732002878900, 84.25854166840096582 ) ) ;
#55500=CARTESIAN_POINT ( 'NONE',  ( 92.69370383062498320, 90.00000000000002842, 84.72156250086715090 ) ) ;
#55503=EDGE_CURVE ( 'NONE', #10929, #48479, #39564, .T. ) ;
#55510=DIRECTION ( 'NONE',  ( 1.000000000000000000, 0.000000000000000000, 0.000000000000000000 ) ) ;
#55515=B_SPLINE_CURVE_WITH_KNOTS ( 'NONE', 3,
 ( #64308, #51155, #52644, #28973, #46639, #57926, #58287, #57186, #62849, #22603, #29329, #1195, #90, #45548, #16961, #448, #45913, #29695 ),
 .UNSPECIFIED., .F., .F.,
 ( 4, 2, 2, 2, 2, 2, 2, 2, 4 ),
 ( -0.004093595874563301339, -0.003575961937392278713, -0.003058328000221256088, -0.002540694063050233029, -0.002023060125879210403, -0.001505426188708187778, -0.0009877922515371647186, -0.0004701583143661420931, 4.747562280488053232E-05 ),
 .UNSPECIFIED. ) ;
#55517=CARTESIAN_POINT ( 'NONE',  ( -95.00000000000002842, 86.94004357329504273, 80.07812500173429271 ) ) ;
#55520=CARTESIAN_POINT ( 'NONE',  ( -92.69370383062498320, -211.3315407142195852, 85.62114583420047609 ) ) ;
#55530=CARTESIAN_POINT ( 'NONE',  ( 97.30629616937498838, 88.66845928578035796, 79.74739583420047495 ) ) ;
#55534=CARTESIAN_POINT ( 'NONE',  ( 96.58546442478332494, 91.70561969393826018, 74.79912739178801928 ) ) ;
#55538=EDGE_CURVE ( 'NONE', #14968, #16250, #39909, .T. ) ;
#55541=FACE_OUTER_BOUND ( 'NONE', #39882, .T. ) ;
#55543=CARTESIAN_POINT ( 'NONE',  ( -97.30629616937501680, 90.00000000000004263, 84.56281250086713897 ) ) ;
#55546=VERTEX_POINT ( 'NONE', #45176 ) ;
#55547=LINE ( 'NONE', #43176, #30655 ) ;
#55551=CARTESIAN_POINT ( 'NONE',  ( 93.84685191531249870, -208.0026889286704943, 77.63072916753381492 ) ) ;
#55556=CARTESIAN_POINT ( 'NONE',  ( -97.64999999993850111, -209.9999881787635729, 81.82400613094797848 ) ) ;
#55559=LINE ( 'NONE', #5191, #43609 ) ;
#55562=CARTESIAN_POINT ( 'NONE',  ( 97.30629616937498838, -211.3315407142195852, 77.36614583420048064 ) ) ;
#55564=PLANE ( 'NONE',  #46743 ) ;
#55574=CARTESIAN_POINT ( 'NONE',  ( 96.32499999999998863, -207.7050326799711968, 79.70770833506762187 ) ) ;
#55575=CARTESIAN_POINT ( 'NONE',  ( 93.67499999999998295, 92.29496732002878900, 80.36916666666665776 ) ) ;
#55577=ORIENTED_EDGE ( 'NONE', *, *, #42010, .F. ) ;
#55583=CARTESIAN_POINT ( 'NONE',  ( -95.00000000000002842, 87.33691857156074434, 83.61031250086715261 ) ) ;
#55584=CARTESIAN_POINT ( 'NONE',  ( 97.30629616937498838, 88.66845928578037217, 79.74739583420047495 ) ) ;
#55592=CARTESIAN_POINT ( 'NONE',  ( -96.15314808468747287, -208.0026889286704943, 79.37697916753380412 ) ) ;
#55595=DIRECTION ( 'NONE',  ( -1.000000000000000000, 0.000000000000000000, -0.000000000000000000 ) ) ;
#55600=( BOUNDED_CURVE ( )  B_SPLINE_CURVE ( 2, ( #22299, #10272, #4286, #38482, #45243, #15166, #61420 ),
 .UNSPECIFIED., .F., .F. ) 
 B_SPLINE_CURVE_WITH_KNOTS ( ( 3, 2, 2, 3 ),
 ( 0.6250000000000003331, 0.6319444444444446418, 0.6388888888888890616, 0.6458333333333334814 ),
 .UNSPECIFIED. ) 
 CURVE ( )  GEOMETRIC_REPRESENTATION_ITEM ( )  RATIONAL_B_SPLINE_CURVE ( ( 0.9999999999999935607, 0.8660254037844451469, 1.000000000000000000, 0.8660254037844387076, 1.000000000000000000, 0.8660254037844365982, 1.000000000000002220 ) ) 
 REPRESENTATION_ITEM ( '' )  );
#55602=CARTESIAN_POINT ( 'NONE',  ( -96.15314808468745866, -211.9973110713294489, 79.58864583420047722 ) ) ;
#55603=ORIENTED_EDGE ( 'NONE', *, *, #24228, .T. ) ;
#55606=DIRECTION ( 'NONE',  ( -1.000000000000000000, 0.000000000000000000, 0.000000000000000000 ) ) ;
#55611=CARTESIAN_POINT ( 'NONE',  ( 92.35003714631601213, -208.4700003402118966, 82.40645685155124056 ) ) ;
#55612=CARTESIAN_POINT ( 'NONE',  ( 94.99999999999998579, 87.33691857156068750, 88.53156250086716739 ) ) ;
#55622=EDGE_CURVE ( 'NONE', #47166, #52810, #56926, .T. ) ;
#55624=FACE_OUTER_BOUND ( 'NONE', #6657, .T. ) ;
#55625=AXIS2_PLACEMENT_3D ( 'NONE', #11107, #28384, #38940 ) ;
#55626=AXIS2_PLACEMENT_3D ( 'NONE', #20661, #33040, #45468 ) ;
#55627=CYLINDRICAL_SURFACE ( 'NONE', #26955, 2.649999999999999467 ) ;
#55631=CARTESIAN_POINT ( 'NONE',  ( -96.32499999999996021, -212.2949673200287179, 86.29583333333333428 ) ) ;
#55637=CARTESIAN_POINT ( 'NONE',  ( 92.69370383062501162, -209.9999999999999716, 89.80156250086714920 ) ) ;
#55644=CARTESIAN_POINT ( 'NONE',  ( 96.15314808468748708, -208.0026889286704943, 78.00114583420048575 ) ) ;
#55645=CARTESIAN_POINT ( 'NONE',  ( 93.84685191531249870, -208.0026889286704943, 86.52072916753382970 ) ) ;
#55647=CARTESIAN_POINT ( 'NONE',  ( 93.84685191531251292, -211.9973110713294489, 85.46239583420047836 ) ) ;
#55648=CARTESIAN_POINT ( 'NONE',  ( 93.67500000000001137, -212.2949673200287179, 78.12020833506763040 ) ) ;
#55651=CARTESIAN_POINT ( 'NONE',  ( -92.34999999999999432, -209.9999999999999716, 78.25249999999999773 ) ) ;
#55652=VERTEX_POINT ( 'NONE', #40267 ) ;
#55653=CARTESIAN_POINT ( 'NONE',  ( -92.69370383062502583, 89.06967028092473981, 74.84209033237942776 ) ) ;
#55657=CARTESIAN_POINT ( 'NONE',  ( -92.35000000035638834, 89.99995654222792041, 89.12687334326074051 ) ) ;
#55659=ORIENTED_EDGE ( 'NONE', *, *, #10251, .F. ) ;
#55674=CARTESIAN_POINT ( 'NONE',  ( 92.69370383062501162, -211.3315407142195852, 75.72572916753381378 ) ) ;
#55675=AXIS2_PLACEMENT_3D ( 'NONE', #21031, #10498, #72164 ) ;
#55678=ORIENTED_EDGE ( 'NONE', *, *, #50656, .T. ) ;
#55683=CARTESIAN_POINT ( 'NONE',  ( -97.65000000000001990, 90.00000000000004263, 90.00000000000000000 ) ) ;
#55685=EDGE_CURVE ( 'NONE', #69332, #56782, #68482, .T. ) ;
#55686=CARTESIAN_POINT ( 'NONE',  ( 97.30629616937498838, 91.33154071421968467, 76.67822916753378593 ) ) ;
#55688=CARTESIAN_POINT ( 'NONE',  ( 97.65000000000000568, 89.99998452726534026, 78.33187446658581621 ) ) ;
#55689=CARTESIAN_POINT ( 'NONE',  ( -97.30629616937495996, -209.9999999999999716, 89.00781250086714635 ) ) ;
#55695=CARTESIAN_POINT ( 'NONE',  ( -96.15314808468747287, -208.0026889286704943, 78.74197916753381321 ) ) ;
#55705=CARTESIAN_POINT ( 'NONE',  ( 94.21072067537654959, -207.7213858236421231, 74.85481846778738202 ) ) ;
#55706=EDGE_CURVE ( 'NONE', #70972, #22766, #21778, .T. ) ;
#55707=CARTESIAN_POINT ( 'NONE',  ( -95.00000000000002842, 87.33691857156074434, 82.81656250086713555 ) ) ;
#55708=DIRECTION ( 'NONE',  ( -0.000000000000000000, -0.000000000000000000, 1.000000000000000000 ) ) ;
#55715=CARTESIAN_POINT ( 'NONE',  ( -92.35000000000003695, 90.00000000000004263, 89.68250000000000455 ) ) ;
#55716=CARTESIAN_POINT ( 'NONE',  ( 92.35000000045006630, -210.0000310946952595, 88.81037122969986797 ) ) ;
#55717=CARTESIAN_POINT ( 'NONE',  ( -92.69370383062498320, -208.6684592857803011, 80.64697916753382856 ) ) ;
#55718=CARTESIAN_POINT ( 'NONE',  ( -92.34999999999999432, -209.9999753241900748, 87.22187585518541653 ) ) ;
#55720=ORIENTED_EDGE ( 'NONE', *, *, #72797, .T. ) ;
#55725=ORIENTED_EDGE ( 'NONE', *, *, #59268, .T. ) ;
#55728=AXIS2_PLACEMENT_3D ( 'NONE', #25009, #47950, #26115 ) ;
#55738=CARTESIAN_POINT ( 'NONE',  ( 92.34999999999999432, 90.00000000000002842, 84.92000000000000171 ) ) ;
#55745=LINE ( 'NONE', #4262, #61255 ) ;
#55751=ORIENTED_EDGE ( 'NONE', *, *, #64317, .F. ) ;
#55757=CARTESIAN_POINT ( 'NONE',  ( 97.30629616937498838, 88.66845928578037217, 76.73114583420048973 ) ) ;
#55764=CARTESIAN_POINT ( 'NONE',  ( 92.69370383062498320, 90.00000000000002842, 87.10281250086714522 ) ) ;
#55766=CARTESIAN_POINT ( 'NONE',  ( 93.84685191531251292, -211.9973110713294489, 84.66864583420047552 ) ) ;
#55769=FACE_OUTER_BOUND ( 'NONE', #54707, .T. ) ;
#55774=CARTESIAN_POINT ( 'NONE',  ( 97.64999999999990621, 90.00000071509185773, 85.31687502647973531 ) ) ;
#55775=CARTESIAN_POINT ( 'NONE',  ( -93.84685191531248449, -208.0026889286704943, 86.89114583420047211 ) ) ;
#55776=CARTESIAN_POINT ( 'NONE',  ( -92.69370383062502583, 88.66845928578038638, 84.35114583420049428 ) ) ;
#55778=CARTESIAN_POINT ( 'NONE',  ( 92.69370383062498320, 91.33154071421968467, 88.31989583420046586 ) ) ;
#55779=CARTESIAN_POINT ( 'NONE',  ( -97.30629616937501680, 90.00000000000004263, 87.73781250086713612 ) ) ;
#55787=CARTESIAN_POINT ( 'NONE',  ( -93.84685191531247028, -211.9973110713294489, 89.21947916753380525 ) ) ;
#55788=CYLINDRICAL_SURFACE ( 'NONE', #13712, 2.649999999999985700 ) ;
#55796=CARTESIAN_POINT ( 'NONE',  ( -96.32500000000001705, 87.70503267997129626, 80.58083333333331666 ) ) ;
#55802=CARTESIAN_POINT ( 'NONE',  ( 96.92442009029373651, 88.17815826261617929, 75.00000000000000000 ) ) ;
#55804=CARTESIAN_POINT ( 'NONE',  ( -96.32499999999996021, -207.7050326799711968, 79.73416666666666686 ) ) ;
#55806=CARTESIAN_POINT ( 'NONE',  ( -95.00000000000002842, 87.33691857156074434, 82.18156250086714465 ) ) ;
#55815=CARTESIAN_POINT ( 'NONE',  ( 92.35000000021534561, -209.9999789922616458, 79.91868729553134187 ) ) ;
#55816=( BOUNDED_CURVE ( )  B_SPLINE_CURVE ( 2, ( #61071, #16319, #55802 ),
 .UNSPECIFIED., .F., .T. ) 
 B_SPLINE_CURVE_WITH_KNOTS ( ( 3, 3 ),
 ( 0.9791666666666669627, 0.9841647806526081510 ),
 .UNSPECIFIED. ) 
 CURVE ( )  GEOMETRIC_REPRESENTATION_ITEM ( )  RATIONAL_B_SPLINE_CURVE ( ( 0.9999999999999935607, 0.9035746763527595649, 0.9459494432169361922 ) ) 
 REPRESENTATION_ITEM ( '' )  );
#55817=CARTESIAN_POINT ( 'NONE',  ( 94.99999999999998579, 92.66308142843932671, 80.11781250086714579 ) ) ;
#55818=CARTESIAN_POINT ( 'NONE',  ( -92.69370383062498320, -208.6684592857803295, 83.82197916753382572 ) ) ;
#55821=CARTESIAN_POINT ( 'NONE',  ( -97.65000000000001990, 90.00000000000004263, 83.09437500173430635 ) ) ;
#55822=CARTESIAN_POINT ( 'NONE',  ( -92.34999999999999432, -208.4700217866474645, 77.67041666666665378 ) ) ;
#55823=CARTESIAN_POINT ( 'NONE',  ( -97.64999999999996305, -209.9999999999999716, 90.00000000000000000 ) ) ;
#55825=CARTESIAN_POINT ( 'NONE',  ( -93.84685191531252713, 88.00268892867056536, 79.21822916753382060 ) ) ;
#55826=CARTESIAN_POINT ( 'NONE',  ( 92.69370383062501162, -208.6684592857803011, 80.69989583420048973 ) ) ;
#55829=VERTEX_POINT ( 'NONE', #24099 ) ;
#55833=CARTESIAN_POINT ( 'NONE',  ( -92.34999999999999432, -209.9999999999999716, 83.33250000000001023 ) ) ;
#55837=VERTEX_POINT ( 'NONE', #32295 ) ;
#55839=VERTEX_POINT ( 'NONE', #38326 ) ;
#55840=EDGE_CURVE ( 'NONE', #51073, #57704, #18908, .T. ) ;
#55842=CARTESIAN_POINT ( 'NONE',  ( 97.64999999999999147, -209.9999999999999716, 90.00000000000000000 ) ) ;
#55846=CARTESIAN_POINT ( 'NONE',  ( 92.69370383062498320, 88.66845928578037217, 86.67947916753382742 ) ) ;
#55848=CARTESIAN_POINT ( 'NONE',  ( 96.32499999999998863, -212.2949673200287179, 78.14666666666667538 ) ) ;
#55850=VERTEX_POINT ( 'NONE', #9376 ) ;
#55854=CARTESIAN_POINT ( 'NONE',  ( -0.0004442498525516064278, 0.001194404164626844313, -64.00000000000000000 ) ) ;
#55855=DIRECTION ( 'NONE',  ( -0.000000000000000000, -0.000000000000000000, 1.000000000000000000 ) ) ;
#55860=EDGE_CURVE ( 'NONE', #46998, #45794, #29443, .T. ) ;
#55863=CARTESIAN_POINT ( 'NONE',  ( -93.67499999999998295, -212.2949673200287179, 81.40104166840096411 ) ) ;
#55867=CARTESIAN_POINT ( 'NONE',  ( 94.99999999999998579, 93.05995642670504253, 82.93562500173429441 ) ) ;
#55868=CARTESIAN_POINT ( 'NONE',  ( -97.65000000000001990, 88.47002178664754979, 81.87729166840097150 ) ) ;
#55870=CARTESIAN_POINT ( 'NONE',  ( 96.15314808468748708, 88.00268892867053694, 81.75822916753382685 ) ) ;
#55871=CARTESIAN_POINT ( 'NONE',  ( -97.64999999999996305, -209.9999999999999716, 86.82500000000000284 ) ) ;
#55873=FACE_OUTER_BOUND ( 'NONE', #13054, .T. ) ;
#55875=CARTESIAN_POINT ( 'NONE',  ( 97.64999999999999147, 90.00000000000002842, 87.77749999999998920 ) ) ;
#55876=VERTEX_POINT ( 'NONE', #66173 ) ;
#55879=EDGE_CURVE ( 'NONE', #68271, #44941, #9755, .T. ) ;
#55881=CARTESIAN_POINT ( 'NONE',  ( 97.64999999999821512, -209.9999969335172807, 75.79187510780352000 ) ) ;
#55885=DIRECTION ( 'NONE',  ( 1.000000000000000000, 0.000000000000000000, 0.000000000000000000 ) ) ;
#55888=CARTESIAN_POINT ( 'NONE',  ( -97.30629616937497417, -211.3315407142195852, 79.69447916753381378 ) ) ;
#55897=CARTESIAN_POINT ( 'NONE',  ( 97.30629616937498838, 91.33154071421968467, 78.58322916753381548 ) ) ;
#55902=CARTESIAN_POINT ( 'NONE',  ( 95.77009744696134419, 92.23316662872740324, 74.81945665767625542 ) ) ;
#55908=CARTESIAN_POINT ( 'NONE',  ( -94.99999999999997158, -213.0599564267049857, 75.63312500173429953 ) ) ;
#55910=CARTESIAN_POINT ( 'NONE',  ( -96.15314808468752972, 91.99731107132950569, 83.82197916753381151 ) ) ;
#55915=FACE_OUTER_BOUND ( 'NONE', #45447, .T. ) ;
#55921=CARTESIAN_POINT ( 'NONE',  ( 92.69370383062501162, -209.9999999999999716, 80.27656250086714351 ) ) ;
#55928=CARTESIAN_POINT ( 'NONE',  ( -97.64999999999996305, -208.4700217866474645, 85.58145833506763722 ) ) ;
#55933=CARTESIAN_POINT ( 'NONE',  ( 92.35000000000002274, -208.4700217866474645, 87.40708333333333258 ) ) ;
#55940=CARTESIAN_POINT ( 'NONE',  ( -92.35000000000005116, 91.52997821335253548, 89.17979166840096639 ) ) ;
#55943=CARTESIAN_POINT ( 'NONE',  ( 97.64999999999999147, -209.9999999999999716, 80.87187500173430976 ) ) ;
#55944=CARTESIAN_POINT ( 'NONE',  ( 92.34999999999999432, 91.52997821335252127, 81.69208333333332916 ) ) ;
#55955=CARTESIAN_POINT ( 'NONE',  ( -96.15314808468751551, 88.00268892867056536, 83.55739583420049144 ) ) ;
#55956=CARTESIAN_POINT ( 'NONE',  ( 97.30629616937498838, 91.33154071421968467, 77.94822916753381037 ) ) ;
#55959=CARTESIAN_POINT ( 'NONE',  ( -97.65000000000001990, 90.00000000000004263, 80.47499999999999432 ) ) ;
#55963=CARTESIAN_POINT ( 'NONE',  ( -97.30629616937497417, -208.6684592857803011, 81.96989583420048575 ) ) ;
#55969=DIRECTION ( 'NONE',  ( 1.000000000000000000, 0.000000000000000000, 0.000000000000000000 ) ) ;
#55971=ORIENTED_EDGE ( 'NONE', *, *, #56467, .F. ) ;
#55972=CARTESIAN_POINT ( 'NONE',  ( -93.84685191531248449, -208.0026889286704943, 74.82614583420047438 ) ) ;
#55977=CARTESIAN_POINT ( 'NONE',  ( -2.500000000000015543, -73.00000000000001421, -208.2999999999999545 ) ) ;
#55980=CARTESIAN_POINT ( 'NONE',  ( 97.30629616937498838, 90.00000000000002842, 88.69031250086715090 ) ) ;
#55983=FACE_OUTER_BOUND ( 'NONE', #28036, .T. ) ;
#55987=CARTESIAN_POINT ( 'NONE',  ( -95.00000000000002842, 86.94004357329504273, 87.69812500173429726 ) ) ;
#55988=CARTESIAN_POINT ( 'NONE',  ( -95.00000000000002842, 93.05995642670504253, 75.87125000000000341 ) ) ;
#55991=EDGE_CURVE ( 'NONE', #30067, #62636, #510, .T. ) ;
#55993=FACE_OUTER_BOUND ( 'NONE', #48437, .T. ) ;
#55994=LINE ( 'NONE', #49970, #46708 ) ;
#55995=AXIS2_PLACEMENT_3D ( 'NONE', #55398, #62544, #43765 ) ;
#55996=CARTESIAN_POINT ( 'NONE',  ( -92.34999999999999432, -208.4700217866474645, 85.29041666666665833 ) ) ;
#56000=DIRECTION ( 'NONE',  ( 1.000000000000000000, 0.000000000000000000, 0.000000000000000000 ) ) ;
#56004=DIRECTION ( 'NONE',  ( 1.000000000000000000, 0.000000000000000000, 0.000000000000000000 ) ) ;
#56008=CARTESIAN_POINT ( 'NONE',  ( 95.00000000000000000, -212.6630814284392557, 88.05531250086716000 ) ) ;
#56012=DIRECTION ( 'NONE',  ( 1.000000000000000000, 0.000000000000000000, 0.000000000000000000 ) ) ;
#56016=CARTESIAN_POINT ( 'NONE',  ( 92.69370383062501162, -208.6684592857803295, 79.42989583420047950 ) ) ;
#56019=CARTESIAN_POINT ( 'NONE',  ( 92.69370383062501162, -208.6684592857803011, 85.30364583420048064 ) ) ;
#56028=CARTESIAN_POINT ( 'NONE',  ( -97.65000000000006253, 88.47002178664756400, 77.35291666666665833 ) ) ;
#56029=CARTESIAN_POINT ( 'NONE',  ( 92.35000000000002274, -208.4700217866474645, 88.75645833506762017 ) ) ;
#56035=( BOUNDED_CURVE ( )  B_SPLINE_CURVE ( 2, ( #64492, #58474, #64133, #6254, #2118, #70857, #12607 ),
 .UNSPECIFIED., .F., .F. ) 
 B_SPLINE_CURVE_WITH_KNOTS ( ( 3, 2, 2, 3 ),
 ( 0.9166666666666662966, 0.9236111111111108274, 0.9305555555555551361, 0.9374999999999995559 ),
 .UNSPECIFIED. ) 
 CURVE ( )  GEOMETRIC_REPRESENTATION_ITEM ( )  RATIONAL_B_SPLINE_CURVE ( ( 1.000000000000006439, 0.8660254037844322683, 1.000000000000000000, 0.8660254037844387076, 1.000000000000000000, 0.8660254037844472563, 0.9999999999999914513 ) ) 
 REPRESENTATION_ITEM ( '' )  );
#56043=CARTESIAN_POINT ( 'NONE',  ( 95.00000000000000000, -212.6630814284392557, 76.46656250086712703 ) ) ;
#56052=B_SPLINE_CURVE_WITH_KNOTS ( 'NONE', 1,
 ( #45366, #61165 ),
 .UNSPECIFIED., .F., .F.,
 ( 2, 2 ),
 ( 0.000000000000000000, 1.000000000000000000 ),
 .UNSPECIFIED. ) ;
#56053=CARTESIAN_POINT ( 'NONE',  ( -97.64999999999996305, -209.9999999999999716, 88.73000000000000398 ) ) ;
#56054=CARTESIAN_POINT ( 'NONE',  ( -95.00000000000002842, 87.33691857156074434, 75.35531250086715715 ) ) ;
#56055=ORIENTED_EDGE ( 'NONE', *, *, #7216, .T. ) ;
#56057=CARTESIAN_POINT ( 'NONE',  ( 96.15314808468748708, 91.99731107132950569, 76.73114583420047552 ) ) ;
#56060=CARTESIAN_POINT ( 'NONE',  ( -93.84685191531248449, -208.0026889286704943, 89.43114583420047836 ) ) ;
#56063=DIRECTION ( 'NONE',  ( -0.000000000000000000, -0.000000000000000000, 1.000000000000000000 ) ) ;
#56066=CARTESIAN_POINT ( 'NONE',  ( -92.69370383062498320, -211.3315407142195852, 81.01739583420048518 ) ) ;
#56068=DIRECTION ( 'NONE',  ( 1.000000000000000000, 0.000000000000000000, 0.000000000000000000 ) ) ;
#56069=CARTESIAN_POINT ( 'NONE',  ( -94.99999999999997158, -206.9400435732949575, 84.12624999999999886 ) ) ;
#56076=LINE ( 'NONE', #33498, #45181 ) ;
#56077=CARTESIAN_POINT ( 'NONE',  ( -95.00000000000002842, 92.66308142843932671, 81.22906250086715829 ) ) ;
#56088=CARTESIAN_POINT ( 'NONE',  ( -97.30629616937497417, -208.6684592857803011, 78.31864583420050963 ) ) ;
#56089=EDGE_CURVE ( 'NONE', #13197, #49491, #37608, .T. ) ;
#56107=CARTESIAN_POINT ( 'NONE',  ( 93.67499999999998295, 92.29496732002878900, 78.46416666666667084 ) ) ;
#56108=CARTESIAN_POINT ( 'NONE',  ( -94.99999999999997158, -209.9999999999999716, 90.00000000000000000 ) ) ;
#56110=CARTESIAN_POINT ( 'NONE',  ( 96.15314808468748708, -208.0026889286704943, 88.16114583420046813 ) ) ;
#56111=CARTESIAN_POINT ( 'NONE',  ( 97.64999999999999147, -209.9999999999999716, 85.87249999999998806 ) ) ;
#56117=VERTEX_POINT ( 'NONE', #40550 ) ;
#56128=CARTESIAN_POINT ( 'NONE',  ( 96.15314808468748708, 91.99731107132950569, 78.15989583420049769 ) ) ;
#56129=DIRECTION ( 'NONE',  ( -0.000000000000000000, -0.000000000000000000, 1.000000000000000000 ) ) ;
#56134=CARTESIAN_POINT ( 'NONE',  ( 97.30629616937498838, 88.66845928578037217, 87.36739583420047950 ) ) ;
#56136=CARTESIAN_POINT ( 'NONE',  ( 96.15314808468748708, -208.0026889286704943, 86.25614583420048120 ) ) ;
#56139=CARTESIAN_POINT ( 'NONE',  ( -95.00000000000002842, 93.05995642670504253, 77.22062500173429100 ) ) ;
#56142=DIRECTION ( 'NONE',  ( -0.000000000000000000, -0.000000000000000000, 1.000000000000000000 ) ) ;
#56144=CARTESIAN_POINT ( 'NONE',  ( -97.30629616937497417, -208.6684592857803011, 87.68489583420047495 ) ) ;
#56145=CARTESIAN_POINT ( 'NONE',  ( -92.69370383062502583, 91.33154071421968467, 86.36197916753383197 ) ) ;
#56147=CARTESIAN_POINT ( 'NONE',  ( 94.99999999999998579, 87.33691857156068750, 87.89656250086713385 ) ) ;
#56148=CARTESIAN_POINT ( 'NONE',  ( -92.69370383062504004, 90.00000000000004263, 88.05531250086713158 ) ) ;
#56155=CARTESIAN_POINT ( 'NONE',  ( -97.30629616937497417, -208.6684592857803295, 88.95489583420048518 ) ) ;
#56163=CARTESIAN_POINT ( 'NONE',  ( -97.65000000000001990, 88.47002178664754979, 82.43291666666665662 ) ) ;
#56165=CARTESIAN_POINT ( 'NONE',  ( 97.64999999999999147, -209.9999999999999716, 75.71250000000000568 ) ) ;
#56166=DIRECTION ( 'NONE',  ( -0.000000000000000000, -0.000000000000000000, 1.000000000000000000 ) ) ;
#56170=CARTESIAN_POINT ( 'NONE',  ( -97.64999999980591383, 89.99998015720542810, 86.27002759516649633 ) ) ;
#56173=CARTESIAN_POINT ( 'NONE',  ( -97.30629616937501680, 91.33154071421968467, 80.69989583420048973 ) ) ;
#56175=CARTESIAN_POINT ( 'NONE',  ( 97.64999322989690711, 88.47001787792670768, 82.72395806468932733 ) ) ;
#56178=AXIS2_PLACEMENT_3D ( 'NONE', #63812, #6654, #64540 ) ;
#56180=LINE ( 'NONE', #44541, #4501 ) ;
#56186=VECTOR ( 'NONE', #71878, 1000.000000000000000 ) ;
#56188=CARTESIAN_POINT ( 'NONE',  ( 97.30629616937498838, 88.66845928578035796, 81.81114583420048803 ) ) ;
#56189=CARTESIAN_POINT ( 'NONE',  ( -94.99999999999997158, -207.3369185715606307, 78.84781250086714977 ) ) ;
#56193=CARTESIAN_POINT ( 'NONE',  ( 95.00000000000000000, -206.9400435732949575, 81.03062500173430749 ) ) ;
#56195=CARTESIAN_POINT ( 'NONE',  ( 92.35000000049295465, 89.99996796756887818, 85.63541623677173220 ) ) ;
#56196=CARTESIAN_POINT ( 'NONE',  ( -96.15314808468751551, 88.00268892867056536, 79.74739583420048916 ) ) ;
#56197=CARTESIAN_POINT ( 'NONE',  ( 95.00000000000000000, -207.3369185715606307, 81.22906250086715829 ) ) ;
#56199=CARTESIAN_POINT ( 'NONE',  ( 97.24889018994932144, 89.40965860031440116, 74.79348190356850523 ) ) ;
#56215=CARTESIAN_POINT ( 'NONE',  ( 97.64999999999999147, -209.9999999999999716, 75.71250000000000568 ) ) ;
#56220=CARTESIAN_POINT ( 'NONE',  ( 93.84685191531248449, 88.00268892867053694, 87.36739583420049371 ) ) ;
#56221=CARTESIAN_POINT ( 'NONE',  ( 97.64999999999999147, 89.99999997928482287, 80.87187500099604165 ) ) ;
#56222=CARTESIAN_POINT ( 'NONE',  ( 93.67500000000001137, -212.2949673200287179, 78.04083333333333883 ) ) ;
#56228=CARTESIAN_POINT ( 'NONE',  ( 97.64999999999999147, -209.9999999999999716, 89.04749999999999943 ) ) ;
#56235=DIRECTION ( 'NONE',  ( 0.000000000000000000, -0.000000000000000000, -1.000000000000000000 ) ) ;
#56236=VECTOR ( 'NONE', #46292, 1000.000000000000000 ) ;
#56237=VERTEX_POINT ( 'NONE', #70954 ) ;
#56238=CARTESIAN_POINT ( 'NONE',  ( -92.34999999999999432, -208.4700217866474645, 81.55979166840097605 ) ) ;
#56239=ORIENTED_EDGE ( 'NONE', *, *, #21732, .T. ) ;
#56242=CARTESIAN_POINT ( 'NONE',  ( 93.67499999999999716, 87.70503267997126784, 81.29520833506762756 ) ) ;
#56243=CARTESIAN_POINT ( 'NONE',  ( -92.35000000000003695, 90.00000000000004263, 82.77687500173431090 ) ) ;
#56244=STYLED_ITEM ( 'NONE', ( #20309 ), #36766 ) ;
#56246=CARTESIAN_POINT ( 'NONE',  ( 94.99999999999998579, 92.66308142843935514, 83.92781250086716227 ) ) ;
#56253=CARTESIAN_POINT ( 'NONE',  ( 96.32499999999998863, -207.7050326799711968, 77.72333333333332916 ) ) ;
#56261=( BOUNDED_CURVE ( )  B_SPLINE_CURVE ( 2, ( #64017, #63653, #35064, #23418, #33950, #69643, #165 ),
 .UNSPECIFIED., .F., .F. ) 
 B_SPLINE_CURVE_WITH_KNOTS ( ( 3, 2, 2, 3 ),
 ( 0.6875000000000000000, 0.6944444444444443088, 0.7013888888888887285, 0.7083333333333331483 ),
 .UNSPECIFIED. ) 
 CURVE ( )  GEOMETRIC_REPRESENTATION_ITEM ( )  RATIONAL_B_SPLINE_CURVE ( ( 1.000000000000000000, 0.8660254037844387076, 1.000000000000000000, 0.8660254037844387076, 1.000000000000000000, 0.8660254037844430375, 0.9999999999999956701 ) ) 
 REPRESENTATION_ITEM ( '' )  );
#56262=CARTESIAN_POINT ( 'NONE',  ( -96.15314808468747287, -208.0026889286704943, 82.71072916753381321 ) ) ;
#56265=ORIENTED_EDGE ( 'NONE', *, *, #14582, .T. ) ;
#56270=CARTESIAN_POINT ( 'NONE',  ( 92.34999999999999432, 90.00000000000002842, 90.00000000000000000 ) ) ;
#56273=DIRECTION ( 'NONE',  ( -0.8571673007021122226, 1.049727191138618572E-16, 0.5150380749100542666 ) ) ;
#56278=DIRECTION ( 'NONE',  ( 1.000000000000000000, 0.000000000000000000, 0.000000000000000000 ) ) ;
#56279=CYLINDRICAL_SURFACE ( 'NONE', #59278, 23.50000000000000355 ) ;
#56284=CARTESIAN_POINT ( 'NONE',  ( 97.65000000000009095, -211.5299782133523649, 83.27958333333332064 ) ) ;
#56289=CARTESIAN_POINT ( 'NONE',  ( -96.15314808468752972, 91.99731107132950569, 80.01197916753380923 ) ) ;
#56294=CARTESIAN_POINT ( 'NONE',  ( 92.69370383062501162, -209.9999999999999716, 89.64281250086713726 ) ) ;
#56295=ORIENTED_EDGE ( 'NONE', *, *, #7290, .F. ) ;
#56300=CARTESIAN_POINT ( 'NONE',  ( -92.35000000000003695, 90.00000000000004263, 90.00000000000000000 ) ) ;
#56303=CARTESIAN_POINT ( 'NONE',  ( 97.30629616937498838, -208.6684592857803011, 76.20197916753382117 ) ) ;
#56304=ORIENTED_EDGE ( 'NONE', *, *, #33689, .T. ) ;
#56305=EDGE_LOOP ( 'NONE', ( #16763, #32325, #8107, #39327 ) ) ;
#56313=CARTESIAN_POINT ( 'NONE',  ( 97.64999999999997726, -208.4700217866474645, 88.46541666666665549 ) ) ;
#56316=EDGE_LOOP ( 'NONE', ( #8783, #31338, #13040, #59456 ) ) ;
#56317=CARTESIAN_POINT ( 'NONE',  ( -92.34999999999996589, -208.4700217866474645, 87.83041666666669300 ) ) ;
#56324=ORIENTED_EDGE ( 'NONE', *, *, #62784, .F. ) ;
#56325=CARTESIAN_POINT ( 'NONE',  ( 97.64999999999997726, 88.47002178664752137, 87.72458333333332803 ) ) ;
#56326=CARTESIAN_POINT ( 'NONE',  ( 93.67500000000001137, -207.7050326799711968, 79.17854166840096752 ) ) ;
#56327=CARTESIAN_POINT ( 'NONE',  ( 96.32499999999997442, 92.29496732002878900, 81.53333333333333144 ) ) ;
#56334=CARTESIAN_POINT ( 'NONE',  ( -95.00000000000002842, 92.66308142843932671, 83.29281250086715715 ) ) ;
#56335=CARTESIAN_POINT ( 'NONE',  ( 94.99999999999998579, 92.66308142843935514, 79.95906250086713385 ) ) ;
#56339=DIRECTION ( 'NONE',  ( 1.000000000000000000, 0.000000000000000000, 0.000000000000000000 ) ) ;
#56340=AXIS2_PLACEMENT_3D ( 'NONE', #53382, #7883, #1919 ) ;
#56341=CARTESIAN_POINT ( 'NONE',  ( 97.64999999964362587, 89.99995654222556141, 89.12687334326064104 ) ) ;
#56344=CARTESIAN_POINT ( 'NONE',  ( -96.32499999999996021, -212.2949673200287179, 86.29583333333333428 ) ) ;
#56347=CARTESIAN_POINT ( 'NONE',  ( -94.99999999999997158, -207.3369185715606307, 77.41906250086714181 ) ) ;
#56353=ORIENTED_EDGE ( 'NONE', *, *, #58583, .F. ) ;
#56358=CARTESIAN_POINT ( 'NONE',  ( -97.30629616937495996, -209.9999999999999716, 75.03781250086713328 ) ) ;
#56360=CARTESIAN_POINT ( 'NONE',  ( 93.67499999999998295, 92.29496732002878900, 88.70354166840097321 ) ) ;
#56366=EDGE_CURVE ( 'NONE', #40438, #18610, #49710, .T. ) ;
#56368=CARTESIAN_POINT ( 'NONE',  ( 94.99999999999998579, 87.33691857156068750, 84.08656250086714579 ) ) ;
#56375=CARTESIAN_POINT ( 'NONE',  ( -97.64999999969894873, 90.00002455906438570, 87.53856274002211535 ) ) ;
#56379=CARTESIAN_POINT ( 'NONE',  ( 93.67499999999999716, 87.70503267997126784, 78.67583333333332973 ) ) ;
#56384=CYLINDRICAL_SURFACE ( 'NONE', #55675, 2.649999999999999467 ) ;
#56386=CARTESIAN_POINT ( 'NONE',  ( -96.32499999999996021, -207.7050326799711968, 83.54416666666666913 ) ) ;
#56389=ADVANCED_FACE ( 'NONE', ( #55156 ), #61552, .F. ) ;
#56399=CARTESIAN_POINT ( 'NONE',  ( 95.00000000000000000, -212.6630814284392557, 87.42031250086715488 ) ) ;
#56405=ORIENTED_EDGE ( 'NONE', *, *, #53911, .F. ) ;
#56407=CARTESIAN_POINT ( 'NONE',  ( 95.00000000000000000, -207.3369185715606307, 76.78406250086712248 ) ) ;
#56409=CARTESIAN_POINT ( 'NONE',  ( 92.69370383062501162, -209.9999999999999716, 82.81656250086714977 ) ) ;
#56413=CARTESIAN_POINT ( 'NONE',  ( -93.33922900947484891, 88.39973697852397549, 74.80065534806809069 ) ) ;
#56416=CARTESIAN_POINT ( 'NONE',  ( 96.32499999999998863, -212.2949673200287179, 76.95604166840095672 ) ) ;
#56418=ORIENTED_EDGE ( 'NONE', *, *, #45856, .F. ) ;
#56420=EDGE_LOOP ( 'NONE', ( #31706, #24995, #41892 ) ) ;
#56423=VERTEX_POINT ( 'NONE', #40459 ) ;
#56424=VECTOR ( 'NONE', #3510, 1000.000000000000000 ) ;
#56427=CARTESIAN_POINT ( 'NONE',  ( 97.30629616937498838, -209.9999999999999716, 75.99031250086714806 ) ) ;
#56430=ORIENTED_EDGE ( 'NONE', *, *, #18608, .F. ) ;
#56432=ORIENTED_EDGE ( 'NONE', *, *, #39737, .T. ) ;
#56434=CARTESIAN_POINT ( 'NONE',  ( 95.00000000000000000, -209.9999999999999716, 90.00000000000000000 ) ) ;
#56436=EDGE_CURVE ( 'NONE', #44823, #20714, #39358, .T. ) ;
#56437=CARTESIAN_POINT ( 'NONE',  ( -95.00000000000002842, 92.66308142843932671, 76.30781250086715772 ) ) ;
#56443=CARTESIAN_POINT ( 'NONE',  ( -93.84685191531247028, -211.9973110713294489, 86.04447916753380809 ) ) ;
#56445=CARTESIAN_POINT ( 'NONE',  ( 96.92442009029420547, -211.8218417373832096, 75.00000000000001421 ) ) ;
#56449=CARTESIAN_POINT ( 'NONE',  ( -97.30629616937497417, -211.3315407142195852, 79.53572916753380184 ) ) ;
#56450=ADVANCED_FACE ( 'NONE', ( #34827 ), #4028, .F. ) ;
#56454=VECTOR ( 'NONE', #25844, 1000.000000000000000 ) ;
#56464=CARTESIAN_POINT ( 'NONE',  ( -95.00000000000002842, 92.66308142843932671, 80.59406250086715318 ) ) ;
#56467=EDGE_CURVE ( 'NONE', #65091, #16429, #5999, .T. ) ;
#56469=CARTESIAN_POINT ( 'NONE',  ( -0.0004442498525516064278, 0.001194404164626844313, -64.00000000000000000 ) ) ;
#56471=CARTESIAN_POINT ( 'NONE',  ( -97.30629616937495996, -209.9999999999999716, 89.64281250086713726 ) ) ;
#56475=CARTESIAN_POINT ( 'NONE',  ( 92.35000000000002274, -210.0000343786552719, 88.80937619077336365 ) ) ;
#56476=CARTESIAN_POINT ( 'NONE',  ( -94.99999999999997158, -212.6630814284392557, 78.53031250086715431 ) ) ;
#56482=CARTESIAN_POINT ( 'NONE',  ( -93.67500000000003979, 92.29496732002878900, 88.51833333333333087 ) ) ;
#56484=ORIENTED_EDGE ( 'NONE', *, *, #59234, .F. ) ;
#56494=( BOUNDED_CURVE ( )  B_SPLINE_CURVE ( 2, ( #70066, #6209, #6567, #28746, #57703, #35498, #63718 ),
 .UNSPECIFIED., .F., .F. ) 
 B_SPLINE_CURVE_WITH_KNOTS ( ( 3, 2, 2, 3 ),
 ( 0.6350190250571088324, 0.6420746642202954657, 0.6491304297611778518, 0.6561861948910820974 ),
 .UNSPECIFIED. ) 
 CURVE ( )  GEOMETRIC_REPRESENTATION_ITEM ( )  RATIONAL_B_SPLINE_CURVE ( ( 0.9999952007766141904, 0.8660278034391124535, 1.000000000000000000, 0.8660254037844387076, 1.000000000000000000, 0.8660254037844387076, 1.000000000000000000 ) ) 
 REPRESENTATION_ITEM ( '' )  );
#56498=CARTESIAN_POINT ( 'NONE',  ( -2.499999999999970690, 73.00000000000001421, -204.9999999999999716 ) ) ;
#56499=VECTOR ( 'NONE', #63391, 1000.000000000000000 ) ;
#56510=ADVANCED_FACE ( 'NONE', ( #63052 ), #56279, .F. ) ;
#56513=CARTESIAN_POINT ( 'NONE',  ( 93.67499999999999716, 87.70503267997126784, 87.56583333333333030 ) ) ;
#56519=CARTESIAN_POINT ( 'NONE',  ( 92.69370383062498320, 90.00000000000002842, 88.37281250086715545 ) ) ;
#56521=CARTESIAN_POINT ( 'NONE',  ( 95.00000000000000000, -207.3369185715606307, 83.76906250086713612 ) ) ;
#56530=CARTESIAN_POINT ( 'NONE',  ( -94.99999999999997158, -212.6630814284392557, 88.53156250086713897 ) ) ;
#56532=CARTESIAN_POINT ( 'NONE',  ( -97.30629616937501680, 91.33154071421968467, 84.66864583420047552 ) ) ;
#56534=CARTESIAN_POINT ( 'NONE',  ( 97.30629616937498838, 91.33154071421968467, 87.47322916753381605 ) ) ;
#56535=CARTESIAN_POINT ( 'NONE',  ( -96.15314808468752972, 91.99731107132950569, 86.36197916753381776 ) ) ;
#56540=CARTESIAN_POINT ( 'NONE',  ( 97.64999999999324132, 90.00000598221777182, 82.14187520865721126 ) ) ;
#56541=CARTESIAN_POINT ( 'NONE',  ( -97.65000000000001990, 90.00000000000004263, 86.82500000000000284 ) ) ;
#56544=EDGE_CURVE ( 'NONE', #47972, #47168, #51002, .T. ) ;
#56552=CARTESIAN_POINT ( 'NONE',  ( -93.67500000000003979, 92.29496732002878900, 80.26333333333332121 ) ) ;
#56554=CARTESIAN_POINT ( 'NONE',  ( 92.34999999999995168, -208.4700217866474929, 75.97708333333333997 ) ) ;
#56563=CARTESIAN_POINT ( 'NONE',  ( -92.69370383062502583, 91.33154071421968467, 79.21822916753380639 ) ) ;
#56571=CARTESIAN_POINT ( 'NONE',  ( -97.65000000000001990, 90.00000000000004263, 89.44437500173430067 ) ) ;
#56572=CARTESIAN_POINT ( 'NONE',  ( -94.99999999999997158, -207.3369185715606307, 89.64281250086715147 ) ) ;
#56575=ADVANCED_FACE ( 'NONE', ( #58872 ), #6621, .F. ) ;
#56576=CARTESIAN_POINT ( 'NONE',  ( 97.30629616937498838, 88.66845928578035796, 79.90614583420048689 ) ) ;
#56577=CARTESIAN_POINT ( 'NONE',  ( -97.30629616937495996, -209.9999999999999716, 79.64156250086715261 ) ) ;
#56580=CARTESIAN_POINT ( 'NONE',  ( -97.65000000000001990, 88.47002178664754979, 86.95729166840096980 ) ) ;
#56581=CARTESIAN_POINT ( 'NONE',  ( -94.99999999999997158, -213.0599564267049857, 75.55375000000000796 ) ) ;
#56583=CARTESIAN_POINT ( 'NONE',  ( -97.30629616937501680, 91.33154071421968467, 78.95364583420045790 ) ) ;
#56584=CARTESIAN_POINT ( 'NONE',  ( 96.15314808468748708, -208.0026889286704943, 79.27114583420046756 ) ) ;
#56589=ORIENTED_EDGE ( 'NONE', *, *, #57672, .F. ) ;
#56596=ORIENTED_EDGE ( 'NONE', *, *, #32088, .T. ) ;
#56598=CARTESIAN_POINT ( 'NONE',  ( 96.15314808468748708, -208.0026889286704943, 74.98489583420048632 ) ) ;
#56601=EDGE_CURVE ( 'NONE', #27271, #44954, #44393, .T. ) ;
#56602=CARTESIAN_POINT ( 'NONE',  ( 96.15314808468748708, 91.99731107132950569, 86.41489583420049314 ) ) ;
#56604=CARTESIAN_POINT ( 'NONE',  ( 93.67500000000001137, -212.2949673200287179, 79.31083333333333485 ) ) ;
#56605=ORIENTED_EDGE ( 'NONE', *, *, #35391, .F. ) ;
#56619=CARTESIAN_POINT ( 'NONE',  ( -97.64995850092280705, -211.5300021728558022, 83.78229332575403987 ) ) ;
#56621=CARTESIAN_POINT ( 'NONE',  ( -97.64999999999994884, -208.4700217866474645, 81.77145833506763495 ) ) ;
#56623=CARTESIAN_POINT ( 'NONE',  ( 94.99999999999998579, 90.00000000000002842, 75.00000000000000000 ) ) ;
#56625=CARTESIAN_POINT ( 'NONE',  ( 94.99999999999998579, 86.94004357329500010, 83.25312500173430408 ) ) ;
#56626=CARTESIAN_POINT ( 'NONE',  ( -96.32500000000001705, 92.29496732002878900, 79.17854166840096752 ) ) ;
#56629=CARTESIAN_POINT ( 'NONE',  ( 94.99999999999998579, 92.66308142843935514, 82.65781250086715204 ) ) ;
#56630=CARTESIAN_POINT ( 'NONE',  ( -97.64999999999999147, -208.4700217866475498, 86.77208333333334167 ) ) ;
#56636=ORIENTED_EDGE ( 'NONE', *, *, #25460, .T. ) ;
#56638=CARTESIAN_POINT ( 'NONE',  ( 92.35000000009274856, -209.9999861897330788, 80.55392363656960697 ) ) ;
#56647=CARTESIAN_POINT ( 'NONE',  ( -94.99999999999997158, -212.6630814284392557, 80.43531250086715545 ) ) ;
#56651=ORIENTED_EDGE ( 'NONE', *, *, #71115, .T. ) ;
#56655=CARTESIAN_POINT ( 'NONE',  ( 92.34999999999999432, 90.00000000000002842, 81.82437500173429612 ) ) ;
#56658=CYLINDRICAL_SURFACE ( 'NONE', #46455, 2.649999999999985700 ) ;
#56665=EDGE_CURVE ( 'NONE', #18290, #58390, #747, .T. ) ;
#56672=CARTESIAN_POINT ( 'NONE',  ( -93.84685191531252713, 88.00268892867056536, 80.96447916753380980 ) ) ;
#56677=CARTESIAN_POINT ( 'NONE',  ( 95.00000000000000000, -213.0599564267049857, 80.07812500173429271 ) ) ;
#56681=CARTESIAN_POINT ( 'NONE',  ( 97.30629616937498838, -211.3315407142195852, 76.09614583420048461 ) ) ;
#56689=CARTESIAN_POINT ( 'NONE',  ( 93.67500000000001137, -212.2949673200287179, 87.56583333333333030 ) ) ;
#56696=ORIENTED_EDGE ( 'NONE', *, *, #34235, .T. ) ;
#56698=FACE_OUTER_BOUND ( 'NONE', #19263, .T. ) ;
#56705=CARTESIAN_POINT ( 'NONE',  ( 97.64999999999997726, -211.5299782133524502, 75.10395833506764518 ) ) ;
#56707=CARTESIAN_POINT ( 'NONE',  ( 92.34999999999999432, 88.47002178664753558, 83.06791666666664753 ) ) ;
#56714=CARTESIAN_POINT ( 'NONE',  ( 97.65000000000000568, 88.47002178664752137, 84.62895833506763665 ) ) ;
#56717=( BOUNDED_CURVE ( )  B_SPLINE_CURVE ( 2, ( #53954, #32110, #65984, #7711, #71214, #48304, #26480 ),
 .UNSPECIFIED., .F., .T. ) 
 B_SPLINE_CURVE_WITH_KNOTS ( ( 3, 2, 2, 3 ),
 ( 0.4583333333333335924, 0.4652777777777780122, 0.4722222222222224319, 0.4791666666666668517 ),
 .UNSPECIFIED. ) 
 CURVE ( )  GEOMETRIC_REPRESENTATION_ITEM ( )  RATIONAL_B_SPLINE_CURVE ( ( 0.9999999999999946709, 0.8660254037844440367, 1.000000000000000000, 0.8660254037844387076, 1.000000000000000000, 0.8660254037844354880, 1.000000000000003109 ) ) 
 REPRESENTATION_ITEM ( '' )  );
#56718=CARTESIAN_POINT ( 'NONE',  ( -95.00000000000002842, 87.33691857156074434, 82.97531250086714749 ) ) ;
#56719=CARTESIAN_POINT ( 'NONE',  ( 93.84685191531248449, 91.99731107132950569, 77.47197916753380298 ) ) ;
#56722=CARTESIAN_POINT ( 'NONE',  ( -95.00000000000002842, 90.00000000000004263, 90.00000000000000000 ) ) ;
#56729=CARTESIAN_POINT ( 'NONE',  ( -93.84685191531248449, -208.0026889286704943, 76.73114583420047552 ) ) ;
#56734=CARTESIAN_POINT ( 'NONE',  ( 97.64999999999999147, 90.00000000000002842, 78.25249999999999773 ) ) ;
#56736=ORIENTED_EDGE ( 'NONE', *, *, #42466, .T. ) ;
#56737=CARTESIAN_POINT ( 'NONE',  ( -97.30629616937497417, -208.6684592857803011, 74.98489583420048632 ) ) ;
#56739=DIRECTION ( 'NONE',  ( -0.000000000000000000, -0.000000000000000000, -1.000000000000000000 ) ) ;
#56746=CARTESIAN_POINT ( 'NONE',  ( 94.99999999999998579, 87.33691857156068750, 84.72156250086713669 ) ) ;
#56752=CARTESIAN_POINT ( 'NONE',  ( 92.35000000000002274, -209.9999719686936430, 87.53937403222813884 ) ) ;
#56755=CARTESIAN_POINT ( 'NONE',  ( 92.34999999999999432, 90.00000000000002842, 78.57000000000000739 ) ) ;
#56758=CARTESIAN_POINT ( 'NONE',  ( -99.99999999999997158, -204.9999999999999716, 90.00000000000000000 ) ) ;
#56761=CARTESIAN_POINT ( 'NONE',  ( -94.99999999999997158, -213.0599564267049857, 83.80875000000000341 ) ) ;
#56770=CARTESIAN_POINT ( 'NONE',  ( 95.00000000000000000, -212.6630814284392557, 86.78531250086716398 ) ) ;
#56776=CARTESIAN_POINT ( 'NONE',  ( 96.15314808468750130, -211.9973110713294489, 79.69447916753379957 ) ) ;
#56778=CARTESIAN_POINT ( 'NONE',  ( 96.15314808468750130, -211.9973110713294489, 84.29822916753381890 ) ) ;
#56779=VERTEX_POINT ( 'NONE', #62101 ) ;
#56782=VERTEX_POINT ( 'NONE', #60981 ) ;
#56788=CARTESIAN_POINT ( 'NONE',  ( 95.00000000000000000, -206.9400435732949575, 85.47562500173431488 ) ) ;
#56799=CARTESIAN_POINT ( 'NONE',  ( 92.69370383062501162, -211.3315407142195852, 75.09072916753382287 ) ) ;
#56805=DIRECTION ( 'NONE',  ( -4.476705744456277943E-17, 1.000000000000000000, -0.000000000000000000 ) ) ;
#56807=EDGE_CURVE ( 'NONE', #48269, #21245, #71145, .T. ) ;
#56808=CARTESIAN_POINT ( 'NONE',  ( -92.69370383062502583, 88.66845928578038638, 76.09614583420048461 ) ) ;
#56815=CARTESIAN_POINT ( 'NONE',  ( -94.99999999999997158, -207.3369185715606307, 86.30906250086715659 ) ) ;
#56818=CARTESIAN_POINT ( 'NONE',  ( 96.74471819418084806, -211.6811075874703931, 74.86350982016034550 ) ) ;
#56821=CARTESIAN_POINT ( 'NONE',  ( -96.15314808468747287, -208.0026889286704943, 74.93197916753379673 ) ) ;
#56830=CARTESIAN_POINT ( 'NONE',  ( -92.34999999999999432, -209.9999999999999716, 90.00000000000000000 ) ) ;
#56831=CARTESIAN_POINT ( 'NONE',  ( -93.84685191531252713, 88.00268892867056536, 82.86947916753379673 ) ) ;
#56840=DIRECTION ( 'NONE',  ( -0.000000000000000000, -0.000000000000000000, -1.000000000000000000 ) ) ;
#56841=CARTESIAN_POINT ( 'NONE',  ( -97.30629616937495996, -209.9999999999999716, 79.64156250086715261 ) ) ;
#56842=CYLINDRICAL_SURFACE ( 'NONE', #30868, 2.649999999999985700 ) ;
#56850=DIRECTION ( 'NONE',  ( 1.000000000000000000, 0.000000000000000000, 0.000000000000000000 ) ) ;
#56855=CARTESIAN_POINT ( 'NONE',  ( 97.64999999999999147, -209.9999999999999716, 90.00000000000000000 ) ) ;
#56856=EDGE_LOOP ( 'NONE', ( #27143, #66403 ) ) ;
#56866=ORIENTED_EDGE ( 'NONE', *, *, #6461, .T. ) ;
#56868=CARTESIAN_POINT ( 'NONE',  ( -97.64999999996706492, -209.9999916046304520, 84.99910573338409847 ) ) ;
#56878=VERTEX_POINT ( 'NONE', #63597 ) ;
#56880=CARTESIAN_POINT ( 'NONE',  ( 97.64999999999997726, 88.47002178664753558, 89.62958333333332916 ) ) ;
#56888=CARTESIAN_POINT ( 'NONE',  ( 92.69370383062498320, 90.00000000000002842, 84.56281250086713897 ) ) ;
#56890=CARTESIAN_POINT ( 'NONE',  ( 95.00000000000000000, -207.3369185715606307, 85.67406250086715147 ) ) ;
#56893=CARTESIAN_POINT ( 'NONE',  ( 92.34999999999999432, 90.00000000000002842, 75.39499999999999602 ) ) ;
#56894=CARTESIAN_POINT ( 'NONE',  ( -97.65000000000001990, 91.52997821335253548, 77.96145833506763267 ) ) ;
#56898=CARTESIAN_POINT ( 'NONE',  ( -92.69370383062498320, -208.6684592857803011, 86.20322916753382003 ) ) ;
#56900=CARTESIAN_POINT ( 'NONE',  ( -92.69370383062502583, 88.66845928578038638, 86.25614583420048120 ) ) ;
#56902=ORIENTED_EDGE ( 'NONE', *, *, #70230, .F. ) ;
#56904=CARTESIAN_POINT ( 'NONE',  ( 96.15314808468748708, 88.00268892867053694, 82.86947916753379673 ) ) ;
#56905=CARTESIAN_POINT ( 'NONE',  ( -96.15314808468751551, 88.00268892867056536, 84.03364583420047040 ) ) ;
#56908=CARTESIAN_POINT ( 'NONE',  ( -97.64999999999996305, -209.9999844236418198, 80.55437446300184945 ) ) ;
#56911=CARTESIAN_POINT ( 'NONE',  ( -92.69370383062498320, -211.3315407142195852, 89.27239583420048064 ) ) ;
#56912=CARTESIAN_POINT ( 'NONE',  ( -97.64999999999992042, -211.5299782133524218, 81.79791666666665151 ) ) ;
#56915=CARTESIAN_POINT ( 'NONE',  ( 92.35000000000003695, 88.47002178664747873, 89.41791666666667027 ) ) ;
#56919=CARTESIAN_POINT ( 'NONE',  ( -97.65000000000001990, 90.00000000000004263, 79.20499999999999829 ) ) ;
#56920=CYLINDRICAL_SURFACE ( 'NONE', #69160, 2.649999999999985700 ) ;
#56923=CARTESIAN_POINT ( 'NONE',  ( -97.64999999999996305, -209.9999999999999716, 90.00000000000000000 ) ) ;
#56924=DIRECTION ( 'NONE',  ( -0.000000000000000000, -0.000000000000000000, 1.000000000000000000 ) ) ;
#56926=( BOUNDED_CURVE ( )  B_SPLINE_CURVE ( 2, ( #5334, #28232, #6077, #50794, #57569, #18080, #51167 ),
 .UNSPECIFIED., .F., .F. ) 
 B_SPLINE_CURVE_WITH_KNOTS ( ( 3, 2, 2, 3 ),
 ( 0.8749999999999997780, 0.8819444444444441977, 0.8888888888888886175, 0.8958333333333331483 ),
 .UNSPECIFIED. ) 
 CURVE ( )  GEOMETRIC_REPRESENTATION_ITEM ( )  RATIONAL_B_SPLINE_CURVE ( ( 1.000000000000004219, 0.8660254037844343777, 1.000000000000000000, 0.8660254037844387076, 1.000000000000000000, 0.8660254037844430375, 0.9999999999999956701 ) ) 
 REPRESENTATION_ITEM ( '' )  );
#56929=VERTEX_POINT ( 'NONE', #52662 ) ;
#56930=CARTESIAN_POINT ( 'NONE',  ( -93.84685191531252713, 88.00268892867056536, 79.05947916753380866 ) ) ;
#56938=DIRECTION ( 'NONE',  ( 1.000000000000000000, 0.000000000000000000, 0.000000000000000000 ) ) ;
#56939=CARTESIAN_POINT ( 'NONE',  ( 94.99999999999998579, 92.66308142843932671, 78.21281250086717307 ) ) ;
#56941=CARTESIAN_POINT ( 'NONE',  ( -93.84685191531247028, -211.9973110713294489, 78.58322916753382970 ) ) ;
#56945=CARTESIAN_POINT ( 'NONE',  ( -93.67499999999998295, -212.2949673200287179, 75.60666666666665492 ) ) ;
#56948=CARTESIAN_POINT ( 'NONE',  ( -92.69370383062504004, 90.00000000000004263, 77.41906250086715602 ) ) ;
#56949=CARTESIAN_POINT ( 'NONE',  ( 92.69370383062501162, -208.6684592857803011, 79.42989583420046529 ) ) ;
#56955=CARTESIAN_POINT ( 'NONE',  ( -97.64999999999996305, -209.9999999999999716, 88.17437500173430465 ) ) ;
#56956=EDGE_LOOP ( 'NONE', ( #67296, #67628, #14101, #32885 ) ) ;
#56959=CARTESIAN_POINT ( 'NONE',  ( 97.64999999999999147, 89.99999989488613039, 86.58687499784845443 ) ) ;
#56964=CARTESIAN_POINT ( 'NONE',  ( 95.00000000000000000, -207.3369185715606307, 75.03781250086714749 ) ) ;
#56968=CARTESIAN_POINT ( 'NONE',  ( 94.99999999999998579, 87.33691857156068750, 82.97531250086716170 ) ) ;
#56969=AXIS2_PLACEMENT_3D ( 'NONE', #36581, #19655, #59529 ) ;
#56970=ADVANCED_FACE ( 'NONE', ( #51921 ), #17342, .F. ) ;
#56971=CARTESIAN_POINT ( 'NONE',  ( 96.32499999999998863, -207.7050326799711968, 78.35833333333333428 ) ) ;
#56972=ORIENTED_EDGE ( 'NONE', *, *, #1312, .F. ) ;
#56973=ORIENTED_EDGE ( 'NONE', *, *, #18562, .F. ) ;
#56984=CARTESIAN_POINT ( 'NONE',  ( 93.67499999999999716, 87.70503267997126784, 83.83520833506763381 ) ) ;
#56986=CARTESIAN_POINT ( 'NONE',  ( -94.99999999999997158, -213.0599564267049857, 83.88812500173429498 ) ) ;
#56987=EDGE_CURVE ( 'NONE', #2356, #67569, #42417, .T. ) ;
#56991=ORIENTED_EDGE ( 'NONE', *, *, #10429, .T. ) ;
#56992=CARTESIAN_POINT ( 'NONE',  ( 96.32499999999997442, 92.29496732002878900, 80.34270833506762699 ) ) ;
#56993=CARTESIAN_POINT ( 'NONE',  ( -92.35000000000005116, 91.52997821335253548, 79.01979166840095559 ) ) ;
#56996=CARTESIAN_POINT ( 'NONE',  ( 93.84685191531248449, 88.00268892867053694, 84.82739583420048746 ) ) ;
#57003=ORIENTED_EDGE ( 'NONE', *, *, #21732, .F. ) ;
#57008=EDGE_LOOP ( 'NONE', ( #17838, #3252, #3506, #42604, #5341 ) ) ;
#57010=DIRECTION ( 'NONE',  ( -0.000000000000000000, -0.000000000000000000, 1.000000000000000000 ) ) ;
#57012=CARTESIAN_POINT ( 'NONE',  ( -97.30629616937495996, -209.9999999999999716, 81.54656250086715374 ) ) ;
#57015=DIRECTION ( 'NONE',  ( -0.000000000000000000, -0.000000000000000000, 1.000000000000000000 ) ) ;
#57017=CARTESIAN_POINT ( 'NONE',  ( -95.12556226663647863, -212.6467947905573510, 74.99648857272255498 ) ) ;
#57020=CARTESIAN_POINT ( 'NONE',  ( 92.35000000000000853, -209.9999999999999716, 83.01499999999998636 ) ) ;
#57028=CARTESIAN_POINT ( 'NONE',  ( 93.84685191531248449, 88.00268892867053694, 86.73239583420048859 ) ) ;
#57029=CARTESIAN_POINT ( 'NONE',  ( -97.30629616937497417, -211.3315407142195852, 89.21947916753381946 ) ) ;
#57034=CARTESIAN_POINT ( 'NONE',  ( -96.15314808468751551, 88.00268892867056536, 78.31864583420048120 ) ) ;
#57037=CARTESIAN_POINT ( 'NONE',  ( 95.00000000000000000, -212.6630814284392557, 89.16656250086712987 ) ) ;
#57049=( BOUNDED_CURVE ( )  B_SPLINE_CURVE ( 2, ( #33039, #48852, #72152, #15011, #67270, #10116, #32667, #25924, #4134, #49589, #73265, #3035, #61630, #60528, #43247, #72517, #37952, #10486, #55980, #44720, #9006, #55612, #27397, #4499, #21378, #31930, #21769, #16134, #54869, #27025, #15379, #66531, #72877, #43611, #44338, #49224, #67638, #38323, #33403, #39071, #71772, #38698, #20279, #3762, #9371, #32292, #66170, #15762, #14643, #60889, #37590, #3389, #26289, #55240, #26660, #66888, #21017, #43970, #17983, #39819, #69133, #33795, #57475, #68762, #45466, #5989, #22523, #28896, #28148, #738, #17250, #40929, #52191, #57849, #11233, #17616, #73632, #57111, #62770, #34167, #63493, #34912, #63137, #39444, #45090, #46559, #68394, #16885, #10, #40545, #62388, #40186, #10871, #56746, #6350, #69485, #11588, #11969, #5614, #28513, #29250, #23628, #4884, #63865, #12337, #56368, #5248, #51450, #34527, #22904, #27784, #16502, #51085, #23266, #46197, #50709, #51828, #22148, #45840, #74009, #68010, #373, #35277, #24367, #19084, #35629, #2213, #7070, #13448, #64587, #54052, #25101, #70950, #2589, #25474, #29992, #53672, #65336, #6706, #41646, #52938, #24004, #41290, #31101, #24732, #19818, #52558, #1478, #70206, #70568, #47302, #18712, #48400, #18344, #42034, #1112, #42768, #8174, #7810, #64971, #30727, #13071, #48035, #42398, #36371, #58204, #59316, #7446, #71313, #29612, #19455, #64229, #46932, #30360, #36009, #58957, #13804, #58570, #36748, #53306, #65702, #69847, #1843, #47660, #59690, #12701, #15295, #55530, #31840, #21292, #26199, #4046, #60079, #9284, #66086, #25836, #43531, #10027, #49141, #38611, #26941, #49510, #49869, #72067, #20578, #72790, #26576, #8557, #61548, #55897, #37134, #32947, #14928, #32583, #43888, #44249, #43154, #48768, #31475, #66809, #4411, #9661, #67178, #66444, #14556, #15678, #32204, #55150, #54784, #27306, #50241, #73177, #21678, #3679, #38231, #44632, #37872, #54413, #60804, #72432, #20935, #14181, #2946, #71688, #61176, #60439, #20189, #37506, #8922, #3308, #62678, #68299, #51739, #17523, #40455, #34822, #44999, #67550, #5895, #57758, #11871, #645, #63400, #40093, #74299, #63048, #67925, #28428, #38983, #16795, #16041, #29162, #52103, #28056, #34074, #6263, #62291, #68674, #284, #22432, #28807, #46105, #23536 ),
 .UNSPECIFIED., .F., .F. ) 
 B_SPLINE_CURVE_WITH_KNOTS ( ( 3, 2, 2, 2, 2, 2, 2, 2, 2, 2, 2, 2, 2, 2, 2, 2, 2, 2, 2, 2, 2, 2, 2, 2, 2, 2, 2, 2, 2, 2, 2, 2, 2, 2, 2, 2, 2, 2, 2, 2, 2, 2, 2, 2, 2, 2, 2, 2, 2, 2, 2, 2, 2, 2, 2, 2, 2, 2, 2, 2, 2, 2, 2, 2, 2, 2, 2, 2, 2, 2, 2, 2, 2, 2, 2, 2, 2, 2, 2, 2, 2, 2, 2, 2, 2, 2, 2, 2, 2, 2, 2, 2, 2, 2, 2, 2, 2, 2, 2, 2, 2, 2, 2, 2, 2, 2, 2, 2, 2, 2, 2, 2, 2, 2, 2, 2, 2, 2, 2, 2, 2, 2, 2, 2, 2, 2, 2, 2, 2, 2, 2, 2, 2, 2, 2, 2, 2, 2, 2, 2, 2, 3 ),
 ( 0.000000000000000000, 0.007055765384978172905, 0.01411153076995634581, 0.02116729615493451871, 0.02822306153991269162, 0.03527882692489087146, 0.04233459230986903743, 0.04939035769484721727, 0.05644612307982538324, 0.06350188846480356308, 0.07055765384978174293, 0.07761341923475992277, 0.08466918461973807486, 0.09172495000471625470, 0.09878071538969443455, 0.1058364807746726005, 0.1128922461596507665, 0.1199480115446289463, 0.1270037769296071262, 0.1340595423145853060, 0.1411153076995634859, 0.1481710730845416657, 0.1552268384695198455, 0.1622826038544979699, 0.1693383692394761497, 0.1763941346244543296, 0.1834499000094325094, 0.1905056653944106893, 0.1975614307793888691, 0.2046171961643670212, 0.2116729615493452010, 0.2187287269343233809, 0.2257844923193015330, 0.2328402577042797128, 0.2398960230892578926, 0.2469517884742360447, 0.2540075538592142523, 0.2610633192441924044, 0.2681190846291706120, 0.2751748500141487086, 0.2822306153991269717, 0.2892863807841050683, 0.2963421461690833314, 0.3033979115540614280, 0.3104536769390396911, 0.3175094423240177877, 0.3245652077089959398, 0.3316209730939741473, 0.3386767384789522994, 0.3457325038639305070, 0.3527882692489086591, 0.3598440346338868112, 0.3668998000188650188, 0.3739555654038431709, 0.3810113307888213785, 0.3880670961737994751, 0.3951228615587777382, 0.4021786269437558348, 0.4092343923287340424, 0.4162901577137121945, 0.4233459230986904021, 0.4304016884836685541, 0.4374574538686467617, 0.4445132192536248583, 0.4515689846386030659, 0.4586247500235812180, 0.4656805154085594256, 0.4727362807935375777, 0.4797920461785157853, 0.4868478115634939374, 0.4939035769484720895, 0.5009593423334502971, 0.5080151077184285047, 0.5150708731034066012, 0.5221266384883848088, 0.5291824038733630164, 0.5362381692583412240, 0.5432939346433193206, 0.5503497000282974172, 0.5574054654132757358, 0.5644612307982539434, 0.5715169961832320400, 0.5785727615682101366, 0.5856285269531882332, 0.5926842923381666628, 0.5997400577231447594, 0.6067958231081228559, 0.6138515884931009525, 0.6209073538780793822, 0.6279631192630574787, 0.6350188846480355753, 0.6420746500330136719, 0.6491304154179918795, 0.6561861808029701981, 0.6632419461879482947, 0.6702977115729263913, 0.6773534769579045989, 0.6844092423428828065, 0.6914650077278610141, 0.6985207731128391107, 0.7055765384978173183, 0.7126323038827954148, 0.7196880692677736224, 0.7267438346527518300, 0.7337996000377300376, 0.7408553654227081342, 0.7479111308076863418, 0.7549668961926644384, 0.7620226615776427570, 0.7690784269626208536, 0.7761341923475989502, 0.7831899577325772688, 0.7902457231175554764, 0.7973014885025335730, 0.8043572538875116695, 0.8114130192724899882, 0.8184687846574680847, 0.8255245500424462923, 0.8325803154274243889, 0.8396360808124025965, 0.8466918461973808041, 0.8537476115823589007, 0.8608033769673371083, 0.8678591423523153159, 0.8749149077372935235, 0.8819706731222716201, 0.8890264385072497166, 0.8960822038922280353, 0.9031379692772061318, 0.9101937346621843394, 0.9172495000471624360, 0.9243052654321407546, 0.9313610308171188512, 0.9384167962020970588, 0.9454725615870751554, 0.9525283269720533630, 0.9595840923570315706, 0.9666398577420096672, 0.9736956231269878748, 0.9807513885119660824, 0.9878071538969441789, 0.9900635123082152100 ),
 .UNSPECIFIED. ) 
 CURVE ( )  GEOMETRIC_REPRESENTATION_ITEM ( )  RATIONAL_B_SPLINE_CURVE ( ( 1.000000000000000000, 0.8660254037844387076, 1.000000000000000000, 0.8660254037844387076, 1.000000000000000000, 0.8660254037844387076, 1.000000000000000000, 0.8660254037844387076, 1.000000000000000000, 0.8660254037844387076, 1.000000000000000000, 0.8660254037844387076, 1.000000000000000000, 0.8660254037844387076, 1.000000000000000000, 0.8660254037844387076, 1.000000000000000000, 0.8660254037844387076, 1.000000000000000000, 0.8660254037844387076, 1.000000000000000000, 0.8660254037844387076, 1.000000000000000000, 0.8660254037844387076, 1.000000000000000000, 0.8660254037844387076, 1.000000000000000000, 0.8660254037844387076, 1.000000000000000000, 0.8660254037844387076, 1.000000000000000000, 0.8660254037844387076, 1.000000000000000000, 0.8660254037844387076, 1.000000000000000000, 0.8660254037844387076, 1.000000000000000000, 0.8660254037844387076, 1.000000000000000000, 0.8660254037844387076, 1.000000000000000000, 0.8660254037844387076, 1.000000000000000000, 0.8660254037844387076, 1.000000000000000000, 0.8660254037844387076, 1.000000000000000000, 0.8660254037844387076, 1.000000000000000000, 0.8660254037844387076, 1.000000000000000000, 0.8660254037844387076, 1.000000000000000000, 0.8660254037844387076, 1.000000000000000000, 0.8660254037844387076, 1.000000000000000000, 0.8660254037844387076, 1.000000000000000000, 0.8660254037844387076, 1.000000000000000000, 0.8660254037844387076, 1.000000000000000000, 0.8660254037844387076, 1.000000000000000000, 0.8660254037844387076, 1.000000000000000000, 0.8660254037844387076, 1.000000000000000000, 0.8660254037844387076, 1.000000000000000000, 0.8660254037844387076, 1.000000000000000000, 0.8660254037844387076, 1.000000000000000000, 0.8660254037844387076, 1.000000000000000000, 0.8660254037844387076, 1.000000000000000000, 0.8660254037844387076, 1.000000000000000000, 0.8660254037844387076, 1.000000000000000000, 0.8660254037844387076, 1.000000000000000000, 0.8660254037844387076, 1.000000000000000000, 0.8660254037844387076, 1.000000000000000000, 0.8660254037844387076, 1.000000000000000000, 0.8660254037844387076, 1.000000000000000000, 0.8660254037844387076, 1.000000000000000000, 0.8660254037844387076, 1.000000000000000000, 0.8660254037844387076, 1.000000000000000000, 0.8660254037844387076, 1.000000000000000000, 0.8660254037844387076, 1.000000000000000000, 0.8660254037844387076, 1.000000000000000000, 0.8660254037844387076, 1.000000000000000000, 0.8660254037844387076, 1.000000000000000000, 0.8660254037844387076, 1.000000000000000000, 0.8660254037844387076, 1.000000000000000000, 0.8660254037844387076, 1.000000000000000000, 0.8660254037844387076, 1.000000000000000000, 0.8660254037844387076, 1.000000000000000000, 0.8660254037844387076, 1.000000000000000000, 0.8660254037844387076, 1.000000000000000000, 0.8660254037844387076, 1.000000000000000000, 0.8660254037844387076, 1.000000000000000000, 0.8660254037844387076, 1.000000000000000000, 0.8660254037844387076, 1.000000000000000000, 0.8660254037844387076, 1.000000000000000000, 0.8660254037844387076, 1.000000000000000000, 0.8660254037844387076, 1.000000000000000000, 0.8660254037844387076, 1.000000000000000000, 0.8660254037844387076, 1.000000000000000000, 0.8660254037844387076, 1.000000000000000000, 0.8660254037844387076, 1.000000000000000000, 0.8660254037844387076, 1.000000000000000000, 0.8660254037844387076, 1.000000000000000000, 0.8660254037844387076, 1.000000000000000000, 0.8660254037844387076, 1.000000000000000000, 0.8660254037844387076, 1.000000000000000000, 0.8660254037844387076, 1.000000000000000000, 0.8660254037844387076, 1.000000000000000000, 0.8660254037844387076, 1.000000000000000000, 0.8660254037844387076, 1.000000000000000000, 0.8660254037844387076, 1.000000000000000000, 0.8660254037844387076, 1.000000000000000000, 0.8660254037844387076, 1.000000000000000000, 0.8660254037844387076, 1.000000000000000000, 0.8660254037844387076, 1.000000000000000000, 0.8660254037844387076, 1.000000000000000000, 0.8660254037844387076, 1.000000000000000000, 0.8660254037844387076, 1.000000000000000000, 0.8660254037844387076, 1.000000000000000000, 0.8660254037844387076, 1.000000000000000000, 0.8660254037844387076, 1.000000000000000000, 0.8660254037844387076, 1.000000000000000000, 0.8660254037844387076, 1.000000000000000000, 0.8660254037844387076, 1.000000000000000000, 0.8660254037844387076, 1.000000000000000000, 0.8660254037844387076, 1.000000000000000000, 0.8660254037844387076, 1.000000000000000000, 0.8660254037844387076, 1.000000000000000000, 0.8660254037844387076, 1.000000000000000000, 0.8660254037844387076, 1.000000000000000000, 0.8660254037844387076, 1.000000000000000000, 0.8660254037844387076, 1.000000000000000000, 0.8660254037844387076, 1.000000000000000000, 0.8660254037844387076, 1.000000000000000000, 0.8660254037844387076, 1.000000000000000000, 0.8660254037844387076, 1.000000000000000000, 0.8660254037844387076, 1.000000000000000000, 0.8660254037844387076, 1.000000000000000000, 0.8660254037844387076, 1.000000000000000000, 0.8660254037844387076, 1.000000000000000000, 0.8660254037844387076, 1.000000000000000000, 0.8660254037844387076, 1.000000000000000000, 0.8660254037844387076, 1.000000000000000000, 0.8660254037844387076, 1.000000000000000000, 0.8660254037844387076, 1.000000000000000000, 0.8660254037844387076, 1.000000000000000000, 0.8660254037844387076, 1.000000000000000000, 0.8660254037844387076, 1.000000000000000000, 0.8660254037844387076, 1.000000000000000000, 0.8660254037844387076, 1.000000000000000000, 0.8660254037844387076, 1.000000000000000000, 0.8660254037844387076, 1.000000000000000000, 0.8660254037844387076, 1.000000000000000000, 0.8660254037844387076, 1.000000000000000000, 0.8660254037844387076, 1.000000000000000000, 0.8660254037844387076, 1.000000000000000000, 0.8660254037844387076, 1.000000000000000000, 0.8660254037844387076, 1.000000000000000000, 0.8660254037844387076, 1.000000000000000000, 0.8660254037844387076, 1.000000000000000000, 0.8660254037844387076, 1.000000000000000000, 0.8660254037844387076, 1.000000000000000000, 0.8660254037844387076, 1.000000000000000000, 0.8660254037844387076, 1.000000000000000000, 0.8660254037844387076, 1.000000000000000000, 0.8660254037844387076, 1.000000000000000000, 0.8660254037844387076, 1.000000000000000000, 0.8660254037844387076, 1.000000000000000000, 0.8660254037844387076, 1.000000000000000000, 0.9571563550410552290, 0.9417145902178747363 ) ) 
 REPRESENTATION_ITEM ( '' )  );
#57051=CARTESIAN_POINT ( 'NONE',  ( 96.15314808468750130, -211.9973110713294489, 86.20322916753382003 ) ) ;
#57053=ADVANCED_FACE ( 'NONE', ( #59796 ), #24829, .T. ) ;
#57055=DIRECTION ( 'NONE',  ( 3.061616997868383141E-16, 1.000000000000000000, -0.000000000000000000 ) ) ;
#57056=CARTESIAN_POINT ( 'NONE',  ( 96.32499999999998863, -212.2949673200287179, 76.87666666666666515 ) ) ;
#57059=CARTESIAN_POINT ( 'NONE',  ( 92.35000000000002274, -208.4700217866474645, 88.67708333333332860 ) ) ;
#57061=ORIENTED_EDGE ( 'NONE', *, *, #30308, .T. ) ;
#57063=EDGE_LOOP ( 'NONE', ( #9047, #8986, #54650, #58931 ) ) ;
#57070=CARTESIAN_POINT ( 'NONE',  ( 93.67500000000001137, -212.2949673200287179, 77.48520833506763950 ) ) ;
#57071=CARTESIAN_POINT ( 'NONE',  ( 93.67499999999999716, 87.70503267997126784, 80.58083333333331666 ) ) ;
#57080=CARTESIAN_POINT ( 'NONE',  ( -97.30629616937501680, 88.66845928578038638, 80.96447916753382401 ) ) ;
#57081=CARTESIAN_POINT ( 'NONE',  ( 94.99999999999998579, 92.66308142843935514, 76.78406250086712248 ) ) ;
#57086=CARTESIAN_POINT ( 'NONE',  ( 92.35000000045006630, 89.99996890530464100, 88.81037122970248276 ) ) ;
#57087=CARTESIAN_POINT ( 'NONE',  ( -93.67499999999998295, -207.7050326799711968, 77.72333333333332916 ) ) ;
#57091=CARTESIAN_POINT ( 'NONE',  ( -94.99999999999997158, -212.6630814284392557, 76.46656250086712703 ) ) ;
#57097=CARTESIAN_POINT ( 'NONE',  ( 97.65000000000009095, 88.47002178664759242, 78.19958333333332234 ) ) ;
#57101=CARTESIAN_POINT ( 'NONE',  ( -94.99999999999997158, -207.3369185715606307, 75.51406250086714067 ) ) ;
#57103=CARTESIAN_POINT ( 'NONE',  ( -93.67499999999998295, -207.7050326799711968, 81.53333333333333144 ) ) ;
#57105=LINE ( 'NONE', #35902, #21308 ) ;
#57111=CARTESIAN_POINT ( 'NONE',  ( 97.30629616937498838, 91.33154071421968467, 85.56822916753380071 ) ) ;
#57117=CARTESIAN_POINT ( 'NONE',  ( -97.65000000000001990, 89.99997747860815878, 84.36437578067155130 ) ) ;
#57125=CARTESIAN_POINT ( 'NONE',  ( -94.99999999999997158, -206.9400435732949575, 86.03125000000000000 ) ) ;
#57126=EDGE_CURVE ( 'NONE', #8233, #69330, #41538, .T. ) ;
#57136=CARTESIAN_POINT ( 'NONE',  ( 95.00000000000000000, -207.3369185715606307, 87.10281250086715943 ) ) ;
#57146=( BOUNDED_CURVE ( )  B_SPLINE_CURVE ( 2, ( #19003, #65629, #25401, #48328, #24296, #71237, #14100 ),
 .UNSPECIFIED., .F., .F. ) 
 B_SPLINE_CURVE_WITH_KNOTS ( ( 3, 2, 2, 3 ),
 ( 0.3598440426530883918, 0.3668998081258832422, 0.3739555736667655728, 0.3810111478265176821 ),
 .UNSPECIFIED. ) 
 CURVE ( )  GEOMETRIC_REPRESENTATION_ITEM ( )  RATIONAL_B_SPLINE_CURVE ( ( 1.000000000000000000, 0.8660254037844387076, 1.000000000000000000, 0.8660254037844387076, 1.000000000000000000, 0.8660290377217475521, 0.9999927323225166198 ) ) 
 REPRESENTATION_ITEM ( '' )  );
#57147=CARTESIAN_POINT ( 'NONE',  ( 97.30629616937498838, -208.6684592857803295, 79.85322916753379729 ) ) ;
#57150=CARTESIAN_POINT ( 'NONE',  ( 95.00000000000000000, -207.3369185715606307, 82.02281250086714692 ) ) ;
#57152=CARTESIAN_POINT ( 'NONE',  ( 92.35001798596591982, 91.52998859755481931, 80.50145761676020584 ) ) ;
#57155=EDGE_CURVE ( 'NONE', #63633, #8129, #13544, .T. ) ;
#57157=CIRCLE ( 'NONE', #24730, 3.299999999999969624 ) ;
#57161=CARTESIAN_POINT ( 'NONE',  ( 97.64999999999999147, -209.9999999999999716, 87.85687500173429498 ) ) ;
#57162=ORIENTED_EDGE ( 'NONE', *, *, #29262, .T. ) ;
#57164=EDGE_CURVE ( 'NONE', #32709, #57704, #20296, .T. ) ;
#57165=ORIENTED_EDGE ( 'NONE', *, *, #57673, .F. ) ;
#57167=VERTEX_POINT ( 'NONE', #67654 ) ;
#57168=ADVANCED_FACE ( 'NONE', ( #55993 ), #56384, .F. ) ;
#57175=ORIENTED_EDGE ( 'NONE', *, *, #13388, .F. ) ;
#57178=CARTESIAN_POINT ( 'NONE',  ( -96.32500000000001705, 92.29496732002878900, 87.98916666666666231 ) ) ;
#57180=CARTESIAN_POINT ( 'NONE',  ( 96.15314808468748708, 91.99731107132950569, 75.46114583420047950 ) ) ;
#57183=CARTESIAN_POINT ( 'NONE',  ( -92.69370383062498320, -208.6684592857803011, 87.47322916753381605 ) ) ;
#57186=CARTESIAN_POINT ( 'NONE',  ( 92.98340954502104694, -211.6055158133078749, 74.95309847082319266 ) ) ;
#57188=CARTESIAN_POINT ( 'NONE',  ( -96.15314808468747287, -208.0026889286704943, 76.83697916753381207 ) ) ;
#57192=CARTESIAN_POINT ( 'NONE',  ( -96.32500000000001705, 87.70503267997129626, 85.10520833506762983 ) ) ;
#57196=CARTESIAN_POINT ( 'NONE',  ( -97.30629616937501680, 88.66845928578038638, 77.63072916753380071 ) ) ;
#57204=CARTESIAN_POINT ( 'NONE',  ( 92.35000000000000853, -208.4700217866474645, 89.39145833506763950 ) ) ;
#57210=DIRECTION ( 'NONE',  ( -0.000000000000000000, -0.000000000000000000, 1.000000000000000000 ) ) ;
#57211=CARTESIAN_POINT ( 'NONE',  ( -92.69370383062498320, -208.6684592857803011, 78.74197916753382742 ) ) ;
#57215=ORIENTED_EDGE ( 'NONE', *, *, #40658, .T. ) ;
#57226=CARTESIAN_POINT ( 'NONE',  ( 92.69370383062501162, -209.9999999999999716, 88.37281250086715545 ) ) ;
#57230=FACE_OUTER_BOUND ( 'NONE', #57063, .T. ) ;
#57232=ORIENTED_EDGE ( 'NONE', *, *, #71609, .T. ) ;
#57246=CIRCLE ( 'NONE', #48797, 23.50000000000000355 ) ;
#57247=ORIENTED_EDGE ( 'NONE', *, *, #58164, .T. ) ;
#57250=VERTEX_POINT ( 'NONE', #14654 ) ;
#57252=CARTESIAN_POINT ( 'NONE',  ( 94.99999999999998579, 87.33691857156068750, 85.99156250086714692 ) ) ;
#57254=CARTESIAN_POINT ( 'NONE',  ( 97.30629616937498838, -208.6684592857803011, 81.12322916753382174 ) ) ;
#57263=CARTESIAN_POINT ( 'NONE',  ( -96.15314808468745866, -211.9973110713294489, 87.20864583420046756 ) ) ;
#57264=CARTESIAN_POINT ( 'NONE',  ( -93.84685191531252713, 88.00268892867056536, 87.47322916753381605 ) ) ;
#57266=CARTESIAN_POINT ( 'NONE',  ( 97.30629616937498838, 88.66845928578037217, 86.09739583420048348 ) ) ;
#57267=CARTESIAN_POINT ( 'NONE',  ( -92.69370383062502583, 88.66845928578038638, 83.55739583420047722 ) ) ;
#57270=DIRECTION ( 'NONE',  ( 0.000000000000000000, 1.000000000000000000, 0.000000000000000000 ) ) ;
#57273=CARTESIAN_POINT ( 'NONE',  ( -93.84685191531247028, -211.9973110713294489, 87.31447916753380412 ) ) ;
#57274=CARTESIAN_POINT ( 'NONE',  ( -96.32499999999996021, -212.2949673200287179, 81.85083333333332689 ) ) ;
#57278=EDGE_LOOP ( 'NONE', ( #60874, #71751, #48338, #56304 ) ) ;
#57280=CARTESIAN_POINT ( 'NONE',  ( -93.67500000000003979, 92.29496732002878900, 76.45333333333333314 ) ) ;
#57282=CARTESIAN_POINT ( 'NONE',  ( -93.26027265873587169, -208.4859488783624215, 74.79348190356851944 ) ) ;
#57288=CARTESIAN_POINT ( 'NONE',  ( -92.69370383062502583, 91.33154071421968467, 77.31322916753380525 ) ) ;
#57289=ADVANCED_FACE ( 'NONE', ( #60899 ), #55627, .F. ) ;
#57290=CARTESIAN_POINT ( 'NONE',  ( 92.35000000046409241, 89.99996903277681781, 77.38038495127642591 ) ) ;
#57298=CARTESIAN_POINT ( 'NONE',  ( -97.30629616937497417, -211.3315407142195852, 89.21947916753381946 ) ) ;
#57299=VECTOR ( 'NONE', #56235, 1000.000000000000000 ) ;
#57303=CARTESIAN_POINT ( 'NONE',  ( 93.84685191531248449, 88.00268892867053694, 77.84239583420048803 ) ) ;
#57304=CARTESIAN_POINT ( 'NONE',  ( -97.30629616937497417, -208.6684592857803295, 78.31864583420050963 ) ) ;
#57308=CARTESIAN_POINT ( 'NONE',  ( -97.64999999999994884, -208.4700217866474645, 75.97708333333333997 ) ) ;
#57311=CARTESIAN_POINT ( 'NONE',  ( 95.00000000000000000, -212.6630814284392557, 81.54656250086715374 ) ) ;
#57319=ORIENTED_EDGE ( 'NONE', *, *, #59234, .T. ) ;
#57329=CARTESIAN_POINT ( 'NONE',  ( 92.69370383062498320, 88.66845928578037217, 84.77447916753381207 ) ) ;
#57331=CARTESIAN_POINT ( 'NONE',  ( 93.67500000000001137, -207.7050326799711968, 77.82916666666665151 ) ) ;
#57333=ORIENTED_EDGE ( 'NONE', *, *, #73727, .T. ) ;
#57338=LINE ( 'NONE', #64464, #15094 ) ;
#57343=CARTESIAN_POINT ( 'NONE',  ( 92.35000000000002274, -209.9999907117589260, 86.90437468048608594 ) ) ;
#57347=CARTESIAN_POINT ( 'NONE',  ( -97.64999999999996305, -209.9999999999999716, 82.45937500173430124 ) ) ;
#57350=VERTEX_POINT ( 'NONE', #6360 ) ;
#57351=CARTESIAN_POINT ( 'NONE',  ( 92.34999999999999432, 88.47002178664753558, 80.60729166840097548 ) ) ;
#57352=CARTESIAN_POINT ( 'NONE',  ( -93.67500000000003979, 87.70503267997129626, 78.22604166840096696 ) ) ;
#57353=( BOUNDED_CURVE ( )  B_SPLINE_CURVE ( 2, ( #66694, #9550, #72676, #67804, #67431, #44129, #21178 ),
 .UNSPECIFIED., .F., .F. ) 
 B_SPLINE_CURVE_WITH_KNOTS ( ( 3, 2, 2, 3 ),
 ( 0.3175094496506952191, 0.3245652148805888704, 0.3316209804214712564, 0.3386766260338262002 ),
 .UNSPECIFIED. ) 
 CURVE ( )  GEOMETRIC_REPRESENTATION_ITEM ( )  RATIONAL_B_SPLINE_CURVE ( ( 1.000000000000000000, 0.8660254037844387076, 1.000000000000000000, 0.8660254037844387076, 1.000000000000000000, 0.8660276809825602218, 0.9999954456811690484 ) ) 
 REPRESENTATION_ITEM ( '' )  );
#57355=CARTESIAN_POINT ( 'NONE',  ( 97.30629616937498838, 91.33154071421968467, 78.74197916753382742 ) ) ;
#57356=CARTESIAN_POINT ( 'NONE',  ( -96.32499999999996021, -207.7050326799711968, 82.27416666666665890 ) ) ;
#57362=CARTESIAN_POINT ( 'NONE',  ( 97.64999999999999147, 90.00000000000002842, 90.00000000000000000 ) ) ;
#57368=EDGE_CURVE ( 'NONE', #9077, #44189, #29265, .T. ) ;
#57375=CARTESIAN_POINT ( 'NONE',  ( -94.99999999999997158, -212.6630814284392557, 81.07031250086716057 ) ) ;
#57378=EDGE_CURVE ( 'NONE', #55000, #47150, #13640, .T. ) ;
#57387=DIRECTION ( 'NONE',  ( -0.000000000000000000, -0.000000000000000000, 1.000000000000000000 ) ) ;
#57391=CARTESIAN_POINT ( 'NONE',  ( 97.30629616937498838, 91.33154071421968467, 88.90197916753382401 ) ) ;
#57393=CARTESIAN_POINT ( 'NONE',  ( -2.499999999999970690, 73.00000000000001421, -258.2999999999999545 ) ) ;
#57396=CARTESIAN_POINT ( 'NONE',  ( -97.30629616937501680, 88.66845928578038638, 78.90072916753381094 ) ) ;
#57398=AXIS2_PLACEMENT_3D ( 'NONE', #71881, #42968, #31297 ) ;
#57403=LINE ( 'NONE', #307, #39050 ) ;
#57408=DIRECTION ( 'NONE',  ( -0.000000000000000000, -0.000000000000000000, 1.000000000000000000 ) ) ;
#57415=CARTESIAN_POINT ( 'NONE',  ( 92.69370383062501162, -209.9999999999999716, 85.99156250086716113 ) ) ;
#57419=CARTESIAN_POINT ( 'NONE',  ( 94.99999999999998579, 93.05995642670504253, 82.85625000000000284 ) ) ;
#57422=CARTESIAN_POINT ( 'NONE',  ( 96.32499999999998863, -207.7050326799711968, 88.51833333333333087 ) ) ;
#57424=ORIENTED_EDGE ( 'NONE', *, *, #67399, .T. ) ;
#57429=CARTESIAN_POINT ( 'NONE',  ( -96.15314808468752972, 91.99731107132950569, 88.42572916753381662 ) ) ;
#57432=CARTESIAN_POINT ( 'NONE',  ( 92.35000000000002274, -208.4700217866474645, 76.05645833506761733 ) ) ;
#57433=CARTESIAN_POINT ( 'NONE',  ( 92.34999999999999432, 88.47002178664753558, 79.89291666666666458 ) ) ;
#57436=ADVANCED_FACE ( 'NONE', ( #67098 ), #72365, .F. ) ;
#57437=VERTEX_POINT ( 'NONE', #14104 ) ;
#57438=CARTESIAN_POINT ( 'NONE',  ( -97.64999999999996305, -210.0000348885099015, 83.09437620840745353 ) ) ;
#57440=CARTESIAN_POINT ( 'NONE',  ( -95.00000000000002842, 93.05995642670501411, 89.28562500173430294 ) ) ;
#57441=CARTESIAN_POINT ( 'NONE',  ( -92.69370383062505425, 91.33154071421968467, 82.55197916753380127 ) ) ;
#57443=CARTESIAN_POINT ( 'NONE',  ( 93.84685191531248449, 91.99731107132950569, 76.20197916753380696 ) ) ;
#57445=CARTESIAN_POINT ( 'NONE',  ( 95.00000000000000000, -209.9999999999999716, 90.00000000000000000 ) ) ;
#57448=DIRECTION ( 'NONE',  ( 1.000000000000000000, 0.000000000000000000, 0.000000000000000000 ) ) ;
#57453=CARTESIAN_POINT ( 'NONE',  ( -93.84685191531247028, -211.9973110713294489, 79.05947916753380866 ) ) ;
#57455=ORIENTED_EDGE ( 'NONE', *, *, #791, .T. ) ;
#57459=EDGE_CURVE ( 'NONE', #9432, #52406, #65633, .T. ) ;
#57464=CARTESIAN_POINT ( 'NONE',  ( -93.84685191531248449, -208.0026889286704943, 76.09614583420047040 ) ) ;
#57475=CARTESIAN_POINT ( 'NONE',  ( 93.84685191531248449, 91.99731107132950569, 86.36197916753381776 ) ) ;
#57476=CARTESIAN_POINT ( 'NONE',  ( -94.99999999999997158, -213.0599564267049857, 83.80875000000000341 ) ) ;
#57477=CARTESIAN_POINT ( 'NONE',  ( -92.35000000000013642, 88.47002178664750716, 88.35958333333334735 ) ) ;
#57488=CARTESIAN_POINT ( 'NONE',  ( -97.30629616937501680, 90.00000000000004263, 88.37281250086715545 ) ) ;
#57493=EDGE_CURVE ( 'NONE', #51207, #6061, #21313, .T. ) ;
#57504=CARTESIAN_POINT ( 'NONE',  ( 92.69370383062501162, -208.6684592857803011, 86.57364583420047666 ) ) ;
#57508=ORIENTED_EDGE ( 'NONE', *, *, #21136, .F. ) ;
#57514=CARTESIAN_POINT ( 'NONE',  ( 92.69370383062501162, -208.6684592857803011, 82.76364583420048859 ) ) ;
#57516=EDGE_LOOP ( 'NONE', ( #48550, #41585 ) ) ;
#57520=DIRECTION ( 'NONE',  ( -0.000000000000000000, -0.000000000000000000, 1.000000000000000000 ) ) ;
#57527=CARTESIAN_POINT ( 'NONE',  ( 95.00000000000000000, -206.9400435732949575, 86.74562500173429669 ) ) ;
#57529=ORIENTED_EDGE ( 'NONE', *, *, #27135, .T. ) ;
#57534=CARTESIAN_POINT ( 'NONE',  ( 97.64999999999689351, 89.99999595380309358, 77.06187486178042434 ) ) ;
#57545=CARTESIAN_POINT ( 'NONE',  ( 97.65000000000000568, 91.52997821335252127, 79.65479166840096070 ) ) ;
#57546=ADVANCED_FACE ( 'NONE', ( #22353 ), #10699, .F. ) ;
#57549=CARTESIAN_POINT ( 'NONE',  ( -97.65000000000001990, 88.47002178664754979, 88.14791666666666003 ) ) ;
#57552=ORIENTED_EDGE ( 'NONE', *, *, #27041, .F. ) ;
#57553=CARTESIAN_POINT ( 'NONE',  ( 92.34999999999999432, 90.00000000000002842, 90.00000000000000000 ) ) ;
#57554=CARTESIAN_POINT ( 'NONE',  ( -92.69370383062498320, -208.6684592857803011, 85.56822916753380071 ) ) ;
#57555=ORIENTED_EDGE ( 'NONE', *, *, #46120, .F. ) ;
#57560=CARTESIAN_POINT ( 'NONE',  ( -92.69370383062498320, -208.6684592857803295, 76.67822916753378593 ) ) ;
#57565=CARTESIAN_POINT ( 'NONE',  ( 94.99999999999998579, 90.00000000000002842, 90.00000000000000000 ) ) ;
#57567=CIRCLE ( 'NONE', #28728, 2.649999999999985700 ) ;
#57569=CARTESIAN_POINT ( 'NONE',  ( -93.67500000000003979, 92.29496732002878900, 76.45333333333333314 ) ) ;
#57570=CARTESIAN_POINT ( 'NONE',  ( 92.35000000021533140, 90.00002100773845370, 79.91868729553033290 ) ) ;
#57571=CARTESIAN_POINT ( 'NONE',  ( -93.84685191531252713, 88.00268892867056536, 78.42447916753381776 ) ) ;
#57577=CARTESIAN_POINT ( 'NONE',  ( 92.34999999999999432, 90.00001433786182758, 79.28437450583713542 ) ) ;
#57581=AXIS2_PLACEMENT_3D ( 'NONE', #12212, #35878, #28764 ) ;
#57586=CARTESIAN_POINT ( 'NONE',  ( -92.35000000045957336, 90.00004935162611730, 87.22187670868784437 ) ) ;
#57587=CARTESIAN_POINT ( 'NONE',  ( -92.69370383062498320, -209.9999999999999716, 77.41906250086715602 ) ) ;
#57592=( BOUNDED_CURVE ( )  B_SPLINE_CURVE ( 2, ( #1875, #52971, #34942, #1143, #23657, #7104, #30394 ),
 .UNSPECIFIED., .F., .F. ) 
 B_SPLINE_CURVE_WITH_KNOTS ( ( 3, 2, 2, 3 ),
 ( 0.08333333333333288462, 0.09027777777777759582, 0.09722222222222230703, 0.1041666666666670182 ),
 .UNSPECIFIED. ) 
 CURVE ( )  GEOMETRIC_REPRESENTATION_ITEM ( )  RATIONAL_B_SPLINE_CURVE ( ( 1.000000000000008660, 0.8660254037844301589, 1.000000000000000000, 0.8660254037844387076, 1.000000000000000000, 0.8660254037844320463, 1.000000000000006661 ) ) 
 REPRESENTATION_ITEM ( '' )  );
#57605=CARTESIAN_POINT ( 'NONE',  ( 92.69370383062501162, -208.6684592857803295, 88.95489583420048518 ) ) ;
#57618=VECTOR ( 'NONE', #27958, 1000.000000000000000 ) ;
#57620=DIRECTION ( 'NONE',  ( -1.000000000000000000, 0.000000000000000000, 0.000000000000000000 ) ) ;
#57623=CARTESIAN_POINT ( 'NONE',  ( 92.59666252161191835, 89.15460556225134781, 74.93511027845775629 ) ) ;
#57627=CARTESIAN_POINT ( 'NONE',  ( 92.69370383062498320, 91.33154071421968467, 85.14489583420048291 ) ) ;
#57630=CARTESIAN_POINT ( 'NONE',  ( 95.00000000000000000, -212.6630814284392557, 80.27656250086714351 ) ) ;
#57636=CARTESIAN_POINT ( 'NONE',  ( -94.95306897617061281, -212.6495843973424655, 75.00000002508416230 ) ) ;
#57638=CARTESIAN_POINT ( 'NONE',  ( 94.99999999999998579, 90.00000000000002842, 90.00000000000000000 ) ) ;
#57642=CONICAL_SURFACE ( 'NONE', #35994, 2.649999999999999467, 1.029744258676654312 ) ;
#57643=CARTESIAN_POINT ( 'NONE',  ( -92.69370383062498320, -211.3315407142195852, 84.82739583420045903 ) ) ;
#57644=CARTESIAN_POINT ( 'NONE',  ( -96.15314808468752972, 91.99731107132950569, 81.44072916753381719 ) ) ;
#57646=CARTESIAN_POINT ( 'NONE',  ( 94.99999999999998579, 87.33691857156068750, 83.45156250086714067 ) ) ;
#57647=CARTESIAN_POINT ( 'NONE',  ( -93.84685191531254134, 91.99731107132950569, 84.98614583420047097 ) ) ;
#57648=ORIENTED_EDGE ( 'NONE', *, *, #25956, .F. ) ;
#57650=CARTESIAN_POINT ( 'NONE',  ( 92.35000000000002274, -209.9999872707216468, 76.10937456147249236 ) ) ;
#57652=CARTESIAN_POINT ( 'NONE',  ( -97.30629616937497417, -211.3315407142195852, 85.88572916753381037 ) ) ;
#57654=DIRECTION ( 'NONE',  ( 1.000000000000000000, 0.000000000000000000, 0.000000000000000000 ) ) ;
#57655=FACE_OUTER_BOUND ( 'NONE', #58279, .T. ) ;
#57656=CYLINDRICAL_SURFACE ( 'NONE', #37238, 2.649999999999999467 ) ;
#57659=CARTESIAN_POINT ( 'NONE',  ( -93.67500000000003979, 87.70503267997129626, 78.14666666666667538 ) ) ;
#57660=CARTESIAN_POINT ( 'NONE',  ( 96.32499999999998863, -212.2949673200287179, 88.94166666666666288 ) ) ;
#57661=DIRECTION ( 'NONE',  ( 1.000000000000000000, 0.000000000000000000, 0.000000000000000000 ) ) ;
#57663=CARTESIAN_POINT ( 'NONE',  ( -92.35000000000003695, 90.00000000000004263, 77.61749999999999261 ) ) ;
#57668=CARTESIAN_POINT ( 'NONE',  ( -97.30629616937501680, 90.00000000000004263, 78.21281250086714465 ) ) ;
#57672=EDGE_CURVE ( 'NONE', #73292, #58350, #8384, .T. ) ;
#57673=EDGE_CURVE ( 'NONE', #13102, #35941, #19359, .T. ) ;
#57678=CARTESIAN_POINT ( 'NONE',  ( -94.99999999999997158, -207.3369185715606307, 87.10281250086715943 ) ) ;
#57681=CARTESIAN_POINT ( 'NONE',  ( 97.30629616937498838, 88.66845928578035796, 78.00114583420049996 ) ) ;
#57682=CARTESIAN_POINT ( 'NONE',  ( -94.99999999999997158, -212.6630814284392557, 80.43531250086715545 ) ) ;
#57684=VECTOR ( 'NONE', #32753, 1000.000000000000000 ) ;
#57686=CARTESIAN_POINT ( 'NONE',  ( 92.34999999999999432, 90.00000000000002842, 87.53937500173429953 ) ) ;
#57687=CARTESIAN_POINT ( 'NONE',  ( -97.64999999999996305, -209.9999999999999716, 75.39499999999999602 ) ) ;
#57692=CARTESIAN_POINT ( 'NONE',  ( -93.33921851433964889, 88.39974787049349914, 74.80065602173004891 ) ) ;
#57693=CARTESIAN_POINT ( 'NONE',  ( 92.69370383062501162, -211.3315407142195852, 76.36072916753381890 ) ) ;
#57696=EDGE_LOOP ( 'NONE', ( #17203, #55720, #41404, #68615 ) ) ;
#57700=VERTEX_POINT ( 'NONE', #35479 ) ;
#57703=CARTESIAN_POINT ( 'NONE',  ( 96.32499999999998863, -207.7050326799711968, 79.70770833506762187 ) ) ;
#57704=VERTEX_POINT ( 'NONE', #7287 ) ;
#57706=CARTESIAN_POINT ( 'NONE',  ( 94.99999999999998579, 92.66308142843935514, 82.65781250086715204 ) ) ;
#57707=CARTESIAN_POINT ( 'NONE',  ( 97.64999999999999147, -209.9999999999999716, 75.71250000000000568 ) ) ;
#57718=ADVANCED_FACE ( 'NONE', ( #69693 ), #573, .F. ) ;
#57726=CARTESIAN_POINT ( 'NONE',  ( -94.99999999999997158, -206.9400435732949575, 78.49062500173430124 ) ) ;
#57730=CARTESIAN_POINT ( 'NONE',  ( 94.99999999999998579, 93.05995642670504253, 80.39562500173431658 ) ) ;
#57731=CARTESIAN_POINT ( 'NONE',  ( -93.67500000000003979, 87.70503267997129626, 79.49604166840096298 ) ) ;
#57734=CARTESIAN_POINT ( 'NONE',  ( 94.99999999999998579, 92.66308142843935514, 80.75281250086715090 ) ) ;
#57739=CARTESIAN_POINT ( 'NONE',  ( -93.67500000000003979, 92.29496732002878900, 80.26333333333332121 ) ) ;
#57740=EDGE_CURVE ( 'NONE', #57704, #22794, #65483, .T. ) ;
#57744=ORIENTED_EDGE ( 'NONE', *, *, #5640, .F. ) ;
#57750=CARTESIAN_POINT ( 'NONE',  ( -100.0000000000000142, 95.00000000000002842, 90.00000000000000000 ) ) ;
#57751=CARTESIAN_POINT ( 'NONE',  ( -97.30629616937497417, -211.3315407142195852, 76.51947916753381662 ) ) ;
#57758=CARTESIAN_POINT ( 'NONE',  ( 97.30629616937498838, 88.66845928578035796, 75.93739583420050110 ) ) ;
#57765=CARTESIAN_POINT ( 'NONE',  ( 94.99999999999998579, 87.33691857156068750, 86.15031250086717307 ) ) ;
#57772=CARTESIAN_POINT ( 'NONE',  ( -92.69370383062505425, 91.33154071421968467, 81.12322916753380753 ) ) ;
#57774=CARTESIAN_POINT ( 'NONE',  ( 92.69370383062501162, -208.6684592857803011, 87.04989583420048405 ) ) ;
#57777=CARTESIAN_POINT ( 'NONE',  ( 93.67499999999999716, 87.70503267997126784, 87.01020833506763097 ) ) ;
#57784=EDGE_CURVE ( 'NONE', #2928, #17937, #13630, .T. ) ;
#57787=ADVANCED_FACE ( 'NONE', ( #17814 ), #69055, .F. ) ;
#57788=CARTESIAN_POINT ( 'NONE',  ( 92.69370383062501162, -211.3315407142195852, 80.32947916753381890 ) ) ;
#57790=CARTESIAN_POINT ( 'NONE',  ( 97.65000000000009095, 91.52997821335246442, 80.84541666666663673 ) ) ;
#57792=( BOUNDED_CURVE ( )  B_SPLINE_CURVE ( 2, ( #28539, #29277, #761, #40955, #28173, #63888, #58230 ),
 .UNSPECIFIED., .F., .F. ) 
 B_SPLINE_CURVE_WITH_KNOTS ( ( 3, 2, 2, 3 ),
 ( 0.7831899741065913023, 0.7902457405788253508, 0.7973015061197077369, 0.8043570860654217780 ),
 .UNSPECIFIED. ) 
 CURVE ( )  GEOMETRIC_REPRESENTATION_ITEM ( )  RATIONAL_B_SPLINE_CURVE ( ( 1.000000000000000000, 0.8660254037844387076, 1.000000000000000000, 0.8660254037844387076, 1.000000000000000000, 0.8660289278581336792, 0.9999929520380047565 ) ) 
 REPRESENTATION_ITEM ( '' )  );
#57794=CARTESIAN_POINT ( 'NONE',  ( 94.99999999999998579, 93.05995642670504253, 83.57062500173429953 ) ) ;
#57796=CARTESIAN_POINT ( 'NONE',  ( 92.35000000000000853, -209.9999999999999716, 84.92000000000000171 ) ) ;
#57803=CARTESIAN_POINT ( 'NONE',  ( -97.30629616937501680, 88.66845928578038638, 88.58447916753382856 ) ) ;
#57807=CARTESIAN_POINT ( 'NONE',  ( 92.35000000000002274, -208.4700217866474645, 77.96145833506763267 ) ) ;
#57808=CARTESIAN_POINT ( 'NONE',  ( 94.99999999999998579, 93.05995642670504253, 77.14124999999999943 ) ) ;
#57814=CARTESIAN_POINT ( 'NONE',  ( 92.35000752690150705, -211.5299825590110743, 88.22729196900364457 ) ) ;
#57815=CARTESIAN_POINT ( 'NONE',  ( -93.84685191531254134, 91.99731107132950569, 80.06489583420048461 ) ) ;
#57817=CARTESIAN_POINT ( 'NONE',  ( 92.69370383062498320, 90.00000000000002842, 88.53156250086716739 ) ) ;
#57818=ORIENTED_EDGE ( 'NONE', *, *, #7280, .T. ) ;
#57821=CARTESIAN_POINT ( 'NONE',  ( 92.34999999999998010, -211.5299782133523934, 85.60791666666665378 ) ) ;
#57825=VERTEX_POINT ( 'NONE', #31680 ) ;
#57828=CARTESIAN_POINT ( 'NONE',  ( -96.15314808468747287, -208.0026889286704943, 77.47197916753380298 ) ) ;
#57836=EDGE_CURVE ( 'NONE', #37739, #51621, #26595, .T. ) ;
#57838=LINE ( 'NONE', #39432, #71244 ) ;
#57840=CARTESIAN_POINT ( 'NONE',  ( -92.69370383062498320, -211.3315407142195852, 88.79614583420050167 ) ) ;
#57842=CARTESIAN_POINT ( 'NONE',  ( -96.32499999999996021, -207.7050326799711968, 81.63916666666666799 ) ) ;
#57849=CARTESIAN_POINT ( 'NONE',  ( 92.69370383062498320, 91.33154071421968467, 85.77989583420048803 ) ) ;
#57853=DIRECTION ( 'NONE',  ( 1.000000000000000000, 0.000000000000000000, 0.000000000000000000 ) ) ;
#57872=CARTESIAN_POINT ( 'NONE',  ( 92.69370383062501162, -208.6684592857803011, 85.93864583420048575 ) ) ;
#57879=CARTESIAN_POINT ( 'NONE',  ( -97.65000000000004832, -208.4700217866474929, 86.13708333333332234 ) ) ;
#57884=ORIENTED_EDGE ( 'NONE', *, *, #9744, .T. ) ;
#57885=CARTESIAN_POINT ( 'NONE',  ( 97.30629616937498838, -208.6684592857803011, 83.82197916753382572 ) ) ;
#57896=CYLINDRICAL_SURFACE ( 'NONE', #43663, 2.649999999999985700 ) ;
#57899=CARTESIAN_POINT ( 'NONE',  ( 97.64999999999997726, -208.4700217866474645, 87.27479166840096525 ) ) ;
#57900=EDGE_LOOP ( 'NONE', ( #54, #51431, #67316, #36238 ) ) ;
#57901=CARTESIAN_POINT ( 'NONE',  ( -97.65000000000001990, 90.00000000000004263, 84.28499999999999659 ) ) ;
#57916=CARTESIAN_POINT ( 'NONE',  ( -96.32500000000001705, 87.70503267997129626, 87.56583333333333030 ) ) ;
#57918=VERTEX_POINT ( 'NONE', #65543 ) ;
#57920=EDGE_LOOP ( 'NONE', ( #16553, #34931, #32039, #64487 ) ) ;
#57921=CARTESIAN_POINT ( 'NONE',  ( 96.32499999999997442, 92.29496732002878900, 75.18333333333332291 ) ) ;
#57922=CARTESIAN_POINT ( 'NONE',  ( -96.15314808468747287, -208.0026889286704943, 87.63197916753379957 ) ) ;
#57926=CARTESIAN_POINT ( 'NONE',  ( 92.71977365048361719, -211.1627451397776269, 74.94226573542110259 ) ) ;
#57927=CARTESIAN_POINT ( 'NONE',  ( 97.65000000000004832, 88.47002178664756400, 81.37458333333333371 ) ) ;
#57928=CARTESIAN_POINT ( 'NONE',  ( -97.30629616937497417, -208.6684592857803295, 75.61989583420047722 ) ) ;
#57933=DIRECTION ( 'NONE',  ( 1.343011723336882952E-16, -1.000000000000000000, 0.000000000000000000 ) ) ;
#57936=CARTESIAN_POINT ( 'NONE',  ( -96.15314808468751551, 88.00268892867056536, 78.95364583420047211 ) ) ;
#57944=LINE ( 'NONE', #73362, #56236 ) ;
#57948=CARTESIAN_POINT ( 'NONE',  ( -97.30629616937497417, -208.6684592857803011, 77.68364583420047609 ) ) ;
#57949=DIRECTION ( 'NONE',  ( -0.000000000000000000, -0.000000000000000000, 1.000000000000000000 ) ) ;
#57956=EDGE_CURVE ( 'NONE', #56878, #66338, #72996, .T. ) ;
#57963=CARTESIAN_POINT ( 'NONE',  ( 92.69370383062501162, -209.9999999999999716, 85.19781250086714408 ) ) ;
#57972=CARTESIAN_POINT ( 'NONE',  ( -93.84685191531254134, 91.99731107132950569, 79.42989583420049371 ) ) ;
#57976=EDGE_LOOP ( 'NONE', ( #13592, #60615, #53191, #56430 ) ) ;
#57985=ORIENTED_EDGE ( 'NONE', *, *, #4675, .F. ) ;
#57989=CARTESIAN_POINT ( 'NONE',  ( 97.30629616937498838, -208.6684592857803011, 81.75822916753381264 ) ) ;
#57997=CARTESIAN_POINT ( 'NONE',  ( -97.64999999999996305, -209.9999999999999716, 85.55499999999999261 ) ) ;
#57998=CARTESIAN_POINT ( 'NONE',  ( -93.84685191531248449, -208.0026889286704943, 83.71614583420047495 ) ) ;
#57999=CARTESIAN_POINT ( 'NONE',  ( -97.30629616937501680, 90.00000000000004263, 82.18156250086715886 ) ) ;
#58001=ORIENTED_EDGE ( 'NONE', *, *, #44931, .T. ) ;
#58002=CARTESIAN_POINT ( 'NONE',  ( 93.84685191531248449, 88.00268892867053694, 84.66864583420047552 ) ) ;
#58004=CARTESIAN_POINT ( 'NONE',  ( -92.35000000053409508, 90.00005320149026034, 78.96687695417308817 ) ) ;
#58008=CARTESIAN_POINT ( 'NONE',  ( -92.69370383062498320, -208.6684592857803295, 85.56822916753380071 ) ) ;
#58015=CARTESIAN_POINT ( 'NONE',  ( -95.00000000000002842, 93.05995642670501411, 79.04625000000000057 ) ) ;
#58017=CARTESIAN_POINT ( 'NONE',  ( -92.69370383062502583, 91.33154071421968467, 88.10822916753380696 ) ) ;
#58021=CARTESIAN_POINT ( 'NONE',  ( 93.67500000000001137, -207.7050326799711968, 77.90854166840097150 ) ) ;
#58023=( BOUNDED_CURVE ( )  B_SPLINE_CURVE ( 2, ( #21894, #15512, #26424, #10611, #50080, #49354, #67388 ),
 .UNSPECIFIED., .F., .F. ) 
 B_SPLINE_CURVE_WITH_KNOTS ( ( 3, 2, 2, 3 ),
 ( 0.1270039290057624060, 0.1340595452774234198, 0.1411153108183404170, 0.1481709449582802873 ),
 .UNSPECIFIED. ) 
 CURVE ( )  GEOMETRIC_REPRESENTATION_ITEM ( )  RATIONAL_B_SPLINE_CURVE ( ( 0.9999943314825013863, 0.8660282381031498833, 1.000000000000000000, 0.8660254037844387076, 1.000000000000000000, 0.8660278988209799689, 0.9999950100198486957 ) ) 
 REPRESENTATION_ITEM ( '' )  );
#58025=CARTESIAN_POINT ( 'NONE',  ( -96.15314808468752972, 91.99731107132950569, 77.47197916753380298 ) ) ;
#58032=CARTESIAN_POINT ( 'NONE',  ( -97.30629616937495996, -209.9999999999999716, 87.26156250086715715 ) ) ;
#58033=CARTESIAN_POINT ( 'NONE',  ( 95.00000000000000000, -213.0599564267049857, 83.17374999999999829 ) ) ;
#58036=CARTESIAN_POINT ( 'NONE',  ( 97.30629616937498838, 91.33154071421968467, 75.56697916753383026 ) ) ;
#58037=EDGE_CURVE ( 'NONE', #7004, #8687, #16247, .T. ) ;
#58038=CARTESIAN_POINT ( 'NONE',  ( -93.84685191531247028, -211.9973110713294489, 75.40822916753381833 ) ) ;
#58042=CARTESIAN_POINT ( 'NONE',  ( 97.64999999999999147, -209.9999999999999716, 80.79249999999998977 ) ) ;
#58051=CARTESIAN_POINT ( 'NONE',  ( 95.00000000000000000, -212.6630814284392557, 77.73656250086713726 ) ) ;
#58067=CARTESIAN_POINT ( 'NONE',  ( 92.69370383062498320, 91.33154071421968467, 84.03364583420049883 ) ) ;
#58069=CARTESIAN_POINT ( 'NONE',  ( 95.00000000000000000, -213.0599564267049857, 76.18874999999999886 ) ) ;
#58070=VERTEX_POINT ( 'NONE', #4989 ) ;
#58072=CARTESIAN_POINT ( 'NONE',  ( -92.34999999999999432, -209.9999999999999716, 83.33250000000001023 ) ) ;
#58075=ORIENTED_EDGE ( 'NONE', *, *, #29840, .T. ) ;
#58076=ADVANCED_FACE ( 'NONE', ( #27892 ), #50817, .F. ) ;
#58077=ORIENTED_EDGE ( 'NONE', *, *, #3601, .T. ) ;
#58083=CARTESIAN_POINT ( 'NONE',  ( -95.00000000000002842, 90.00000000000004263, 90.00000000000000000 ) ) ;
#58088=CARTESIAN_POINT ( 'NONE',  ( -94.99999999999997158, -206.9400435732949575, 77.85562500173429612 ) ) ;
#58093=CARTESIAN_POINT ( 'NONE',  ( 96.32499999999998863, 87.70503267997126784, 78.22604166840096696 ) ) ;
#58094=CARTESIAN_POINT ( 'NONE',  ( -92.35000000000005116, 88.47002178664754979, 78.91395833506763324 ) ) ;
#58097=CARTESIAN_POINT ( 'NONE',  ( 96.15314808468748708, 88.00268892867053694, 78.58322916753382970 ) ) ;
#58099=CARTESIAN_POINT ( 'NONE',  ( 92.34999999999999432, 90.00000000000002842, 75.39499999999999602 ) ) ;
#58113=CARTESIAN_POINT ( 'NONE',  ( -93.84685191531247028, -211.9973110713294489, 79.21822916753382060 ) ) ;
#58117=CARTESIAN_POINT ( 'NONE',  ( -97.20211296431911308, -211.3166576149945115, 74.94590613650854038 ) ) ;
#58125=AXIS2_PLACEMENT_3D ( 'NONE', #10766, #27296, #23169 ) ;
#58126=CARTESIAN_POINT ( 'NONE',  ( 94.99999999999998579, 87.33691857156068750, 88.69031250086716511 ) ) ;
#58132=CARTESIAN_POINT ( 'NONE',  ( -97.30629616937501680, 91.33154071421968467, 74.98489583420048632 ) ) ;
#58137=CARTESIAN_POINT ( 'NONE',  ( 95.00000000000000000, -212.6630814284392557, 86.62656250086715204 ) ) ;
#58149=CARTESIAN_POINT ( 'NONE',  ( 96.15314808468748708, -208.0026889286704943, 82.60489583420049087 ) ) ;
#58156=CARTESIAN_POINT ( 'NONE',  ( 92.35000000000002274, -211.5299782133524502, 83.70291666666668107 ) ) ;
#58164=EDGE_CURVE ( 'NONE', #32383, #13338, #33847, .T. ) ;
#58165=CARTESIAN_POINT ( 'NONE',  ( -96.15314808468751551, 88.00268892867056536, 88.00239583420048461 ) ) ;
#58168=CARTESIAN_POINT ( 'NONE',  ( 93.67500000000001137, -207.7050326799711968, 76.00354166840097037 ) ) ;
#58169=CARTESIAN_POINT ( 'NONE',  ( 96.32499999999998863, 87.70503267997126784, 76.87666666666666515 ) ) ;
#58171=CARTESIAN_POINT ( 'NONE',  ( -92.34999999999999432, -208.4700217866474645, 89.17979166840096639 ) ) ;
#58175=FACE_OUTER_BOUND ( 'NONE', #51343, .T. ) ;
#58176=CARTESIAN_POINT ( 'NONE',  ( -93.84685191531254134, 91.99731107132950569, 81.33489583420049485 ) ) ;
#58177=CARTESIAN_POINT ( 'NONE',  ( 96.15314808468748708, 91.99731107132950569, 75.46114583420047950 ) ) ;
#58185=CARTESIAN_POINT ( 'NONE',  ( -95.00000000000002842, 93.05995642670504253, 81.66562500173431260 ) ) ;
#58189=ORIENTED_EDGE ( 'NONE', *, *, #41239, .T. ) ;
#58193=CARTESIAN_POINT ( 'NONE',  ( -93.84685191531247028, -211.9973110713294489, 86.83822916753382515 ) ) ;
#58198=VECTOR ( 'NONE', #67327, 1000.000000000000000 ) ;
#58202=AXIS2_PLACEMENT_3D ( 'NONE', #58409, #35840, #29824 ) ;
#58204=CARTESIAN_POINT ( 'NONE',  ( 94.99999999999998579, 87.33691857156068750, 80.91156250086714863 ) ) ;
#58206=CARTESIAN_POINT ( 'NONE',  ( -97.64999999990727986, 90.00001381026693537, 80.55392363656929433 ) ) ;
#58210=CARTESIAN_POINT ( 'NONE',  ( -93.67500000000003979, 92.29496732002878900, 84.15270833506762926 ) ) ;
#58217=CARTESIAN_POINT ( 'NONE',  ( -93.84685191531254134, 91.99731107132950569, 88.79614583420047325 ) ) ;
#58224=( BOUNDED_CURVE ( )  B_SPLINE_CURVE ( 2, ( #33158, #60649, #56107, #27525, #66651, #26420, #15131 ),
 .UNSPECIFIED., .F., .F. ) 
 B_SPLINE_CURVE_WITH_KNOTS ( ( 3, 2, 2, 3 ),
 ( 0.7499999999999996669, 0.7569444444444439757, 0.7638888888888883955, 0.7708333333333328152 ),
 .UNSPECIFIED. ) 
 CURVE ( )  GEOMETRIC_REPRESENTATION_ITEM ( )  RATIONAL_B_SPLINE_CURVE ( ( 1.000000000000006439, 0.8660254037844322683, 1.000000000000000000, 0.8660254037844387076, 1.000000000000000000, 0.8660254037844493658, 0.9999999999999893419 ) ) 
 REPRESENTATION_ITEM ( '' )  );
#58226=CARTESIAN_POINT ( 'NONE',  ( -97.64999999999996305, -209.9999999999999716, 90.00000000000000000 ) ) ;
#58229=CYLINDRICAL_SURFACE ( 'NONE', #17806, 2.649999999999985700 ) ;
#58230=CARTESIAN_POINT ( 'NONE',  ( -97.64999999953592180, 89.99996903277666149, 77.38038495128051864 ) ) ;
#58233=CARTESIAN_POINT ( 'NONE',  ( 92.69370383062501162, -208.6684592857803011, 85.30364583420048064 ) ) ;
#58241=CARTESIAN_POINT ( 'NONE',  ( 96.15314808468750130, -211.9973110713294489, 75.88447916753381151 ) ) ;
#58245=CARTESIAN_POINT ( 'NONE',  ( 93.84685191531251292, -211.9973110713294489, 78.47739583420049314 ) ) ;
#58257=CARTESIAN_POINT ( 'NONE',  ( 97.64999999999997726, -208.4700217866474645, 86.63979166840097434 ) ) ;
#58258=CARTESIAN_POINT ( 'NONE',  ( 96.32499999999998863, 87.70503267997126784, 88.30666666666665776 ) ) ;
#58265=CARTESIAN_POINT ( 'NONE',  ( 93.67499999999999716, 87.70503267997126784, 85.10520833506762983 ) ) ;
#58268=EDGE_LOOP ( 'NONE', ( #21948, #13399, #44862, #6052 ) ) ;
#58278=CARTESIAN_POINT ( 'NONE',  ( -92.35000000000005116, 91.52997821335253548, 89.10041666666667481 ) ) ;
#58279=EDGE_LOOP ( 'NONE', ( #42514, #67141, #68631, #6382 ) ) ;
#58283=CARTESIAN_POINT ( 'NONE',  ( 97.64999999999999147, 90.00000000000002842, 90.00000000000000000 ) ) ;
#58284=CARTESIAN_POINT ( 'NONE',  ( -96.15314808468745866, -211.9973110713294489, 83.39864583420047950 ) ) ;
#58287=CARTESIAN_POINT ( 'NONE',  ( 92.79788703567045616, -211.3166576149753269, 74.94590613650809985 ) ) ;
#58289=CARTESIAN_POINT ( 'NONE',  ( -94.99999999999997158, -207.3369185715606307, 76.78406250086712248 ) ) ;
#58295=ADVANCED_FACE ( 'NONE', ( #55915 ), #9681, .F. ) ;
#58299=CARTESIAN_POINT ( 'NONE',  ( -93.84685191531254134, 91.99731107132950569, 77.36614583420046642 ) ) ;
#58312=CARTESIAN_POINT ( 'NONE',  ( -97.30629616937495996, -209.9999999999999716, 75.83156250086716454 ) ) ;
#58319=CARTESIAN_POINT ( 'NONE',  ( 95.00000000000000000, -213.0599564267049857, 88.25374999999999659 ) ) ;
#58329=CARTESIAN_POINT ( 'NONE',  ( 97.30629616937498838, -209.9999999999999716, 83.61031250086713840 ) ) ;
#58331=ADVANCED_FACE ( 'NONE', ( #39003 ), #38634, .F. ) ;
#58335=CARTESIAN_POINT ( 'NONE',  ( 92.35000000000002274, -209.9999907079572381, 84.99937468035460597 ) ) ;
#58337=CARTESIAN_POINT ( 'NONE',  ( -97.30629616937501680, 90.00000000000004263, 80.91156250086716284 ) ) ;
#58342=CARTESIAN_POINT ( 'NONE',  ( 95.00000000000000000, -206.9400435732949575, 84.84062500173429555 ) ) ;
#58346=VERTEX_POINT ( 'NONE', #61193 ) ;
#58349=ORIENTED_EDGE ( 'NONE', *, *, #37623, .F. ) ;
#58350=VERTEX_POINT ( 'NONE', #9303 ) ;
#58352=CARTESIAN_POINT ( 'NONE',  ( 97.30629616937498838, -208.6684592857803011, 83.02822916753379445 ) ) ;
#58353=SHAPE_DEFINITION_REPRESENTATION ( #43387, #65179 ) ;
#58356=CARTESIAN_POINT ( 'NONE',  ( 92.34999999999999432, 88.47002178664752137, 84.97291666666667709 ) ) ;
#58360=CARTESIAN_POINT ( 'NONE',  ( -95.00000000000002842, 86.94004357329504273, 82.53874999999999318 ) ) ;
#58361=CARTESIAN_POINT ( 'NONE',  ( -93.84685191531247028, -211.9973110713294489, 83.50447916753381605 ) ) ;
#58362=CARTESIAN_POINT ( 'NONE',  ( -95.00000000000002842, 87.33691857156074434, 81.70531250086715147 ) ) ;
#58364=AXIS2_PLACEMENT_3D ( 'NONE', #71499, #25651, #48588 ) ;
#58365=CARTESIAN_POINT ( 'NONE',  ( 96.15314808468748708, 91.99731107132950569, 84.35114583420048007 ) ) ;
#58368=CARTESIAN_POINT ( 'NONE',  ( -97.65000000000001990, 90.00001683226682303, 78.64937441956426767 ) ) ;
#58373=CARTESIAN_POINT ( 'NONE',  ( -96.15314808468745866, -211.9973110713294489, 87.20864583420046756 ) ) ;
#58376=DIRECTION ( 'NONE',  ( -0.000000000000000000, -0.000000000000000000, 1.000000000000000000 ) ) ;
#58383=CARTESIAN_POINT ( 'NONE',  ( -95.00000000000002842, 86.94004357329504273, 79.36374999999999602 ) ) ;
#58384=EDGE_CURVE ( 'NONE', #28568, #31708, #55547, .T. ) ;
#58385=CARTESIAN_POINT ( 'NONE',  ( -97.30629616937501680, 90.00000000000004263, 89.64281250086713726 ) ) ;
#58386=FACE_OUTER_BOUND ( 'NONE', #56305, .T. ) ;
#58390=VERTEX_POINT ( 'NONE', #66102 ) ;
#58391=CARTESIAN_POINT ( 'NONE',  ( -2.500000000000020428, -90.00000000000000000, -90.00000000000000000 ) ) ;
#58399=CARTESIAN_POINT ( 'NONE',  ( -97.30629616937495996, -209.9999999999999716, 84.72156250086715090 ) ) ;
#58402=VECTOR ( 'NONE', #56063, 1000.000000000000000 ) ;
#58403=CARTESIAN_POINT ( 'NONE',  ( 92.69370383062498320, 91.33154071421968467, 77.68364583420047609 ) ) ;
#58404=CARTESIAN_POINT ( 'NONE',  ( -93.84685191531247028, -211.9973110713294489, 76.04322916753382344 ) ) ;
#58406=ORIENTED_EDGE ( 'NONE', *, *, #49580, .F. ) ;
#58407=CARTESIAN_POINT ( 'NONE',  ( 96.32499999999998863, 87.70503267997126784, 87.75104166840095843 ) ) ;
#58409=CARTESIAN_POINT ( 'NONE',  ( 95.00000000000000000, -209.9999999999999716, 90.00000000000000000 ) ) ;
#58413=CARTESIAN_POINT ( 'NONE',  ( 97.30629616937498838, -209.9999999999999716, 77.89531250086714920 ) ) ;
#58425=EDGE_LOOP ( 'NONE', ( #20031, #28178, #29317, #24052 ) ) ;
#58430=CARTESIAN_POINT ( 'NONE',  ( 93.84685191531248449, 88.00268892867053694, 82.28739583420048120 ) ) ;
#58433=VERTEX_POINT ( 'NONE', #72452 ) ;
#58435=ORIENTED_EDGE ( 'NONE', *, *, #3599, .F. ) ;
#58436=DIRECTION ( 'NONE',  ( -1.000000000000000000, 3.061616997868382648E-16, 0.000000000000000000 ) ) ;
#58443=DIRECTION ( 'NONE',  ( -0.000000000000000000, -0.000000000000000000, 1.000000000000000000 ) ) ;
#58445=CARTESIAN_POINT ( 'NONE',  ( -92.34999999999999432, -208.4700217866474645, 80.92479166840098515 ) ) ;
#58449=ADVANCED_FACE ( 'NONE', ( #43909 ), #41460, .F. ) ;
#58450=CARTESIAN_POINT ( 'NONE',  ( 92.34999999999999432, 91.52997821335252127, 78.59645833506763779 ) ) ;
#58451=CARTESIAN_POINT ( 'NONE',  ( -97.65000000000001990, 91.52997821335253548, 76.69145833506763665 ) ) ;
#58452=( BOUNDED_SURFACE ( )  B_SPLINE_SURFACE ( 1, 2, ( 
 ( #42841, #60151, #10104, #72861, #21367, #61250, #54855, #49575, #20267, #44326, #33028, #27383, #25913, #66517, #55223, #9735, #3747, #48839, #26648, #66155, #21006, #67255, #72504, #60512, #50324, #14632, #73250, #66874, #8993, #31917, #15364, #38311, #19148, #24420, #71009, #1538, #65032, #53731, #59015, #53001, #58628, #792, #19512, #6405, #1904, #29670, #35340, #70633, #13509, #24068, #47357, #36803, #52618, #30417, #7137, #1171, #46992, #30783, #46614, #64646, #42093, #35687, #25169, #63921, #53363, #36434, #59380, #2273, #24789, #65400, #70263, #52250, #69904, #30050, #7868, #18770, #47720, #48095, #13131, #6761, #42460, #69547, #58265, #13865, #29306, #18044, #40986, #18400, #64289, #41347, #12393, #41709, #23682, #12760, #36069, #7507, #71376, #45344, #27277, #19880, #67518, #4757, #25898, #16383, #25526, #61888, #60137, #42827, #33670, #31165, #16006, #5124, #67893, #59752, #50588, #73888, #31905, #56625, #37195, #22397, #10368, #22022, #33288, #55867, #54115, #39325, #20247, #44601, #48460, #43217, #4379, #73515, #66140, #14617, #8234, #2647, #28025, #62261, #44967, #27663, #71744, #38952, #8619, #10746, #50967, #68268, #65757, #37566, #60499, #16764, #8980, #14240, #50207, #31530, #56242, #54469, #73141, #3005, #48826, #21647, #35523, #46074, #23883, #70093, #47181, #617, #45724, #57351, #6948, #40060, #260, #57730, #56992, #46439, #63021, #23508, #1366, #39702, #35157, #69367, #69734, #989, #69009, #24257, #64111, #29136, #52072, #62641, #17495, #12592, #5863, #11117, #46819, #5497, #28393, #29872, #12220, #34789, #63372, #17863, #52435, #6236, #52824, #40809, #18234, #58450, #63744, #11838, #40424, #34041, #51329, #74265, #58093, #11480, #68646, #29499, #41175, #28772, #6595, #22782, #34408, #17128, #51712, #23151, #36262, #43026, #65588, #65220, #42650, #71574, #7333, #24980, #14055, #47915, #19702, #30608, #53936, #35885, #7691, #70834, #49015, #8443, #71196, #2831, #64473, #59958, #42291, #31354, #13691, #12948, #8059, #65967, #18960, #58833, #53556, #2093, #54667, #36628, #59573, #30249, #37393, #37005, #54306, #2474, #24612, #25361, #19335, #30980, #3195, #48288, #25720, #48659, #64849, #20071, #14439, #60327, #47549, #70453, #8805, #26085, #31722, #13328, #53188, #18596, #41536 ),
 ( #1724, #41909, #59200, #14809, #39235, #4666, #33203, #15924, #9547, #4296, #49395, #73429, #44879, #67801, #60690, #32463, #3928, #38857, #49750, #20460, #38490, #9169, #16295, #44511, #73047, #55778, #3561, #27184, #26824, #72673, #33577, #21175, #61800, #56147, #43772, #55405, #44126, #67050, #26459, #72321, #27573, #56534, #15557, #66691, #43414, #9908, #62165, #61050, #20820, #61429, #10281, #32829, #71946, #38111, #32092, #50112, #67428, #10651, #21553, #50501, #37756, #5037, #27942, #21936, #66336, #55032, #15177, #57266, #63659, #11390, #17041, #46726, #34324, #29405, #23062, #74173, #63286, #12500, #5771, #900, #39977, #35435, #35071, #68170, #39608, #41090, #23423, #45991, #171, #29052, #12128, #68919, #64023, #17405, #58002, #23787, #51982, #40340, #28678, #45253, #58365, #50872, #46354, #22688, #5410, #40715, #6506, #68554, #11745, #6865, #45636, #528, #51619, #62932, #34692, #69650, #69284, #57646, #17769, #52353, #62550, #6146, #18144, #73795, #22309, #16670, #11031, #33955, #56904, #28305, #51241, #19616, #7972, #13968, #1280, #71110, #53468, #42562, #2005, #24167, #19250, #54219, #30157, #47100, #18873, #41811, #65868, #47822, #70744, #36536, #48199, #70367, #59859, #70004, #30890, #53102, #64389, #2749, #18507, #59482, #48569, #36912, #29776, #65501, #42937, #24895, #25633, #7245, #14353, #53834, #8348, #2382, #42200, #41447, #31270, #64758, #13609, #12861, #13243, #65135, #71481, #36172, #59118, #52730, #35790, #19982, #37304, #60239, #58745, #7607, #25275, #1640, #24525, #47460, #30521, #71847, #43682, #15082, #27094, #60955, #31635, #49660, #54578, #61339, #21454, #26729, #26368, #72951, #3105, #4574, #38023, #67337, #39140, #16201, #44043, #14716, #49298, #50407, #9078, #66602, #72585, #25999, #15454, #32003, #66957, #44788, #8718, #4202, #38399, #38766, #44416, #9446, #67711, #33108, #21085, #48924, #9818, #15837, #32371, #27470, #66242, #32734, #61704, #10186, #56057, #55686, #20364, #50026, #43321, #3463, #55314, #73334, #21841, #37667, #60601, #54943, #72223, #20730, #3832, #16573, #23336, #17688, #73706, #27850, #74082, #45540, #10941, #22216, #57180, #62078, #69560, #69196, #5321, #45158, #46632, #28585, #68082, #62840, #33864, #28219, #12042, #34602, #34236, #11660, #40625 ) ),
 .UNSPECIFIED., .F., .F., .F. ) 
 B_SPLINE_SURFACE_WITH_KNOTS ( ( 2, 2 ),
 ( 3, 2, 2, 2, 2, 2, 2, 2, 2, 2, 2, 2, 2, 2, 2, 2, 2, 2, 2, 2, 2, 2, 2, 2, 2, 2, 2, 2, 2, 2, 2, 2, 2, 2, 2, 2, 2, 2, 2, 2, 2, 2, 2, 2, 2, 2, 2, 2, 2, 2, 2, 2, 2, 2, 2, 2, 2, 2, 2, 2, 2, 2, 2, 2, 2, 2, 2, 2, 2, 2, 2, 2, 2, 2, 2, 2, 2, 2, 2, 2, 2, 2, 2, 2, 2, 2, 2, 2, 2, 2, 2, 2, 2, 2, 2, 2, 2, 2, 2, 2, 2, 2, 2, 2, 2, 2, 2, 2, 2, 2, 2, 2, 2, 2, 2, 2, 2, 2, 2, 2, 2, 2, 2, 2, 2, 2, 2, 2, 2, 2, 2, 2, 2, 2, 2, 2, 2, 2, 2, 2, 2, 2, 3 ),
 ( 0.000000000000000000, 1.000000000000000000 ),
 ( 0.000000000000000000, 0.006944444444444444059, 0.01388888888888888812, 0.02083333333333333218, 0.02777777777777777624, 0.03472222222222222376, 0.04166666666666666435, 0.04861111111111111188, 0.05555555555555555247, 0.06250000000000000000, 0.06944444444444444753, 0.07638888888888889506, 0.08333333333333332871, 0.09027777777777777624, 0.09722222222222222376, 0.1041666666666666713, 0.1111111111111111049, 0.1180555555555555525, 0.1250000000000000000, 0.1319444444444444475, 0.1388888888888888951, 0.1458333333333333426, 0.1527777777777777901, 0.1597222222222222099, 0.1666666666666666574, 0.1736111111111111049, 0.1805555555555555525, 0.1875000000000000000, 0.1944444444444444475, 0.2013888888888888951, 0.2083333333333333426, 0.2152777777777777901, 0.2222222222222222099, 0.2291666666666666574, 0.2361111111111111049, 0.2430555555555555525, 0.2500000000000000000, 0.2569444444444444198, 0.2638888888888888951, 0.2708333333333333148, 0.2777777777777777901, 0.2847222222222222099, 0.2916666666666666852, 0.2986111111111111049, 0.3055555555555555802, 0.3125000000000000000, 0.3194444444444444198, 0.3263888888888888951, 0.3333333333333333148, 0.3402777777777777901, 0.3472222222222222099, 0.3541666666666666852, 0.3611111111111111049, 0.3680555555555555802, 0.3750000000000000000, 0.3819444444444444198, 0.3888888888888888951, 0.3958333333333333148, 0.4027777777777777901, 0.4097222222222222099, 0.4166666666666666852, 0.4236111111111111049, 0.4305555555555555802, 0.4375000000000000000, 0.4444444444444444198, 0.4513888888888888951, 0.4583333333333333148, 0.4652777777777777901, 0.4722222222222222099, 0.4791666666666666852, 0.4861111111111111049, 0.4930555555555555802, 0.5000000000000000000, 0.5069444444444444198, 0.5138888888888888395, 0.5208333333333333703, 0.5277777777777777901, 0.5347222222222222099, 0.5416666666666666297, 0.5486111111111111605, 0.5555555555555555802, 0.5625000000000000000, 0.5694444444444444198, 0.5763888888888888395, 0.5833333333333333703, 0.5902777777777777901, 0.5972222222222222099, 0.6041666666666666297, 0.6111111111111111605, 0.6180555555555555802, 0.6250000000000000000, 0.6319444444444444198, 0.6388888888888888395, 0.6458333333333333703, 0.6527777777777777901, 0.6597222222222222099, 0.6666666666666666297, 0.6736111111111111605, 0.6805555555555555802, 0.6875000000000000000, 0.6944444444444444198, 0.7013888888888888395, 0.7083333333333333703, 0.7152777777777777901, 0.7222222222222222099, 0.7291666666666666297, 0.7361111111111111605, 0.7430555555555555802, 0.7500000000000000000, 0.7569444444444444198, 0.7638888888888888395, 0.7708333333333333703, 0.7777777777777777901, 0.7847222222222222099, 0.7916666666666666297, 0.7986111111111111605, 0.8055555555555555802, 0.8125000000000000000, 0.8194444444444444198, 0.8263888888888888395, 0.8333333333333333703, 0.8402777777777777901, 0.8472222222222222099, 0.8541666666666666297, 0.8611111111111111605, 0.8680555555555555802, 0.8750000000000000000, 0.8819444444444444198, 0.8888888888888888395, 0.8958333333333333703, 0.9027777777777777901, 0.9097222222222222099, 0.9166666666666666297, 0.9236111111111111605, 0.9305555555555555802, 0.9375000000000000000, 0.9444444444444444198, 0.9513888888888888395, 0.9583333333333333703, 0.9652777777777777901, 0.9722222222222222099, 0.9791666666666666297, 0.9842226981114291506 ),
 .UNSPECIFIED. ) 
 GEOMETRIC_REPRESENTATION_ITEM ( )  RATIONAL_B_SPLINE_SURFACE ( (
 ( 1.000000000000000000, 0.8660254037844387076, 1.000000000000000000, 0.8660254037844387076, 1.000000000000000000, 0.8660254037844387076, 1.000000000000000000, 0.8660254037844387076, 1.000000000000000000, 0.8660254037844387076, 1.000000000000000000, 0.8660254037844387076, 1.000000000000000000, 0.8660254037844387076, 1.000000000000000000, 0.8660254037844387076, 1.000000000000000000, 0.8660254037844387076, 1.000000000000000000, 0.8660254037844387076, 1.000000000000000000, 0.8660254037844387076, 1.000000000000000000, 0.8660254037844387076, 1.000000000000000000, 0.8660254037844387076, 1.000000000000000000, 0.8660254037844387076, 1.000000000000000000, 0.8660254037844387076, 1.000000000000000000, 0.8660254037844387076, 1.000000000000000000, 0.8660254037844387076, 1.000000000000000000, 0.8660254037844387076, 1.000000000000000000, 0.8660254037844387076, 1.000000000000000000, 0.8660254037844387076, 1.000000000000000000, 0.8660254037844387076, 1.000000000000000000, 0.8660254037844387076, 1.000000000000000000, 0.8660254037844387076, 1.000000000000000000, 0.8660254037844387076, 1.000000000000000000, 0.8660254037844387076, 1.000000000000000000, 0.8660254037844387076, 1.000000000000000000, 0.8660254037844387076, 1.000000000000000000, 0.8660254037844387076, 1.000000000000000000, 0.8660254037844387076, 1.000000000000000000, 0.8660254037844387076, 1.000000000000000000, 0.8660254037844387076, 1.000000000000000000, 0.8660254037844387076, 1.000000000000000000, 0.8660254037844387076, 1.000000000000000000, 0.8660254037844387076, 1.000000000000000000, 0.8660254037844387076, 1.000000000000000000, 0.8660254037844387076, 1.000000000000000000, 0.8660254037844387076, 1.000000000000000000, 0.8660254037844387076, 1.000000000000000000, 0.8660254037844387076, 1.000000000000000000, 0.8660254037844387076, 1.000000000000000000, 0.8660254037844387076, 1.000000000000000000, 0.8660254037844387076, 1.000000000000000000, 0.8660254037844387076, 1.000000000000000000, 0.8660254037844387076, 1.000000000000000000, 0.8660254037844387076, 1.000000000000000000, 0.8660254037844387076, 1.000000000000000000, 0.8660254037844387076, 1.000000000000000000, 0.8660254037844387076, 1.000000000000000000, 0.8660254037844387076, 1.000000000000000000, 0.8660254037844387076, 1.000000000000000000, 0.8660254037844387076, 1.000000000000000000, 0.8660254037844387076, 1.000000000000000000, 0.8660254037844387076, 1.000000000000000000, 0.8660254037844387076, 1.000000000000000000, 0.8660254037844387076, 1.000000000000000000, 0.8660254037844387076, 1.000000000000000000, 0.8660254037844387076, 1.000000000000000000, 0.8660254037844387076, 1.000000000000000000, 0.8660254037844387076, 1.000000000000000000, 0.8660254037844387076, 1.000000000000000000, 0.8660254037844387076, 1.000000000000000000, 0.8660254037844387076, 1.000000000000000000, 0.8660254037844387076, 1.000000000000000000, 0.8660254037844387076, 1.000000000000000000, 0.8660254037844387076, 1.000000000000000000, 0.8660254037844387076, 1.000000000000000000, 0.8660254037844387076, 1.000000000000000000, 0.8660254037844387076, 1.000000000000000000, 0.8660254037844387076, 1.000000000000000000, 0.8660254037844387076, 1.000000000000000000, 0.8660254037844387076, 1.000000000000000000, 0.8660254037844387076, 1.000000000000000000, 0.8660254037844387076, 1.000000000000000000, 0.8660254037844387076, 1.000000000000000000, 0.8660254037844387076, 1.000000000000000000, 0.8660254037844387076, 1.000000000000000000, 0.8660254037844387076, 1.000000000000000000, 0.8660254037844387076, 1.000000000000000000, 0.8660254037844387076, 1.000000000000000000, 0.8660254037844387076, 1.000000000000000000, 0.8660254037844387076, 1.000000000000000000, 0.8660254037844387076, 1.000000000000000000, 0.8660254037844387076, 1.000000000000000000, 0.8660254037844387076, 1.000000000000000000, 0.8660254037844387076, 1.000000000000000000, 0.8660254037844387076, 1.000000000000000000, 0.8660254037844387076, 1.000000000000000000, 0.8660254037844387076, 1.000000000000000000, 0.8660254037844387076, 1.000000000000000000, 0.8660254037844387076, 1.000000000000000000, 0.8660254037844387076, 1.000000000000000000, 0.8660254037844387076, 1.000000000000000000, 0.8660254037844387076, 1.000000000000000000, 0.8660254037844387076, 1.000000000000000000, 0.8660254037844387076, 1.000000000000000000, 0.8660254037844387076, 1.000000000000000000, 0.8660254037844387076, 1.000000000000000000, 0.8660254037844387076, 1.000000000000000000, 0.8660254037844387076, 1.000000000000000000, 0.8660254037844387076, 1.000000000000000000, 0.8660254037844387076, 1.000000000000000000, 0.8660254037844387076, 1.000000000000000000, 0.8660254037844387076, 1.000000000000000000, 0.8660254037844387076, 1.000000000000000000, 0.8660254037844387076, 1.000000000000000000, 0.8660254037844387076, 1.000000000000000000, 0.8660254037844387076, 1.000000000000000000, 0.8660254037844387076, 1.000000000000000000, 0.8660254037844387076, 1.000000000000000000, 0.8660254037844387076, 1.000000000000000000, 0.8660254037844387076, 1.000000000000000000, 0.8660254037844387076, 1.000000000000000000, 0.8660254037844387076, 1.000000000000000000, 0.8660254037844387076, 1.000000000000000000, 0.8660254037844387076, 1.000000000000000000, 0.8660254037844387076, 1.000000000000000000, 0.8660254037844387076, 1.000000000000000000, 0.8660254037844387076, 1.000000000000000000, 0.8660254037844387076, 1.000000000000000000, 0.8660254037844387076, 1.000000000000000000, 0.8660254037844387076, 1.000000000000000000, 0.8660254037844387076, 1.000000000000000000, 0.8660254037844387076, 1.000000000000000000, 0.8660254037844387076, 1.000000000000000000, 0.8660254037844387076, 1.000000000000000000, 0.8660254037844387076, 1.000000000000000000, 0.8660254037844387076, 1.000000000000000000, 0.8660254037844387076, 1.000000000000000000, 0.8660254037844387076, 1.000000000000000000, 0.8660254037844387076, 1.000000000000000000, 0.8660254037844387076, 1.000000000000000000, 0.8660254037844387076, 1.000000000000000000, 0.8660254037844387076, 1.000000000000000000, 0.8660254037844387076, 1.000000000000000000, 0.8660254037844387076, 1.000000000000000000, 0.8660254037844387076, 1.000000000000000000, 0.8660254037844387076, 1.000000000000000000, 0.8660254037844387076, 1.000000000000000000, 0.8660254037844387076, 1.000000000000000000, 0.8660254037844387076, 1.000000000000000000, 0.8660254037844387076, 1.000000000000000000, 0.9024573129378067327, 0.9469501470576184854),
 ( 1.000000000000000000, 0.8660254037844387076, 1.000000000000000000, 0.8660254037844387076, 1.000000000000000000, 0.8660254037844387076, 1.000000000000000000, 0.8660254037844387076, 1.000000000000000000, 0.8660254037844387076, 1.000000000000000000, 0.8660254037844387076, 1.000000000000000000, 0.8660254037844387076, 1.000000000000000000, 0.8660254037844387076, 1.000000000000000000, 0.8660254037844387076, 1.000000000000000000, 0.8660254037844387076, 1.000000000000000000, 0.8660254037844387076, 1.000000000000000000, 0.8660254037844387076, 1.000000000000000000, 0.8660254037844387076, 1.000000000000000000, 0.8660254037844387076, 1.000000000000000000, 0.8660254037844387076, 1.000000000000000000, 0.8660254037844387076, 1.000000000000000000, 0.8660254037844387076, 1.000000000000000000, 0.8660254037844387076, 1.000000000000000000, 0.8660254037844387076, 1.000000000000000000, 0.8660254037844387076, 1.000000000000000000, 0.8660254037844387076, 1.000000000000000000, 0.8660254037844387076, 1.000000000000000000, 0.8660254037844387076, 1.000000000000000000, 0.8660254037844387076, 1.000000000000000000, 0.8660254037844387076, 1.000000000000000000, 0.8660254037844387076, 1.000000000000000000, 0.8660254037844387076, 1.000000000000000000, 0.8660254037844387076, 1.000000000000000000, 0.8660254037844387076, 1.000000000000000000, 0.8660254037844387076, 1.000000000000000000, 0.8660254037844387076, 1.000000000000000000, 0.8660254037844387076, 1.000000000000000000, 0.8660254037844387076, 1.000000000000000000, 0.8660254037844387076, 1.000000000000000000, 0.8660254037844387076, 1.000000000000000000, 0.8660254037844387076, 1.000000000000000000, 0.8660254037844387076, 1.000000000000000000, 0.8660254037844387076, 1.000000000000000000, 0.8660254037844387076, 1.000000000000000000, 0.8660254037844387076, 1.000000000000000000, 0.8660254037844387076, 1.000000000000000000, 0.8660254037844387076, 1.000000000000000000, 0.8660254037844387076, 1.000000000000000000, 0.8660254037844387076, 1.000000000000000000, 0.8660254037844387076, 1.000000000000000000, 0.8660254037844387076, 1.000000000000000000, 0.8660254037844387076, 1.000000000000000000, 0.8660254037844387076, 1.000000000000000000, 0.8660254037844387076, 1.000000000000000000, 0.8660254037844387076, 1.000000000000000000, 0.8660254037844387076, 1.000000000000000000, 0.8660254037844387076, 1.000000000000000000, 0.8660254037844387076, 1.000000000000000000, 0.8660254037844387076, 1.000000000000000000, 0.8660254037844387076, 1.000000000000000000, 0.8660254037844387076, 1.000000000000000000, 0.8660254037844387076, 1.000000000000000000, 0.8660254037844387076, 1.000000000000000000, 0.8660254037844387076, 1.000000000000000000, 0.8660254037844387076, 1.000000000000000000, 0.8660254037844387076, 1.000000000000000000, 0.8660254037844387076, 1.000000000000000000, 0.8660254037844387076, 1.000000000000000000, 0.8660254037844387076, 1.000000000000000000, 0.8660254037844387076, 1.000000000000000000, 0.8660254037844387076, 1.000000000000000000, 0.8660254037844387076, 1.000000000000000000, 0.8660254037844387076, 1.000000000000000000, 0.8660254037844387076, 1.000000000000000000, 0.8660254037844387076, 1.000000000000000000, 0.8660254037844387076, 1.000000000000000000, 0.8660254037844387076, 1.000000000000000000, 0.8660254037844387076, 1.000000000000000000, 0.8660254037844387076, 1.000000000000000000, 0.8660254037844387076, 1.000000000000000000, 0.8660254037844387076, 1.000000000000000000, 0.8660254037844387076, 1.000000000000000000, 0.8660254037844387076, 1.000000000000000000, 0.8660254037844387076, 1.000000000000000000, 0.8660254037844387076, 1.000000000000000000, 0.8660254037844387076, 1.000000000000000000, 0.8660254037844387076, 1.000000000000000000, 0.8660254037844387076, 1.000000000000000000, 0.8660254037844387076, 1.000000000000000000, 0.8660254037844387076, 1.000000000000000000, 0.8660254037844387076, 1.000000000000000000, 0.8660254037844387076, 1.000000000000000000, 0.8660254037844387076, 1.000000000000000000, 0.8660254037844387076, 1.000000000000000000, 0.8660254037844387076, 1.000000000000000000, 0.8660254037844387076, 1.000000000000000000, 0.8660254037844387076, 1.000000000000000000, 0.8660254037844387076, 1.000000000000000000, 0.8660254037844387076, 1.000000000000000000, 0.8660254037844387076, 1.000000000000000000, 0.8660254037844387076, 1.000000000000000000, 0.8660254037844387076, 1.000000000000000000, 0.8660254037844387076, 1.000000000000000000, 0.8660254037844387076, 1.000000000000000000, 0.8660254037844387076, 1.000000000000000000, 0.8660254037844387076, 1.000000000000000000, 0.8660254037844387076, 1.000000000000000000, 0.8660254037844387076, 1.000000000000000000, 0.8660254037844387076, 1.000000000000000000, 0.8660254037844387076, 1.000000000000000000, 0.8660254037844387076, 1.000000000000000000, 0.8660254037844387076, 1.000000000000000000, 0.8660254037844387076, 1.000000000000000000, 0.8660254037844387076, 1.000000000000000000, 0.8660254037844387076, 1.000000000000000000, 0.8660254037844387076, 1.000000000000000000, 0.8660254037844387076, 1.000000000000000000, 0.8660254037844387076, 1.000000000000000000, 0.8660254037844387076, 1.000000000000000000, 0.8660254037844387076, 1.000000000000000000, 0.8660254037844387076, 1.000000000000000000, 0.8660254037844387076, 1.000000000000000000, 0.8660254037844387076, 1.000000000000000000, 0.8660254037844387076, 1.000000000000000000, 0.8660254037844387076, 1.000000000000000000, 0.8660254037844387076, 1.000000000000000000, 0.8660254037844387076, 1.000000000000000000, 0.8660254037844387076, 1.000000000000000000, 0.8660254037844387076, 1.000000000000000000, 0.8660254037844387076, 1.000000000000000000, 0.8660254037844387076, 1.000000000000000000, 0.8660254037844387076, 1.000000000000000000, 0.8660254037844387076, 1.000000000000000000, 0.8660254037844387076, 1.000000000000000000, 0.8660254037844387076, 1.000000000000000000, 0.8660254037844387076, 1.000000000000000000, 0.8660254037844387076, 1.000000000000000000, 0.8660254037844387076, 1.000000000000000000, 0.8660254037844387076, 1.000000000000000000, 0.8660254037844387076, 1.000000000000000000, 0.8660254037844387076, 1.000000000000000000, 0.8660254037844387076, 1.000000000000000000, 0.8660254037844387076, 1.000000000000000000, 0.8660254037844387076, 1.000000000000000000, 0.8660254037844387076, 1.000000000000000000, 0.8660254037844387076, 1.000000000000000000, 0.9024573129378067327, 0.9469501470576184854) ) ) 
 REPRESENTATION_ITEM ( '' )  SURFACE ( )  );
#58454=CARTESIAN_POINT ( 'NONE',  ( 97.30629616937498838, 91.33154071421968467, 80.64697916753382856 ) ) ;
#58459=CARTESIAN_POINT ( 'NONE',  ( 94.99999999999998579, 90.00000000000002842, 90.00000000000000000 ) ) ;
#58462=DIRECTION ( 'NONE',  ( 0.8571673007021122226, 0.000000000000000000, 0.5150380749100542666 ) ) ;
#58472=AXIS2_PLACEMENT_3D ( 'NONE', #24471, #2323, #42504 ) ;
#58474=CARTESIAN_POINT ( 'NONE',  ( -97.65000000000003411, -208.4700217866474929, 75.97708333333333997 ) ) ;
#58475=CARTESIAN_POINT ( 'NONE',  ( -97.30629616937497417, -211.3315407142195852, 77.15447916753382174 ) ) ;
#58478=EDGE_CURVE ( 'NONE', #40782, #70651, #34459, .T. ) ;
#58481=LINE ( 'NONE', #1390, #2250 ) ;
#58482=DIRECTION ( 'NONE',  ( -0.000000000000000000, -0.000000000000000000, 1.000000000000000000 ) ) ;
#58484=LINE ( 'NONE', #6978, #31237 ) ;
#58490=EDGE_CURVE ( 'NONE', #44844, #11817, #57403, .T. ) ;
#58491=CARTESIAN_POINT ( 'NONE',  ( 92.69370383062498320, 90.00000000000002842, 87.89656250086714806 ) ) ;
#58492=CARTESIAN_POINT ( 'NONE',  ( -94.99999999999997158, -207.3369185715606307, 87.10281250086715943 ) ) ;
#58495=CARTESIAN_POINT ( 'NONE',  ( -93.67500000000003979, 92.29496732002878900, 81.53333333333333144 ) ) ;
#58496=CARTESIAN_POINT ( 'NONE',  ( -96.32499999999996021, -212.2949673200287179, 82.48583333333333201 ) ) ;
#58497=CARTESIAN_POINT ( 'NONE',  ( -97.30629616937501680, 88.66845928578038638, 76.99572916753380980 ) ) ;
#58499=CARTESIAN_POINT ( 'NONE',  ( 93.84685191531251292, -211.9973110713294489, 87.84364583420047268 ) ) ;
#58504=AXIS2_PLACEMENT_3D ( 'NONE', #70199, #2938, #30720 ) ;
#58508=DIRECTION ( 'NONE',  ( -0.000000000000000000, -0.000000000000000000, 1.000000000000000000 ) ) ;
#58514=CARTESIAN_POINT ( 'NONE',  ( 93.84685191531251292, -211.9973110713294489, 82.28739583420048120 ) ) ;
#58516=DIRECTION ( 'NONE',  ( -1.000000000000000000, -1.343011723336883198E-16, -0.000000000000000000 ) ) ;
#58520=CARTESIAN_POINT ( 'NONE',  ( 95.00000000000000000, -213.0599564267049857, 84.44375000000000853 ) ) ;
#58523=VERTEX_POINT ( 'NONE', #62317 ) ;
#58528=CARTESIAN_POINT ( 'NONE',  ( -97.30629616937501680, 91.33154071421968467, 86.57364583420047666 ) ) ;
#58531=CARTESIAN_POINT ( 'NONE',  ( 92.69370383062501162, -208.6684592857803011, 88.31989583420046586 ) ) ;
#58532=CARTESIAN_POINT ( 'NONE',  ( 93.67499999999998295, 92.29496732002878900, 79.73416666666666686 ) ) ;
#58535=CARTESIAN_POINT ( 'NONE',  ( -92.34999999999999432, -209.9999999999999716, 87.85687500173429498 ) ) ;
#58536=ORIENTED_EDGE ( 'NONE', *, *, #10429, .F. ) ;
#58538=VERTEX_POINT ( 'NONE', #669 ) ;
#58539=CARTESIAN_POINT ( 'NONE',  ( -95.00000000000002842, 86.94004357329504273, 87.69812500173429726 ) ) ;
#58540=CARTESIAN_POINT ( 'NONE',  ( 96.15314808468748708, 91.99731107132950569, 76.09614583420047040 ) ) ;
#58545=EDGE_CURVE ( 'NONE', #69481, #7050, #67895, .T. ) ;
#58546=CYLINDRICAL_SURFACE ( 'NONE', #58727, 2.649999999999985700 ) ;
#58548=CARTESIAN_POINT ( 'NONE',  ( -92.35000000045957336, 90.00004935162611730, 87.22187670868784437 ) ) ;
#58559=CARTESIAN_POINT ( 'NONE',  ( -94.99999999999997158, -212.6630814284392557, 86.78531250086716398 ) ) ;
#58563=VERTEX_POINT ( 'NONE', #15996 ) ;
#58565=ORIENTED_EDGE ( 'NONE', *, *, #16114, .T. ) ;
#58570=CARTESIAN_POINT ( 'NONE',  ( 94.99999999999998579, 87.33691857156068750, 80.27656250086714351 ) ) ;
#58571=AXIS2_PLACEMENT_3D ( 'NONE', #9110, #8378, #55343 ) ;
#58579=DIRECTION ( 'NONE',  ( -0.000000000000000000, -0.000000000000000000, 1.000000000000000000 ) ) ;
#58580=CARTESIAN_POINT ( 'NONE',  ( 95.00000000000000000, -206.9400435732949575, 85.47562500173430067 ) ) ;
#58582=CARTESIAN_POINT ( 'NONE',  ( -96.15314808468752972, 91.99731107132950569, 85.09197916753380753 ) ) ;
#58583=EDGE_CURVE ( 'NONE', #58994, #29135, #5115, .T. ) ;
#58585=CARTESIAN_POINT ( 'NONE',  ( -92.35000000018069954, 89.99996905681452120, 78.33187387208522523 ) ) ;
#58597=CARTESIAN_POINT ( 'NONE',  ( 97.30629616937498838, -208.6684592857803011, 81.28197916753381946 ) ) ;
#58598=ORIENTED_EDGE ( 'NONE', *, *, #331, .T. ) ;
#58603=CARTESIAN_POINT ( 'NONE',  ( 92.69370383062501162, -208.6684592857803295, 75.61989583420047722 ) ) ;
#58605=VERTEX_POINT ( 'NONE', #34031 ) ;
#58606=CARTESIAN_POINT ( 'NONE',  ( 92.69370383062501162, -208.6684592857803011, 80.22364583420048234 ) ) ;
#58618=CARTESIAN_POINT ( 'NONE',  ( -95.00000000000002842, 93.05995642670504253, 84.12624999999999886 ) ) ;
#58619=CARTESIAN_POINT ( 'NONE',  ( 95.00000000000000000, -213.0599564267049857, 83.88812500173429498 ) ) ;
#58620=CARTESIAN_POINT ( 'NONE',  ( 93.67499999999998295, 92.29496732002878900, 89.89416666666666345 ) ) ;
#58622=CARTESIAN_POINT ( 'NONE',  ( 97.64999999999999147, 89.99999988321010846, 84.68187499741277691 ) ) ;
#58628=CARTESIAN_POINT ( 'NONE',  ( 96.32499999999997442, 92.29496732002878900, 87.32770833506762642 ) ) ;
#58633=CARTESIAN_POINT ( 'NONE',  ( -96.32499999999996021, -212.2949673200287179, 78.12020833506763040 ) ) ;
#58636=AXIS2_PLACEMENT_3D ( 'NONE', #20709, #3447, #61317 ) ;
#58646=CARTESIAN_POINT ( 'NONE',  ( -95.00000000000002842, 86.94004357329504273, 87.61875000000000568 ) ) ;
#58647=ORIENTED_EDGE ( 'NONE', *, *, #35787, .F. ) ;
#58653=CARTESIAN_POINT ( 'NONE',  ( -92.69370383062498320, -209.9999999999999716, 82.97531250086714749 ) ) ;
#58665=CARTESIAN_POINT ( 'NONE',  ( 93.67499999999999716, 87.70503267997126784, 88.20083333333332121 ) ) ;
#58667=CARTESIAN_POINT ( 'NONE',  ( -93.84685191531254134, 91.99731107132950569, 79.27114583420046756 ) ) ;
#58669=LINE ( 'NONE', #63219, #9835 ) ;
#58670=( BOUNDED_CURVE ( )  B_SPLINE_CURVE ( 2, ( #31931, #37225, #54870, #49958, #42491, #43248, #13893 ),
 .UNSPECIFIED., .F., .F. ) 
 B_SPLINE_CURVE_WITH_KNOTS ( ( 3, 2, 2, 3 ),
 ( 0.2708333333333337034, 0.2777777777777781232, 0.2847222222222224874, 0.2916666666666669072 ),
 .UNSPECIFIED. ) 
 CURVE ( )  GEOMETRIC_REPRESENTATION_ITEM ( )  RATIONAL_B_SPLINE_CURVE ( ( 0.9999999999999924505, 0.8660254037844462571, 1.000000000000000000, 0.8660254037844387076, 1.000000000000000000, 0.8660254037844343777, 1.000000000000004219 ) ) 
 REPRESENTATION_ITEM ( '' )  );
#58683=CARTESIAN_POINT ( 'NONE',  ( -92.69370383062498320, -208.6684592857803011, 76.83697916753382628 ) ) ;
#58697=CARTESIAN_POINT ( 'NONE',  ( 92.34999999999999432, 90.00000000000002842, 86.18999999999999773 ) ) ;
#58701=CARTESIAN_POINT ( 'NONE',  ( 97.30629616937498838, -209.9999999999999716, 84.24531250086714351 ) ) ;
#58702=CARTESIAN_POINT ( 'NONE',  ( 92.69370383062501162, -209.9999999999999716, 87.26156250086715715 ) ) ;
#58704=CARTESIAN_POINT ( 'NONE',  ( 96.15314808468748708, -208.0026889286704943, 88.31989583420048007 ) ) ;
#58708=CARTESIAN_POINT ( 'NONE',  ( -95.00000000000002842, 92.66308142843932671, 81.38781250086715602 ) ) ;
#58720=EDGE_CURVE ( 'NONE', #64725, #1126, #50078, .T. ) ;
#58725=CIRCLE ( 'NONE', #32242, 15.69999999999999929 ) ;
#58726=EDGE_CURVE ( 'NONE', #47064, #11565, #11502, .T. ) ;
#58727=AXIS2_PLACEMENT_3D ( 'NONE', #24344, #7044, #70183 ) ;
#58730=CARTESIAN_POINT ( 'NONE',  ( 95.00000000000000000, -207.3369185715606307, 81.22906250086715829 ) ) ;
#58735=DIRECTION ( 'NONE',  ( -0.8571673007021122226, 1.049727191138618572E-16, 0.5150380749100542666 ) ) ;
#58736=CARTESIAN_POINT ( 'NONE',  ( 96.32499999999998863, -207.7050326799711968, 78.99333333333332519 ) ) ;
#58742=CARTESIAN_POINT ( 'NONE',  ( -96.15314808468747287, -208.0026889286704943, 84.45697916753380241 ) ) ;
#58743=CARTESIAN_POINT ( 'NONE',  ( -97.30629616937501680, 88.66845928578038638, 82.23447916753383424 ) ) ;
#58744=ORIENTED_EDGE ( 'NONE', *, *, #13557, .F. ) ;
#58745=CARTESIAN_POINT ( 'NONE',  ( 96.15314808468748708, 88.00268892867053694, 79.69447916753379957 ) ) ;
#58746=ORIENTED_EDGE ( 'NONE', *, *, #70578, .F. ) ;
#58747=CARTESIAN_POINT ( 'NONE',  ( 95.00000000000000000, -209.9999999999999716, 90.00000000000000000 ) ) ;
#58754=CARTESIAN_POINT ( 'NONE',  ( -92.69370383062498320, -209.9999999999999716, 84.88031250086713442 ) ) ;
#58765=EDGE_CURVE ( 'NONE', #21866, #45116, #37151, .T. ) ;
#58774=DIRECTION ( 'NONE',  ( 1.000000000000000000, 0.000000000000000000, 0.000000000000000000 ) ) ;
#58779=CARTESIAN_POINT ( 'NONE',  ( -93.84685191531247028, -211.9973110713294489, 85.56822916753381492 ) ) ;
#58784=CARTESIAN_POINT ( 'NONE',  ( -92.69370383062498320, -209.9999999999999716, 74.87906250086714977 ) ) ;
#58790=CARTESIAN_POINT ( 'NONE',  ( 94.99999999999998579, 93.05995642670504253, 85.47562500173430067 ) ) ;
#58792=CARTESIAN_POINT ( 'NONE',  ( -96.15314808468751551, 88.00268892867056536, 76.57239583420049200 ) ) ;
#58793=CARTESIAN_POINT ( 'NONE',  ( 92.69370383062501162, -208.6684592857803011, 75.61989583420047722 ) ) ;
#58795=EDGE_CURVE ( 'NONE', #29381, #66094, #44838, .T. ) ;
#58802=VECTOR ( 'NONE', #63383, 1000.000000000000000 ) ;
#58806=AXIS2_PLACEMENT_3D ( 'NONE', #15155, #55384, #49368 ) ;
#58810=EDGE_CURVE ( 'NONE', #30842, #43302, #57338, .T. ) ;
#58813=CARTESIAN_POINT ( 'NONE',  ( 94.99999999999998579, 87.33691857156068750, 78.53031250086715431 ) ) ;
#58827=DIRECTION ( 'NONE',  ( -1.000000000000000000, 0.000000000000000000, 0.000000000000000000 ) ) ;
#58830=CARTESIAN_POINT ( 'NONE',  ( -94.99999999999997158, -213.0599564267049857, 80.71312500173431204 ) ) ;
#58833=CARTESIAN_POINT ( 'NONE',  ( 92.34999999999999432, 91.52997821335252127, 76.05645833506761733 ) ) ;
#58834=CARTESIAN_POINT ( 'NONE',  ( -93.67500000000003979, 87.70503267997129626, 76.32104166840096582 ) ) ;
#58836=ORIENTED_EDGE ( 'NONE', *, *, #4241, .F. ) ;
#58837=CARTESIAN_POINT ( 'NONE',  ( 96.15314808468748708, 91.99731107132950569, 81.33489583420049485 ) ) ;
#58855=CARTESIAN_POINT ( 'NONE',  ( 97.64999999999999147, -209.9999999999999716, 90.00000000000000000 ) ) ;
#58857=CARTESIAN_POINT ( 'NONE',  ( -92.69370383062498320, -208.6684592857803011, 77.47197916753381719 ) ) ;
#58858=EDGE_CURVE ( 'NONE', #18340, #61621, #39124, .T. ) ;
#58865=DIRECTION ( 'NONE',  ( 1.000000000000000000, 0.000000000000000000, 0.000000000000000000 ) ) ;
#58872=FACE_OUTER_BOUND ( 'NONE', #35764, .T. ) ;
#58874=CARTESIAN_POINT ( 'NONE',  ( -92.34999999999999432, -209.9999999999999716, 76.34749999999999659 ) ) ;
#58876=CARTESIAN_POINT ( 'NONE',  ( 97.30629616937498838, 90.00000000000002842, 82.49906250086715431 ) ) ;
#58877=CARTESIAN_POINT ( 'NONE',  ( -97.30629616937497417, -211.3315407142195852, 86.04447916753382231 ) ) ;
#58881=CARTESIAN_POINT ( 'NONE',  ( -93.67499999999998295, -207.7050326799711968, 82.80333333333332746 ) ) ;
#58882=CARTESIAN_POINT ( 'NONE',  ( -93.84685191531254134, 91.99731107132950569, 76.73114583420047552 ) ) ;
#58884=CARTESIAN_POINT ( 'NONE',  ( 92.69370383062501162, -211.3315407142195852, 87.79072916753381151 ) ) ;
#58899=CARTESIAN_POINT ( 'NONE',  ( 92.69370383062501162, -209.9999999999999716, 80.91156250086716284 ) ) ;
#58901=CYLINDRICAL_SURFACE ( 'NONE', #6421, 2.649999999999999467 ) ;
#58903=( BOUNDED_CURVE ( )  B_SPLINE_CURVE ( 2, ( #28140, #69122, #16497, #62382, #10859, #51076, #68389 ),
 .UNSPECIFIED., .F., .F. ) 
 B_SPLINE_CURVE_WITH_KNOTS ( ( 3, 2, 2, 3 ),
 ( 0.8541666666666666297, 0.8611111111111110494, 0.8680555555555554692, 0.8749999999999997780 ),
 .UNSPECIFIED. ) 
 CURVE ( )  GEOMETRIC_REPRESENTATION_ITEM ( )  RATIONAL_B_SPLINE_CURVE ( ( 1.000000000000000000, 0.8660254037844387076, 1.000000000000000000, 0.8660254037844387076, 1.000000000000000000, 0.8660254037844430375, 0.9999999999999956701 ) ) 
 REPRESENTATION_ITEM ( '' )  );
#58906=CARTESIAN_POINT ( 'NONE',  ( 93.67500000000001137, -212.2949673200287179, 84.39083333333333314 ) ) ;
#58911=ORIENTED_EDGE ( 'NONE', *, *, #72797, .F. ) ;
#58916=CARTESIAN_POINT ( 'NONE',  ( -97.30629616937501680, 90.00000000000004263, 86.62656250086715204 ) ) ;
#58917=DIRECTION ( 'NONE',  ( 0.000000000000000000, -0.000000000000000000, -1.000000000000000000 ) ) ;
#58920=CARTESIAN_POINT ( 'NONE',  ( 92.69370383062501162, -211.3315407142195852, 88.42572916753380241 ) ) ;
#58921=CARTESIAN_POINT ( 'NONE',  ( 96.32499999999998863, 87.70503267997126784, 80.05166666666666231 ) ) ;
#58922=ORIENTED_EDGE ( 'NONE', *, *, #61870, .T. ) ;
#58923=CARTESIAN_POINT ( 'NONE',  ( -94.99999999999997158, -206.9400435732949575, 88.65062500173431204 ) ) ;
#58928=CARTESIAN_POINT ( 'NONE',  ( -96.32500000000001705, 92.29496732002878900, 84.89354166840095672 ) ) ;
#58929=CARTESIAN_POINT ( 'NONE',  ( 97.30629616937498838, 90.00000000000002842, 76.62531250086713897 ) ) ;
#58931=ORIENTED_EDGE ( 'NONE', *, *, #73385, .F. ) ;
#58939=CARTESIAN_POINT ( 'NONE',  ( -92.69370383062499741, -210.9303163890424173, 74.68334086212730938 ) ) ;
#58946=CARTESIAN_POINT ( 'NONE',  ( -94.99999999999997158, -207.3369185715606307, 87.10281250086715943 ) ) ;
#58948=CARTESIAN_POINT ( 'NONE',  ( -93.67499999999998295, -212.2949673200287179, 82.59166666666665435 ) ) ;
#58955=CARTESIAN_POINT ( 'NONE',  ( 92.69370383062498320, 91.33154071421968467, 89.11364583420049712 ) ) ;
#58956=DIRECTION ( 'NONE',  ( -0.000000000000000000, -0.000000000000000000, 1.000000000000000000 ) ) ;
#58957=CARTESIAN_POINT ( 'NONE',  ( 97.30629616937498838, 88.66845928578035796, 80.38239583420049428 ) ) ;
#58968=CARTESIAN_POINT ( 'NONE',  ( -96.15314808468751551, 88.00268892867056536, 85.30364583420046642 ) ) ;
#58981=CARTESIAN_POINT ( 'NONE',  ( 95.00000000000000000, -207.3369185715606307, 83.29281250086717137 ) ) ;
#58988=CARTESIAN_POINT ( 'NONE',  ( -97.64999999999996305, -209.9999999999999716, 88.09499999999999886 ) ) ;
#58990=CARTESIAN_POINT ( 'NONE',  ( 97.30629616937498838, -211.3315407142195852, 75.93739583420050110 ) ) ;
#58992=CARTESIAN_POINT ( 'NONE',  ( 96.15314808468748708, -208.0026889286704943, 79.42989583420049371 ) ) ;
#58994=VERTEX_POINT ( 'NONE', #7683 ) ;
#59003=CARTESIAN_POINT ( 'NONE',  ( 96.32499999999998863, -207.7050326799711968, 82.24770833506762813 ) ) ;
#59004=CARTESIAN_POINT ( 'NONE',  ( 92.34999999999999432, 90.00000000000002842, 88.09499999999999886 ) ) ;
#59011=CARTESIAN_POINT ( 'NONE',  ( -96.15314808468751551, 88.00268892867056536, 86.73239583420048859 ) ) ;
#59012=CARTESIAN_POINT ( 'NONE',  ( 93.84685191531248449, 91.99731107132950569, 84.45697916753380241 ) ) ;
#59015=CARTESIAN_POINT ( 'NONE',  ( 93.67499999999998295, 92.29496732002878900, 87.43354166840096298 ) ) ;
#59022=CARTESIAN_POINT ( 'NONE',  ( -93.67499999999998295, -207.7050326799711968, 75.18333333333332291 ) ) ;
#59026=EDGE_LOOP ( 'NONE', ( #10824, #68883, #21503, #32343 ) ) ;
#59030=CARTESIAN_POINT ( 'NONE',  ( -95.00000000000002842, 93.05995642670501411, 85.39624999999998067 ) ) ;
#59033=CARTESIAN_POINT ( 'NONE',  ( 97.30629616937500259, 90.00000000000002842, 74.79348190356851944 ) ) ;
#59034=CYLINDRICAL_SURFACE ( 'NONE', #56340, 2.649999999999985700 ) ;
#59037=CARTESIAN_POINT ( 'NONE',  ( -97.30629616937495996, -209.9999999999999716, 81.38781250086714181 ) ) ;
#59042=CARTESIAN_POINT ( 'NONE',  ( 7.103376864691351012E-17, -120.0000000000000000, -90.00000000000000000 ) ) ;
#59049=CARTESIAN_POINT ( 'NONE',  ( -93.84685191531254134, 91.99731107132950569, 89.58989583420049030 ) ) ;
#59060=CARTESIAN_POINT ( 'NONE',  ( -96.15314808468745866, -211.9973110713294489, 75.30239583420048177 ) ) ;
#59064=VECTOR ( 'NONE', #54376, 1000.000000000000000 ) ;
#59070=VECTOR ( 'NONE', #39528, 1000.000000000000000 ) ;
#59075=ORIENTED_EDGE ( 'NONE', *, *, #7974, .T. ) ;
#59080=CARTESIAN_POINT ( 'NONE',  ( 95.00000000000000000, -207.3369185715606307, 85.67406250086715147 ) ) ;
#59081=CARTESIAN_POINT ( 'NONE',  ( 93.84685191531249870, -208.0026889286704943, 89.69572916753382685 ) ) ;
#59082=ORIENTED_EDGE ( 'NONE', *, *, #65104, .T. ) ;
#59083=CARTESIAN_POINT ( 'NONE',  ( 93.84685191531251292, -211.9973110713294489, 89.27239583420049485 ) ) ;
#59087=CARTESIAN_POINT ( 'NONE',  ( -92.69370383062502583, 88.66845928578038638, 81.17614583420048291 ) ) ;
#59092=CARTESIAN_POINT ( 'NONE',  ( 97.65000000000000568, -208.4700217866474645, 84.73479166840094479 ) ) ;
#59094=EDGE_CURVE ( 'NONE', #19675, #32344, #49380, .T. ) ;
#59101=VECTOR ( 'NONE', #8077, 1000.000000000000000 ) ;
#59104=CARTESIAN_POINT ( 'NONE',  ( 97.30629616937498838, -209.9999999999999716, 77.26031250086714408 ) ) ;
#59112=CARTESIAN_POINT ( 'NONE',  ( -97.64999999999996305, -209.9999999999999716, 75.39499999999999602 ) ) ;
#59115=CARTESIAN_POINT ( 'NONE',  ( -92.69370383062498320, -208.6684592857803011, 84.29822916753380468 ) ) ;
#59116=CARTESIAN_POINT ( 'NONE',  ( -95.00000000000002842, 92.66308142843932671, 82.02281250086714692 ) ) ;
#59118=CARTESIAN_POINT ( 'NONE',  ( 93.84685191531248449, 91.99731107132950569, 80.01197916753380923 ) ) ;
#59120=( BOUNDED_CURVE ( )  B_SPLINE_CURVE ( 2, ( #10805, #51383, #50643, #67949, #68700, #5554, #67202 ),
 .UNSPECIFIED., .F., .F. ) 
 B_SPLINE_CURVE_WITH_KNOTS ( ( 3, 2, 2, 3 ),
 ( 0.3333333333333333703, 0.3402777777777777901, 0.3472222222222221544, 0.3541666666666665741 ),
 .UNSPECIFIED. ) 
 CURVE ( )  GEOMETRIC_REPRESENTATION_ITEM ( )  RATIONAL_B_SPLINE_CURVE ( ( 0.9999999999999988898, 0.8660254037844398178, 1.000000000000000000, 0.8660254037844387076, 1.000000000000000000, 0.8660254037844408170, 0.9999999999999978906 ) ) 
 REPRESENTATION_ITEM ( '' )  );
#59127=CARTESIAN_POINT ( 'NONE',  ( -92.69370383062498320, -211.3315407142195852, 84.19239583420048234 ) ) ;
#59133=ORIENTED_EDGE ( 'NONE', *, *, #577, .T. ) ;
#59134=CARTESIAN_POINT ( 'NONE',  ( -93.09170270117418511, 88.16127723152901297, 74.99909419456534465 ) ) ;
#59136=CARTESIAN_POINT ( 'NONE',  ( -93.84685191531254134, 91.99731107132950569, 89.43114583420047836 ) ) ;
#59147=CARTESIAN_POINT ( 'NONE',  ( -93.84685191531248449, -208.0026889286704943, 85.77989583420048803 ) ) ;
#59152=ADVANCED_FACE ( 'NONE', ( #61036 ), #9899, .F. ) ;
#59153=CARTESIAN_POINT ( 'NONE',  ( -92.69370383062498320, -211.3315407142195852, 76.73114583420048973 ) ) ;
#59158=DIRECTION ( 'NONE',  ( -0.000000000000000000, -0.000000000000000000, 1.000000000000000000 ) ) ;
#59159=CARTESIAN_POINT ( 'NONE',  ( -97.30629616937495996, -209.9999999999999716, 89.80156250086714920 ) ) ;
#59162=CARTESIAN_POINT ( 'NONE',  ( 96.15314808468748708, -208.0026889286704943, 76.73114583420047552 ) ) ;
#59178=CARTESIAN_POINT ( 'NONE',  ( -92.35000000000003695, 90.00000000000004263, 90.00000000000000000 ) ) ;
#59183=CARTESIAN_POINT ( 'NONE',  ( 94.99999999999998579, 92.66308142843935514, 81.38781250086715602 ) ) ;
#59185=CARTESIAN_POINT ( 'NONE',  ( 92.35000000000000853, -209.9999999999999716, 75.39499999999999602 ) ) ;
#59198=CARTESIAN_POINT ( 'NONE',  ( -97.64999999999994884, -208.4700217866474645, 77.96145833506763267 ) ) ;
#59200=CARTESIAN_POINT ( 'NONE',  ( 93.84685191531248449, 91.99731107132950569, 89.53697916753381492 ) ) ;
#59201=CARTESIAN_POINT ( 'NONE',  ( -96.32500000000001705, 92.29496732002878900, 74.73354166840096013 ) ) ;
#59203=CARTESIAN_POINT ( 'NONE',  ( 93.84685191531248449, 91.99731107132950569, 76.36072916753381890 ) ) ;
#59205=FACE_OUTER_BOUND ( 'NONE', #67996, .T. ) ;
#59207=CARTESIAN_POINT ( 'NONE',  ( 92.35004024445041182, -211.5300014484966766, 77.43229327564786502 ) ) ;
#59213=ORIENTED_EDGE ( 'NONE', *, *, #54318, .T. ) ;
#59218=CARTESIAN_POINT ( 'NONE',  ( -92.35000000005462084, -210.0000170173125014, 88.49187441316038871 ) ) ;
#59221=CARTESIAN_POINT ( 'NONE',  ( -94.99999999999997158, -207.3369185715606307, 77.57781250086715374 ) ) ;
#59224=ADVANCED_FACE ( 'NONE', ( #55769 ), #27174, .F. ) ;
#59226=DIRECTION ( 'NONE',  ( -0.000000000000000000, -0.000000000000000000, 1.000000000000000000 ) ) ;
#59233=CARTESIAN_POINT ( 'NONE',  ( -2.500000000000015543, -73.00000000000001421, -201.6999999999999886 ) ) ;
#59234=EDGE_CURVE ( 'NONE', #6682, #27925, #54924, .T. ) ;
#59237=PLANE ( 'NONE',  #34018 ) ;
#59240=CARTESIAN_POINT ( 'NONE',  ( 93.84685191531248449, 88.00268892867053694, 83.55739583420049144 ) ) ;
#59242=CARTESIAN_POINT ( 'NONE',  ( -94.99999999999997158, -207.3369185715606307, 85.83281250086717762 ) ) ;
#59245=CARTESIAN_POINT ( 'NONE',  ( -97.65000000000001990, 90.00000000000004263, 81.74500000000000455 ) ) ;
#59246=CARTESIAN_POINT ( 'NONE',  ( -96.32499999999996021, -207.7050326799711968, 79.73416666666666686 ) ) ;
#59247=CARTESIAN_POINT ( 'NONE',  ( -97.30629616937501680, 90.00000000000004263, 77.57781250086713953 ) ) ;
#59248=CARTESIAN_POINT ( 'NONE',  ( 93.84685191531251292, -211.9973110713294489, 85.93864583420048575 ) ) ;
#59250=VECTOR ( 'NONE', #16801, 1000.000000000000000 ) ;
#59260=CARTESIAN_POINT ( 'NONE',  ( 95.00000000000000000, -207.3369185715606307, 81.38781250086715602 ) ) ;
#59268=EDGE_CURVE ( 'NONE', #32344, #66338, #24206, .T. ) ;
#59271=CARTESIAN_POINT ( 'NONE',  ( 92.35000000000000853, -209.9999999999999716, 84.28499999999999659 ) ) ;
#59278=AXIS2_PLACEMENT_3D ( 'NONE', #5900, #28060, #27310 ) ;
#59279=CARTESIAN_POINT ( 'NONE',  ( -95.00000000000002842, 87.33691857156074434, 84.88031250086714863 ) ) ;
#59282=CARTESIAN_POINT ( 'NONE',  ( 92.69370383062501162, -208.6684592857803011, 88.95489583420048518 ) ) ;
#59283=CARTESIAN_POINT ( 'NONE',  ( 97.64999999999999147, 90.00000000000002842, 76.34749999999999659 ) ) ;
#59285=CARTESIAN_POINT ( 'NONE',  ( -92.34999999999999432, -208.4700217866474645, 88.54479166840097548 ) ) ;
#59289=CARTESIAN_POINT ( 'NONE',  ( -97.65000000000001990, 91.52997821335253548, 84.94645833506763211 ) ) ;
#59290=CARTESIAN_POINT ( 'NONE',  ( 97.30629616937498838, 90.00000000000002842, 86.94406250086716170 ) ) ;
#59298=CARTESIAN_POINT ( 'NONE',  ( -97.30629616937497417, -211.3315407142195852, 75.09072916753382287 ) ) ;
#59299=ORIENTED_EDGE ( 'NONE', *, *, #4778, .T. ) ;
#59301=FACE_BOUND ( 'NONE', #10822, .T. ) ;
#59305=CARTESIAN_POINT ( 'NONE',  ( -94.99999999999997158, -212.6630814284392557, 88.69031250086716511 ) ) ;
#59314=CARTESIAN_POINT ( 'NONE',  ( 94.99999999999998579, 92.66308142843935514, 89.00781250086716057 ) ) ;
#59316=CARTESIAN_POINT ( 'NONE',  ( 93.84685191531248449, 88.00268892867053694, 80.85864583420047325 ) ) ;
#59318=FACE_OUTER_BOUND ( 'NONE', #56856, .T. ) ;
#59319=EDGE_CURVE ( 'NONE', #16870, #34217, #6730, .T. ) ;
#59325=CARTESIAN_POINT ( 'NONE',  ( 96.32499999999998863, 87.70503267997126784, 83.86166666666666458 ) ) ;
#59327=( BOUNDED_CURVE ( )  B_SPLINE_CURVE ( 2, ( #53309, #65339, #1115, #24735, #46936, #47305, #69851 ),
 .UNSPECIFIED., .F., .F. ) 
 B_SPLINE_CURVE_WITH_KNOTS ( ( 3, 2, 2, 3 ),
 ( 0.2916666666666669072, 0.2986111111111113270, 0.3055555555555557468, 0.3125000000000001665 ),
 .UNSPECIFIED. ) 
 CURVE ( )  GEOMETRIC_REPRESENTATION_ITEM ( )  RATIONAL_B_SPLINE_CURVE ( ( 0.9999999999999956701, 0.8660254037844430375, 1.000000000000000000, 0.8660254037844387076, 1.000000000000000000, 0.8660254037844354880, 1.000000000000003109 ) ) 
 REPRESENTATION_ITEM ( '' )  );
#59334=CARTESIAN_POINT ( 'NONE',  ( -93.84685191531252713, 88.00268892867056536, 84.77447916753381207 ) ) ;
#59336=DIRECTION ( 'NONE',  ( 1.000000000000000000, 0.000000000000000000, 0.000000000000000000 ) ) ;
#59340=( BOUNDED_CURVE ( )  B_SPLINE_CURVE ( 2, ( #532, #46359, #175, #23067, #41452, #17046, #6509, #57650, #62937 ),
 .UNSPECIFIED., .F., .F. ) 
 B_SPLINE_CURVE_WITH_KNOTS ( ( 3, 2, 2, 2, 3 ),
 ( 0.8678591737214820245, 0.8749149270694132063, 0.8819706926102950373, 0.8890264581511769792, 0.8890265259358470784 ),
 .UNSPECIFIED. ) 
 CURVE ( )  GEOMETRIC_REPRESENTATION_ITEM ( )  RATIONAL_B_SPLINE_CURVE ( ( 1.000000000000000000, 0.8660254037844387076, 1.000000000000000000, 0.8660254037844387076, 1.000000000000000000, 0.8660254037844387076, 1.000000000000000000, 0.9999987129073719672, 0.9999974258394741522 ) ) 
 REPRESENTATION_ITEM ( '' )  );
#59346=CARTESIAN_POINT ( 'NONE',  ( -97.64998530153626177, -208.4700133004854479, 76.05645774805350356 ) ) ;
#59347=CARTESIAN_POINT ( 'NONE',  ( 92.69370383062501162, -208.6684592857803011, 82.76364583420048859 ) ) ;
#59356=ORIENTED_EDGE ( 'NONE', *, *, #24116, .T. ) ;
#59357=CARTESIAN_POINT ( 'NONE',  ( 92.69370383062501162, -209.9999999999999716, 80.91156250086716284 ) ) ;
#59359=CARTESIAN_POINT ( 'NONE',  ( 92.35000000000003695, 88.47002178664747873, 79.25791666666667368 ) ) ;
#59360=EDGE_LOOP ( 'NONE', ( #28303, #52351, #20509, #47627 ) ) ;
#59361=EDGE_LOOP ( 'NONE', ( #1923, #59583, #64457, #71824 ) ) ;
#59362=CARTESIAN_POINT ( 'NONE',  ( -92.35000000000003695, 90.00000000000004263, 83.33250000000001023 ) ) ;
#59364=PRESENTATION_STYLE_ASSIGNMENT (( #69890 ) ) ;
#59365=CARTESIAN_POINT ( 'NONE',  ( -95.00000000000002842, 93.05995642670504253, 82.85625000000000284 ) ) ;
#59366=VERTEX_POINT ( 'NONE', #54207 ) ;
#59368=CARTESIAN_POINT ( 'NONE',  ( 96.32499999999998863, -212.2949673200287179, 83.94104166840097037 ) ) ;
#59369=CARTESIAN_POINT ( 'NONE',  ( 93.67499999999999716, 87.70503267997126784, 84.39083333333333314 ) ) ;
#59376=CARTESIAN_POINT ( 'NONE',  ( -92.69370383062504004, 90.00000000000004263, 88.21406250086714351 ) ) ;
#59378=CARTESIAN_POINT ( 'NONE',  ( 97.30629616937498838, 91.33154071421968467, 84.93322916753379559 ) ) ;
#59380=CARTESIAN_POINT ( 'NONE',  ( 97.64999999999999147, 90.00000000000002842, 85.95187500173430806 ) ) ;
#59382=ORIENTED_EDGE ( 'NONE', *, *, #25028, .F. ) ;
#59388=CARTESIAN_POINT ( 'NONE',  ( -93.26027265873601380, 91.51405112163766375, 74.79348190356853365 ) ) ;
#59389=DIRECTION ( 'NONE',  ( 1.000000000000000000, 0.000000000000000000, 0.000000000000000000 ) ) ;
#59391=CARTESIAN_POINT ( 'NONE',  ( -97.65000000000001990, 91.52997821335253548, 84.86708333333334053 ) ) ;
#59392=VERTEX_POINT ( 'NONE', #71469 ) ;
#59398=CARTESIAN_POINT ( 'NONE',  ( -93.84685191531248449, -208.0026889286704943, 83.08114583420048405 ) ) ;
#59400=LINE ( 'NONE', #71764, #41072 ) ;
#59406=EDGE_CURVE ( 'NONE', #14986, #6029, #16064, .T. ) ;
#59407=CARTESIAN_POINT ( 'NONE',  ( -92.35000000000003695, 90.00000000000004263, 79.52249999999999375 ) ) ;
#59408=CARTESIAN_POINT ( 'NONE',  ( 97.64999999999999147, 90.00000000000002842, 89.04749999999999943 ) ) ;
#59409=CARTESIAN_POINT ( 'NONE',  ( 96.76339072695076027, -211.4937631030103375, 74.79348190356849102 ) ) ;
#59412=DIRECTION ( 'NONE',  ( 1.000000000000000000, 0.000000000000000000, 0.000000000000000000 ) ) ;
#59413=CARTESIAN_POINT ( 'NONE',  ( -97.30629616937501680, 91.33154071421968467, 74.98489583420048632 ) ) ;
#59417=EDGE_CURVE ( 'NONE', #51295, #32186, #1632, .T. ) ;
#59418=CARTESIAN_POINT ( 'NONE',  ( 92.34999999999999432, 90.00000000000002842, 90.00000000000000000 ) ) ;
#59424=CARTESIAN_POINT ( 'NONE',  ( -97.64999999999996305, -209.9999999999999716, 86.82500000000000284 ) ) ;
#59426=EDGE_CURVE ( 'NONE', #53644, #45497, #53822, .T. ) ;
#59429=CARTESIAN_POINT ( 'NONE',  ( -92.34999999999999432, -209.9999999999999716, 90.00000000000000000 ) ) ;
#59430=EDGE_CURVE ( 'NONE', #58523, #62043, #46821, .T. ) ;
#59444=CARTESIAN_POINT ( 'NONE',  ( 97.30629616937498838, -209.9999999999999716, 84.88031250086713442 ) ) ;
#59445=CARTESIAN_POINT ( 'NONE',  ( 92.69370383062501162, -209.9999999999999716, 88.53156250086716739 ) ) ;
#59446=ORIENTED_EDGE ( 'NONE', *, *, #36143, .F. ) ;
#59453=CARTESIAN_POINT ( 'NONE',  ( -97.30629616937501680, 90.00000000000004263, 80.27656250086714351 ) ) ;
#59456=ORIENTED_EDGE ( 'NONE', *, *, #1490, .F. ) ;
#59460=CARTESIAN_POINT ( 'NONE',  ( 95.00000000000000000, -213.0599564267049857, 79.36374999999996760 ) ) ;
#59462=DIRECTION ( 'NONE',  ( -0.000000000000000000, -0.000000000000000000, 1.000000000000000000 ) ) ;
#59465=LINE ( 'NONE', #7948, #1274 ) ;
#59468=ORIENTED_EDGE ( 'NONE', *, *, #38685, .F. ) ;
#59469=CARTESIAN_POINT ( 'NONE',  ( 92.69370383062501162, -209.9999999999999716, 76.94281250086713442 ) ) ;
#59477=CARTESIAN_POINT ( 'NONE',  ( -92.34999999999999432, -210.0000085086564070, 88.49187470744925577 ) ) ;
#59479=CARTESIAN_POINT ( 'NONE',  ( -93.84685191531247028, -211.9973110713294489, 80.96447916753380980 ) ) ;
#59480=CARTESIAN_POINT ( 'NONE',  ( -96.15314808468752972, 91.99731107132950569, 77.63072916753381492 ) ) ;
#59482=CARTESIAN_POINT ( 'NONE',  ( 94.99999999999998579, 92.66308142843935514, 81.22906250086715829 ) ) ;
#59486=CARTESIAN_POINT ( 'NONE',  ( -92.35000000010064980, -209.9999769027738239, 83.41187580057901130 ) ) ;
#59487=AXIS2_PLACEMENT_3D ( 'NONE', #20465, #37010, #59964 ) ;
#59490=CARTESIAN_POINT ( 'NONE',  ( -96.15314808468745866, -211.9973110713294489, 84.66864583420047552 ) ) ;
#59503=CARTESIAN_POINT ( 'NONE',  ( -97.65000000000001990, 90.00000000000004263, 76.03000000000000114 ) ) ;
#59505=CARTESIAN_POINT ( 'NONE',  ( -96.15314808468751551, 88.00268892867056536, 84.03364583420047040 ) ) ;
#59512=CARTESIAN_POINT ( 'NONE',  ( -92.69370383062502583, 88.66845928578038638, 76.57239583420046358 ) ) ;
#59519=ADVANCED_FACE ( 'NONE', ( #65853 ), #31258, .F. ) ;
#59520=CARTESIAN_POINT ( 'NONE',  ( 97.64999999999999147, -209.9999999999999716, 82.69749999999999091 ) ) ;
#59521=CARTESIAN_POINT ( 'NONE',  ( -97.30629616937497417, -208.6684592857803011, 83.39864583420050792 ) ) ;
#59523=EDGE_CURVE ( 'NONE', #9512, #44823, #21833, .T. ) ;
#59526=CARTESIAN_POINT ( 'NONE',  ( -92.69370383062498320, -208.6684592857803295, 78.10697916753383652 ) ) ;
#59529=DIRECTION ( 'NONE',  ( 4.476705744456277943E-17, -1.000000000000000000, 0.000000000000000000 ) ) ;
#59531=CARTESIAN_POINT ( 'NONE',  ( -93.67500000000003979, 87.70503267997129626, 88.38604166840097776 ) ) ;
#59535=CARTESIAN_POINT ( 'NONE',  ( 93.84685191531251292, -211.9973110713294489, 88.00239583420048461 ) ) ;
#59548=ORIENTED_EDGE ( 'NONE', *, *, #28166, .T. ) ;
#59549=FACE_OUTER_BOUND ( 'NONE', #34578, .T. ) ;
#59554=( BOUNDED_CURVE ( )  B_SPLINE_CURVE ( 2, ( #6847, #23405, #881, #23769, #69631, #13221, #41069, #35772, #24153 ),
 .UNSPECIFIED., .F., .F. ) 
 B_SPLINE_CURVE_WITH_KNOTS ( ( 3, 2, 2, 2, 3 ),
 ( 0.5715170088666295944, 0.5785727743523535471, 0.5856285398932350450, 0.5926843054341166539, 0.5926843883797353607 ),
 .UNSPECIFIED. ) 
 CURVE ( )  GEOMETRIC_REPRESENTATION_ITEM ( )  RATIONAL_B_SPLINE_CURVE ( ( 1.000000000000000000, 0.8660254037844387076, 1.000000000000000000, 0.8660254037844387076, 1.000000000000000000, 0.8660254037844387076, 1.000000000000000000, 0.9999984250318816326, 0.9999968501007930888 ) ) 
 REPRESENTATION_ITEM ( '' )  );
#59555=CARTESIAN_POINT ( 'NONE',  ( 92.69370383062498320, 91.33154071421968467, 78.31864583420050963 ) ) ;
#59556=PLANE ( 'NONE',  #68425 ) ;
#59558=EDGE_LOOP ( 'NONE', ( #59968, #35133 ) ) ;
#59560=EDGE_LOOP ( 'NONE', ( #31511, #17872, #61386, #1030 ) ) ;
#59566=CARTESIAN_POINT ( 'NONE',  ( -93.59478774260956868, 91.86781405990323890, 74.80441578173237360 ) ) ;
#59571=CARTESIAN_POINT ( 'NONE',  ( -94.99999999999997158, -213.0599564267049857, 76.90312500173429555 ) ) ;
#59572=CARTESIAN_POINT ( 'NONE',  ( -96.15314808468751551, 88.00268892867056536, 89.27239583420049485 ) ) ;
#59573=CARTESIAN_POINT ( 'NONE',  ( 97.64999999999999147, 90.00000000000002842, 75.79187500173429726 ) ) ;
#59574=CARTESIAN_POINT ( 'NONE',  ( -92.35000000000003695, 90.00000000000004263, 75.79187500173429726 ) ) ;
#59576=CARTESIAN_POINT ( 'NONE',  ( 92.69370383062498320, 90.00000000000002842, 77.73656250086715147 ) ) ;
#59581=CARTESIAN_POINT ( 'NONE',  ( -97.64999999989191792, -209.9999848944890175, 78.64888723590522090 ) ) ;
#59583=ORIENTED_EDGE ( 'NONE', *, *, #3502, .T. ) ;
#59589=VERTEX_POINT ( 'NONE', #20717 ) ;
#59593=CARTESIAN_POINT ( 'NONE',  ( 93.67500000000001137, -207.7050326799711968, 88.06854166840095388 ) ) ;
#59596=CARTESIAN_POINT ( 'NONE',  ( 96.32499999999998863, 87.70503267997126784, 84.49666666666666970 ) ) ;
#59602=CARTESIAN_POINT ( 'NONE',  ( 97.65000000000000568, 88.47002178664752137, 85.89895833506763267 ) ) ;
#59604=FACE_OUTER_BOUND ( 'NONE', #12263, .T. ) ;
#59612=EDGE_CURVE ( 'NONE', #64725, #62043, #38757, .T. ) ;
#59615=CARTESIAN_POINT ( 'NONE',  ( 93.84685191531248449, 88.00268892867053694, 84.82739583420048746 ) ) ;
#59616=CARTESIAN_POINT ( 'NONE',  ( -96.15314808468745866, -211.9973110713294489, 86.73239583420048859 ) ) ;
#59618=ORIENTED_EDGE ( 'NONE', *, *, #4778, .F. ) ;
#59620=CARTESIAN_POINT ( 'NONE',  ( -97.64999999999994884, -208.4700217866474645, 81.69208333333332916 ) ) ;
#59621=CARTESIAN_POINT ( 'NONE',  ( -97.30629616937501680, 88.66845928578038638, 75.09072916753380866 ) ) ;
#59624=VECTOR ( 'NONE', #50369, 1000.000000000000000 ) ;
#59625=CARTESIAN_POINT ( 'NONE',  ( 96.15314808468750130, -211.9973110713294489, 84.13947916753380696 ) ) ;
#59629=CARTESIAN_POINT ( 'NONE',  ( 92.69370383062498320, 90.00000000000002842, 89.80156250086714920 ) ) ;
#59633=CARTESIAN_POINT ( 'NONE',  ( 97.30629616937498838, -208.6684592857803295, 80.01197916753382344 ) ) ;
#59636=CARTESIAN_POINT ( 'NONE',  ( 96.32499999999998863, -212.2949673200287179, 80.68666666666665321 ) ) ;
#59640=CARTESIAN_POINT ( 'NONE',  ( 92.35000000000002274, -211.5299782133524502, 81.16291666666666060 ) ) ;
#59648=CARTESIAN_POINT ( 'NONE',  ( -97.30629616937501680, 90.00000000000004263, 84.72156250086715090 ) ) ;
#59650=CARTESIAN_POINT ( 'NONE',  ( -97.64999999992180335, 90.00001303125199570, 79.28395951162846700 ) ) ;
#59651=ADVANCED_FACE ( 'NONE', ( #9437, #32362, #15829, #55305, #3822 ), #61694, .T. ) ;
#59654=CARTESIAN_POINT ( 'NONE',  ( 92.34999999999999432, 88.47002178664753558, 76.71791666666666742 ) ) ;
#59663=CARTESIAN_POINT ( 'NONE',  ( -93.67500000000003979, 92.29496732002878900, 86.69270833506763552 ) ) ;
#59664=CARTESIAN_POINT ( 'NONE',  ( 93.84685191531248449, 91.99731107132950569, 88.42572916753381662 ) ) ;
#59674=AXIS2_PLACEMENT_3D ( 'NONE', #34851, #29557, #63808 ) ;
#59678=VECTOR ( 'NONE', #52805, 1000.000000000000000 ) ;
#59681=CARTESIAN_POINT ( 'NONE',  ( -92.69370383062498320, -209.9999999999999716, 83.76906250086716454 ) ) ;
#59688=CARTESIAN_POINT ( 'NONE',  ( 96.15314808468748708, 91.99731107132950569, 89.58989583420049030 ) ) ;
#59690=CARTESIAN_POINT ( 'NONE',  ( 96.15314808468748708, 91.99731107132950569, 79.90614583420047268 ) ) ;
#59691=B_SPLINE_CURVE_WITH_KNOTS ( 'NONE', 3,
 ( #60416, #37849, #15273, #19795, #9264, #19425, #54760, #42741 ),
 .UNSPECIFIED., .F., .F.,
 ( 4, 2, 2, 4 ),
 ( 0.001653806717454685358, 0.002539064216007148531, 0.002981692965283379900, 0.003424321714559611270 ),
 .UNSPECIFIED. ) ;
#59702=CARTESIAN_POINT ( 'NONE',  ( -93.26027265873587169, -208.4859488783624215, 74.79348190356851944 ) ) ;
#59703=PRODUCT_DEFINITION_CONTEXT ( 'detailed design', #5718, 'design' ) ;
#59707=CARTESIAN_POINT ( 'NONE',  ( -97.30629616937501680, 88.66845928578038638, 86.52072916753381548 ) ) ;
#59713=ORIENTED_EDGE ( 'NONE', *, *, #34310, .T. ) ;
#59715=LINE ( 'NONE', #35652, #8367 ) ;
#59716=CARTESIAN_POINT ( 'NONE',  ( -97.65000000000001990, 90.00000000000004263, 80.47499999999999432 ) ) ;
#59717=CARTESIAN_POINT ( 'NONE',  ( 92.69370383062501162, -211.3315407142195852, 83.50447916753383026 ) ) ;
#59719=ORIENTED_EDGE ( 'NONE', *, *, #72236, .T. ) ;
#59726=CYLINDRICAL_SURFACE ( 'NONE', #46021, 2.649999999999985700 ) ;
#59729=CARTESIAN_POINT ( 'NONE',  ( 97.30629616937498838, -209.9999999999999716, 81.22906250086715829 ) ) ;
#59733=VERTEX_POINT ( 'NONE', #5673 ) ;
#59734=CARTESIAN_POINT ( 'NONE',  ( 7.103376864691351012E-17, -120.0000000000000000, -80.00000000000000000 ) ) ;
#59739=CARTESIAN_POINT ( 'NONE',  ( 97.64999999999997726, -211.5299782133524502, 84.62895833506763665 ) ) ;
#59740=CARTESIAN_POINT ( 'NONE',  ( 94.99999999999998579, 86.94004357329500010, 86.34874999999999545 ) ) ;
#59747=CARTESIAN_POINT ( 'NONE',  ( -97.30629616937501680, 91.33154071421968467, 87.20864583420048177 ) ) ;
#59749=CARTESIAN_POINT ( 'NONE',  ( 97.30629616937498838, 88.66845928578037217, 80.38239583420049428 ) ) ;
#59752=CARTESIAN_POINT ( 'NONE',  ( 97.64999999999997726, 91.52997821335252127, 83.46479166840096298 ) ) ;
#59763=CARTESIAN_POINT ( 'NONE',  ( -97.65000000000001990, 91.52997821335253548, 84.23208333333333542 ) ) ;
#59766=( BOUNDED_CURVE ( )  B_SPLINE_CURVE ( 2, ( #50608, #22421, #44620, #55517, #4782, #67166, #4401, #27295, #50228 ),
 .UNSPECIFIED., .F., .F. ) 
 B_SPLINE_CURVE_WITH_KNOTS ( ( 3, 2, 2, 2, 3 ),
 ( 0.6138516023186938453, 0.6209073675976485296, 0.6279631331385309156, 0.6350188986794131907, 0.6350190250571088324 ),
 .UNSPECIFIED. ) 
 CURVE ( )  GEOMETRIC_REPRESENTATION_ITEM ( )  RATIONAL_B_SPLINE_CURVE ( ( 1.000000000000000000, 0.8660254037844387076, 1.000000000000000000, 0.8660254037844387076, 1.000000000000000000, 0.8660254037844387076, 1.000000000000000000, 0.9999976003453283635, 0.9999952007766184092 ) ) 
 REPRESENTATION_ITEM ( '' )  );
#59769=CARTESIAN_POINT ( 'NONE',  ( 97.64999999999999147, -209.9999999999999716, 85.23749999999999716 ) ) ;
#59770=CARTESIAN_POINT ( 'NONE',  ( -97.30629616937497417, -208.6684592857803011, 83.23989583420046756 ) ) ;
#59777=ADVANCED_BREP_SHAPE_REPRESENTATION ( '', ( #36766, #43395 ), #14652 ) ;
#59788=EDGE_CURVE ( 'NONE', #70067, #38969, #54486, .T. ) ;
#59789=CARTESIAN_POINT ( 'NONE',  ( -93.33922900947484891, 88.39973697852397549, 74.64190534806806454 ) ) ;
#59790=FACE_OUTER_BOUND ( 'NONE', #13776, .T. ) ;
#59793=( BOUNDED_CURVE ( )  B_SPLINE_CURVE ( 2, ( #12225, #18964, #64477, #35161, #35527, #12952, #58099 ),
 .UNSPECIFIED., .F., .F. ) 
 B_SPLINE_CURVE_WITH_KNOTS ( ( 3, 2, 2, 3 ),
 ( 0.9374999999999995559, 0.9444444444444441977, 0.9513888888888889506, 0.9583333333333337034 ),
 .UNSPECIFIED. ) 
 CURVE ( )  GEOMETRIC_REPRESENTATION_ITEM ( )  RATIONAL_B_SPLINE_CURVE ( ( 1.000000000000008660, 0.8660254037844301589, 1.000000000000000000, 0.8660254037844387076, 1.000000000000000000, 0.8660254037844322683, 1.000000000000006439 ) ) 
 REPRESENTATION_ITEM ( '' )  );
#59796=FACE_OUTER_BOUND ( 'NONE', #57278, .T. ) ;
#59797=CYLINDRICAL_SURFACE ( 'NONE', #47799, 2.649999999999985700 ) ;
#59798=CARTESIAN_POINT ( 'NONE',  ( 95.00000000000000000, -213.0599564267049857, 77.45874999999999488 ) ) ;
#59800=DIRECTION ( 'NONE',  ( -0.000000000000000000, -0.000000000000000000, 1.000000000000000000 ) ) ;
#59801=CARTESIAN_POINT ( 'NONE',  ( -93.67499999999998295, -212.2949673200287179, 86.40166666666667084 ) ) ;
#59802=DIRECTION ( 'NONE',  ( -1.000000000000000000, -0.000000000000000000, -0.000000000000000000 ) ) ;
#59804=CIRCLE ( 'NONE', #18940, 26.50000000000000355 ) ;
#59807=CARTESIAN_POINT ( 'NONE',  ( 97.65000000000000568, -208.4700217866474645, 81.55979166840097605 ) ) ;
#59812=ORIENTED_EDGE ( 'NONE', *, *, #59417, .T. ) ;
#59817=CARTESIAN_POINT ( 'NONE',  ( 97.30629616937498838, -209.9999999999999716, 81.70531250086713726 ) ) ;
#59818=CARTESIAN_POINT ( 'NONE',  ( 97.30629616937498838, -209.9999999999999716, 86.94406250086716170 ) ) ;
#59820=CARTESIAN_POINT ( 'NONE',  ( 96.15314808468750130, -211.9973110713294489, 88.10822916753382117 ) ) ;
#59824=CARTESIAN_POINT ( 'NONE',  ( -92.69370383062502583, 91.33154071421968467, 76.20197916753382117 ) ) ;
#59826=VECTOR ( 'NONE', #27256, 1000.000000000000000 ) ;
#59830=CARTESIAN_POINT ( 'NONE',  ( -93.67499999999998295, -212.2949673200287179, 87.75104166840095843 ) ) ;
#59834=CARTESIAN_POINT ( 'NONE',  ( 97.65000000000000568, 91.52997821335252127, 87.90979166840097037 ) ) ;
#59840=CARTESIAN_POINT ( 'NONE',  ( 96.32499999999998863, -212.2949673200287179, 86.40166666666667084 ) ) ;
#59845=CARTESIAN_POINT ( 'NONE',  ( 92.69370383062501162, -209.9999999999999716, 80.11781250086713158 ) ) ;
#59848=VERTEX_POINT ( 'NONE', #24793 ) ;
#59855=CARTESIAN_POINT ( 'NONE',  ( -92.69370383062498320, -209.9999999999999716, 80.43531250086714124 ) ) ;
#59856=CARTESIAN_POINT ( 'NONE',  ( -97.30629616937501680, 91.33154071421968467, 78.31864583420050963 ) ) ;
#59859=CARTESIAN_POINT ( 'NONE',  ( 96.15314808468748708, 88.00268892867053694, 81.59947916753381492 ) ) ;
#59860=VERTEX_POINT ( 'NONE', #47365 ) ;
#59863=VECTOR ( 'NONE', #20530, 1000.000000000000000 ) ;
#59868=CARTESIAN_POINT ( 'NONE',  ( -93.84685191531248449, -208.0026889286704943, 82.44614583420046472 ) ) ;
#59880=CARTESIAN_POINT ( 'NONE',  ( 92.34999999999998010, 91.52997821335250705, 84.86708333333332632 ) ) ;
#59882=CARTESIAN_POINT ( 'NONE',  ( -97.30629616937501680, 90.00000000000004263, 86.46781250086714010 ) ) ;
#59896=CARTESIAN_POINT ( 'NONE',  ( -94.99999999999997158, -207.3369185715606307, 81.38781250086715602 ) ) ;
#59902=CARTESIAN_POINT ( 'NONE',  ( 96.66079198124940319, 88.39975876321993553, 74.80065669543249385 ) ) ;
#59903=LINE ( 'NONE', #8757, #46605 ) ;
#59906=CARTESIAN_POINT ( 'NONE',  ( 92.34999999999999432, 90.00000000000002842, 90.00000000000000000 ) ) ;
#59909=( BOUNDED_CURVE ( )  B_SPLINE_CURVE ( 2, ( #32491, #56175, #9197, #55058, #44155, #9572, #3589, #72348, #15949 ),
 .UNSPECIFIED., .F., .F. ) 
 B_SPLINE_CURVE_WITH_KNOTS ( ( 3, 2, 2, 2, 3 ),
 ( 0.4445132602971398339, 0.4515689946164713753, 0.4586247601573539279, 0.4656805256982363694, 0.4656806970056960315 ),
 .UNSPECIFIED. ) 
 CURVE ( )  GEOMETRIC_REPRESENTATION_ITEM ( )  RATIONAL_B_SPLINE_CURVE ( ( 0.9999988143381067784, 0.8660259966180086089, 1.000000000000000000, 0.8660254037844387076, 1.000000000000000000, 0.8660254037844387076, 1.000000000000000000, 0.9999967472207509367, 0.9999934945994508606 ) ) 
 REPRESENTATION_ITEM ( '' )  );
#59911=CARTESIAN_POINT ( 'NONE',  ( 97.30629616937498838, -209.9999999999999716, 88.21406250086714351 ) ) ;
#59920=VECTOR ( 'NONE', #65937, 1000.000000000000000 ) ;
#59925=ORIENTED_EDGE ( 'NONE', *, *, #29444, .F. ) ;
#59926=ORIENTED_EDGE ( 'NONE', *, *, #20865, .F. ) ;
#59928=EDGE_CURVE ( 'NONE', #48739, #31708, #73143, .T. ) ;
#59934=CARTESIAN_POINT ( 'NONE',  ( 97.30629616937498838, 88.66845928578037217, 81.17614583420048291 ) ) ;
#59935=DIRECTION ( 'NONE',  ( 1.000000000000000000, 0.000000000000000000, 0.000000000000000000 ) ) ;
#59936=CARTESIAN_POINT ( 'NONE',  ( -96.32500000000001705, 92.29496732002878900, 88.06854166840095388 ) ) ;
#59940=ORIENTED_EDGE ( 'NONE', *, *, #10723, .F. ) ;
#59955=CARTESIAN_POINT ( 'NONE',  ( -93.67499999999998295, -207.7050326799711968, 76.53270833506762472 ) ) ;
#59956=CARTESIAN_POINT ( 'NONE',  ( -92.69370383062502583, 88.66845928578038638, 89.43114583420049257 ) ) ;
#59958=CARTESIAN_POINT ( 'NONE',  ( 97.64999999999997726, 91.52997821335252127, 76.47979166840096354 ) ) ;
#59959=CARTESIAN_POINT ( 'NONE',  ( -92.35000000000005116, 91.52997821335253548, 77.74979166840097378 ) ) ;
#59962=CARTESIAN_POINT ( 'NONE',  ( 92.69370383062498320, 91.33154071421968467, 77.68364583420047609 ) ) ;
#59964=DIRECTION ( 'NONE',  ( 1.000000000000000000, 0.000000000000000000, 0.000000000000000000 ) ) ;
#59968=ORIENTED_EDGE ( 'NONE', *, *, #18401, .F. ) ;
#59969=CARTESIAN_POINT ( 'NONE',  ( -96.32499999999996021, -212.2949673200287179, 87.56583333333333030 ) ) ;
#59971=EDGE_CURVE ( 'NONE', #50746, #35410, #49639, .T. ) ;
#59983=ORIENTED_EDGE ( 'NONE', *, *, #44654, .T. ) ;
#59986=DIRECTION ( 'NONE',  ( -0.000000000000000000, -0.000000000000000000, 1.000000000000000000 ) ) ;
#59994=CARTESIAN_POINT ( 'NONE',  ( 97.30629616937498838, 88.66845928578035796, 83.71614583420048916 ) ) ;
#59995=CARTESIAN_POINT ( 'NONE',  ( -97.30629616937497417, -208.6684592857803295, 84.66864583420047552 ) ) ;
#59996=FACE_OUTER_BOUND ( 'NONE', #45616, .T. ) ;
#59997=AXIS2_PLACEMENT_3D ( 'NONE', #68749, #17235, #39057 ) ;
#60000=CARTESIAN_POINT ( 'NONE',  ( -93.67499999999998295, -207.7050326799711968, 78.99333333333332519 ) ) ;
#60004=AXIS2_PLACEMENT_3D ( 'NONE', #11008, #56129, #34300 ) ;
#60006=CARTESIAN_POINT ( 'NONE',  ( 92.69370383062501162, -209.9999999999999716, 83.29281250086714294 ) ) ;
#60010=( BOUNDED_CURVE ( )  B_SPLINE_CURVE ( 2, ( #14709, #19607, #37660, #42554, #48558, #61605, #55959 ),
 .UNSPECIFIED., .F., .F. ) 
 B_SPLINE_CURVE_WITH_KNOTS ( ( 3, 2, 2, 3 ),
 ( 0.6041666666666670737, 0.6111111111111116045, 0.6180555555555559133, 0.6250000000000003331 ),
 .UNSPECIFIED. ) 
 CURVE ( )  GEOMETRIC_REPRESENTATION_ITEM ( )  RATIONAL_B_SPLINE_CURVE ( ( 0.9999999999999914513, 0.8660254037844472563, 1.000000000000000000, 0.8660254037844387076, 1.000000000000000000, 0.8660254037844322683, 1.000000000000006439 ) ) 
 REPRESENTATION_ITEM ( '' )  );
#60011=ORIENTED_EDGE ( 'NONE', *, *, #67849, .T. ) ;
#60018=CARTESIAN_POINT ( 'NONE',  ( 95.00000000000000000, -207.3369185715606307, 78.84781250086714977 ) ) ;
#60022=CARTESIAN_POINT ( 'NONE',  ( 92.34999999999999432, 90.00000000000002842, 76.66499999999999204 ) ) ;
#60026=CARTESIAN_POINT ( 'NONE',  ( 96.32499999999998863, -212.2949673200287179, 80.05166666666666231 ) ) ;
#60036=CARTESIAN_POINT ( 'NONE',  ( -92.69370383062502583, 88.66845928578038638, 85.62114583420047609 ) ) ;
#60040=CARTESIAN_POINT ( 'NONE',  ( 92.34999999999999432, 90.00000000000002842, 75.39499999999999602 ) ) ;
#60044=CARTESIAN_POINT ( 'NONE',  ( -96.32499999999996021, -212.2949673200287179, 84.47020833506762472 ) ) ;
#60046=EDGE_CURVE ( 'NONE', #30489, #8961, #39707, .T. ) ;
#60049=CARTESIAN_POINT ( 'NONE',  ( -92.35000000000003695, 90.00000000000004263, 85.31687500173428873 ) ) ;
#60050=VERTEX_POINT ( 'NONE', #61517 ) ;
#60051=CARTESIAN_POINT ( 'NONE',  ( 97.30629616937498838, 88.66845928578037217, 86.89114583420050053 ) ) ;
#60056=DIRECTION ( 'NONE',  ( -0.000000000000000000, -0.000000000000000000, 1.000000000000000000 ) ) ;
#60060=VECTOR ( 'NONE', #35430, 1000.000000000000000 ) ;
#60062=EDGE_CURVE ( 'NONE', #18753, #40498, #22788, .T. ) ;
#60067=FACE_BOUND ( 'NONE', #72196, .T. ) ;
#60072=CARTESIAN_POINT ( 'NONE',  ( -97.30629616937495996, -209.9999999999999716, 82.81656250086714977 ) ) ;
#60074=CYLINDRICAL_SURFACE ( 'NONE', #58504, 2.649999999999999467 ) ;
#60078=CARTESIAN_POINT ( 'NONE',  ( 93.84685191531248449, 88.00268892867053694, 88.63739583420048973 ) ) ;
#60079=CARTESIAN_POINT ( 'NONE',  ( 92.69370383062498320, 90.00000000000002842, 79.48281250086714067 ) ) ;
#60083=CARTESIAN_POINT ( 'NONE',  ( 94.56602944578222036, 92.35870626171012532, 74.84690984288803861 ) ) ;
#60084=CARTESIAN_POINT ( 'NONE',  ( -95.00000000000002842, 86.94004357329504273, 76.90312500173429555 ) ) ;
#60090=CARTESIAN_POINT ( 'NONE',  ( -96.15314808468752972, 91.99731107132950569, 85.72697916753379843 ) ) ;
#60097=CARTESIAN_POINT ( 'NONE',  ( 93.67500000000001137, -207.7050326799711968, 83.54416666666666913 ) ) ;
#60104=CARTESIAN_POINT ( 'NONE',  ( 96.15314808468750130, -211.9973110713294489, 78.58322916753382970 ) ) ;
#60111=CARTESIAN_POINT ( 'NONE',  ( -92.34999999999999432, -209.9999999999999716, 86.50750000000000739 ) ) ;
#60115=CARTESIAN_POINT ( 'NONE',  ( 92.35000000000002274, -208.4700217866474645, 89.94708333333333883 ) ) ;
#60117=CARTESIAN_POINT ( 'NONE',  ( 92.34999999999999432, 90.00000000000002842, 79.20499999999999829 ) ) ;
#60120=CARTESIAN_POINT ( 'NONE',  ( -93.67500000000003979, 87.70503267997129626, 83.22666666666665947 ) ) ;
#60125=CARTESIAN_POINT ( 'NONE',  ( 93.67500000000001137, -207.7050326799711968, 82.35354166840096468 ) ) ;
#60126=CARTESIAN_POINT ( 'NONE',  ( 92.34999999999999432, 90.00000000000002842, 84.92000000000000171 ) ) ;
#60134=CARTESIAN_POINT ( 'NONE',  ( -97.30629616937501680, 91.33154071421968467, 87.84364583420048689 ) ) ;
#60135=CARTESIAN_POINT ( 'NONE',  ( 93.84685191531248449, 88.00268892867053694, 82.12864583420046927 ) ) ;
#60137=CARTESIAN_POINT ( 'NONE',  ( 93.67499999999999716, 87.70503267997126784, 83.83520833506763381 ) ) ;
#60141=CARTESIAN_POINT ( 'NONE',  ( 97.65000000000009095, -211.5299782133523649, 78.19958333333332234 ) ) ;
#60143=ORIENTED_EDGE ( 'NONE', *, *, #70434, .T. ) ;
#60148=CARTESIAN_POINT ( 'NONE',  ( -92.35000000000005116, 88.47002178664754979, 84.54958333333333087 ) ) ;
#60151=CARTESIAN_POINT ( 'NONE',  ( 92.34999999999999432, 91.52997821335252127, 89.39145833506763950 ) ) ;
#60152=ORIENTED_EDGE ( 'NONE', *, *, #21651, .T. ) ;
#60154=CARTESIAN_POINT ( 'NONE',  ( -97.30629616937495996, -209.9999999999999716, 79.48281250086714067 ) ) ;
#60161=CARTESIAN_POINT ( 'NONE',  ( 92.35000000000002274, -210.0000359395330634, 83.72937624475873974 ) ) ;
#60163=AXIS2_PLACEMENT_3D ( 'NONE', #23693, #17314, #7517 ) ;
#60168=CARTESIAN_POINT ( 'NONE',  ( -97.64999999954994792, 89.99996890530464100, 88.81037122970319331 ) ) ;
#60171=CARTESIAN_POINT ( 'NONE',  ( -97.30629616937501680, 88.66845928578038638, 75.72572916753381378 ) ) ;
#60177=UNCERTAINTY_MEASURE_WITH_UNIT (LENGTH_MEASURE( 1.000000000000000082E-05 ), #35673, 'distance_accuracy_value', 'NONE');
#60178=CARTESIAN_POINT ( 'NONE',  ( -92.34999999999999432, -211.5299782133524218, 84.62895833506763665 ) ) ;
#60179=CARTESIAN_POINT ( 'NONE',  ( -95.00000000000002842, 90.00000000000004263, 90.00000000000000000 ) ) ;
#60180=CARTESIAN_POINT ( 'NONE',  ( -0.0004442498525516064278, 0.001194404164626844313, -85.59999999999999432 ) ) ;
#60183=CARTESIAN_POINT ( 'NONE',  ( -93.67499999999998295, -212.2949673200287179, 87.67166666666666686 ) ) ;
#60186=CYLINDRICAL_SURFACE ( 'NONE', #70973, 2.649999999999985700 ) ;
#60190=EDGE_CURVE ( 'NONE', #54357, #46588, #53194, .T. ) ;
#60197=CARTESIAN_POINT ( 'NONE',  ( 97.30629616937498838, -209.9999999999999716, 82.34031250086714238 ) ) ;
#60198=CARTESIAN_POINT ( 'NONE',  ( 97.30629616937498838, -208.6684592857803295, 88.26697916753381890 ) ) ;
#60201=CARTESIAN_POINT ( 'NONE',  ( 97.30629616937498838, -211.3315407142195852, 86.89114583420050053 ) ) ;
#60205=VECTOR ( 'NONE', #10660, 1000.000000000000000 ) ;
#60206=CARTESIAN_POINT ( 'NONE',  ( -93.84685191531252713, 88.00268892867056536, 77.94822916753382458 ) ) ;
#60213=CARTESIAN_POINT ( 'NONE',  ( 92.34999999999999432, 90.00000000000002842, 88.17437500173430465 ) ) ;
#60216=ORIENTED_EDGE ( 'NONE', *, *, #49113, .T. ) ;
#60220=( BOUNDED_CURVE ( )  B_SPLINE_CURVE ( 2, ( #30695, #53642, #64557, #41618, #19050, #1074, #18677 ),
 .UNSPECIFIED., .F., .F. ) 
 B_SPLINE_CURVE_WITH_KNOTS ( ( 3, 2, 2, 3 ),
 ( 0.3125000000000001665, 0.3194444444444445308, 0.3263888888888890061, 0.3333333333333333703 ),
 .UNSPECIFIED. ) 
 CURVE ( )  GEOMETRIC_REPRESENTATION_ITEM ( )  RATIONAL_B_SPLINE_CURVE ( ( 0.9999999999999967804, 0.8660254037844419273, 1.000000000000000000, 0.8660254037844387076, 1.000000000000000000, 0.8660254037844375974, 1.000000000000001110 ) ) 
 REPRESENTATION_ITEM ( '' )  );
#60226=CARTESIAN_POINT ( 'NONE',  ( 97.30629616937498838, -209.9999999999999716, 79.80031250086713612 ) ) ;
#60230=VERTEX_POINT ( 'NONE', #995 ) ;
#60236=CARTESIAN_POINT ( 'NONE',  ( -93.84685191531247028, -211.9973110713294489, 79.69447916753379957 ) ) ;
#60237=CARTESIAN_POINT ( 'NONE',  ( -93.84685191531252713, 88.00268892867056536, 78.58322916753382970 ) ) ;
#60238=ORIENTED_EDGE ( 'NONE', *, *, #10435, .F. ) ;
#60239=CARTESIAN_POINT ( 'NONE',  ( 97.30629616937498838, 88.66845928578037217, 79.74739583420047495 ) ) ;
#60245=CARTESIAN_POINT ( 'NONE',  ( -97.65000000000001990, 90.00000000000004263, 90.00000000000000000 ) ) ;
#60246=CARTESIAN_POINT ( 'NONE',  ( -93.84685191531248449, -208.0026889286704943, 83.71614583420047495 ) ) ;
#60251=VERTEX_POINT ( 'NONE', #46826 ) ;
#60255=DIRECTION ( 'NONE',  ( -0.000000000000000000, -0.000000000000000000, 1.000000000000000000 ) ) ;
#60257=CARTESIAN_POINT ( 'NONE',  ( -92.69370383062502583, 91.33154071421968467, 84.93322916753379559 ) ) ;
#60260=DIRECTION ( 'NONE',  ( 0.000000000000000000, 0.000000000000000000, 1.000000000000000000 ) ) ;
#60270=CARTESIAN_POINT ( 'NONE',  ( 96.32499999999998863, -212.2949673200287179, 82.59166666666665435 ) ) ;
#60271=CARTESIAN_POINT ( 'NONE',  ( -92.69370383062498320, -208.6684592857803011, 82.55197916753382970 ) ) ;
#60282=CARTESIAN_POINT ( 'NONE',  ( -93.67500000000003979, 92.29496732002878900, 78.35833333333333428 ) ) ;
#60291=EDGE_CURVE ( 'NONE', #62567, #20422, #9175, .T. ) ;
#60296=VECTOR ( 'NONE', #74252, 1000.000000000000000 ) ;
#60301=DIRECTION ( 'NONE',  ( -0.000000000000000000, -0.000000000000000000, 1.000000000000000000 ) ) ;
#60305=ADVANCED_FACE ( 'NONE', ( #59205 ), #3566, .F. ) ;
#60308=CARTESIAN_POINT ( 'NONE',  ( 93.84685191531248449, 91.99731107132950569, 78.90072916753382515 ) ) ;
#60319=CARTESIAN_POINT ( 'NONE',  ( -97.19210266091323547, 91.16770611573559790, 74.89296886168685319 ) ) ;
#60324=CARTESIAN_POINT ( 'NONE',  ( -97.30629616937497417, -208.6684592857803011, 89.58989583420047609 ) ) ;
#60325=CARTESIAN_POINT ( 'NONE',  ( -97.30629616937501680, 91.33154071421968467, 87.84364583420048689 ) ) ;
#60327=CARTESIAN_POINT ( 'NONE',  ( 92.34999999999999432, 88.47002178664753558, 74.89229166840097207 ) ) ;
#60328=CARTESIAN_POINT ( 'NONE',  ( -95.00000000000002842, 87.33691857156074434, 88.53156250086713897 ) ) ;
#60330=CARTESIAN_POINT ( 'NONE',  ( 94.99999999999998579, 92.66308142843935514, 76.30781250086715772 ) ) ;
#60332=CARTESIAN_POINT ( 'NONE',  ( 97.64999999999690772, -210.0000040461968638, 77.06187486178042434 ) ) ;
#60344=CARTESIAN_POINT ( 'NONE',  ( -92.69370383062498320, -209.9999999999999716, 74.87906250086714977 ) ) ;
#60345=ORIENTED_EDGE ( 'NONE', *, *, #50593, .T. ) ;
#60348=B_SPLINE_CURVE_WITH_KNOTS ( 'NONE', 3,
 ( #11859, #41931, #23900, #23526 ),
 .UNSPECIFIED., .F., .F.,
 ( 4, 4 ),
 ( 2.446487931514598506E-06, 1.000000000000000000 ),
 .UNSPECIFIED. ) ;
#60349=CARTESIAN_POINT ( 'NONE',  ( 95.00000000000000000, -209.9999999999999716, 90.00000000000000000 ) ) ;
#60357=EDGE_CURVE ( 'NONE', #41327, #35941, #42297, .T. ) ;
#60362=CARTESIAN_POINT ( 'NONE',  ( 93.84685191531248449, 88.00268892867053694, 82.92239583420048632 ) ) ;
#60363=CARTESIAN_POINT ( 'NONE',  ( -94.99999999999997158, -212.6630814284392557, 84.88031250086713442 ) ) ;
#60366=ADVANCED_FACE ( 'NONE', ( #14061 ), #43031, .F. ) ;
#60368=CARTESIAN_POINT ( 'NONE',  ( -92.34999999999999432, -209.9999999999999716, 78.25249999999999773 ) ) ;
#60369=DIRECTION ( 'NONE',  ( -0.000000000000000000, -0.000000000000000000, 1.000000000000000000 ) ) ;
#60372=CARTESIAN_POINT ( 'NONE',  ( 97.30629616937498838, -209.9999999999999716, 84.24531250086714351 ) ) ;
#60381=EDGE_CURVE ( 'NONE', #42834, #7474, #62188, .T. ) ;
#60383=CARTESIAN_POINT ( 'NONE',  ( 97.30629616937498838, -209.9999999999999716, 77.41906250086715602 ) ) ;
#60391=CARTESIAN_POINT ( 'NONE',  ( 92.35000000000002274, -211.5299782133524502, 82.43291666666665662 ) ) ;
#60394=PRODUCT_DEFINITION_FORMATION_WITH_SPECIFIED_SOURCE ( 'ANY', '', #31948, .NOT_KNOWN. ) ;
#60400=CARTESIAN_POINT ( 'NONE',  ( -92.69370383062504004, 90.00000000000004263, 82.49906250086715431 ) ) ;
#60403=DIRECTION ( 'NONE',  ( -0.000000000000000000, -0.000000000000000000, 1.000000000000000000 ) ) ;
#60404=CARTESIAN_POINT ( 'NONE',  ( -92.34999999999999432, -211.5299782133524218, 83.99395833506763154 ) ) ;
#60406=CARTESIAN_POINT ( 'NONE',  ( -92.34999999999999432, -208.4700217866474645, 86.63979166840097434 ) ) ;
#60407=ORIENTED_EDGE ( 'NONE', *, *, #42139, .T. ) ;
#60410=CARTESIAN_POINT ( 'NONE',  ( -92.35000000000005116, 88.47002178664754979, 83.99395833506763154 ) ) ;
#60413=CARTESIAN_POINT ( 'NONE',  ( 94.99999999999998579, 87.33691857156068750, 85.51531250086713953 ) ) ;
#60416=CARTESIAN_POINT ( 'NONE',  ( -92.69370383062502583, 90.00000000000007105, 74.79348190356851944 ) ) ;
#60417=CARTESIAN_POINT ( 'NONE',  ( 92.35000000000007958, 88.47002178664749295, 88.78291666666667936 ) ) ;
#60428=CYLINDRICAL_SURFACE ( 'NONE', #26930, 2.649999999999985700 ) ;
#60429=CARTESIAN_POINT ( 'NONE',  ( -96.15314808468745866, -211.9973110713294489, 83.55739583420049144 ) ) ;
#60433=B_SPLINE_CURVE_WITH_KNOTS ( 'NONE', 1,
 ( #31002, #37026 ),
 .UNSPECIFIED., .F., .F.,
 ( 2, 2 ),
 ( 0.000000000000000000, 1.000000000000000000 ),
 .UNSPECIFIED. ) ;
#60435=CARTESIAN_POINT ( 'NONE',  ( 92.69370383062501162, -209.9999999999999716, 89.80156250086714920 ) ) ;
#60439=CARTESIAN_POINT ( 'NONE',  ( 97.30629616937498838, 91.33154071421968467, 76.67822916753378593 ) ) ;
#60443=CARTESIAN_POINT ( 'NONE',  ( 95.05423112903699234, 92.38875495131965465, 74.83591575723767164 ) ) ;
#60445=CARTESIAN_POINT ( 'NONE',  ( -93.67500000000003979, 87.70503267997129626, 76.95604166840095672 ) ) ;
#60447=CARTESIAN_POINT ( 'NONE',  ( 92.35000000000006537, -211.5299782133524786, 84.33791666666667197 ) ) ;
#60449=( BOUNDED_CURVE ( )  B_SPLINE_CURVE ( 2, ( #36900, #48189, #71471, #2737, #47814, #4106, #65856, #30880, #7233, #25265, #25623 ),
 .UNSPECIFIED., .F., .F. ) 
 B_SPLINE_CURVE_WITH_KNOTS ( ( 3, 2, 2, 2, 2, 3 ),
 ( 0.6985206468877303010, 0.6985207885507850323, 0.7055765540917019463, 0.7126323196326189713, 0.7196880851735359963, 0.7196881748069930973 ),
 .UNSPECIFIED. ) 
 CURVE ( )  GEOMETRIC_REPRESENTATION_ITEM ( )  RATIONAL_B_SPLINE_CURVE ( ( 0.9999946203230871689, 0.9999973101075368964, 1.000000000000000000, 0.8660254037844387076, 1.000000000000000000, 0.8660254037844387076, 1.000000000000000000, 0.8660254037844387076, 1.000000000000000000, 0.9999982980434729551, 0.9999965961301877648 ) ) 
 REPRESENTATION_ITEM ( '' )  );
#60450=DIRECTION ( 'NONE',  ( 1.000000000000000000, 0.000000000000000000, 0.000000000000000000 ) ) ;
#60453=CARTESIAN_POINT ( 'NONE',  ( -92.69370383062504004, 90.00000000000004263, 82.97531250086714749 ) ) ;
#60463=DIRECTION ( 'NONE',  ( 1.000000000000000000, 1.343011723336883198E-16, -0.000000000000000000 ) ) ;
#60465=VECTOR ( 'NONE', #44349, 1000.000000000000000 ) ;
#60466=CARTESIAN_POINT ( 'NONE',  ( 92.35000000046503033, 89.99996900126896548, 83.09538598081184091 ) ) ;
#60470=CARTESIAN_POINT ( 'NONE',  ( 93.84685191531251292, -211.9973110713294489, 78.47739583420049314 ) ) ;
#60478=CARTESIAN_POINT ( 'NONE',  ( 92.69370383062501162, -211.3315407142195852, 77.78947916753381264 ) ) ;
#60484=DIRECTION ( 'NONE',  ( 0.000000000000000000, 0.000000000000000000, 1.000000000000000000 ) ) ;
#60485=CARTESIAN_POINT ( 'NONE',  ( 97.64999999999999147, -209.9999999999999716, 90.00000000000000000 ) ) ;
#60488=CARTESIAN_POINT ( 'NONE',  ( 95.00000000000000000, -213.0599564267049857, 80.07812500173432113 ) ) ;
#60489=CARTESIAN_POINT ( 'NONE',  ( 97.64999999999997726, 91.52997821335252127, 85.92541666666664923 ) ) ;
#60496=CARTESIAN_POINT ( 'NONE',  ( -92.69370383062504004, 90.00000000000004263, 89.48406250086715374 ) ) ;
#60497=CARTESIAN_POINT ( 'NONE',  ( 97.30629616937498838, 91.33154071421968467, 80.48822916753383083 ) ) ;
#60499=CARTESIAN_POINT ( 'NONE',  ( 96.32499999999997442, 92.29496732002878900, 81.61270833506763722 ) ) ;
#60512=CARTESIAN_POINT ( 'NONE',  ( 92.34999999999999432, 88.47002178664753558, 88.22729166840096582 ) ) ;
#60515=CARTESIAN_POINT ( 'NONE',  ( -97.30629616937497417, -211.3315407142195852, 80.80572916753382628 ) ) ;
#60528=CARTESIAN_POINT ( 'NONE',  ( 92.69370383062498320, 91.33154071421968467, 88.95489583420048518 ) ) ;
#60530=CARTESIAN_POINT ( 'NONE',  ( 99.99999999999998579, 95.00000000000002842, -90.00000000000000000 ) ) ;
#60531=CARTESIAN_POINT ( 'NONE',  ( -96.32499999999996021, -207.7050326799711968, 86.79854166840097207 ) ) ;
#60532=ADVANCED_FACE ( 'NONE', ( #55410 ), #50877, .F. ) ;
#60537=CYLINDRICAL_SURFACE ( 'NONE', #70052, 2.649999999999985700 ) ;
#60543=CARTESIAN_POINT ( 'NONE',  ( -94.99999999999997158, -213.0599564267049857, 89.52375000000000682 ) ) ;
#60545=CARTESIAN_POINT ( 'NONE',  ( -92.35000000000003695, 90.00000000000004263, 90.00000000000000000 ) ) ;
#60546=ADVANCED_FACE ( 'NONE', ( #15929 ), #15562, .F. ) ;
#60562=CARTESIAN_POINT ( 'NONE',  ( 97.30629616937498838, -209.9999999999999716, 81.07031250086714635 ) ) ;
#60563=CARTESIAN_POINT ( 'NONE',  ( 96.15314808468748708, -208.0026889286704943, 84.50989583420049200 ) ) ;
#60566=CARTESIAN_POINT ( 'NONE',  ( 96.15314808468748708, -208.0026889286704943, 85.14489583420048291 ) ) ;
#60571=CARTESIAN_POINT ( 'NONE',  ( -95.00000000000002842, 87.33691857156074434, 76.62531250086715318 ) ) ;
#60576=VERTEX_POINT ( 'NONE', #51985 ) ;
#60578=ORIENTED_EDGE ( 'NONE', *, *, #72990, .F. ) ;
#60583=ORIENTED_EDGE ( 'NONE', *, *, #57673, .T. ) ;
#60588=CARTESIAN_POINT ( 'NONE',  ( 96.15314808468748708, -208.0026889286704943, 78.63614583420047666 ) ) ;
#60596=CARTESIAN_POINT ( 'NONE',  ( -96.32499999999996021, -212.2949673200287179, 84.39083333333333314 ) ) ;
#60599=CARTESIAN_POINT ( 'NONE',  ( -96.15314808468751551, 88.00268892867056536, 78.47739583420049314 ) ) ;
#60601=CARTESIAN_POINT ( 'NONE',  ( 93.84685191531248449, 91.99731107132950569, 76.20197916753380696 ) ) ;
#60608=CARTESIAN_POINT ( 'NONE',  ( -92.69370383062498320, -208.6684592857803295, 82.39322916753381776 ) ) ;
#60610=CARTESIAN_POINT ( 'NONE',  ( -92.34999999999999432, -209.9999999999999716, 89.68250000000000455 ) ) ;
#60611=CARTESIAN_POINT ( 'NONE',  ( -92.69370383062502583, 90.00000000000007105, 74.79348190356851944 ) ) ;
#60615=ORIENTED_EDGE ( 'NONE', *, *, #38130, .T. ) ;
#60619=CARTESIAN_POINT ( 'NONE',  ( -93.84685191531252713, 88.00268892867056536, 86.04447916753380809 ) ) ;
#60620=CARTESIAN_POINT ( 'NONE',  ( -92.34999999999999432, -209.9999999999999716, 90.00000000000000000 ) ) ;
#60621=LINE ( 'NONE', #70768, #49382 ) ;
#60632=CARTESIAN_POINT ( 'NONE',  ( 92.35000000000000853, -211.5299782133524218, 82.43291666666665662 ) ) ;
#60633=CARTESIAN_POINT ( 'NONE',  ( -97.30629616937497417, -211.3315407142195852, 84.13947916753383538 ) ) ;
#60636=CARTESIAN_POINT ( 'NONE',  ( -96.32499999999996021, -212.2949673200287179, 87.01020833506763097 ) ) ;
#60649=CARTESIAN_POINT ( 'NONE',  ( 92.34999999999990905, 91.52997821335249284, 78.51708333333334622 ) ) ;
#60651=ORIENTED_EDGE ( 'NONE', *, *, #60046, .T. ) ;
#60652=( BOUNDED_CURVE ( )  B_SPLINE_CURVE ( 2, ( #46869, #30941, #65923, #18285, #42250, #37353, #57777, #42613, #13656, #8767, #31685 ),
 .UNSPECIFIED., .F., .F. ) 
 B_SPLINE_CURVE_WITH_KNOTS ( ( 3, 2, 2, 2, 2, 3 ),
 ( 0.1481709449575277227, 0.1481710763585297463, 0.1552268418994118271, 0.1622826074402939078, 0.1693383729811760163, 0.1693384224419981210 ),
 .UNSPECIFIED. ) 
 CURVE ( )  GEOMETRIC_REPRESENTATION_ITEM ( )  RATIONAL_B_SPLINE_CURVE ( ( 0.9999950100189032298, 0.9999975049629860058, 1.000000000000000000, 0.8660254037844387076, 1.000000000000000000, 0.8660254037844387076, 1.000000000000000000, 0.8660254037844387076, 1.000000000000000000, 0.9999990608398716674, 0.9999981216929102468 ) ) 
 REPRESENTATION_ITEM ( '' )  );
#60661=ORIENTED_EDGE ( 'NONE', *, *, #56089, .T. ) ;
#60666=CARTESIAN_POINT ( 'NONE',  ( 94.99999999999998579, 92.66308142843935514, 78.21281250086717307 ) ) ;
#60669=CARTESIAN_POINT ( 'NONE',  ( -97.65000000000001990, 90.00000000000004263, 88.17437500173430465 ) ) ;
#60672=ORIENTED_EDGE ( 'NONE', *, *, #35393, .F. ) ;
#60673=CARTESIAN_POINT ( 'NONE',  ( 97.30629616937498838, 88.66845928578037217, 89.27239583420048064 ) ) ;
#60676=CARTESIAN_POINT ( 'NONE',  ( 96.15314808468750130, -211.9973110713294489, 89.21947916753380525 ) ) ;
#60679=CARTESIAN_POINT ( 'NONE',  ( -95.31113939543074309, 92.37342585364828551, 74.84415580543368662 ) ) ;
#60684=CARTESIAN_POINT ( 'NONE',  ( -94.99999999999997158, -206.9400435732949575, 82.85625000000000284 ) ) ;
#60686=CARTESIAN_POINT ( 'NONE',  ( -97.64999999999996305, -209.9999999999999716, 76.10937500173430692 ) ) ;
#60688=CARTESIAN_POINT ( 'NONE',  ( -92.69370383062502583, 91.33154071421968467, 87.63197916753382799 ) ) ;
#60690=CARTESIAN_POINT ( 'NONE',  ( 93.84685191531248449, 91.99731107132950569, 88.90197916753380980 ) ) ;
#60691=CARTESIAN_POINT ( 'NONE',  ( -92.69370383062502583, 88.66845928578038638, 88.63739583420047552 ) ) ;
#60693=CARTESIAN_POINT ( 'NONE',  ( 97.30629616937498838, 90.00000000000002842, 76.78406250086715090 ) ) ;
#60694=CARTESIAN_POINT ( 'NONE',  ( -92.35000000000003695, 90.00000000000004263, 83.33250000000001023 ) ) ;
#60700=EDGE_CURVE ( 'NONE', #50672, #769, #24531, .T. ) ;
#60706=ORIENTED_EDGE ( 'NONE', *, *, #48798, .T. ) ;
#60707=CARTESIAN_POINT ( 'NONE',  ( -93.67500000000003979, 92.29496732002878900, 82.16833333333332234 ) ) ;
#60714=ADVANCED_FACE ( 'NONE', ( #17413 ), #34697, .F. ) ;
#60716=CARTESIAN_POINT ( 'NONE',  ( -96.15314808468751551, 88.00268892867056536, 80.85864583420047325 ) ) ;
#60721=CYLINDRICAL_SURFACE ( 'NONE', #55728, 2.649999999999985700 ) ;
#60729=CARTESIAN_POINT ( 'NONE',  ( 97.30629616937498838, 91.33154071421968467, 81.28197916753381946 ) ) ;
#60730=CARTESIAN_POINT ( 'NONE',  ( -97.30629616937495996, -209.9999999999999716, 84.72156250086715090 ) ) ;
#60734=CARTESIAN_POINT ( 'NONE',  ( -97.64999999999994884, -211.5299782133524502, 76.71791666666666742 ) ) ;
#60739=CARTESIAN_POINT ( 'NONE',  ( 97.30629616937498838, -208.6684592857803011, 82.39322916753381776 ) ) ;
#60744=CARTESIAN_POINT ( 'NONE',  ( -93.67499999999998295, -207.7050326799711968, 75.89770833506763381 ) ) ;
#60746=CARTESIAN_POINT ( 'NONE',  ( -97.65000000000001990, 90.00000000000004263, 79.28437500173430408 ) ) ;
#60748=CARTESIAN_POINT ( 'NONE',  ( 97.30629616937498838, -211.3315407142195852, 79.90614583420048689 ) ) ;
#60752=CARTESIAN_POINT ( 'NONE',  ( -97.28022634951636860, 88.83725486022233042, 74.94226573542110259 ) ) ;
#60753=CARTESIAN_POINT ( 'NONE',  ( 92.69370383062498320, 91.33154071421968467, 86.57364583420047666 ) ) ;
#60755=CARTESIAN_POINT ( 'NONE',  ( 95.00000000000000000, -206.9400435732949575, 80.95125000000000171 ) ) ;
#60757=VERTEX_POINT ( 'NONE', #37672 ) ;
#60759=ORIENTED_EDGE ( 'NONE', *, *, #67293, .T. ) ;
#60760=EDGE_LOOP ( 'NONE', ( #35975, #32461, #22886, #3813 ) ) ;
#60761=CYLINDRICAL_SURFACE ( 'NONE', #1024, 26.50000000000000355 ) ;
#60763=CARTESIAN_POINT ( 'NONE',  ( -96.15314808468752972, 91.99731107132950569, 85.25072916753381946 ) ) ;
#60767=CARTESIAN_POINT ( 'NONE',  ( 92.34999999999999432, 88.47002178664753558, 76.08291666666666231 ) ) ;
#60770=CARTESIAN_POINT ( 'NONE',  ( -97.64999999999996305, -209.9999999999999716, 86.90437500173429441 ) ) ;
#60774=CARTESIAN_POINT ( 'NONE',  ( -92.35000000000005116, 91.52997821335253548, 82.19479166840095274 ) ) ;
#60776=CARTESIAN_POINT ( 'NONE',  ( 96.15314808468748708, 88.00268892867053694, 85.56822916753381492 ) ) ;
#60781=CARTESIAN_POINT ( 'NONE',  ( 94.99999999999998579, 86.94004357329502852, 88.88875000000000171 ) ) ;
#60786=FACE_OUTER_BOUND ( 'NONE', #73232, .T. ) ;
#60794=FACE_OUTER_BOUND ( 'NONE', #59361, .T. ) ;
#60795=CARTESIAN_POINT ( 'NONE',  ( -94.99999999999997158, -207.3369185715606307, 83.29281250086717137 ) ) ;
#60804=CARTESIAN_POINT ( 'NONE',  ( 93.84685191531248449, 88.00268892867053694, 77.04864583420047097 ) ) ;
#60814=CARTESIAN_POINT ( 'NONE',  ( -97.64998927314377397, 88.47001559349419608, 78.06729209680058545 ) ) ;
#60816=CARTESIAN_POINT ( 'NONE',  ( -97.30629616937501680, 91.33154071421968467, 82.60489583420049087 ) ) ;
#60824=CARTESIAN_POINT ( 'NONE',  ( -92.34999999999999432, -209.9999999999999716, 89.68250000000000455 ) ) ;
#60826=CARTESIAN_POINT ( 'NONE',  ( 95.00000000000000000, -212.6630814284392557, 77.89531250086714920 ) ) ;
#60829=AXIS2_PLACEMENT_3D ( 'NONE', #29129, #17489, #23145 ) ;
#60833=CARTESIAN_POINT ( 'NONE',  ( -92.34999999999999432, -209.9999999999999716, 81.42749999999999488 ) ) ;
#60836=CARTESIAN_POINT ( 'NONE',  ( 97.30629616937498838, -211.3315407142195852, 76.73114583420048973 ) ) ;
#60848=CARTESIAN_POINT ( 'NONE',  ( 93.67500000000001137, -212.2949673200287179, 78.75520833506763552 ) ) ;
#60850=CARTESIAN_POINT ( 'NONE',  ( 92.34999999999999432, 91.52997821335252127, 85.50208333333331723 ) ) ;
#60855=CARTESIAN_POINT ( 'NONE',  ( -93.33864827736697123, -211.6008015735577033, 74.79754476654878204 ) ) ;
#60858=CARTESIAN_POINT ( 'NONE',  ( -92.69370383062504004, 90.00000000000004263, 85.03906250086714635 ) ) ;
#60859=CARTESIAN_POINT ( 'NONE',  ( 92.69370383062498320, 91.33154071421968467, 81.96989583420048575 ) ) ;
#60863=CARTESIAN_POINT ( 'NONE',  ( -97.64999999999996305, -209.9999999999999716, 86.18999999999999773 ) ) ;
#60872=DIRECTION ( 'NONE',  ( 1.000000000000000000, 0.000000000000000000, 0.000000000000000000 ) ) ;
#60874=ORIENTED_EDGE ( 'NONE', *, *, #69362, .T. ) ;
#60875=( BOUNDED_CURVE ( )  B_SPLINE_CURVE ( 2, ( #3123, #30907, #7621, #49314, #71870, #19998, #54597 ),
 .UNSPECIFIED., .F., .F. ) 
 B_SPLINE_CURVE_WITH_KNOTS ( ( 3, 2, 2, 3 ),
 ( 0.3175094496506953856, 0.3245652148805889259, 0.3316209804214713119, 0.3386766260338262002 ),
 .UNSPECIFIED. ) 
 CURVE ( )  GEOMETRIC_REPRESENTATION_ITEM ( )  RATIONAL_B_SPLINE_CURVE ( ( 1.000000000000000000, 0.8660254037844387076, 1.000000000000000000, 0.8660254037844387076, 1.000000000000000000, 0.8660276809825613320, 0.9999954456811669390 ) ) 
 REPRESENTATION_ITEM ( '' )  );
#60876=CARTESIAN_POINT ( 'NONE',  ( -93.84685191531247028, -211.9973110713294489, 79.05947916753380866 ) ) ;
#60878=CARTESIAN_POINT ( 'NONE',  ( -97.65000000000001990, 90.00000000000004263, 90.00000000000000000 ) ) ;
#60882=DIRECTION ( 'NONE',  ( 1.000000000000000000, 0.000000000000000000, 0.000000000000000000 ) ) ;
#60883=AXIS2_PLACEMENT_3D ( 'NONE', #74146, #69627, #29386 ) ;
#60884=CARTESIAN_POINT ( 'NONE',  ( 92.35000000000000853, -208.4700217866474645, 83.67645833506763609 ) ) ;
#60889=CARTESIAN_POINT ( 'NONE',  ( 92.69370383062498320, 91.33154071421968467, 87.04989583420046984 ) ) ;
#60892=CARTESIAN_POINT ( 'NONE',  ( -92.35000000000003695, 90.00000000000004263, 88.49187500173430010 ) ) ;
#60894=CARTESIAN_POINT ( 'NONE',  ( 92.69370383062498320, 90.00000000000002842, 89.64281250086713726 ) ) ;
#60898=CARTESIAN_POINT ( 'NONE',  ( -95.00000000000002842, 90.00000000000004263, 90.00000000000000000 ) ) ;
#60899=FACE_OUTER_BOUND ( 'NONE', #70429, .T. ) ;
#60903=CARTESIAN_POINT ( 'NONE',  ( -94.99999999999997158, -206.9400435732949575, 87.30124999999999602 ) ) ;
#60913=CARTESIAN_POINT ( 'NONE',  ( 92.52185191531248165, 90.00000000000002842, 89.90078125043358170 ) ) ;
#60916=CARTESIAN_POINT ( 'NONE',  ( 97.30629616937498838, -209.9999999999999716, 80.43531250086714124 ) ) ;
#60917=CARTESIAN_POINT ( 'NONE',  ( 93.84685191531249870, -208.0026889286704943, 85.88572916753381037 ) ) ;
#60919=CARTESIAN_POINT ( 'NONE',  ( 95.00000000000000000, -207.3369185715606307, 85.83281250086714920 ) ) ;
#60924=ORIENTED_EDGE ( 'NONE', *, *, #28697, .T. ) ;
#60925=CARTESIAN_POINT ( 'NONE',  ( -96.15314808468752972, 91.99731107132950569, 77.63072916753381492 ) ) ;
#60930=DIRECTION ( 'NONE',  ( 1.000000000000000000, 0.000000000000000000, 0.000000000000000000 ) ) ;
#60936=FACE_OUTER_BOUND ( 'NONE', #43901, .T. ) ;
#60941=ORIENTED_EDGE ( 'NONE', *, *, #2231, .T. ) ;
#60944=CARTESIAN_POINT ( 'NONE',  ( -90.00000000000002842, 85.00000000000002842, 90.00000000000000000 ) ) ;
#60949=CARTESIAN_POINT ( 'NONE',  ( -94.99999999999997158, -209.9999999999999716, 90.00000000000000000 ) ) ;
#60952=CARTESIAN_POINT ( 'NONE',  ( -96.15314808468752972, 91.99731107132950569, 79.53572916753381605 ) ) ;
#60953=ADVANCED_FACE ( 'NONE', ( #27856, #49303 ), #21461, .T. ) ;
#60955=CARTESIAN_POINT ( 'NONE',  ( 97.30629616937498838, 88.66845928578037217, 79.11239583420046984 ) ) ;
#60962=CARTESIAN_POINT ( 'NONE',  ( -97.30629616937497417, -211.3315407142195852, 80.17072916753380696 ) ) ;
#60966=ORIENTED_EDGE ( 'NONE', *, *, #36313, .T. ) ;
#60972=CARTESIAN_POINT ( 'NONE',  ( 92.57708711457300410, -209.3980460039466891, 74.90604073465182466 ) ) ;
#60973=CARTESIAN_POINT ( 'NONE',  ( -96.15314808468751551, 88.00268892867056536, 84.66864583420047552 ) ) ;
#60977=ORIENTED_EDGE ( 'NONE', *, *, #20410, .F. ) ;
#60981=CARTESIAN_POINT ( 'NONE',  ( 92.35000000003284981, 90.00000839192529156, 86.90410584365271518 ) ) ;
#60985=CARTESIAN_POINT ( 'NONE',  ( -97.30629616937497417, -208.6684592857803011, 82.12864583420048348 ) ) ;
#60987=CARTESIAN_POINT ( 'NONE',  ( 92.34999999999999432, 90.00001272927832474, 76.10937456147250657 ) ) ;
#60993=LINE ( 'NONE', #42606, #37126 ) ;
#60996=VECTOR ( 'NONE', #73561, 1000.000000000000000 ) ;
#60999=DIRECTION ( 'NONE',  ( -1.000000000000000000, -0.000000000000000000, -0.000000000000000000 ) ) ;
#61000=ORIENTED_EDGE ( 'NONE', *, *, #14572, .T. ) ;
#61002=EDGE_CURVE ( 'NONE', #21836, #49121, #44422, .T. ) ;
#61008=CARTESIAN_POINT ( 'NONE',  ( 93.67500000000001137, -207.7050326799711968, 86.08416666666666117 ) ) ;
#61009=ORIENTED_EDGE ( 'NONE', *, *, #21629, .T. ) ;
#61018=EDGE_LOOP ( 'NONE', ( #1702, #1424, #43676, #39878 ) ) ;
#61022=CARTESIAN_POINT ( 'NONE',  ( 94.99999999999998579, 87.33691857156068750, 75.99031250086716227 ) ) ;
#61025=CIRCLE ( 'NONE', #45435, 26.50000000000000355 ) ;
#61032=CARTESIAN_POINT ( 'NONE',  ( 93.84685191531248449, 88.00268892867053694, 87.20864583420046756 ) ) ;
#61034=CARTESIAN_POINT ( 'NONE',  ( 95.00000000000000000, -213.0599564267049857, 74.99812500173430863 ) ) ;
#61036=FACE_OUTER_BOUND ( 'NONE', #73323, .T. ) ;
#61044=CARTESIAN_POINT ( 'NONE',  ( -96.32499999999996021, -207.7050326799711968, 77.27354166840096639 ) ) ;
#61050=CARTESIAN_POINT ( 'NONE',  ( 92.69370383062498320, 88.66845928578037217, 87.15572916753380639 ) ) ;
#61051=CARTESIAN_POINT ( 'NONE',  ( -93.84685191531254134, 91.99731107132950569, 88.16114583420046813 ) ) ;
#61057=CARTESIAN_POINT ( 'NONE',  ( -94.99999999999997158, -212.6630814284392557, 88.53156250086716739 ) ) ;
#61062=ORIENTED_EDGE ( 'NONE', *, *, #55153, .F. ) ;
#61067=CARTESIAN_POINT ( 'NONE',  ( -97.65000000000001990, 91.52997821335253548, 79.78708333333332803 ) ) ;
#61069=CARTESIAN_POINT ( 'NONE',  ( 96.32499999999998863, -212.2949673200287179, 75.68604166840097491 ) ) ;
#61071=CARTESIAN_POINT ( 'NONE',  ( 97.64999999999999147, 90.00000000000002842, 75.07749999999998636 ) ) ;
#61075=CARTESIAN_POINT ( 'NONE',  ( -96.15314808468752972, 91.99731107132950569, 81.28197916753380525 ) ) ;
#61085=( BOUNDED_SURFACE ( )  B_SPLINE_SURFACE ( 1, 2, ( 
 ( #1447, #24332, #64555, #52154, #699, #58171, #19418, #23590, #41256, #17949, #6669, #29575, #64937, #70172, #24696, #58923, #70918, #59285, #46521, #69446, #40891, #63828, #64195, #1072, #69811, #65304, #1810, #12668, #13033, #35600, #58535, #7413, #53272, #71279, #43116, #3276, #20904, #66048, #14521, #49475, #8141, #37839, #37475, #43855, #26542, #20155, #14896, #32171, #60770, #32547, #15265, #26167, #66770, #60406, #8887, #9629, #66415, #42732, #55493, #2913, #61139, #21256, #48733, #49103, #3642, #65666, #72399, #71657, #38197, #31804, #9250, #4008, #26908, #55115, #72029, #49838, #72756, #31065, #54748, #25803, #44217, #38577, #67140, #15643, #54021, #20542, #2559, #25439, #48367, #43495, #54381, #19783, #14144, #37094, #60044, #8528, #31440, #68264, #33283, #44962, #67888, #39321, #46070, #73884, #45719, #56986, #5493, #45340, #34037, #17124, #5859, #50584, #38946, #73509, #28389, #5121, #61509, #27659, #50203, #33666, #51324, #34404, #51708, #69003, #16759, #74261, #17491, #40055, #28768, #44596, #255, #50962, #57347, #68642, #67514, #16379, #63016, #10364, #16002, #11474, #9991, #22392, #61884, #22018, #73137, #56621, #62256, #22778, #10742, #56238, #23147, #32911, #55863, #4374, #27272, #21643, #4753, #39698, #28019, #62637, #11113, #58445, #29868, #41906, #69361, #58830, #18593, #6232, #2091, #30606, #52068, #7328, #41170, #1362, #12944, #63740, #63368, #17859, #70450, #64107, #47913, #40418, #35519, #1721, #41532, #29131, #24977, #53554, #611, #30246, #12586, #24253, #35881, #12216, #11834, #40805, #18958, #6943, #70831, #34785, #52818, #24609, #47177, #23503, #64846, #35153, #13326, #57726, #6590, #70089, #53185, #46435, #47547, #29494, #36258, #52430, #64470, #59198, #7689, #58088, #985, #23877, #46815, #69730, #18230, #37003, #20457, #49746, #55028, #38108, #61044, #14053, #37751, #49390, #65215, #25718, #65586, #59571, #3558, #71943, #43768, #65964, #2472, #26082, #59955, #2827, #48655, #71572, #3924, #31718, #26456, #14804, #60686, #3190, #66331, #72318, #9544, #8440, #71193, #31352, #9165, #37389, #19332, #54303, #8057, #14436, #32087, #66688, #32459, #26820, #49011, #20816, #42289, #15172, #55401, #25357, #13689, #8800, #36626, #30978, #48285, #20067, #53933, #42648, #19698 ),
 ( #43023, #60324, #54663, #43410, #10648, #27181, #5768, #21933, #68551, #28675, #73043, #67424, #39605, #11385, #61425, #17037, #44875, #44506, #15921, #16666, #72670, #56530, #33574, #50109, #21172, #67798, #39973, #44121, #21550, #38853, #62547, #34320, #9905, #62928, #16291, #61797, #10278, #56144, #67047, #4292, #5407, #50498, #22305, #32825, #45250, #33199, #57263, #15552, #38487, #4663, #28301, #27569, #55775, #27937, #11026, #51238, #73423, #39232, #62161, #5033, #50868, #73792, #68166, #74170, #33952, #56898, #22684, #45632, #29402, #45988, #1637, #896, #1277, #41442, #29773, #52348, #64019, #46723, #29047, #35066, #23058, #23782, #69647, #12494, #7604, #51615, #34689, #41808, #167, #63656, #40335, #57643, #6142, #64385, #18141, #47096, #6861, #70361, #58742, #68914, #17402, #59115, #63282, #12125, #11742, #51979, #24521, #24164, #70001, #41087, #525, #30154, #57998, #35432, #23419, #6502, #58361, #12857, #52725, #18502, #35786, #46351, #7240, #53098, #47456, #18869, #64754, #13240, #36167, #69278, #17766, #40712, #48563, #15743, #65498, #31267, #33018, #44316, #61987, #36908, #42197, #54215, #25271, #42558, #27006, #55963, #49939, #4480, #21750, #39051, #14349, #67248, #16110, #10096, #73244, #13606, #44703, #19978, #27376, #38679, #36532, #13964, #61609, #53829, #59479, #50313, #30517, #42933, #7968, #19611, #19246, #2744, #8343, #67616, #59855, #2379, #53465, #2000, #24889, #47819, #70740, #65129, #30885, #65865, #71478, #72855, #48195, #37299, #60236, #71106, #25630, #21356, #8713, #31631, #55592, #4110, #22125, #51810, #11215, #45821, #57453, #33773, #33385, #39424, #40525, #34144, #17965, #10468, #5596, #46174, #68744, #45067, #34892, #5228, #63472, #23608, #51064, #28491, #5971, #67991, #28877, #73988, #357, #22503, #11572, #23246, #6334, #17227, #51430, #34507, #57828, #56347, #45444, #28127, #69110, #40907, #17595, #29230, #52169, #68377, #11945, #716, #4862, #16866, #56729, #50691, #46538, #63117, #69465, #57091, #16485, #40162, #39796, #62750, #17246, #22885, #27764, #73614, #62369, #10849, #7790, #47645, #36358, #19433, #8155, #52921, #41271, #1461, #30709, #7431, #63845, #29976, #52535, #35989, #24712, #59298, #12683, #12319, #18330, #42383, #64568, #71296, #35257, #58939, #25081 ) ),
 .UNSPECIFIED., .F., .F., .T. ) 
 B_SPLINE_SURFACE_WITH_KNOTS ( ( 2, 2 ),
 ( 3, 2, 2, 2, 2, 2, 2, 2, 2, 2, 2, 2, 2, 2, 2, 2, 2, 2, 2, 2, 2, 2, 2, 2, 2, 2, 2, 2, 2, 2, 2, 2, 2, 2, 2, 2, 2, 2, 2, 2, 2, 2, 2, 2, 2, 2, 2, 2, 2, 2, 2, 2, 2, 2, 2, 2, 2, 2, 2, 2, 2, 2, 2, 2, 2, 2, 2, 2, 2, 2, 2, 2, 2, 2, 2, 2, 2, 2, 2, 2, 2, 2, 2, 2, 2, 2, 2, 2, 2, 2, 2, 2, 2, 2, 2, 2, 2, 2, 2, 2, 2, 2, 2, 2, 2, 2, 2, 2, 2, 2, 2, 2, 2, 2, 2, 2, 2, 2, 2, 2, 2, 2, 2, 2, 2, 2, 2, 2, 2, 2, 2, 2, 2, 2, 2, 2, 2, 2, 2, 2, 2, 2, 3 ),
 ( 0.000000000000000000, 1.000000000000000000 ),
 ( 0.000000000000000000, 0.006944444444444444059, 0.01388888888888888812, 0.02083333333333333218, 0.02777777777777777624, 0.03472222222222222376, 0.04166666666666666435, 0.04861111111111111188, 0.05555555555555555247, 0.06250000000000000000, 0.06944444444444444753, 0.07638888888888889506, 0.08333333333333332871, 0.09027777777777777624, 0.09722222222222222376, 0.1041666666666666713, 0.1111111111111111049, 0.1180555555555555525, 0.1250000000000000000, 0.1319444444444444475, 0.1388888888888888951, 0.1458333333333333426, 0.1527777777777777901, 0.1597222222222222099, 0.1666666666666666574, 0.1736111111111111049, 0.1805555555555555525, 0.1875000000000000000, 0.1944444444444444475, 0.2013888888888888951, 0.2083333333333333426, 0.2152777777777777901, 0.2222222222222222099, 0.2291666666666666574, 0.2361111111111111049, 0.2430555555555555525, 0.2500000000000000000, 0.2569444444444444198, 0.2638888888888888951, 0.2708333333333333148, 0.2777777777777777901, 0.2847222222222222099, 0.2916666666666666852, 0.2986111111111111049, 0.3055555555555555802, 0.3125000000000000000, 0.3194444444444444198, 0.3263888888888888951, 0.3333333333333333148, 0.3402777777777777901, 0.3472222222222222099, 0.3541666666666666852, 0.3611111111111111049, 0.3680555555555555802, 0.3750000000000000000, 0.3819444444444444198, 0.3888888888888888951, 0.3958333333333333148, 0.4027777777777777901, 0.4097222222222222099, 0.4166666666666666852, 0.4236111111111111049, 0.4305555555555555802, 0.4375000000000000000, 0.4444444444444444198, 0.4513888888888888951, 0.4583333333333333148, 0.4652777777777777901, 0.4722222222222222099, 0.4791666666666666852, 0.4861111111111111049, 0.4930555555555555802, 0.5000000000000000000, 0.5069444444444444198, 0.5138888888888888395, 0.5208333333333333703, 0.5277777777777777901, 0.5347222222222222099, 0.5416666666666666297, 0.5486111111111111605, 0.5555555555555555802, 0.5625000000000000000, 0.5694444444444444198, 0.5763888888888888395, 0.5833333333333333703, 0.5902777777777777901, 0.5972222222222222099, 0.6041666666666666297, 0.6111111111111111605, 0.6180555555555555802, 0.6250000000000000000, 0.6319444444444444198, 0.6388888888888888395, 0.6458333333333333703, 0.6527777777777777901, 0.6597222222222222099, 0.6666666666666666297, 0.6736111111111111605, 0.6805555555555555802, 0.6875000000000000000, 0.6944444444444444198, 0.7013888888888888395, 0.7083333333333333703, 0.7152777777777777901, 0.7222222222222222099, 0.7291666666666666297, 0.7361111111111111605, 0.7430555555555555802, 0.7500000000000000000, 0.7569444444444444198, 0.7638888888888888395, 0.7708333333333333703, 0.7777777777777777901, 0.7847222222222222099, 0.7916666666666666297, 0.7986111111111111605, 0.8055555555555555802, 0.8125000000000000000, 0.8194444444444444198, 0.8263888888888888395, 0.8333333333333333703, 0.8402777777777777901, 0.8472222222222222099, 0.8541666666666666297, 0.8611111111111111605, 0.8680555555555555802, 0.8750000000000000000, 0.8819444444444444198, 0.8888888888888888395, 0.8958333333333333703, 0.9027777777777777901, 0.9097222222222222099, 0.9166666666666666297, 0.9236111111111111605, 0.9305555555555555802, 0.9375000000000000000, 0.9444444444444444198, 0.9513888888888888395, 0.9583333333333333703, 0.9652777777777777901, 0.9722222222222222099, 0.9791666666666666297, 0.9842226981114290396 ),
 .UNSPECIFIED. ) 
 GEOMETRIC_REPRESENTATION_ITEM ( )  RATIONAL_B_SPLINE_SURFACE ( (
 ( 1.000000000000000000, 0.8660254037844387076, 1.000000000000000000, 0.8660254037844387076, 1.000000000000000000, 0.8660254037844387076, 1.000000000000000000, 0.8660254037844387076, 1.000000000000000000, 0.8660254037844387076, 1.000000000000000000, 0.8660254037844387076, 1.000000000000000000, 0.8660254037844387076, 1.000000000000000000, 0.8660254037844387076, 1.000000000000000000, 0.8660254037844387076, 1.000000000000000000, 0.8660254037844387076, 1.000000000000000000, 0.8660254037844387076, 1.000000000000000000, 0.8660254037844387076, 1.000000000000000000, 0.8660254037844387076, 1.000000000000000000, 0.8660254037844387076, 1.000000000000000000, 0.8660254037844387076, 1.000000000000000000, 0.8660254037844387076, 1.000000000000000000, 0.8660254037844387076, 1.000000000000000000, 0.8660254037844387076, 1.000000000000000000, 0.8660254037844387076, 1.000000000000000000, 0.8660254037844387076, 1.000000000000000000, 0.8660254037844387076, 1.000000000000000000, 0.8660254037844387076, 1.000000000000000000, 0.8660254037844387076, 1.000000000000000000, 0.8660254037844387076, 1.000000000000000000, 0.8660254037844387076, 1.000000000000000000, 0.8660254037844387076, 1.000000000000000000, 0.8660254037844387076, 1.000000000000000000, 0.8660254037844387076, 1.000000000000000000, 0.8660254037844387076, 1.000000000000000000, 0.8660254037844387076, 1.000000000000000000, 0.8660254037844387076, 1.000000000000000000, 0.8660254037844387076, 1.000000000000000000, 0.8660254037844387076, 1.000000000000000000, 0.8660254037844387076, 1.000000000000000000, 0.8660254037844387076, 1.000000000000000000, 0.8660254037844387076, 1.000000000000000000, 0.8660254037844387076, 1.000000000000000000, 0.8660254037844387076, 1.000000000000000000, 0.8660254037844387076, 1.000000000000000000, 0.8660254037844387076, 1.000000000000000000, 0.8660254037844387076, 1.000000000000000000, 0.8660254037844387076, 1.000000000000000000, 0.8660254037844387076, 1.000000000000000000, 0.8660254037844387076, 1.000000000000000000, 0.8660254037844387076, 1.000000000000000000, 0.8660254037844387076, 1.000000000000000000, 0.8660254037844387076, 1.000000000000000000, 0.8660254037844387076, 1.000000000000000000, 0.8660254037844387076, 1.000000000000000000, 0.8660254037844387076, 1.000000000000000000, 0.8660254037844387076, 1.000000000000000000, 0.8660254037844387076, 1.000000000000000000, 0.8660254037844387076, 1.000000000000000000, 0.8660254037844387076, 1.000000000000000000, 0.8660254037844387076, 1.000000000000000000, 0.8660254037844387076, 1.000000000000000000, 0.8660254037844387076, 1.000000000000000000, 0.8660254037844387076, 1.000000000000000000, 0.8660254037844387076, 1.000000000000000000, 0.8660254037844387076, 1.000000000000000000, 0.8660254037844387076, 1.000000000000000000, 0.8660254037844387076, 1.000000000000000000, 0.8660254037844387076, 1.000000000000000000, 0.8660254037844387076, 1.000000000000000000, 0.8660254037844387076, 1.000000000000000000, 0.8660254037844387076, 1.000000000000000000, 0.8660254037844387076, 1.000000000000000000, 0.8660254037844387076, 1.000000000000000000, 0.8660254037844387076, 1.000000000000000000, 0.8660254037844387076, 1.000000000000000000, 0.8660254037844387076, 1.000000000000000000, 0.8660254037844387076, 1.000000000000000000, 0.8660254037844387076, 1.000000000000000000, 0.8660254037844387076, 1.000000000000000000, 0.8660254037844387076, 1.000000000000000000, 0.8660254037844387076, 1.000000000000000000, 0.8660254037844387076, 1.000000000000000000, 0.8660254037844387076, 1.000000000000000000, 0.8660254037844387076, 1.000000000000000000, 0.8660254037844387076, 1.000000000000000000, 0.8660254037844387076, 1.000000000000000000, 0.8660254037844387076, 1.000000000000000000, 0.8660254037844387076, 1.000000000000000000, 0.8660254037844387076, 1.000000000000000000, 0.8660254037844387076, 1.000000000000000000, 0.8660254037844387076, 1.000000000000000000, 0.8660254037844387076, 1.000000000000000000, 0.8660254037844387076, 1.000000000000000000, 0.8660254037844387076, 1.000000000000000000, 0.8660254037844387076, 1.000000000000000000, 0.8660254037844387076, 1.000000000000000000, 0.8660254037844387076, 1.000000000000000000, 0.8660254037844387076, 1.000000000000000000, 0.8660254037844387076, 1.000000000000000000, 0.8660254037844387076, 1.000000000000000000, 0.8660254037844387076, 1.000000000000000000, 0.8660254037844387076, 1.000000000000000000, 0.8660254037844387076, 1.000000000000000000, 0.8660254037844387076, 1.000000000000000000, 0.8660254037844387076, 1.000000000000000000, 0.8660254037844387076, 1.000000000000000000, 0.8660254037844387076, 1.000000000000000000, 0.8660254037844387076, 1.000000000000000000, 0.8660254037844387076, 1.000000000000000000, 0.8660254037844387076, 1.000000000000000000, 0.8660254037844387076, 1.000000000000000000, 0.8660254037844387076, 1.000000000000000000, 0.8660254037844387076, 1.000000000000000000, 0.8660254037844387076, 1.000000000000000000, 0.8660254037844387076, 1.000000000000000000, 0.8660254037844387076, 1.000000000000000000, 0.8660254037844387076, 1.000000000000000000, 0.8660254037844387076, 1.000000000000000000, 0.8660254037844387076, 1.000000000000000000, 0.8660254037844387076, 1.000000000000000000, 0.8660254037844387076, 1.000000000000000000, 0.8660254037844387076, 1.000000000000000000, 0.8660254037844387076, 1.000000000000000000, 0.8660254037844387076, 1.000000000000000000, 0.8660254037844387076, 1.000000000000000000, 0.8660254037844387076, 1.000000000000000000, 0.8660254037844387076, 1.000000000000000000, 0.8660254037844387076, 1.000000000000000000, 0.8660254037844387076, 1.000000000000000000, 0.8660254037844387076, 1.000000000000000000, 0.8660254037844387076, 1.000000000000000000, 0.8660254037844387076, 1.000000000000000000, 0.8660254037844387076, 1.000000000000000000, 0.8660254037844387076, 1.000000000000000000, 0.8660254037844387076, 1.000000000000000000, 0.8660254037844387076, 1.000000000000000000, 0.8660254037844387076, 1.000000000000000000, 0.8660254037844387076, 1.000000000000000000, 0.8660254037844387076, 1.000000000000000000, 0.8660254037844387076, 1.000000000000000000, 0.8660254037844387076, 1.000000000000000000, 0.8660254037844387076, 1.000000000000000000, 0.8660254037844387076, 1.000000000000000000, 0.8660254037844387076, 1.000000000000000000, 0.8660254037844387076, 1.000000000000000000, 0.8660254037844387076, 1.000000000000000000, 0.9024573129378088421, 0.9469501470576167090),
 ( 1.000000000000000000, 0.8660254037844387076, 1.000000000000000000, 0.8660254037844387076, 1.000000000000000000, 0.8660254037844387076, 1.000000000000000000, 0.8660254037844387076, 1.000000000000000000, 0.8660254037844387076, 1.000000000000000000, 0.8660254037844387076, 1.000000000000000000, 0.8660254037844387076, 1.000000000000000000, 0.8660254037844387076, 1.000000000000000000, 0.8660254037844387076, 1.000000000000000000, 0.8660254037844387076, 1.000000000000000000, 0.8660254037844387076, 1.000000000000000000, 0.8660254037844387076, 1.000000000000000000, 0.8660254037844387076, 1.000000000000000000, 0.8660254037844387076, 1.000000000000000000, 0.8660254037844387076, 1.000000000000000000, 0.8660254037844387076, 1.000000000000000000, 0.8660254037844387076, 1.000000000000000000, 0.8660254037844387076, 1.000000000000000000, 0.8660254037844387076, 1.000000000000000000, 0.8660254037844387076, 1.000000000000000000, 0.8660254037844387076, 1.000000000000000000, 0.8660254037844387076, 1.000000000000000000, 0.8660254037844387076, 1.000000000000000000, 0.8660254037844387076, 1.000000000000000000, 0.8660254037844387076, 1.000000000000000000, 0.8660254037844387076, 1.000000000000000000, 0.8660254037844387076, 1.000000000000000000, 0.8660254037844387076, 1.000000000000000000, 0.8660254037844387076, 1.000000000000000000, 0.8660254037844387076, 1.000000000000000000, 0.8660254037844387076, 1.000000000000000000, 0.8660254037844387076, 1.000000000000000000, 0.8660254037844387076, 1.000000000000000000, 0.8660254037844387076, 1.000000000000000000, 0.8660254037844387076, 1.000000000000000000, 0.8660254037844387076, 1.000000000000000000, 0.8660254037844387076, 1.000000000000000000, 0.8660254037844387076, 1.000000000000000000, 0.8660254037844387076, 1.000000000000000000, 0.8660254037844387076, 1.000000000000000000, 0.8660254037844387076, 1.000000000000000000, 0.8660254037844387076, 1.000000000000000000, 0.8660254037844387076, 1.000000000000000000, 0.8660254037844387076, 1.000000000000000000, 0.8660254037844387076, 1.000000000000000000, 0.8660254037844387076, 1.000000000000000000, 0.8660254037844387076, 1.000000000000000000, 0.8660254037844387076, 1.000000000000000000, 0.8660254037844387076, 1.000000000000000000, 0.8660254037844387076, 1.000000000000000000, 0.8660254037844387076, 1.000000000000000000, 0.8660254037844387076, 1.000000000000000000, 0.8660254037844387076, 1.000000000000000000, 0.8660254037844387076, 1.000000000000000000, 0.8660254037844387076, 1.000000000000000000, 0.8660254037844387076, 1.000000000000000000, 0.8660254037844387076, 1.000000000000000000, 0.8660254037844387076, 1.000000000000000000, 0.8660254037844387076, 1.000000000000000000, 0.8660254037844387076, 1.000000000000000000, 0.8660254037844387076, 1.000000000000000000, 0.8660254037844387076, 1.000000000000000000, 0.8660254037844387076, 1.000000000000000000, 0.8660254037844387076, 1.000000000000000000, 0.8660254037844387076, 1.000000000000000000, 0.8660254037844387076, 1.000000000000000000, 0.8660254037844387076, 1.000000000000000000, 0.8660254037844387076, 1.000000000000000000, 0.8660254037844387076, 1.000000000000000000, 0.8660254037844387076, 1.000000000000000000, 0.8660254037844387076, 1.000000000000000000, 0.8660254037844387076, 1.000000000000000000, 0.8660254037844387076, 1.000000000000000000, 0.8660254037844387076, 1.000000000000000000, 0.8660254037844387076, 1.000000000000000000, 0.8660254037844387076, 1.000000000000000000, 0.8660254037844387076, 1.000000000000000000, 0.8660254037844387076, 1.000000000000000000, 0.8660254037844387076, 1.000000000000000000, 0.8660254037844387076, 1.000000000000000000, 0.8660254037844387076, 1.000000000000000000, 0.8660254037844387076, 1.000000000000000000, 0.8660254037844387076, 1.000000000000000000, 0.8660254037844387076, 1.000000000000000000, 0.8660254037844387076, 1.000000000000000000, 0.8660254037844387076, 1.000000000000000000, 0.8660254037844387076, 1.000000000000000000, 0.8660254037844387076, 1.000000000000000000, 0.8660254037844387076, 1.000000000000000000, 0.8660254037844387076, 1.000000000000000000, 0.8660254037844387076, 1.000000000000000000, 0.8660254037844387076, 1.000000000000000000, 0.8660254037844387076, 1.000000000000000000, 0.8660254037844387076, 1.000000000000000000, 0.8660254037844387076, 1.000000000000000000, 0.8660254037844387076, 1.000000000000000000, 0.8660254037844387076, 1.000000000000000000, 0.8660254037844387076, 1.000000000000000000, 0.8660254037844387076, 1.000000000000000000, 0.8660254037844387076, 1.000000000000000000, 0.8660254037844387076, 1.000000000000000000, 0.8660254037844387076, 1.000000000000000000, 0.8660254037844387076, 1.000000000000000000, 0.8660254037844387076, 1.000000000000000000, 0.8660254037844387076, 1.000000000000000000, 0.8660254037844387076, 1.000000000000000000, 0.8660254037844387076, 1.000000000000000000, 0.8660254037844387076, 1.000000000000000000, 0.8660254037844387076, 1.000000000000000000, 0.8660254037844387076, 1.000000000000000000, 0.8660254037844387076, 1.000000000000000000, 0.8660254037844387076, 1.000000000000000000, 0.8660254037844387076, 1.000000000000000000, 0.8660254037844387076, 1.000000000000000000, 0.8660254037844387076, 1.000000000000000000, 0.8660254037844387076, 1.000000000000000000, 0.8660254037844387076, 1.000000000000000000, 0.8660254037844387076, 1.000000000000000000, 0.8660254037844387076, 1.000000000000000000, 0.8660254037844387076, 1.000000000000000000, 0.8660254037844387076, 1.000000000000000000, 0.8660254037844387076, 1.000000000000000000, 0.8660254037844387076, 1.000000000000000000, 0.8660254037844387076, 1.000000000000000000, 0.8660254037844387076, 1.000000000000000000, 0.8660254037844387076, 1.000000000000000000, 0.8660254037844387076, 1.000000000000000000, 0.8660254037844387076, 1.000000000000000000, 0.8660254037844387076, 1.000000000000000000, 0.8660254037844387076, 1.000000000000000000, 0.8660254037844387076, 1.000000000000000000, 0.8660254037844387076, 1.000000000000000000, 0.8660254037844387076, 1.000000000000000000, 0.8660254037844387076, 1.000000000000000000, 0.8660254037844387076, 1.000000000000000000, 0.8660254037844387076, 1.000000000000000000, 0.8660254037844387076, 1.000000000000000000, 0.8660254037844387076, 1.000000000000000000, 0.8660254037844387076, 1.000000000000000000, 0.8660254037844387076, 1.000000000000000000, 0.8660254037844387076, 1.000000000000000000, 0.9024573129378088421, 0.9469501470576167090) ) ) 
 REPRESENTATION_ITEM ( '' )  SURFACE ( )  );
#61087=CARTESIAN_POINT ( 'NONE',  ( 97.30629616937498838, 90.00000000000002842, 80.59406250086715318 ) ) ;
#61089=VECTOR ( 'NONE', #12349, 1000.000000000000000 ) ;
#61090=CARTESIAN_POINT ( 'NONE',  ( -94.99999999999997158, -207.3369185715606307, 82.65781250086715204 ) ) ;
#61092=ORIENTED_EDGE ( 'NONE', *, *, #24514, .F. ) ;
#61093=CARTESIAN_POINT ( 'NONE',  ( -94.99999999999997158, -213.0599564267049857, 81.26874999999999716 ) ) ;
#61094=CARTESIAN_POINT ( 'NONE',  ( -92.34999999999999432, -208.4700217866474645, 78.30541666666668732 ) ) ;
#61099=CARTESIAN_POINT ( 'NONE',  ( -93.84685191531254134, 91.99731107132950569, 76.88989583420048746 ) ) ;
#61100=CARTESIAN_POINT ( 'NONE',  ( 93.84685191531251292, -211.9973110713294489, 84.66864583420047552 ) ) ;
#61110=EDGE_CURVE ( 'NONE', #42810, #30067, #55515, .T. ) ;
#61118=CARTESIAN_POINT ( 'NONE',  ( 96.15314808468748708, -208.0026889286704943, 78.15989583420049769 ) ) ;
#61120=CARTESIAN_POINT ( 'NONE',  ( -92.35000000000003695, 90.00000000000004263, 90.00000000000000000 ) ) ;
#61123=CARTESIAN_POINT ( 'NONE',  ( 97.30629616937498838, 91.33154071421968467, 87.63197916753382799 ) ) ;
#61126=CARTESIAN_POINT ( 'NONE',  ( 92.35000000000000853, -209.9999999999999716, 81.74500000000000455 ) ) ;
#61128=ORIENTED_EDGE ( 'NONE', *, *, #6940, .T. ) ;
#61130=ORIENTED_EDGE ( 'NONE', *, *, #10256, .T. ) ;
#61133=DIRECTION ( 'NONE',  ( -0.000000000000000000, -0.000000000000000000, 1.000000000000000000 ) ) ;
#61137=ORIENTED_EDGE ( 'NONE', *, *, #4426, .F. ) ;
#61139=CARTESIAN_POINT ( 'NONE',  ( -97.64999999999996305, -209.9999999999999716, 86.26937500173430351 ) ) ;
#61144=CARTESIAN_POINT ( 'NONE',  ( -93.67500000000003979, 92.29496732002878900, 81.61270833506763722 ) ) ;
#61145=VECTOR ( 'NONE', #41005, 1000.000000000000000 ) ;
#61148=CARTESIAN_POINT ( 'NONE',  ( 93.84685191531248449, 88.00268892867053694, 82.28739583420048120 ) ) ;
#61154=CARTESIAN_POINT ( 'NONE',  ( 96.32499999999998863, 87.70503267997126784, 88.94166666666666288 ) ) ;
#61158=FACE_OUTER_BOUND ( 'NONE', #20341, .T. ) ;
#61165=CARTESIAN_POINT ( 'NONE',  ( 92.34999999999999432, 90.00000000000002842, 90.00000000000000000 ) ) ;
#61167=CARTESIAN_POINT ( 'NONE',  ( -92.69370383062498320, -209.9999999999999716, 84.40406250086715545 ) ) ;
#61169=CARTESIAN_POINT ( 'NONE',  ( 97.64999999999999147, -209.9999999999999716, 81.42749999999999488 ) ) ;
#61175=CARTESIAN_POINT ( 'NONE',  ( 92.35000000046504454, -210.0000309987310061, 83.09538598081256566 ) ) ;
#61176=CARTESIAN_POINT ( 'NONE',  ( 96.15314808468748708, 91.99731107132950569, 76.73114583420047552 ) ) ;
#61178=CARTESIAN_POINT ( 'NONE',  ( 93.67499999999998295, 92.29496732002878900, 86.79854166840097207 ) ) ;
#61184=CARTESIAN_POINT ( 'NONE',  ( 100.0010000000000900, 64.99999999999997158, -290.0000000000000568 ) ) ;
#61185=ORIENTED_EDGE ( 'NONE', *, *, #57836, .T. ) ;
#61186=CARTESIAN_POINT ( 'NONE',  ( -96.15314808468751551, 88.00268892867056536, 83.39864583420047950 ) ) ;
#61193=CARTESIAN_POINT ( 'NONE',  ( -97.64999999993850111, -209.9999881782113675, 76.10900611559516449 ) ) ;
#61199=CARTESIAN_POINT ( 'NONE',  ( 97.64999999999999147, 90.00000000000002842, 83.41187500173430180 ) ) ;
#61200=CARTESIAN_POINT ( 'NONE',  ( 97.30629616937498838, -208.6684592857803011, 80.01197916753380923 ) ) ;
#61204=CYLINDRICAL_SURFACE ( 'NONE', #33244, 2.649999999999999467 ) ;
#61212=CARTESIAN_POINT ( 'NONE',  ( 95.00000000000000000, -212.6630814284392557, 77.26031250086714408 ) ) ;
#61216=ORIENTED_EDGE ( 'NONE', *, *, #12961, .F. ) ;
#61222=AXIS2_PLACEMENT_3D ( 'NONE', #14454, #71585, #55042 ) ;
#61224=CARTESIAN_POINT ( 'NONE',  ( -92.35000000035638834, 89.99995654222792041, 89.12687334326074051 ) ) ;
#61226=ORIENTED_EDGE ( 'NONE', *, *, #33427, .F. ) ;
#61228=CARTESIAN_POINT ( 'NONE',  ( 92.35000000000002274, -208.4700217866474645, 81.77145833506763495 ) ) ;
#61229=CARTESIAN_POINT ( 'NONE',  ( 94.99999999999998579, 93.05995642670504253, 82.85625000000000284 ) ) ;
#61235=CARTESIAN_POINT ( 'NONE',  ( 94.99999999999998579, 93.05995642670504253, 81.03062500173430749 ) ) ;
#61237=CARTESIAN_POINT ( 'NONE',  ( 97.64999999999999147, 89.99999997442942856, 84.04687500080852658 ) ) ;
#61238=CARTESIAN_POINT ( 'NONE',  ( -97.30629616937501680, 91.33154071421968467, 83.39864583420049371 ) ) ;
#61239=CARTESIAN_POINT ( 'NONE',  ( 92.69370383062498320, 90.00000000000002842, 83.29281250086714294 ) ) ;
#61240=ORIENTED_EDGE ( 'NONE', *, *, #24107, .T. ) ;
#61242=DIRECTION ( 'NONE',  ( -0.000000000000000000, -0.000000000000000000, 1.000000000000000000 ) ) ;
#61249=DIRECTION ( 'NONE',  ( -0.000000000000000000, -0.000000000000000000, 1.000000000000000000 ) ) ;
#61250=CARTESIAN_POINT ( 'NONE',  ( 97.64999999999997726, 91.52997821335252127, 89.17979166840096639 ) ) ;
#61253=CARTESIAN_POINT ( 'NONE',  ( -94.99999999999997158, -212.6630814284392557, 80.91156250086714863 ) ) ;
#61255=VECTOR ( 'NONE', #70513, 1000.000000000000000 ) ;
#61257=CARTESIAN_POINT ( 'NONE',  ( 7.103376864691351012E-17, -120.0000000000000000, -64.00000000000000000 ) ) ;
#61259=CARTESIAN_POINT ( 'NONE',  ( -92.35000000035631729, -210.0000434577671911, 89.12687334326093946 ) ) ;
#61260=AXIS2_PLACEMENT_3D ( 'NONE', #6171, #33042, #38702 ) ;
#61262=CARTESIAN_POINT ( 'NONE',  ( -92.35000000000000853, 88.47002178664756400, 89.62958333333334338 ) ) ;
#61266=CARTESIAN_POINT ( 'NONE',  ( -96.32500000000001705, 87.70503267997129626, 86.93083333333332519 ) ) ;
#61269=CARTESIAN_POINT ( 'NONE',  ( 92.34999999999996589, 88.47002178664753558, 77.35291666666665833 ) ) ;
#61270=CARTESIAN_POINT ( 'NONE',  ( -95.00000000000002842, 90.00000000000004263, 90.00000000000000000 ) ) ;
#61271=CARTESIAN_POINT ( 'NONE',  ( 93.67499999999998295, 92.29496732002878900, 76.00354166840097037 ) ) ;
#61278=CARTESIAN_POINT ( 'NONE',  ( -96.32499999999996021, -212.2949673200287179, 83.12083333333332291 ) ) ;
#61290=CARTESIAN_POINT ( 'NONE',  ( 92.69370383062501162, -208.6684592857803011, 89.74864583420048803 ) ) ;
#61296=CARTESIAN_POINT ( 'NONE',  ( 96.15314808468748708, -208.0026889286704943, 81.17614583420048291 ) ) ;
#61297=CARTESIAN_POINT ( 'NONE',  ( 97.30629616937498838, -211.3315407142195852, 84.98614583420047097 ) ) ;
#61300=CARTESIAN_POINT ( 'NONE',  ( 93.84685191531249870, -208.0026889286704943, 87.79072916753381151 ) ) ;
#61301=AXIS2_PLACEMENT_3D ( 'NONE', #28152, #23631, #57853 ) ;
#61308=CARTESIAN_POINT ( 'NONE',  ( -92.69370383062502583, 88.66845928578038638, 76.73114583420048973 ) ) ;
#61317=DIRECTION ( 'NONE',  ( 1.000000000000000000, 0.000000000000000000, 0.000000000000000000 ) ) ;
#61320=( BOUNDED_CURVE ( )  B_SPLINE_CURVE ( 2, ( #29798, #70384, #18888, #47120, #11763, #13260, #52370 ),
 .UNSPECIFIED., .F., .F. ) 
 B_SPLINE_CURVE_WITH_KNOTS ( ( 3, 2, 2, 3 ),
 ( 0.7291666666666665186, 0.7361111111111109384, 0.7430555555555553582, 0.7499999999999996669 ),
 .UNSPECIFIED. ) 
 CURVE ( )  GEOMETRIC_REPRESENTATION_ITEM ( )  RATIONAL_B_SPLINE_CURVE ( ( 1.000000000000002220, 0.8660254037844365982, 1.000000000000000000, 0.8660254037844387076, 1.000000000000000000, 0.8660254037844451469, 0.9999999999999935607 ) ) 
 REPRESENTATION_ITEM ( '' )  );
#61330=ORIENTED_EDGE ( 'NONE', *, *, #41126, .F. ) ;
#61337=CARTESIAN_POINT ( 'NONE',  ( -93.84685191531252713, 88.00268892867056536, 75.40822916753381833 ) ) ;
#61339=CARTESIAN_POINT ( 'NONE',  ( 92.69370383062498320, 88.66845928578037217, 78.90072916753381094 ) ) ;
#61343=ORIENTED_EDGE ( 'NONE', *, *, #26971, .F. ) ;
#61347=CARTESIAN_POINT ( 'NONE',  ( -94.99999999999997158, -207.3369185715606307, 81.22906250086714408 ) ) ;
#61351=ORIENTED_EDGE ( 'NONE', *, *, #7544, .T. ) ;
#61352=EDGE_LOOP ( 'NONE', ( #47796, #46353, #31091, #58836, #508, #73289, #71506, #42046, #4263, #20807, #61771, #35159, #34040, #15826, #59940, #42537, #40860, #38113, #55288, #44300, #70349, #48275, #56295, #20242, #41057, #39508, #60238, #29469, #40592, #32189, #6762, #8115, #17679, #31411, #51551, #39111, #18210, #52536, #42055, #35571, #46422, #56418, #54910, #3372, #25700, #16672, #35848, #59446, #13970, #56605, #17362, #13659 ) ) ;
#61356=CARTESIAN_POINT ( 'NONE',  ( -95.00000000000002842, 87.33691857156074434, 80.91156250086714863 ) ) ;
#61363=VECTOR ( 'NONE', #74199, 1000.000000000000000 ) ;
#61368=CARTESIAN_POINT ( 'NONE',  ( -92.35000000053402403, -209.9999467984910382, 78.96687695417375608 ) ) ;
#61369=CARTESIAN_POINT ( 'NONE',  ( -92.69370383062498320, -209.9999999999999716, 79.95906250086714806 ) ) ;
#61372=CARTESIAN_POINT ( 'NONE',  ( 97.65000000000000568, 88.47002178664752137, 76.37395833506761278 ) ) ;
#61383=VECTOR ( 'NONE', #71323, 1000.000000000000000 ) ;
#61386=ORIENTED_EDGE ( 'NONE', *, *, #60190, .T. ) ;
#61390=CARTESIAN_POINT ( 'NONE',  ( 92.35000000000000853, -209.9999999999999716, 90.00000000000000000 ) ) ;
#61403=ORIENTED_EDGE ( 'NONE', *, *, #64050, .F. ) ;
#61404=EDGE_LOOP ( 'NONE', ( #57555, #43036, #19597, #51037 ) ) ;
#61405=CARTESIAN_POINT ( 'NONE',  ( 97.30629616937498838, 90.00000000000002842, 76.78406250086715090 ) ) ;
#61408=ORIENTED_EDGE ( 'NONE', *, *, #28366, .T. ) ;
#61413=CARTESIAN_POINT ( 'NONE',  ( 92.69370383062498320, 88.66845928578037217, 87.79072916753381151 ) ) ;
#61415=VERTEX_POINT ( 'NONE', #73255 ) ;
#61416=CARTESIAN_POINT ( 'NONE',  ( 95.00000000000000000, -212.6630814284392557, 84.08656250086713158 ) ) ;
#61420=CARTESIAN_POINT ( 'NONE',  ( -92.34999999999999432, -209.9999999999999716, 80.15749999999999886 ) ) ;
#61425=CARTESIAN_POINT ( 'NONE',  ( -96.15314808468747287, -208.0026889286704943, 88.90197916753380980 ) ) ;
#61426=CARTESIAN_POINT ( 'NONE',  ( -97.30629616937501680, 90.00000000000004263, 85.35656250086715602 ) ) ;
#61429=CARTESIAN_POINT ( 'NONE',  ( 92.69370383062498320, 91.33154071421968467, 87.04989583420048405 ) ) ;
#61430=CARTESIAN_POINT ( 'NONE',  ( -97.30629616937501680, 90.00000000000004263, 89.64281250086713726 ) ) ;
#61436=CARTESIAN_POINT ( 'NONE',  ( -92.35000000000013642, 91.52997821335257811, 86.56041666666668277 ) ) ;
#61439=FACE_OUTER_BOUND ( 'NONE', #12657, .T. ) ;
#61443=VECTOR ( 'NONE', #68311, 1000.000000000000000 ) ;
#61444=CARTESIAN_POINT ( 'NONE',  ( -95.00000000000002842, 93.05995642670501411, 80.95125000000000171 ) ) ;
#61453=CARTESIAN_POINT ( 'NONE',  ( -95.00000000000002842, 87.33691857156074434, 80.27656250086714351 ) ) ;
#61455=DIRECTION ( 'NONE',  ( -0.000000000000000000, -0.000000000000000000, 1.000000000000000000 ) ) ;
#61459=CARTESIAN_POINT ( 'NONE',  ( -6.938893903907228378E-15, -80.00000000000000000, -110.0000000000000000 ) ) ;
#61463=LINE ( 'NONE', #55066, #42453 ) ;
#61466=CARTESIAN_POINT ( 'NONE',  ( 92.69370383062498320, 91.33154071421968467, 81.49364583420049257 ) ) ;
#61467=CARTESIAN_POINT ( 'NONE',  ( -96.15314808468745866, -211.9973110713294489, 82.92239583420048632 ) ) ;
#61473=CARTESIAN_POINT ( 'NONE',  ( -97.64999999999996305, -209.9999999999999716, 77.93499999999998806 ) ) ;
#61474=CARTESIAN_POINT ( 'NONE',  ( 97.64999999999987779, -208.4700217866473793, 78.30541666666667311 ) ) ;
#61475=CARTESIAN_POINT ( 'NONE',  ( -92.69370383062505425, 91.33154071421968467, 76.83697916753382628 ) ) ;
#61476=CARTESIAN_POINT ( 'NONE',  ( 97.30629616937498838, -209.9999999999999716, 81.07031250086714635 ) ) ;
#61481=DIRECTION ( 'NONE',  ( 1.000000000000000000, 0.000000000000000000, 0.000000000000000000 ) ) ;
#61487=DIRECTION ( 'NONE',  ( -0.000000000000000000, -0.000000000000000000, 1.000000000000000000 ) ) ;
#61494=CARTESIAN_POINT ( 'NONE',  ( -96.67299840332304939, 88.01659165168840104, 74.96344747200083702 ) ) ;
#61495=CARTESIAN_POINT ( 'NONE',  ( 94.99999999999998579, 92.66308142843935514, 88.37281250086715545 ) ) ;
#61496=LINE ( 'NONE', #4358, #59826 ) ;
#61497=CARTESIAN_POINT ( 'NONE',  ( 97.64999999999997726, -208.4700217866474645, 77.03541666666666288 ) ) ;
#61499=ORIENTED_EDGE ( 'NONE', *, *, #57493, .T. ) ;
#61509=CARTESIAN_POINT ( 'NONE',  ( -93.67499999999998295, -212.2949673200287179, 83.30604166840096525 ) ) ;
#61511=CARTESIAN_POINT ( 'NONE',  ( 97.64999999999999147, -209.9999999999999716, 90.00000000000000000 ) ) ;
#61513=CARTESIAN_POINT ( 'NONE',  ( -92.35000000000005116, 91.52997821335253548, 82.82979166840095786 ) ) ;
#61515=CARTESIAN_POINT ( 'NONE',  ( 97.30629616937498838, 88.66845928578037217, 81.81114583420048803 ) ) ;
#61517=CARTESIAN_POINT ( 'NONE',  ( -92.34999999999999432, -209.9999999999999716, 82.69749999999999091 ) ) ;
#61522=CARTESIAN_POINT ( 'NONE',  ( 92.35000000000003695, 91.52997821335253548, 88.04208333333330927 ) ) ;
#61531=ADVANCED_FACE ( 'NONE', ( #21372 ), #49582, .T. ) ;
#61537=( BOUNDED_CURVE ( )  B_SPLINE_CURVE ( 2, ( #8389, #20408, #65915, #8758, #71522, #25674, #14755 ),
 .UNSPECIFIED., .F., .F. ) 
 B_SPLINE_CURVE_WITH_KNOTS ( ( 3, 2, 2, 3 ),
 ( 0.06249999999999966693, 0.06944444444444407283, 0.07638888888888849260, 0.08333333333333288462 ),
 .UNSPECIFIED. ) 
 CURVE ( )  GEOMETRIC_REPRESENTATION_ITEM ( )  RATIONAL_B_SPLINE_CURVE ( ( 1.000000000000006439, 0.8660254037844322683, 1.000000000000000000, 0.8660254037844387076, 1.000000000000000000, 0.8660254037844472563, 0.9999999999999914513 ) ) 
 REPRESENTATION_ITEM ( '' )  );
#61538=CARTESIAN_POINT ( 'NONE',  ( -94.99999999999997158, -212.6630814284392557, 79.80031250086715033 ) ) ;
#61539=ORIENTED_EDGE ( 'NONE', *, *, #40338, .T. ) ;
#61547=CARTESIAN_POINT ( 'NONE',  ( -97.64999999999996305, -211.5299782133524218, 76.16229166840095388 ) ) ;
#61548=CARTESIAN_POINT ( 'NONE',  ( 96.15314808468748708, 91.99731107132950569, 78.63614583420047666 ) ) ;
#61550=DIRECTION ( 'NONE',  ( 1.000000000000000000, 0.000000000000000000, 0.000000000000000000 ) ) ;
#61552=CYLINDRICAL_SURFACE ( 'NONE', #70053, 2.649999999999999467 ) ;
#61554=CARTESIAN_POINT ( 'NONE',  ( 95.00000000000000000, -213.0599564267049857, 84.44374999999999432 ) ) ;
#61560=CARTESIAN_POINT ( 'NONE',  ( -97.30629616937501680, 90.00000000000004263, 83.29281250086714294 ) ) ;
#61571=CARTESIAN_POINT ( 'NONE',  ( 92.69370383062501162, -209.9999999999999716, 77.73656250086715147 ) ) ;
#61576=CARTESIAN_POINT ( 'NONE',  ( 97.64999999999999147, -210.0000001167898631, 84.68187499741277691 ) ) ;
#61578=CARTESIAN_POINT ( 'NONE',  ( 96.66135172262724495, 88.39919842643632819, 74.79754476654878204 ) ) ;
#61581=CARTESIAN_POINT ( 'NONE',  ( 92.35000000000002274, -211.5299782133524502, 88.14791666666666003 ) ) ;
#61590=ORIENTED_EDGE ( 'NONE', *, *, #59430, .T. ) ;
#61591=CARTESIAN_POINT ( 'NONE',  ( 97.64999999999324132, -209.9999940177821713, 82.14187520865721126 ) ) ;
#61592=CARTESIAN_POINT ( 'NONE',  ( 96.32499999999998863, -207.7050326799711968, 79.07270833506763097 ) ) ;
#61593=CARTESIAN_POINT ( 'NONE',  ( 97.64999999999999147, 90.00000000000002842, 80.15749999999999886 ) ) ;
#61597=CARTESIAN_POINT ( 'NONE',  ( -92.35002509397452286, -211.5299927013654155, 89.07395733288689144 ) ) ;
#61600=CARTESIAN_POINT ( 'NONE',  ( -92.69370383062505425, 88.66845928578038638, 83.08114583420048405 ) ) ;
#61601=CARTESIAN_POINT ( 'NONE',  ( 92.69370383062498320, 91.33154071421968467, 79.42989583420046529 ) ) ;
#61605=CARTESIAN_POINT ( 'NONE',  ( -97.65000000000009095, 88.47002178664760663, 80.52791666666665549 ) ) ;
#61609=CARTESIAN_POINT ( 'NONE',  ( -92.69370383062498320, -209.9999999999999716, 81.07031250086714635 ) ) ;
#61613=CARTESIAN_POINT ( 'NONE',  ( 92.34999999999999432, 90.00000000000002842, 79.20499999999999829 ) ) ;
#61620=CARTESIAN_POINT ( 'NONE',  ( -96.15314808468747287, -208.0026889286704943, 80.64697916753381435 ) ) ;
#61621=VERTEX_POINT ( 'NONE', #22896 ) ;
#61622=CARTESIAN_POINT ( 'NONE',  ( 92.34999999999999432, 89.99996562134467126, 88.80937619077334944 ) ) ;
#61624=DIRECTION ( 'NONE',  ( 1.000000000000000000, 0.000000000000000000, 0.000000000000000000 ) ) ;
#61627=CARTESIAN_POINT ( 'NONE',  ( 96.92442009029373651, 88.17815826261617929, 75.00000000000000000 ) ) ;
#61630=CARTESIAN_POINT ( 'NONE',  ( 92.69370383062498320, 90.00000000000002842, 89.00781250086714635 ) ) ;
#61634=CARTESIAN_POINT ( 'NONE',  ( -92.35000000000005116, 91.52997821335253548, 88.54479166840097548 ) ) ;
#61641=CARTESIAN_POINT ( 'NONE',  ( 96.32499999999997442, 92.29496732002878900, 75.89770833506763381 ) ) ;
#61648=CARTESIAN_POINT ( 'NONE',  ( -96.32499999999996021, -207.7050326799711968, 84.17916666666666003 ) ) ;
#61656=CARTESIAN_POINT ( 'NONE',  ( 97.30629616937498838, -208.6684592857803011, 87.63197916753382799 ) ) ;
#61661=ORIENTED_EDGE ( 'NONE', *, *, #72144, .T. ) ;
#61663=CARTESIAN_POINT ( 'NONE',  ( 93.84685191531251292, -211.9973110713294489, 78.31864583420048120 ) ) ;
#61664=CARTESIAN_POINT ( 'NONE',  ( 95.00000000000000000, -212.6630814284392557, 86.78531250086713555 ) ) ;
#61666=CARTESIAN_POINT ( 'NONE',  ( 92.69370383062501162, -208.6684592857803011, 87.84364583420048689 ) ) ;
#61673=AXIS2_PLACEMENT_3D ( 'NONE', #72740, #22000, #44195 ) ;
#61677=CARTESIAN_POINT ( 'NONE',  ( -92.35000000000009379, 88.47002178664750716, 77.56458333333333144 ) ) ;
#61678=CARTESIAN_POINT ( 'NONE',  ( 92.35000000000000853, -209.9999999999999716, 88.80937500173430976 ) ) ;
#61680=DIRECTION ( 'NONE',  ( -0.000000000000000000, -0.000000000000000000, 1.000000000000000000 ) ) ;
#61691=CARTESIAN_POINT ( 'NONE',  ( 97.30629616937497417, -210.9303163890423605, 74.68334086212732359 ) ) ;
#61694=PLANE ( 'NONE',  #19811 ) ;
#61701=CARTESIAN_POINT ( 'NONE',  ( 92.35000000000000853, -209.9999999999999716, 86.82500000000000284 ) ) ;
#61702=CARTESIAN_POINT ( 'NONE',  ( -96.15314808468751551, 88.00268892867056536, 77.20739583420048291 ) ) ;
#61704=CARTESIAN_POINT ( 'NONE',  ( 93.84685191531248449, 91.99731107132950569, 76.83697916753381207 ) ) ;
#61706=CARTESIAN_POINT ( 'NONE',  ( -92.69370383062498320, -211.3315407142195852, 89.27239583420048064 ) ) ;
#61711=CARTESIAN_POINT ( 'NONE',  ( -92.69370383062498320, -211.3315407142195852, 79.74739583420047495 ) ) ;
#61714=CYLINDRICAL_SURFACE ( 'NONE', #32646, 2.649999999999999467 ) ;
#61716=CARTESIAN_POINT ( 'NONE',  ( -92.34999999999999432, -211.5299782133524218, 79.46958333333331836 ) ) ;
#61721=CARTESIAN_POINT ( 'NONE',  ( 94.32747394040364952, -207.6887180216937452, 74.85222950654851104 ) ) ;
#61722=CARTESIAN_POINT ( 'NONE',  ( -96.15314808468752972, 91.99731107132950569, 81.28197916753380525 ) ) ;
#61731=EDGE_CURVE ( 'NONE', #423, #26840, #42392, .T. ) ;
#61737=DIRECTION ( 'NONE',  ( -0.000000000000000000, -0.000000000000000000, 1.000000000000000000 ) ) ;
#61738=CARTESIAN_POINT ( 'NONE',  ( -96.15314808468745866, -211.9973110713294489, 78.47739583420049314 ) ) ;
#61740=ADVANCED_FACE ( 'NONE', ( #42760 ), #60074, .F. ) ;
#61741=( BOUNDED_CURVE ( )  B_SPLINE_CURVE ( 2, ( #54857, #51346, #71761, #32657, #45362 ),
 .UNSPECIFIED., .F., .F. ) 
 B_SPLINE_CURVE_WITH_KNOTS ( ( 3, 2, 3 ),
 ( 0.9525283480368235134, 0.9595841135647146247, 0.9629953541097220349 ),
 .UNSPECIFIED. ) 
 CURVE ( )  GEOMETRIC_REPRESENTATION_ITEM ( )  RATIONAL_B_SPLINE_CURVE ( ( 1.000000000000000000, 0.8660254037844387076, 1.000000000000000000, 0.9352274998423326657, 0.9330859296547711068 ) ) 
 REPRESENTATION_ITEM ( '' )  );
#61745=CARTESIAN_POINT ( 'NONE',  ( 97.64999999999601243, 89.99999541993086893, 76.42687486206342840 ) ) ;
#61746=DIRECTION ( 'NONE',  ( -0.000000000000000000, -0.000000000000000000, 1.000000000000000000 ) ) ;
#61753=CARTESIAN_POINT ( 'NONE',  ( -92.35000000035631729, -210.0000434577671911, 89.12687334326093946 ) ) ;
#61758=( BOUNDED_CURVE ( )  B_SPLINE_CURVE ( 2, ( #39062, #61622, #21371, #67260, #56360, #4875, #50702, #52545, #45832, #6344, #730 ),
 .UNSPECIFIED., .F., .F. ) 
 B_SPLINE_CURVE_WITH_KNOTS ( ( 3, 2, 2, 2, 2, 3 ),
 ( 0.04233441017594429673, 0.04233459324529424694, 0.04939035878617636238, 0.05644612432705847088, 0.06350188986794058632, 0.06350193517735322479 ),
 .UNSPECIFIED. ) 
 CURVE ( )  GEOMETRIC_REPRESENTATION_ITEM ( )  RATIONAL_B_SPLINE_CURVE ( ( 0.9999930479532725958, 0.9999965238864447770, 1.000000000000000000, 0.8660254037844387076, 1.000000000000000000, 0.8660254037844387076, 1.000000000000000000, 0.8660254037844387076, 1.000000000000000000, 0.9999991396666700894, 0.9999982793443895623 ) ) 
 REPRESENTATION_ITEM ( '' )  );
#61759=CARTESIAN_POINT ( 'NONE',  ( 96.15314808468750130, -211.9973110713294489, 87.31447916753380412 ) ) ;
#61771=ORIENTED_EDGE ( 'NONE', *, *, #48863, .F. ) ;
#61776=CARTESIAN_POINT ( 'NONE',  ( 96.15314808468748708, 91.99731107132950569, 77.52489583420047836 ) ) ;
#61783=CARTESIAN_POINT ( 'NONE',  ( 92.69370383062498320, 90.00000000000002842, 89.00781250086714635 ) ) ;
#61785=CARTESIAN_POINT ( 'NONE',  ( 92.69370383062501162, -208.6684592857803011, 85.77989583420048803 ) ) ;
#61789=EDGE_CURVE ( 'NONE', #60050, #35038, #69856, .T. ) ;
#61795=CARTESIAN_POINT ( 'NONE',  ( 93.67499999999999716, 87.70503267997126784, 85.10520833506762983 ) ) ;
#61797=CARTESIAN_POINT ( 'NONE',  ( -97.30629616937497417, -211.3315407142195852, 87.79072916753381151 ) ) ;
#61798=CARTESIAN_POINT ( 'NONE',  ( -97.30629616937501680, 91.33154071421968467, 86.57364583420047666 ) ) ;
#61800=CARTESIAN_POINT ( 'NONE',  ( 96.15314808468748708, 88.00268892867053694, 87.94947916753380923 ) ) ;
#61801=CARTESIAN_POINT ( 'NONE',  ( -97.30629616937501680, 91.33154071421968467, 88.31989583420046586 ) ) ;
#61807=DIRECTION ( 'NONE',  ( -0.000000000000000000, -0.000000000000000000, 1.000000000000000000 ) ) ;
#61810=DIRECTION ( 'NONE',  ( 1.000000000000000000, 0.000000000000000000, 0.000000000000000000 ) ) ;
#61815=ADVANCED_FACE ( 'NONE', ( #26190 ), #10396, .F. ) ;
#61816=CARTESIAN_POINT ( 'NONE',  ( -96.32500000000001705, 92.29496732002878900, 81.63916666666666799 ) ) ;
#61825=CARTESIAN_POINT ( 'NONE',  ( -95.00000000000002842, 92.66308142843932671, 81.86406250086714920 ) ) ;
#61830=CARTESIAN_POINT ( 'NONE',  ( -92.35000000000003695, 90.00000000000004263, 85.87249999999998806 ) ) ;
#61833=LINE ( 'NONE', #49784, #43726 ) ;
#61836=CARTESIAN_POINT ( 'NONE',  ( 92.69370383062498320, 90.00000000000002842, 82.18156250086715886 ) ) ;
#61837=CARTESIAN_POINT ( 'NONE',  ( -94.99999999999997158, -207.3369185715606307, 79.48281250086715488 ) ) ;
#61840=CARTESIAN_POINT ( 'NONE',  ( 92.35004305005914205, -208.4699969316842214, 81.13645661577282908 ) ) ;
#61841=CARTESIAN_POINT ( 'NONE',  ( -94.99999999999997158, -206.9400435732949575, 75.87125000000000341 ) ) ;
#61842=CARTESIAN_POINT ( 'NONE',  ( 92.35000000000000853, -209.9999831677331770, 78.64937441956426767 ) ) ;
#61844=CARTESIAN_POINT ( 'NONE',  ( -97.30629616937501680, 90.00000000000004263, 78.37156250086715659 ) ) ;
#61845=CARTESIAN_POINT ( 'NONE',  ( 92.69370383062501162, -208.6684592857803011, 80.06489583420047040 ) ) ;
#61859=CARTESIAN_POINT ( 'NONE',  ( 95.00000000000000000, -212.6630814284392557, 75.35531250086715715 ) ) ;
#61861=CARTESIAN_POINT ( 'NONE',  ( -97.64999999999996305, -209.9999999999999716, 77.93499999999998806 ) ) ;
#61862=CARTESIAN_POINT ( 'NONE',  ( 92.35000000000010800, -211.5299782133525071, 83.70291666666668107 ) ) ;
#61863=CARTESIAN_POINT ( 'NONE',  ( 97.30629616937498838, 90.00000000000002842, 86.30906250086715659 ) ) ;
#61865=CARTESIAN_POINT ( 'NONE',  ( 95.00000000000000000, -206.9400435732949575, 79.68124999999999147 ) ) ;
#61870=EDGE_CURVE ( 'NONE', #73668, #9811, #20181, .T. ) ;
#61871=ORIENTED_EDGE ( 'NONE', *, *, #41317, .T. ) ;
#61878=CARTESIAN_POINT ( 'NONE',  ( -93.33864827737279768, 88.39919842643631398, 74.79754476654878204 ) ) ;
#61881=CARTESIAN_POINT ( 'NONE',  ( -2.499999999999973355, 65.00000000000000000, -290.0000000000000568 ) ) ;
#61882=EDGE_CURVE ( 'NONE', #36423, #55652, #3139, .T. ) ;
#61884=CARTESIAN_POINT ( 'NONE',  ( -96.32499999999996021, -212.2949673200287179, 81.93020833506763267 ) ) ;
#61888=CARTESIAN_POINT ( 'NONE',  ( 94.99999999999998579, 86.94004357329500010, 83.88812500173429498 ) ) ;
#61889=CARTESIAN_POINT ( 'NONE',  ( -97.65000000000001990, 91.52997821335253548, 81.77145833506763495 ) ) ;
#61892=CARTESIAN_POINT ( 'NONE',  ( 93.84685191531248449, 91.99731107132950569, 82.71072916753381321 ) ) ;
#61894=CARTESIAN_POINT ( 'NONE',  ( -97.64999999999996305, -209.9999678301198571, 82.45937388908916432 ) ) ;
#61899=CYLINDRICAL_SURFACE ( 'NONE', #20677, 2.649999999999999467 ) ;
#61904=ADVANCED_FACE ( 'NONE', ( #66439 ), #14920, .F. ) ;
#61908=CARTESIAN_POINT ( 'NONE',  ( -94.99999999999997158, -207.3369185715606307, 80.11781250086714579 ) ) ;
#61918=FACE_OUTER_BOUND ( 'NONE', #43137, .T. ) ;
#61925=CARTESIAN_POINT ( 'NONE',  ( -97.64999999999996305, -209.9999999999999716, 76.66499999999999204 ) ) ;
#61928=CARTESIAN_POINT ( 'NONE',  ( 92.35000000000000853, -209.9999999999999716, 83.01499999999998636 ) ) ;
#61929=CARTESIAN_POINT ( 'NONE',  ( -89.99999999999998579, -116.0000000000000000, -40.00000000000002132 ) ) ;
#61930=CARTESIAN_POINT ( 'NONE',  ( 7.103376864691351012E-17, -120.0000000000000000, -64.00000000000000000 ) ) ;
#61931=CARTESIAN_POINT ( 'NONE',  ( 97.65000000000000568, 88.47002178664752137, 77.00895833506763211 ) ) ;
#61933=CARTESIAN_POINT ( 'NONE',  ( -92.69370383062505425, 88.66845928578038638, 79.74739583420047495 ) ) ;
#61940=CARTESIAN_POINT ( 'NONE',  ( 92.35000000000000853, -209.9999999999999716, 85.55499999999999261 ) ) ;
#61941=CARTESIAN_POINT ( 'NONE',  ( 93.84685191531251292, -211.9973110713294489, 76.57239583420049200 ) ) ;
#61942=EDGE_LOOP ( 'NONE', ( #1982, #25172, #31327, #52368 ) ) ;
#61948=ADVANCED_FACE ( 'NONE', ( #12880 ), #27032, .F. ) ;
#61949=PLANE ( 'NONE',  #26841 ) ;
#61953=CARTESIAN_POINT ( 'NONE',  ( 95.00000000000000000, -206.9400435732949575, 87.93625000000000114 ) ) ;
#61955=ORIENTED_EDGE ( 'NONE', *, *, #59523, .F. ) ;
#61962=EDGE_CURVE ( 'NONE', #20422, #67440, #27442, .T. ) ;
#61967=CARTESIAN_POINT ( 'NONE',  ( 92.35000000000002274, -211.5299782133524502, 81.24229166840098060 ) ) ;
#61968=CARTESIAN_POINT ( 'NONE',  ( 97.64999999999997726, 91.52997821335252127, 81.48041666666665606 ) ) ;
#61972=CARTESIAN_POINT ( 'NONE',  ( -92.35000000002592913, -210.0000117261698165, 82.77687459617060028 ) ) ;
#61976=( BOUNDED_CURVE ( )  B_SPLINE_CURVE ( 2, ( #16712, #6186, #29084, #62207, #22349, #50542, #73465 ),
 .UNSPECIFIED., .F., .F. ) 
 B_SPLINE_CURVE_WITH_KNOTS ( ( 3, 2, 2, 3 ),
 ( 0.2963422021981254040, 0.3033979182579412681, 0.3104536837988239317, 0.3175094496506953856 ),
 .UNSPECIFIED. ) 
 CURVE ( )  GEOMETRIC_REPRESENTATION_ITEM ( )  RATIONAL_B_SPLINE_CURVE ( ( 0.9999981209241102231, 0.8660263433289724366, 1.000000000000000000, 0.8660254037844387076, 1.000000000000000000, 0.8660254037844387076, 1.000000000000000000 ) ) 
 REPRESENTATION_ITEM ( '' )  );
#61977=CARTESIAN_POINT ( 'NONE',  ( -92.69370383062505425, 88.66845928578038638, 85.62114583420047609 ) ) ;
#61979=CARTESIAN_POINT ( 'NONE',  ( 92.69370383062498320, 91.33154071421968467, 78.79489583420047438 ) ) ;
#61981=CARTESIAN_POINT ( 'NONE',  ( -97.30629616937495996, -209.9999999999999716, 89.80156250086714920 ) ) ;
#61983=CARTESIAN_POINT ( 'NONE',  ( 97.64999999999989200, -211.5299782133525071, 85.81958333333332689 ) ) ;
#61987=CARTESIAN_POINT ( 'NONE',  ( -92.69370383062498320, -209.9999999999999716, 82.34031250086714238 ) ) ;
#61995=CARTESIAN_POINT ( 'NONE',  ( 96.32499999999998863, 87.70503267997126784, 78.14666666666667538 ) ) ;
#61998=CARTESIAN_POINT ( 'NONE',  ( -93.84685191531247028, -211.9973110713294489, 76.51947916753380241 ) ) ;
#61999=VERTEX_POINT ( 'NONE', #22192 ) ;
#62000=CARTESIAN_POINT ( 'NONE',  ( -93.67500000000003979, 87.70503267997129626, 86.40166666666667084 ) ) ;
#62012=CARTESIAN_POINT ( 'NONE',  ( 93.67499999999999716, 87.70503267997126784, 86.37520833506764006 ) ) ;
#62014=CARTESIAN_POINT ( 'NONE',  ( 97.64999999999993463, 88.47002178664747873, 77.56458333333333144 ) ) ;
#62023=CARTESIAN_POINT ( 'NONE',  ( -93.67499999999998295, -212.2949673200287179, 85.13166666666666060 ) ) ;
#62026=CARTESIAN_POINT ( 'NONE',  ( -92.35000000000007958, 88.94459177146599416, 75.04099707143593889 ) ) ;
#62034=CARTESIAN_POINT ( 'NONE',  ( 92.69370383062501162, -211.3315407142195852, 88.58447916753382856 ) ) ;
#62042=CARTESIAN_POINT ( 'NONE',  ( 95.00000000000000000, -207.3369185715606307, 78.05406250086714692 ) ) ;
#62043=VERTEX_POINT ( 'NONE', #18754 ) ;
#62044=CARTESIAN_POINT ( 'NONE',  ( 96.15314808468748708, -208.0026889286704943, 82.60489583420049087 ) ) ;
#62047=EDGE_LOOP ( 'NONE', ( #32644, #17044, #672, #17457 ) ) ;
#62050=CARTESIAN_POINT ( 'NONE',  ( -95.00000000000002842, 87.33691857156074434, 75.35531250086715715 ) ) ;
#62052=ORIENTED_EDGE ( 'NONE', *, *, #4809, .T. ) ;
#62053=CARTESIAN_POINT ( 'NONE',  ( 92.34999999999989484, 91.52997821335246442, 86.13708333333332234 ) ) ;
#62055=EDGE_LOOP ( 'NONE', ( #71059, #57247, #30398, #30404 ) ) ;
#62065=CARTESIAN_POINT ( 'NONE',  ( 96.15314808468748708, -208.0026889286704943, 75.46114583420047950 ) ) ;
#62066=DIRECTION ( 'NONE',  ( -0.000000000000000000, -0.000000000000000000, 1.000000000000000000 ) ) ;
#62070=ORIENTED_EDGE ( 'NONE', *, *, #15627, .T. ) ;
#62073=CARTESIAN_POINT ( 'NONE',  ( 97.64999999999999147, -209.9999999999999716, 78.88750000000000284 ) ) ;
#62074=CARTESIAN_POINT ( 'NONE',  ( -95.00000000000002842, 86.94004357329504273, 89.52375000000000682 ) ) ;
#62076=ORIENTED_EDGE ( 'NONE', *, *, #331, .F. ) ;
#62078=CARTESIAN_POINT ( 'NONE',  ( 97.30629616937498838, 91.33154071421968467, 75.40822916753381833 ) ) ;
#62081=CARTESIAN_POINT ( 'NONE',  ( -92.69370383062498320, -209.9999999999999716, 86.78531250086714977 ) ) ;
#62083=EDGE_CURVE ( 'NONE', #14143, #58563, #10799, .T. ) ;
#62088=CARTESIAN_POINT ( 'NONE',  ( -93.84685191531247028, -211.9973110713294489, 79.05947916753380866 ) ) ;
#62089=CARTESIAN_POINT ( 'NONE',  ( -97.64999999999996305, -209.9999999999999716, 89.44437500173430067 ) ) ;
#62096=CARTESIAN_POINT ( 'NONE',  ( -92.69370383062502583, 88.66845928578038638, 82.92239583420045790 ) ) ;
#62101=CARTESIAN_POINT ( 'NONE',  ( -2.500000000000012879, -65.00000000000000000, -290.0000000000000568 ) ) ;
#62104=CARTESIAN_POINT ( 'NONE',  ( 96.92442009029420547, -211.8218417373832096, 75.00000000000001421 ) ) ;
#62106=CARTESIAN_POINT ( 'NONE',  ( -92.69370383062498320, -211.3315407142195852, 78.00114583420049996 ) ) ;
#62121=EDGE_CURVE ( 'NONE', #56423, #62654, #35672, .T. ) ;
#62127=CARTESIAN_POINT ( 'NONE',  ( 96.15314808468748708, -208.0026889286704943, 89.43114583420047836 ) ) ;
#62135=CARTESIAN_POINT ( 'NONE',  ( -97.64999999999994884, -209.9999762675147110, 79.91937418090952860 ) ) ;
#62143=CARTESIAN_POINT ( 'NONE',  ( 97.30629616937498838, 91.33154071421968467, 78.10697916753383652 ) ) ;
#62153=CARTESIAN_POINT ( 'NONE',  ( 92.69370383062501162, -211.3315407142195852, 83.98072916753380923 ) ) ;
#62157=CARTESIAN_POINT ( 'NONE',  ( -97.65000000000001990, 89.99999071025123953, 78.01437532303467037 ) ) ;
#62161=CARTESIAN_POINT ( 'NONE',  ( -96.15314808468745866, -211.9973110713294489, 86.57364583420047666 ) ) ;
#62162=CARTESIAN_POINT ( 'NONE',  ( -96.15314808468751551, 88.00268892867056536, 84.82739583420048746 ) ) ;
#62165=CARTESIAN_POINT ( 'NONE',  ( 93.84685191531248449, 88.00268892867053694, 87.20864583420046756 ) ) ;
#62166=CARTESIAN_POINT ( 'NONE',  ( -97.30629616937501680, 90.00000000000004263, 85.19781250086714408 ) ) ;
#62173=CARTESIAN_POINT ( 'NONE',  ( -97.30629616937497417, -208.6684592857803295, 88.31989583420048007 ) ) ;
#62181=CARTESIAN_POINT ( 'NONE',  ( -97.65000000000001990, 91.52997821335253548, 81.05708333333333826 ) ) ;
#62185=CARTESIAN_POINT ( 'NONE',  ( -97.64999999978466860, 90.00002100773832581, 79.91868729552945183 ) ) ;
#62188=( BOUNDED_CURVE ( )  B_SPLINE_CURVE ( 2, ( #8810, #31729, #54673, #71951, #43419, #37761, #33582 ),
 .UNSPECIFIED., .F., .F. ) 
 B_SPLINE_CURVE_WITH_KNOTS ( ( 3, 2, 2, 3 ),
 ( 0.1458333333333334536, 0.1527777777777778734, 0.1597222222222222654, 0.1666666666666666852 ),
 .UNSPECIFIED. ) 
 CURVE ( )  GEOMETRIC_REPRESENTATION_ITEM ( )  RATIONAL_B_SPLINE_CURVE ( ( 0.9999999999999978906, 0.8660254037844408170, 1.000000000000000000, 0.8660254037844387076, 1.000000000000000000, 0.8660254037844381525, 1.000000000000000444 ) ) 
 REPRESENTATION_ITEM ( '' )  );
#62191=CARTESIAN_POINT ( 'NONE',  ( -97.30629616937501680, 91.33154071421968467, 83.23989583420046756 ) ) ;
#62203=( BOUNDED_CURVE ( )  B_SPLINE_CURVE ( 2, ( #26029, #61372, #14751, #26405, #20760, #10222, #66277, #60987, #32770 ),
 .UNSPECIFIED., .F., .F. ) 
 B_SPLINE_CURVE_WITH_KNOTS ( ( 3, 2, 2, 2, 3 ),
 ( 0.8678591737214816915, 0.8749149270694133174, 0.8819706926102951483, 0.8890264581511769792, 0.8890265259358468564 ),
 .UNSPECIFIED. ) 
 CURVE ( )  GEOMETRIC_REPRESENTATION_ITEM ( )  RATIONAL_B_SPLINE_CURVE ( ( 1.000000000000000000, 0.8660254037844387076, 1.000000000000000000, 0.8660254037844387076, 1.000000000000000000, 0.8660254037844387076, 1.000000000000000000, 0.9999987129073762970, 0.9999974258394828119 ) ) 
 REPRESENTATION_ITEM ( '' )  );
#62204=CARTESIAN_POINT ( 'NONE',  ( 93.84685191531248449, 91.99731107132950569, 80.17072916753382117 ) ) ;
#62206=CARTESIAN_POINT ( 'NONE',  ( -92.69370383062498320, -209.9999999999999716, 79.32406250086715715 ) ) ;
#62207=CARTESIAN_POINT ( 'NONE',  ( -95.00000000000002842, 93.05995642670504253, 84.84062500173429555 ) ) ;
#62210=LINE ( 'NONE', #68600, #20200 ) ;
#62213=EDGE_CURVE ( 'NONE', #71356, #44790, #59804, .T. ) ;
#62215=CARTESIAN_POINT ( 'NONE',  ( -97.30629616937501680, 91.33154071421968467, 79.58864583420049144 ) ) ;
#62216=CARTESIAN_POINT ( 'NONE',  ( 93.84685191531251292, -211.9973110713294489, 79.58864583420047722 ) ) ;
#62217=EDGE_LOOP ( 'NONE', ( #38391, #57319, #54123, #55971 ) ) ;
#62232=CARTESIAN_POINT ( 'NONE',  ( 97.30629616937498838, -208.6684592857803295, 75.56697916753383026 ) ) ;
#62236=CARTESIAN_POINT ( 'NONE',  ( 93.84685191531248449, 91.99731107132950569, 87.79072916753381151 ) ) ;
#62238=CARTESIAN_POINT ( 'NONE',  ( 96.32499999999998863, -207.7050326799711968, 76.45333333333333314 ) ) ;
#62240=VECTOR ( 'NONE', #56938, 1000.000000000000000 ) ;
#62256=CARTESIAN_POINT ( 'NONE',  ( -96.32499999999996021, -207.7050326799711968, 81.71854166840095957 ) ) ;
#62261=CARTESIAN_POINT ( 'NONE',  ( 97.64999999999997726, 91.52997821335252127, 82.19479166840095274 ) ) ;
#62262=CARTESIAN_POINT ( 'NONE',  ( -97.65000000000001990, 88.47002178664754979, 78.06729166840096923 ) ) ;
#62265=CARTESIAN_POINT ( 'NONE',  ( 96.15314808468748708, 88.00268892867053694, 83.66322916753382799 ) ) ;
#62266=CARTESIAN_POINT ( 'NONE',  ( 93.67499999999998295, 92.29496732002878900, 83.54416666666666913 ) ) ;
#62267=CARTESIAN_POINT ( 'NONE',  ( -97.64999999960633659, -209.9999706968024782, 82.45844277047601167 ) ) ;
#62272=CARTESIAN_POINT ( 'NONE',  ( -96.32500000000001705, 92.29496732002878900, 80.36916666666665776 ) ) ;
#62277=CARTESIAN_POINT ( 'NONE',  ( -94.99999999999997158, -209.9999999999999716, 90.00000000000000000 ) ) ;
#62280=CARTESIAN_POINT ( 'NONE',  ( -96.15314808468747287, -208.0026889286704943, 81.44072916753381719 ) ) ;
#62283=CARTESIAN_POINT ( 'NONE',  ( -93.84685191531254134, 91.99731107132950569, 87.52614583420047722 ) ) ;
#62291=CARTESIAN_POINT ( 'NONE',  ( 92.69370383062498320, 90.00000000000002842, 75.03781250086713328 ) ) ;
#62292=VECTOR ( 'NONE', #19201, 1000.000000000000000 ) ;
#62295=CARTESIAN_POINT ( 'NONE',  ( -12.75044424985254921, 0.001194404164626844313, 127.4927882439603195 ) ) ;
#62300=DIRECTION ( 'NONE',  ( -0.000000000000000000, -0.000000000000000000, 1.000000000000000000 ) ) ;
#62307=CARTESIAN_POINT ( 'NONE',  ( -93.84685191531252713, 88.00268892867056536, 78.42447916753381776 ) ) ;
#62311=VECTOR ( 'NONE', #64800, 1000.000000000000000 ) ;
#62312=EDGE_CURVE ( 'NONE', #3737, #32728, #18466, .T. ) ;
#62313=CARTESIAN_POINT ( 'NONE',  ( 92.69370383062501162, -211.3315407142195852, 89.06072916753379332 ) ) ;
#62317=CARTESIAN_POINT ( 'NONE',  ( -92.34999999999999432, -210.0000000198591295, 85.95187500101400246 ) ) ;
#62318=CARTESIAN_POINT ( 'NONE',  ( 92.34999999999999432, 90.00000000000002842, 78.57000000000000739 ) ) ;
#62319=DIRECTION ( 'NONE',  ( -0.000000000000000000, -0.000000000000000000, 1.000000000000000000 ) ) ;
#62321=CARTESIAN_POINT ( 'NONE',  ( 97.30629616937498838, -209.9999999999999716, 76.78406250086715090 ) ) ;
#62323=( BOUNDED_CURVE ( )  B_SPLINE_CURVE ( 2, ( #13906, #31209, #48506, #19919, #49880, #65805, #9672 ),
 .UNSPECIFIED., .F., .F. ) 
 B_SPLINE_CURVE_WITH_KNOTS ( ( 3, 2, 2, 3 ),
 ( 0.7291666666666665186, 0.7361111111111109384, 0.7430555555555553582, 0.7499999999999996669 ),
 .UNSPECIFIED. ) 
 CURVE ( )  GEOMETRIC_REPRESENTATION_ITEM ( )  RATIONAL_B_SPLINE_CURVE ( ( 1.000000000000002220, 0.8660254037844365982, 1.000000000000000000, 0.8660254037844387076, 1.000000000000000000, 0.8660254037844451469, 0.9999999999999935607 ) ) 
 REPRESENTATION_ITEM ( '' )  );
#62325=EDGE_CURVE ( 'NONE', #35410, #44776, #6422, .T. ) ;
#62330=DIRECTION ( 'NONE',  ( -0.000000000000000000, -0.000000000000000000, 1.000000000000000000 ) ) ;
#62334=CARTESIAN_POINT ( 'NONE',  ( 97.64999999999999147, -209.9999999999999716, 89.04749999999999943 ) ) ;
#62340=EDGE_LOOP ( 'NONE', ( #43300, #16464, #69632, #48545 ) ) ;
#62349=CARTESIAN_POINT ( 'NONE',  ( 95.00000000000000000, -213.0599564267049857, 76.90312500173429555 ) ) ;
#62350=CARTESIAN_POINT ( 'NONE',  ( 92.34999999999999432, 91.52997821335252127, 82.32708333333332007 ) ) ;
#62357=CARTESIAN_POINT ( 'NONE',  ( -95.00000000000002842, 92.66308142843932671, 83.92781250086716227 ) ) ;
#62358=CARTESIAN_POINT ( 'NONE',  ( 93.84685191531248449, 88.00268892867053694, 78.31864583420048120 ) ) ;
#62363=AXIS2_PLACEMENT_3D ( 'NONE', #43596, #72502, #55969 ) ;
#62366=ORIENTED_EDGE ( 'NONE', *, *, #58858, .T. ) ;
#62367=CARTESIAN_POINT ( 'NONE',  ( -94.99999999999997158, -213.0599564267049857, 86.34874999999999545 ) ) ;
#62369=CARTESIAN_POINT ( 'NONE',  ( -92.69370383062498320, -209.9999999999999716, 75.99031250086714806 ) ) ;
#62372=CARTESIAN_POINT ( 'NONE',  ( 94.99999999999998579, 93.05995642670504253, 79.04624999999997215 ) ) ;
#62376=FACE_OUTER_BOUND ( 'NONE', #23248, .T. ) ;
#62378=CARTESIAN_POINT ( 'NONE',  ( 94.99999999999998579, 86.94004357329502852, 80.63375000000000625 ) ) ;
#62380=CARTESIAN_POINT ( 'NONE',  ( -92.69370383062498320, -209.9999999999999716, 74.72031250086713783 ) ) ;
#62381=ORIENTED_EDGE ( 'NONE', *, *, #9226, .F. ) ;
#62382=CARTESIAN_POINT ( 'NONE',  ( -95.00000000000002842, 86.94004357329504273, 76.82374999999998977 ) ) ;
#62387=CARTESIAN_POINT ( 'NONE',  ( 97.65000000000000568, -208.4700217866474645, 82.19479166840095274 ) ) ;
#62388=CARTESIAN_POINT ( 'NONE',  ( 97.30629616937498838, 90.00000000000002842, 84.88031250086713442 ) ) ;
#62391=DIRECTION ( 'NONE',  ( 0.000000000000000000, 0.000000000000000000, 1.000000000000000000 ) ) ;
#62405=CARTESIAN_POINT ( 'NONE',  ( -97.30629616937501680, 91.33154071421968467, 88.31989583420048007 ) ) ;
#62406=CARTESIAN_POINT ( 'NONE',  ( -95.00000000000002842, 90.00000000000004263, 90.00000000000000000 ) ) ;
#62408=CARTESIAN_POINT ( 'NONE',  ( -92.34999999999999432, -211.5299782133524502, 84.54958333333333087 ) ) ;
#62411=CARTESIAN_POINT ( 'NONE',  ( 93.67499999999999716, 87.70503267997126784, 85.66083333333332916 ) ) ;
#62419=CARTESIAN_POINT ( 'NONE',  ( 96.15314808468750130, -211.9973110713294489, 86.20322916753382003 ) ) ;
#62420=ORIENTED_EDGE ( 'NONE', *, *, #62661, .T. ) ;
#62422=ORIENTED_EDGE ( 'NONE', *, *, #61882, .F. ) ;
#62425=CARTESIAN_POINT ( 'NONE',  ( -97.64999999969894873, 90.00002455906438570, 87.53856274002211535 ) ) ;
#62427=CARTESIAN_POINT ( 'NONE',  ( -92.34999999999999432, -209.9999998456625860, 79.60187500750915035 ) ) ;
#62428=( BOUNDED_CURVE ( )  B_SPLINE_CURVE ( 2, ( #50942, #7582, #51305, #58342, #65478, #59092, #41423 ),
 .UNSPECIFIED., .F., .F. ) 
 B_SPLINE_CURVE_WITH_KNOTS ( ( 3, 2, 2, 3 ),
 ( 0.2963422021981251264, 0.3033979182579412126, 0.3104536837988238762, 0.3175094496506952191 ),
 .UNSPECIFIED. ) 
 CURVE ( )  GEOMETRIC_REPRESENTATION_ITEM ( )  RATIONAL_B_SPLINE_CURVE ( ( 0.9999981209241187718, 0.8660263433289682178, 1.000000000000000000, 0.8660254037844387076, 1.000000000000000000, 0.8660254037844387076, 1.000000000000000000 ) ) 
 REPRESENTATION_ITEM ( '' )  );
#62429=CARTESIAN_POINT ( 'NONE',  ( 92.69370383062501162, -208.6684592857803295, 78.15989583420048348 ) ) ;
#62431=CARTESIAN_POINT ( 'NONE',  ( 97.30629616937498838, -208.6684592857803011, 83.18697916753382060 ) ) ;
#62436=CARTESIAN_POINT ( 'NONE',  ( -93.84685191531254134, 91.99731107132950569, 74.98489583420048632 ) ) ;
#62443=ORIENTED_EDGE ( 'NONE', *, *, #8766, .F. ) ;
#62451=CARTESIAN_POINT ( 'NONE',  ( 92.69370383062501162, -208.6684592857803011, 75.61989583420047722 ) ) ;
#62453=ORIENTED_EDGE ( 'NONE', *, *, #66780, .T. ) ;
#62457=CARTESIAN_POINT ( 'NONE',  ( 90.00000000000000000, 95.00000000000002842, -79.99999999999998579 ) ) ;
#62459=CARTESIAN_POINT ( 'NONE',  ( -93.84685191531252713, 88.00268892867056536, 76.67822916753381435 ) ) ;
#62461=CARTESIAN_POINT ( 'NONE',  ( 96.32499999999998863, -207.7050326799711968, 89.78833333333332689 ) ) ;
#62463=CARTESIAN_POINT ( 'NONE',  ( 97.64999999999999147, 90.00000000000002842, 75.07749999999998636 ) ) ;
#62464=CARTESIAN_POINT ( 'NONE',  ( -97.30629616937497417, -208.6684592857803011, 86.41489583420047893 ) ) ;
#62466=CARTESIAN_POINT ( 'NONE',  ( 92.35000000000000853, -209.9999999999999716, 76.66499999999999204 ) ) ;
#62469=CARTESIAN_POINT ( 'NONE',  ( -97.30629616937497417, -208.6684592857803295, 80.06489583420047040 ) ) ;
#62473=CARTESIAN_POINT ( 'NONE',  ( 92.34999999999999432, 90.00000000000002842, 89.36499999999999488 ) ) ;
#62477=ADVANCED_FACE ( 'NONE', ( #56698 ), #39023, .F. ) ;
#62483=CARTESIAN_POINT ( 'NONE',  ( -92.69370383062502583, 88.66845928578038638, 81.65239583420049030 ) ) ;
#62487=CARTESIAN_POINT ( 'NONE',  ( 97.65000000000000568, 88.47002178664752137, 79.54895833506762415 ) ) ;
#62490=CARTESIAN_POINT ( 'NONE',  ( 2.500000000000034639, 90.00000000000000000, -90.00000000000000000 ) ) ;
#62494=CARTESIAN_POINT ( 'NONE',  ( -94.99999999999997158, -207.3369185715606307, 80.11781250086714579 ) ) ;
#62506=DIRECTION ( 'NONE',  ( 1.000000000000000000, 0.000000000000000000, 0.000000000000000000 ) ) ;
#62511=CYLINDRICAL_SURFACE ( 'NONE', #27124, 2.649999999999985700 ) ;
#62513=CARTESIAN_POINT ( 'NONE',  ( 92.69370383062501162, -208.6684592857803295, 88.31989583420048007 ) ) ;
#62530=ORIENTED_EDGE ( 'NONE', *, *, #33712, .F. ) ;
#62531=CARTESIAN_POINT ( 'NONE',  ( 96.32499999999998863, 87.70503267997126784, 87.03666666666666174 ) ) ;
#62532=DIRECTION ( 'NONE',  ( -0.000000000000000000, -0.000000000000000000, 1.000000000000000000 ) ) ;
#62536=ORIENTED_EDGE ( 'NONE', *, *, #20092, .T. ) ;
#62537=CARTESIAN_POINT ( 'NONE',  ( 97.30629616937498838, 90.00000000000002842, 85.51531250086713953 ) ) ;
#62539=CARTESIAN_POINT ( 'NONE',  ( 93.84685191531251292, -211.9973110713294489, 86.57364583420047666 ) ) ;
#62544=DIRECTION ( 'NONE',  ( 0.000000000000000000, 0.000000000000000000, -1.000000000000000000 ) ) ;
#62547=CARTESIAN_POINT ( 'NONE',  ( -92.69370383062498320, -209.9999999999999716, 88.05531250086713158 ) ) ;
#62548=CARTESIAN_POINT ( 'NONE',  ( -93.84685191531254134, 91.99731107132950569, 86.41489583420049314 ) ) ;
#62550=CARTESIAN_POINT ( 'NONE',  ( 92.69370383062498320, 90.00000000000002842, 83.29281250086714294 ) ) ;
#62551=CARTESIAN_POINT ( 'NONE',  ( -97.30629616937501680, 90.00000000000004263, 84.56281250086713897 ) ) ;
#62557=CARTESIAN_POINT ( 'NONE',  ( -93.84685191531247028, -211.9973110713294489, 88.58447916753381435 ) ) ;
#62565=CARTESIAN_POINT ( 'NONE',  ( -97.65000000000001990, 90.00000000000004263, 90.00000000000000000 ) ) ;
#62566=ORIENTED_EDGE ( 'NONE', *, *, #19860, .T. ) ;
#62567=VERTEX_POINT ( 'NONE', #70163 ) ;
#62569=CARTESIAN_POINT ( 'NONE',  ( -96.32500000000001705, 87.70503267997129626, 78.67583333333332973 ) ) ;
#62572=CARTESIAN_POINT ( 'NONE',  ( 97.64999999999821512, -209.9999969335172807, 75.79187510780352000 ) ) ;
#62575=CARTESIAN_POINT ( 'NONE',  ( -97.64997399525483956, 88.47000677280088610, 86.32229270695526679 ) ) ;
#62577=ORIENTED_EDGE ( 'NONE', *, *, #70434, .F. ) ;
#62578=CARTESIAN_POINT ( 'NONE',  ( -95.00000000000002842, 92.66308142843932671, 77.41906250086714181 ) ) ;
#62583=AXIS2_PLACEMENT_3D ( 'NONE', #31823, #26185, #8908 ) ;
#62587=CARTESIAN_POINT ( 'NONE',  ( -97.30629616937497417, -208.6684592857803011, 89.74864583420048803 ) ) ;
#62591=CARTESIAN_POINT ( 'NONE',  ( 96.15314808468748708, 91.99731107132950569, 75.61989583420049144 ) ) ;
#62592=CARTESIAN_POINT ( 'NONE',  ( -96.15314808468747287, -208.0026889286704943, 80.80572916753382628 ) ) ;
#62595=CARTESIAN_POINT ( 'NONE',  ( 97.64999999999999147, -210.0000000207152198, 80.87187500099602744 ) ) ;
#62598=CARTESIAN_POINT ( 'NONE',  ( -92.69370383062505425, 91.33154071421968467, 79.37697916753381833 ) ) ;
#62599=CARTESIAN_POINT ( 'NONE',  ( 92.69370383062501162, -208.6684592857803011, 78.79489583420047438 ) ) ;
#62609=LINE ( 'NONE', #21614, #17742 ) ;
#62610=VECTOR ( 'NONE', #29252, 1000.000000000000000 ) ;
#62615=CARTESIAN_POINT ( 'NONE',  ( 92.69370383062501162, -211.3315407142195852, 76.51947916753381662 ) ) ;
#62620=CARTESIAN_POINT ( 'NONE',  ( 92.69370383062498320, 90.00000000000002842, 84.72156250086715090 ) ) ;
#62622=CARTESIAN_POINT ( 'NONE',  ( 93.67500000000001137, -212.2949673200287179, 78.67583333333332973 ) ) ;
#62631=CARTESIAN_POINT ( 'NONE',  ( 95.00000000000000000, -209.9999999999999716, 90.00000000000000000 ) ) ;
#62634=LINE ( 'NONE', #50198, #55197 ) ;
#62636=VERTEX_POINT ( 'NONE', #35228 ) ;
#62637=CARTESIAN_POINT ( 'NONE',  ( -94.99999999999997158, -206.9400435732949575, 81.03062500173430749 ) ) ;
#62638=VERTEX_POINT ( 'NONE', #64546 ) ;
#62641=CARTESIAN_POINT ( 'NONE',  ( 97.64999999999997726, 88.47002178664753558, 79.54895833506762415 ) ) ;
#62642=CARTESIAN_POINT ( 'NONE',  ( -97.65000000000001990, 88.47002178664754979, 81.24229166840098060 ) ) ;
#62643=( BOUNDED_CURVE ( )  B_SPLINE_CURVE ( 2, ( #68557, #45994, #17045, #39980, #29056, #62935, #11394 ),
 .UNSPECIFIED., .F., .F. ) 
 B_SPLINE_CURVE_WITH_KNOTS ( ( 3, 2, 2, 3 ),
 ( 0.1250000000000002220, 0.1319444444444446418, 0.1388888888888890338, 0.1458333333333334536 ),
 .UNSPECIFIED. ) 
 CURVE ( )  GEOMETRIC_REPRESENTATION_ITEM ( )  RATIONAL_B_SPLINE_CURVE ( ( 0.9999999999999956701, 0.8660254037844430375, 1.000000000000000000, 0.8660254037844387076, 1.000000000000000000, 0.8660254037844365982, 1.000000000000002220 ) ) 
 REPRESENTATION_ITEM ( '' )  );
#62647=CARTESIAN_POINT ( 'NONE',  ( 92.69370383062498320, 91.33154071421968467, 83.39864583420050792 ) ) ;
#62652=CARTESIAN_POINT ( 'NONE',  ( 92.35001469785312622, 91.52998669916200924, 81.77145774807789280 ) ) ;
#62654=VERTEX_POINT ( 'NONE', #2550 ) ;
#62659=EDGE_CURVE ( 'NONE', #48302, #21733, #8879, .T. ) ;
#62661=EDGE_CURVE ( 'NONE', #65748, #65117, #14082, .T. ) ;
#62666=DIRECTION ( 'NONE',  ( -0.000000000000000000, -0.000000000000000000, 1.000000000000000000 ) ) ;
#62667=CARTESIAN_POINT ( 'NONE',  ( -92.69370383062498320, -211.3315407142195852, 80.54114583420049200 ) ) ;
#62669=( BOUNDED_CURVE ( )  B_SPLINE_CURVE ( 2, ( #12069, #465, #11682, #69221, #17708, #10963, #33891 ),
 .UNSPECIFIED., .F., .F. ) 
 B_SPLINE_CURVE_WITH_KNOTS ( ( 3, 2, 2, 3 ),
 ( 0.5926843883826560244, 0.5997400709779450168, 0.6067958365188629299, 0.6138516023217082118 ),
 .UNSPECIFIED. ) 
 CURVE ( )  GEOMETRIC_REPRESENTATION_ITEM ( )  RATIONAL_B_SPLINE_CURVE ( ( 0.9999968501004118382, 0.8660269787527477003, 1.000000000000000000, 0.8660254037844387076, 1.000000000000000000, 0.8660254037844387076, 1.000000000000000000 ) ) 
 REPRESENTATION_ITEM ( '' )  );
#62670=CARTESIAN_POINT ( 'NONE',  ( -95.00000000000002842, 92.66308142843932671, 89.48406250086713953 ) ) ;
#62675=CARTESIAN_POINT ( 'NONE',  ( -95.79297114434442051, -212.5043059285055733, 74.98272308147976162 ) ) ;
#62678=CARTESIAN_POINT ( 'NONE',  ( 93.84685191531248449, 88.00268892867053694, 76.41364583420048007 ) ) ;
#62680=CARTESIAN_POINT ( 'NONE',  ( 92.35001072685618340, 88.47001559349421029, 78.06729209680057124 ) ) ;
#62689=CARTESIAN_POINT ( 'NONE',  ( 97.30629616937498838, 91.33154071421968467, 86.99697916753382287 ) ) ;
#62690=CARTESIAN_POINT ( 'NONE',  ( -93.84685191531248449, -208.0026889286704943, 88.95489583420049939 ) ) ;
#62694=CARTESIAN_POINT ( 'NONE',  ( -95.00000000000002842, 87.33691857156074434, 80.91156250086714863 ) ) ;
#62700=CARTESIAN_POINT ( 'NONE',  ( 95.00000000000000000, -207.3369185715606307, 89.48406250086713953 ) ) ;
#62704=CARTESIAN_POINT ( 'NONE',  ( 92.34999999999999432, 90.00000000000002842, 83.01499999999998636 ) ) ;
#62706=ADVANCED_FACE ( 'NONE', ( #19039 ), #60761, .T. ) ;
#62707=CARTESIAN_POINT ( 'NONE',  ( 92.35004149090323722, -211.5300021681365763, 85.68729332542764610 ) ) ;
#62708=CARTESIAN_POINT ( 'NONE',  ( 97.64999999999999147, 90.00000000000002842, 90.00000000000000000 ) ) ;
#62711=CARTESIAN_POINT ( 'NONE',  ( 94.99999999999998579, 90.00000000000002842, 90.00000000000000000 ) ) ;
#62713=FACE_OUTER_BOUND ( 'NONE', #13702, .T. ) ;
#62716=CARTESIAN_POINT ( 'NONE',  ( 97.64999999999997726, -208.4700217866474645, 86.56041666666665435 ) ) ;
#62721=CARTESIAN_POINT ( 'NONE',  ( -97.64999999947052345, 90.00003365185393989, 81.18829462297244959 ) ) ;
#62728=CARTESIAN_POINT ( 'NONE',  ( 93.67500000000001137, -207.7050326799711968, 77.27354166840096639 ) ) ;
#62729=CARTESIAN_POINT ( 'NONE',  ( 96.32499999999998863, 87.70503267997126784, 80.68666666666665321 ) ) ;
#62731=CYLINDRICAL_SURFACE ( 'NONE', #20313, 2.649999999999999467 ) ;
#62734=CARTESIAN_POINT ( 'NONE',  ( 92.34999999999999432, 90.00000000000002842, 90.00000000000000000 ) ) ;
#62736=DIRECTION ( 'NONE',  ( 0.000000000000000000, -0.000000000000000000, -1.000000000000000000 ) ) ;
#62738=CARTESIAN_POINT ( 'NONE',  ( -96.15314808468752972, 91.99731107132950569, 80.80572916753382628 ) ) ;
#62739=CARTESIAN_POINT ( 'NONE',  ( 92.69370383062498320, 90.00000000000002842, 76.94281250086713442 ) ) ;
#62749=AXIS2_PLACEMENT_3D ( 'NONE', #47179, #41533, #64471 ) ;
#62750=CARTESIAN_POINT ( 'NONE',  ( -97.30629616937497417, -208.6684592857803011, 76.25489583420049655 ) ) ;
#62752=EDGE_CURVE ( 'NONE', #69024, #52406, #1187, .T. ) ;
#62754=DIRECTION ( 'NONE',  ( 0.000000000000000000, -1.000000000000000000, 0.000000000000000000 ) ) ;
#62759=DIRECTION ( 'NONE',  ( 0.000000000000000000, -0.000000000000000000, -1.000000000000000000 ) ) ;
#62761=CARTESIAN_POINT ( 'NONE',  ( -97.30629616937495996, -209.9999999999999716, 77.57781250086713953 ) ) ;
#62765=CARTESIAN_POINT ( 'NONE',  ( -94.95306897617061281, -212.6495843973424655, 75.00000002508416230 ) ) ;
#62766=CARTESIAN_POINT ( 'NONE',  ( 96.32499999999998863, -207.7050326799711968, 81.53333333333333144 ) ) ;
#62768=CARTESIAN_POINT ( 'NONE',  ( 92.35000000019411459, -210.0000198427945861, 86.27002759516706476 ) ) ;
#62770=CARTESIAN_POINT ( 'NONE',  ( 97.30629616937498838, 90.00000000000002842, 85.51531250086713953 ) ) ;
#62774=CARTESIAN_POINT ( 'NONE',  ( -2.500000000000015543, -73.00000000000001421, -255.0000000000000000 ) ) ;
#62784=EDGE_CURVE ( 'NONE', #41411, #72954, #8827, .T. ) ;
#62788=CARTESIAN_POINT ( 'NONE',  ( -93.67499999999998295, -207.7050326799711968, 84.07333333333333769 ) ) ;
#62790=CARTESIAN_POINT ( 'NONE',  ( -97.65000000000006253, 88.47002178664756400, 79.89291666666666458 ) ) ;
#62792=ORIENTED_EDGE ( 'NONE', *, *, #72144, .F. ) ;
#62799=CARTESIAN_POINT ( 'NONE',  ( 92.69370383062501162, -209.9999999999999716, 84.72156250086715090 ) ) ;
#62800=EDGE_LOOP ( 'NONE', ( #69784, #17768, #41174, #23295 ) ) ;
#62803=ORIENTED_EDGE ( 'NONE', *, *, #35702, .F. ) ;
#62805=CARTESIAN_POINT ( 'NONE',  ( 92.69370383062501162, -211.3315407142195852, 78.26572916753380582 ) ) ;
#62807=CARTESIAN_POINT ( 'NONE',  ( 97.30629616937498838, -211.3315407142195852, 83.71614583420050337 ) ) ;
#62816=CARTESIAN_POINT ( 'NONE',  ( 92.35000000000002274, -211.5299782133524502, 87.59229166840096070 ) ) ;
#62820=CARTESIAN_POINT ( 'NONE',  ( -96.15314808468752972, 91.99731107132950569, 89.69572916753382685 ) ) ;
#62824=EDGE_CURVE ( 'NONE', #44809, #2269, #61025, .T. ) ;
#62832=ORIENTED_EDGE ( 'NONE', *, *, #243, .T. ) ;
#62838=CARTESIAN_POINT ( 'NONE',  ( -97.30629616937501680, 90.00000000000004263, 75.83156250086716454 ) ) ;
#62840=CARTESIAN_POINT ( 'NONE',  ( 92.69370383062498320, 91.33154071421968467, 74.98489583420048632 ) ) ;
#62844=CARTESIAN_POINT ( 'NONE',  ( -96.15314808468745866, -211.9973110713294489, 84.66864583420047552 ) ) ;
#62846=ORIENTED_EDGE ( 'NONE', *, *, #29189, .F. ) ;
#62849=CARTESIAN_POINT ( 'NONE',  ( 93.08933536981351153, -211.7387787020258259, 74.95660481729454716 ) ) ;
#62850=CARTESIAN_POINT ( 'NONE',  ( 96.32499999999998863, -207.7050326799711968, 87.88333333333332575 ) ) ;
#62851=CARTESIAN_POINT ( 'NONE',  ( -94.99999999999997158, -207.3369185715606307, 76.14906250086716000 ) ) ;
#62856=CARTESIAN_POINT ( 'NONE',  ( -97.64999999996712177, 90.00000839536629371, 84.99910573348492449 ) ) ;
#62861=CARTESIAN_POINT ( 'NONE',  ( -93.84685191531254134, 91.99731107132950569, 79.90614583420047268 ) ) ;
#62865=CARTESIAN_POINT ( 'NONE',  ( 92.34999999999999432, 88.47002178664752137, 79.33729166840096525 ) ) ;
#62872=CARTESIAN_POINT ( 'NONE',  ( -95.00000000000002842, 93.05995642670504253, 85.47562500173430067 ) ) ;
#62873=CARTESIAN_POINT ( 'NONE',  ( -96.15314808468747287, -208.0026889286704943, 80.17072916753382117 ) ) ;
#62874=CARTESIAN_POINT ( 'NONE',  ( -95.00000000000002842, 90.00000000000004263, 90.00000000000000000 ) ) ;
#62876=( BOUNDED_CURVE ( )  B_SPLINE_CURVE ( 2, ( #64176, #69071, #69429, #57419, #47246, #5930, #52886 ),
 .UNSPECIFIED., .F., .F. ) 
 B_SPLINE_CURVE_WITH_KNOTS ( ( 3, 2, 2, 3 ),
 ( 0.4583333333333335924, 0.4652777777777780122, 0.4722222222222224319, 0.4791666666666668517 ),
 .UNSPECIFIED. ) 
 CURVE ( )  GEOMETRIC_REPRESENTATION_ITEM ( )  RATIONAL_B_SPLINE_CURVE ( ( 0.9999999999999946709, 0.8660254037844440367, 1.000000000000000000, 0.8660254037844387076, 1.000000000000000000, 0.8660254037844354880, 1.000000000000003109 ) ) 
 REPRESENTATION_ITEM ( '' )  );
#62879=DIRECTION ( 'NONE',  ( -0.000000000000000000, -0.000000000000000000, 1.000000000000000000 ) ) ;
#62885=ORIENTED_EDGE ( 'NONE', *, *, #11183, .T. ) ;
#62890=CARTESIAN_POINT ( 'NONE',  ( 93.84685191531249870, -208.0026889286704943, 86.99697916753380866 ) ) ;
#62891=CARTESIAN_POINT ( 'NONE',  ( -97.64999999999996305, -209.9999999999999716, 83.72937500173429726 ) ) ;
#62897=ORIENTED_EDGE ( 'NONE', *, *, #66902, .F. ) ;
#62899=CARTESIAN_POINT ( 'NONE',  ( 95.00000000000000000, -213.0599564267049857, 85.15812500173429100 ) ) ;
#62902=CARTESIAN_POINT ( 'NONE',  ( -92.34999999999999432, -210.0000000983656605, 80.23687499810813506 ) ) ;
#62911=ORIENTED_EDGE ( 'NONE', *, *, #7906, .F. ) ;
#62918=CARTESIAN_POINT ( 'NONE',  ( 97.30629616937498838, 88.66845928578037217, 83.55739583420047722 ) ) ;
#62920=CARTESIAN_POINT ( 'NONE',  ( 96.15314808468748708, -208.0026889286704943, 85.62114583420046188 ) ) ;
#62922=CARTESIAN_POINT ( 'NONE',  ( -96.32499999999996021, -207.7050326799711968, 76.55916666666666970 ) ) ;
#62923=CARTESIAN_POINT ( 'NONE',  ( -97.64999999999996305, -209.9999999999999716, 83.01499999999998636 ) ) ;
#62928=CARTESIAN_POINT ( 'NONE',  ( -94.99999999999997158, -212.6630814284392557, 87.89656250086713385 ) ) ;
#62929=CARTESIAN_POINT ( 'NONE',  ( -93.84685191531252713, 88.00268892867056536, 86.20322916753382003 ) ) ;
#62932=CARTESIAN_POINT ( 'NONE',  ( 97.30629616937498838, 91.33154071421968467, 83.66322916753379957 ) ) ;
#62933=CARTESIAN_POINT ( 'NONE',  ( -93.84685191531254134, 91.99731107132950569, 83.71614583420047495 ) ) ;
#62935=CARTESIAN_POINT ( 'NONE',  ( -92.35000000000000853, 91.52997821335252127, 87.83041666666669300 ) ) ;
#62937=CARTESIAN_POINT ( 'NONE',  ( 92.35000000006147047, -209.9999881782113107, 76.10900611559200968 ) ) ;
#62939=DIRECTION ( 'NONE',  ( -0.000000000000000000, -0.000000000000000000, 1.000000000000000000 ) ) ;
#62940=CARTESIAN_POINT ( 'NONE',  ( -97.30629616937497417, -208.6684592857803295, 87.04989583420046984 ) ) ;
#62942=CARTESIAN_POINT ( 'NONE',  ( 93.67500000000001137, -207.7050326799711968, 82.27416666666665890 ) ) ;
#62943=DIRECTION ( 'NONE',  ( -0.000000000000000000, -0.000000000000000000, 1.000000000000000000 ) ) ;
#62948=CARTESIAN_POINT ( 'NONE',  ( -97.65000000000001990, 90.00000000000004263, 76.66499999999999204 ) ) ;
#62949=EDGE_CURVE ( 'NONE', #70635, #70258, #38267, .T. ) ;
#62953=CARTESIAN_POINT ( 'NONE',  ( -96.32499999999996021, -212.2949673200287179, 76.85020833506763438 ) ) ;
#62961=CARTESIAN_POINT ( 'NONE',  ( -97.30629616937501680, 91.33154071421968467, 77.52489583420046415 ) ) ;
#62966=CYLINDRICAL_SURFACE ( 'NONE', #40485, 2.649999999999985700 ) ;
#62967=CARTESIAN_POINT ( 'NONE',  ( -97.64999999994218172, 89.99998877583867340, 75.47473230081648410 ) ) ;
#62968=LINE ( 'NONE', #22343, #62240 ) ;
#62969=CARTESIAN_POINT ( 'NONE',  ( 92.69370383062498320, 91.33154071421968467, 78.31864583420050963 ) ) ;
#62971=CARTESIAN_POINT ( 'NONE',  ( -97.30629616937497417, -211.3315407142195852, 78.42447916753380355 ) ) ;
#62974=CARTESIAN_POINT ( 'NONE',  ( 96.32499999999998863, -207.7050326799711968, 80.97770833506763211 ) ) ;
#62978=CARTESIAN_POINT ( 'NONE',  ( 92.69370383062501162, -209.9999999999999716, 81.38781250086714181 ) ) ;
#62983=ORIENTED_EDGE ( 'NONE', *, *, #63245, .T. ) ;
#62985=ORIENTED_EDGE ( 'NONE', *, *, #40937, .T. ) ;
#62986=CYLINDRICAL_SURFACE ( 'NONE', #44213, 2.649999999999999467 ) ;
#62988=ORIENTED_EDGE ( 'NONE', *, *, #50593, .F. ) ;
#62991=ORIENTED_EDGE ( 'NONE', *, *, #56366, .F. ) ;
#62997=CARTESIAN_POINT ( 'NONE',  ( 94.99999999999998579, 87.33691857156068750, 81.70531250086715147 ) ) ;
#62999=CARTESIAN_POINT ( 'NONE',  ( 95.00000000000000000, -213.0599564267049857, 77.45874999999999488 ) ) ;
#63010=CARTESIAN_POINT ( 'NONE',  ( -93.25528180581933668, 88.31889241252943634, 74.86350982016035971 ) ) ;
#63014=FACE_OUTER_BOUND ( 'NONE', #43394, .T. ) ;
#63016=CARTESIAN_POINT ( 'NONE',  ( -93.67499999999998295, -207.7050326799711968, 82.24770833506762813 ) ) ;
#63021=CARTESIAN_POINT ( 'NONE',  ( 97.64999999999999147, 90.00000000000002842, 80.23687500173429044 ) ) ;
#63022=CARTESIAN_POINT ( 'NONE',  ( -92.35000000000003695, 90.00000000000004263, 78.33187500173430351 ) ) ;
#63024=CARTESIAN_POINT ( 'NONE',  ( 93.84685191531248449, 91.99731107132950569, 79.53572916753381605 ) ) ;
#63031=CARTESIAN_POINT ( 'NONE',  ( -92.34999999999998010, -209.9999999999999716, 75.00000000000000000 ) ) ;
#63039=DIRECTION ( 'NONE',  ( 1.000000000000000000, 0.000000000000000000, 0.000000000000000000 ) ) ;
#63040=CARTESIAN_POINT ( 'NONE',  ( 92.35000000000000853, -209.9999999999999716, 90.00000000000000000 ) ) ;
#63041=CARTESIAN_POINT ( 'NONE',  ( -96.15314808468745866, -211.9973110713294489, 82.28739583420048120 ) ) ;
#63046=DIRECTION ( 'NONE',  ( 1.000000000000000000, 0.000000000000000000, 0.000000000000000000 ) ) ;
#63048=CARTESIAN_POINT ( 'NONE',  ( 92.69370383062498320, 91.33154071421968467, 75.61989583420047722 ) ) ;
#63052=FACE_OUTER_BOUND ( 'NONE', #53158, .T. ) ;
#63056=AXIS2_PLACEMENT_3D ( 'NONE', #48914, #15443, #33098 ) ;
#63057=CARTESIAN_POINT ( 'NONE',  ( 97.30629616937498838, 91.33154071421968467, 85.72697916753381264 ) ) ;
#63058=CARTESIAN_POINT ( 'NONE',  ( -94.99999999999997158, -207.3369185715606307, 88.37281250086715545 ) ) ;
#63059=CARTESIAN_POINT ( 'NONE',  ( 92.34999999999999432, 88.47002178664752137, 82.43291666666665662 ) ) ;
#63062=CARTESIAN_POINT ( 'NONE',  ( -95.00000000000002842, 92.66308142843932671, 78.05406250086714692 ) ) ;
#63073=CARTESIAN_POINT ( 'NONE',  ( 93.84685191531249870, -208.0026889286704943, 76.99572916753382401 ) ) ;
#63076=EDGE_CURVE ( 'NONE', #73949, #69471, #54652, .T. ) ;
#63078=CARTESIAN_POINT ( 'NONE',  ( 96.15314808468748708, -208.0026889286704943, 85.14489583420048291 ) ) ;
#63081=( BOUNDED_CURVE ( )  B_SPLINE_CURVE ( 2, ( #14655, #51008, #68308, #73931, #31941, #22442, #3405, #26306, #33322, #45385, #31206, #49238, #21686, #44642, #2688, #25569, #52113, #57391, #69771, #293, #23548, #58126, #28817, #40851, #52476, #35561, #46477, #69400, #40102, #6627, #11516, #23187, #5905, #63785, #70131, #1025, #58491, #6986, #34448, #29538, #18273, #29909, #39741, #51746, #28437, #45759, #68684, #23917, #34833, #35193, #17900, #52862, #46859, #62689, #11160, #47221, #34082, #46114, #57028, #5538, #12623, #12260, #11880, #51369, #41210, #69049, #64148, #74306, #17533, #57765, #1400, #40463, #63410, #24294, #22821, #17169, #6271, #63057, #29169, #655, #25399, #31761, #8098, #14478, #2867, #24653, #2133, #48690, #41953, #1766, #71613, #3233, #31019, #7368, #59615, #8479, #42688, #70876, #54344, #53594, #64891, #2517, #19375, #26123, #53973, #25761, #14098, #37046, #48326, #65627, #20111, #37430, #7733, #70488, #30648, #59994, #36669, #18632, #59240, #30285, #65259, #25015, #31392, #41571, #71235, #47958, #43070, #66004, #42326, #19740, #60362, #8846, #54704, #49058, #64512, #12988, #13731, #35926, #58876, #53230, #47584, #18999, #13365, #36298, #61836, #21593, #49789, #33236, #32505, #43812, #67841, #56188, #66370, #21971, #44920, #27611, #50540, #61466, #38529, #15959, #72359, #60729, #16333, #44169, #66729, #9584, #55445, #27974, #3602, #4706, #72709, #44548, #9207, #67466, #61087, #39275, #5075, #10690, #15219, #73463, #3964, #67090, #62204, #55817, #32126, #33619, #38150, #56576, #71984, #26862, #15593, #38898, #55068, #10319, #21215, #20499, #9946, #73089, #43450, #14849, #4330, #37796, #26502, #49430, #32867, #27223, #20855, #50157, #22347, #51658, #205, #63323, #6903, #50911, #33993, #41128, #73835, #62969, #39646, #56939, #5447, #23098, #28344, #57681, #22729, #34359, #57303, #23826, #64062, #58403, #34737, #63696, #35472, #29445, #18184, #51280, #12535, #40372, #46766, #35107, #74214, #11425, #46029, #52388, #12169, #45296, #5813, #566, #17081, #23460, #45668, #46389, #936, #68594, #69315, #68215, #6184, #11786, #40016, #16707, #68958, #69687, #29081, #17444, #17807, #28719, #52018, #40755, #62591, #58036, #6542, #11070, #70044, #65913, #20019, #41482, #71146, #30562, #65169, #2421, #53138, #37336, #42975, #24566, #59902, #13278, #12901 ),
 .UNSPECIFIED., .F., .F. ) 
 B_SPLINE_CURVE_WITH_KNOTS ( ( 3, 2, 2, 2, 2, 2, 2, 2, 2, 2, 2, 2, 2, 2, 2, 2, 2, 2, 2, 2, 2, 2, 2, 2, 2, 2, 2, 2, 2, 2, 2, 2, 2, 2, 2, 2, 2, 2, 2, 2, 2, 2, 2, 2, 2, 2, 2, 2, 2, 2, 2, 2, 2, 2, 2, 2, 2, 2, 2, 2, 2, 2, 2, 2, 2, 2, 2, 2, 2, 2, 2, 2, 2, 2, 2, 2, 2, 2, 2, 2, 2, 2, 2, 2, 2, 2, 2, 2, 2, 2, 2, 2, 2, 2, 2, 2, 2, 2, 2, 2, 2, 2, 2, 2, 2, 2, 2, 2, 2, 2, 2, 2, 2, 2, 2, 2, 2, 2, 2, 2, 2, 2, 2, 2, 2, 2, 2, 2, 2, 2, 2, 2, 2, 2, 2, 2, 2, 2, 2, 2, 2, 2, 2, 3 ),
 ( 0.000000000000000000, 0.007055764916269564521, 0.01411152983253912904, 0.02116729474880869530, 0.02822305966507825808, 0.03527882458134782434, 0.04233458949761739060, 0.04939035441388695685, 0.05644611933015651617, 0.06350188424642608243, 0.07055764916269564868, 0.07761341407896522882, 0.08466917899523478119, 0.09172494391150434745, 0.09878070882777391370, 0.1058364737440434800, 0.1128922386603130323, 0.1199480035765825986, 0.1270037684928521649, 0.1340595334091217450, 0.1411152983253912974, 0.1481710632416608775, 0.1552268281579304576, 0.1622825930741999823, 0.1693383579904695624, 0.1763941229067391148, 0.1834498878230086949, 0.1905056527392782473, 0.1975614176555478274, 0.2046171825718174075, 0.2116729474880869599, 0.2187287124043565401, 0.2257844773206260647, 0.2328402422368956448, 0.2398960071531651972, 0.2469517720694347773, 0.2540075369857043297, 0.2610633019019739098, 0.2681190668182434900, 0.2751748317345130146, 0.2822305966507825947, 0.2892863615670521749, 0.2963421264833217550, 0.3033978913995912796, 0.3104536563158609153, 0.3175094212321304399, 0.3245651861483999645, 0.3316209510646695446, 0.3386767159809391248, 0.3457324808972087049, 0.3527882458134782295, 0.3598440107297478652, 0.3668997756460173898, 0.3739555405622869699, 0.3810113054785564946, 0.3880670703948260747, 0.3951228353110956548, 0.4021786002273651794, 0.4092343651436348151, 0.4162901300599043397, 0.4233458949761739198, 0.4304016598924434445, 0.4374574248087130801, 0.4445131897249826047, 0.4515689546412521294, 0.4586247195575217650, 0.4656804844737912896, 0.4727362493900608698, 0.4797920143063303944, 0.4868477792226000300, 0.4939035441388695546, 0.5009593090551391903, 0.5080150739714086594, 0.5150708388876782395, 0.5221266038039478197, 0.5291823687202173998, 0.5362381336364869799, 0.5432938985527564490, 0.5503496634690260292, 0.5574054283852957203, 0.5644611933015651895, 0.5715169582178347696, 0.5785727231341043497, 0.5856284880503738188, 0.5926842529666435100, 0.5997400178829130901, 0.6067957827991825592, 0.6138515477154521394, 0.6209073126317218305, 0.6279630775479912996, 0.6350188424642608798, 0.6420746073805303489, 0.6491303722967999290, 0.6561861372130696202, 0.6632419021293390893, 0.6702976670456086694, 0.6773534319618782495, 0.6844091968781478297, 0.6914649617944174098, 0.6985207267106869899, 0.7055764916269564591, 0.7126322565432260392, 0.7196880214594957303, 0.7267437863757651995, 0.7337995512920347796, 0.7408553162083042487, 0.7479110811245739399, 0.7549668460408435200, 0.7620226109571129891, 0.7690783758733825692, 0.7761341407896521494, 0.7831899057059217295, 0.7902456706221913096, 0.7973014355384608898, 0.8043572004547303589, 0.8114129653710000500, 0.8184687302872696302, 0.8255244952035390993, 0.8325802601198086794, 0.8396360250360781485, 0.8466917899523478397, 0.8537475548686174198, 0.8608033197848868889, 0.8678590847011564691, 0.8749148496174261602, 0.8819706145336956293, 0.8890263794499652095, 0.8960821443662347896, 0.9031379092825042587, 0.9101936741987739499, 0.9172494391150435300, 0.9243052040313129991, 0.9313609689475825792, 0.9384167338638521594, 0.9454724987801217395, 0.9525282636963913196, 0.9595840286126607888, 0.9666397935289303689, 0.9736955584452000600, 0.9807513233614695292, 0.9878070882777391093, 0.9948628531940086894, 0.9999999123559569769, 1.000000000000000000 ),
 .UNSPECIFIED. ) 
 CURVE ( )  GEOMETRIC_REPRESENTATION_ITEM ( )  RATIONAL_B_SPLINE_CURVE ( ( 1.000000000000000000, 0.8660254037844387076, 1.000000000000000000, 0.8660254037844387076, 1.000000000000000000, 0.8660254037844387076, 1.000000000000000000, 0.8660254037844387076, 1.000000000000000000, 0.8660254037844387076, 1.000000000000000000, 0.8660254037844387076, 1.000000000000000000, 0.8660254037844387076, 1.000000000000000000, 0.8660254037844387076, 1.000000000000000000, 0.8660254037844387076, 1.000000000000000000, 0.8660254037844387076, 1.000000000000000000, 0.8660254037844387076, 1.000000000000000000, 0.8660254037844387076, 1.000000000000000000, 0.8660254037844387076, 1.000000000000000000, 0.8660254037844387076, 1.000000000000000000, 0.8660254037844387076, 1.000000000000000000, 0.8660254037844387076, 1.000000000000000000, 0.8660254037844387076, 1.000000000000000000, 0.8660254037844387076, 1.000000000000000000, 0.8660254037844387076, 1.000000000000000000, 0.8660254037844387076, 1.000000000000000000, 0.8660254037844387076, 1.000000000000000000, 0.8660254037844387076, 1.000000000000000000, 0.8660254037844387076, 1.000000000000000000, 0.8660254037844387076, 1.000000000000000000, 0.8660254037844387076, 1.000000000000000000, 0.8660254037844387076, 1.000000000000000000, 0.8660254037844387076, 1.000000000000000000, 0.8660254037844387076, 1.000000000000000000, 0.8660254037844387076, 1.000000000000000000, 0.8660254037844387076, 1.000000000000000000, 0.8660254037844387076, 1.000000000000000000, 0.8660254037844387076, 1.000000000000000000, 0.8660254037844387076, 1.000000000000000000, 0.8660254037844387076, 1.000000000000000000, 0.8660254037844387076, 1.000000000000000000, 0.8660254037844387076, 1.000000000000000000, 0.8660254037844387076, 1.000000000000000000, 0.8660254037844387076, 1.000000000000000000, 0.8660254037844387076, 1.000000000000000000, 0.8660254037844387076, 1.000000000000000000, 0.8660254037844387076, 1.000000000000000000, 0.8660254037844387076, 1.000000000000000000, 0.8660254037844387076, 1.000000000000000000, 0.8660254037844387076, 1.000000000000000000, 0.8660254037844387076, 1.000000000000000000, 0.8660254037844387076, 1.000000000000000000, 0.8660254037844387076, 1.000000000000000000, 0.8660254037844387076, 1.000000000000000000, 0.8660254037844387076, 1.000000000000000000, 0.8660254037844387076, 1.000000000000000000, 0.8660254037844387076, 1.000000000000000000, 0.8660254037844387076, 1.000000000000000000, 0.8660254037844387076, 1.000000000000000000, 0.8660254037844387076, 1.000000000000000000, 0.8660254037844387076, 1.000000000000000000, 0.8660254037844387076, 1.000000000000000000, 0.8660254037844387076, 1.000000000000000000, 0.8660254037844387076, 1.000000000000000000, 0.8660254037844387076, 1.000000000000000000, 0.8660254037844387076, 1.000000000000000000, 0.8660254037844387076, 1.000000000000000000, 0.8660254037844387076, 1.000000000000000000, 0.8660254037844387076, 1.000000000000000000, 0.8660254037844387076, 1.000000000000000000, 0.8660254037844387076, 1.000000000000000000, 0.8660254037844387076, 1.000000000000000000, 0.8660254037844387076, 1.000000000000000000, 0.8660254037844387076, 1.000000000000000000, 0.8660254037844387076, 1.000000000000000000, 0.8660254037844387076, 1.000000000000000000, 0.8660254037844387076, 1.000000000000000000, 0.8660254037844387076, 1.000000000000000000, 0.8660254037844387076, 1.000000000000000000, 0.8660254037844387076, 1.000000000000000000, 0.8660254037844387076, 1.000000000000000000, 0.8660254037844387076, 1.000000000000000000, 0.8660254037844387076, 1.000000000000000000, 0.8660254037844387076, 1.000000000000000000, 0.8660254037844387076, 1.000000000000000000, 0.8660254037844387076, 1.000000000000000000, 0.8660254037844387076, 1.000000000000000000, 0.8660254037844387076, 1.000000000000000000, 0.8660254037844387076, 1.000000000000000000, 0.8660254037844387076, 1.000000000000000000, 0.8660254037844387076, 1.000000000000000000, 0.8660254037844387076, 1.000000000000000000, 0.8660254037844387076, 1.000000000000000000, 0.8660254037844387076, 1.000000000000000000, 0.8660254037844387076, 1.000000000000000000, 0.8660254037844387076, 1.000000000000000000, 0.8660254037844387076, 1.000000000000000000, 0.8660254037844387076, 1.000000000000000000, 0.8660254037844387076, 1.000000000000000000, 0.8660254037844387076, 1.000000000000000000, 0.8660254037844387076, 1.000000000000000000, 0.8660254037844387076, 1.000000000000000000, 0.8660254037844387076, 1.000000000000000000, 0.8660254037844387076, 1.000000000000000000, 0.8660254037844387076, 1.000000000000000000, 0.8660254037844387076, 1.000000000000000000, 0.8660254037844387076, 1.000000000000000000, 0.8660254037844387076, 1.000000000000000000, 0.8660254037844387076, 1.000000000000000000, 0.8660254037844387076, 1.000000000000000000, 0.8660254037844387076, 1.000000000000000000, 0.8660254037844387076, 1.000000000000000000, 0.8660254037844387076, 1.000000000000000000, 0.8660254037844387076, 1.000000000000000000, 0.8660254037844387076, 1.000000000000000000, 0.8660254037844387076, 1.000000000000000000, 0.8660254037844387076, 1.000000000000000000, 0.8660254037844387076, 1.000000000000000000, 0.8660254037844387076, 1.000000000000000000, 0.8660254037844387076, 1.000000000000000000, 0.8660254037844387076, 1.000000000000000000, 0.8660254037844387076, 1.000000000000000000, 0.8660254037844387076, 1.000000000000000000, 0.8660254037844387076, 1.000000000000000000, 0.8660254037844387076, 1.000000000000000000, 0.8660254037844387076, 1.000000000000000000, 0.8660254037844387076, 1.000000000000000000, 0.8660254037844387076, 1.000000000000000000, 0.8660254037844387076, 1.000000000000000000, 0.8660254037844387076, 1.000000000000000000, 0.8660254037844387076, 1.000000000000000000, 0.8660254037844387076, 1.000000000000000000, 0.8660254037844387076, 1.000000000000000000, 0.8660254037844387076, 1.000000000000000000, 0.8660254037844387076, 1.000000000000000000, 0.8660254037844387076, 1.000000000000000000, 0.8660254037844387076, 1.000000000000000000, 0.8660254037844387076, 1.000000000000000000, 0.8660254037844387076, 1.000000000000000000, 0.8660254037844387076, 1.000000000000000000, 0.8660254037844387076, 1.000000000000000000, 0.8660254037844387076, 1.000000000000000000, 0.8660254037844387076, 1.000000000000000000, 0.8660254037844387076, 1.000000000000000000, 0.8660254037844387076, 1.000000000000000000, 0.8660254037844387076, 1.000000000000000000, 0.8660254037844387076, 1.000000000000000000, 0.9024577157650908177, 0.9469497795711379062, 0.9469497795711379062, 0.9469497795711379062 ) ) 
 REPRESENTATION_ITEM ( '' )  );
#63085=CARTESIAN_POINT ( 'NONE',  ( 97.64999999999997726, -211.5299782133524502, 88.99458333333333826 ) ) ;
#63086=ORIENTED_EDGE ( 'NONE', *, *, #61731, .F. ) ;
#63096=CARTESIAN_POINT ( 'NONE',  ( 97.64999999999997726, -211.5299782133524502, 76.37395833506761278 ) ) ;
#63097=CARTESIAN_POINT ( 'NONE',  ( 93.67499999999998295, 92.29496732002878900, 79.09916666666666174 ) ) ;
#63102=EDGE_CURVE ( 'NONE', #71746, #27263, #42637, .T. ) ;
#63104=FACE_OUTER_BOUND ( 'NONE', #22382, .T. ) ;
#63105=CARTESIAN_POINT ( 'NONE',  ( -97.30629616937501680, 91.33154071421968467, 81.49364583420049257 ) ) ;
#63106=CARTESIAN_POINT ( 'NONE',  ( 92.69370383062498320, 91.33154071421968467, 78.15989583420048348 ) ) ;
#63109=ORIENTED_EDGE ( 'NONE', *, *, #58720, .F. ) ;
#63112=CARTESIAN_POINT ( 'NONE',  ( -96.32499999999996021, -207.7050326799711968, 77.82916666666665151 ) ) ;
#63115=EDGE_CURVE ( 'NONE', #44409, #41316, #15458, .T. ) ;
#63117=CARTESIAN_POINT ( 'NONE',  ( -92.69370383062498320, -211.3315407142195852, 76.57239583420046358 ) ) ;
#63127=CARTESIAN_POINT ( 'NONE',  ( -94.99999999999997158, -212.6630814284392557, 77.10156250086711793 ) ) ;
#63128=VERTEX_POINT ( 'NONE', #20058 ) ;
#63131=CARTESIAN_POINT ( 'NONE',  ( 97.64999999999999147, -209.9999999999999716, 81.42749999999999488 ) ) ;
#63135=CARTESIAN_POINT ( 'NONE',  ( -95.00000000000002842, 93.05995642670504253, 83.57062500173429953 ) ) ;
#63137=CARTESIAN_POINT ( 'NONE',  ( 93.84685191531248449, 88.00268892867053694, 85.30364583420046642 ) ) ;
#63145=CARTESIAN_POINT ( 'NONE',  ( -93.84685191531252713, 88.00268892867056536, 88.58447916753381435 ) ) ;
#63146=DIRECTION ( 'NONE',  ( -0.000000000000000000, -0.000000000000000000, 1.000000000000000000 ) ) ;
#63147=CARTESIAN_POINT ( 'NONE',  ( 92.34999999999993747, 88.47002178664756400, 85.60791666666665378 ) ) ;
#63155=CARTESIAN_POINT ( 'NONE',  ( 95.00000000000000000, -207.3369185715606307, 83.92781250086716227 ) ) ;
#63167=CARTESIAN_POINT ( 'NONE',  ( 93.84685191531251292, -211.9973110713294489, 77.04864583420047097 ) ) ;
#63169=CARTESIAN_POINT ( 'NONE',  ( 97.30629616937498838, -209.9999999999999716, 84.40406250086715545 ) ) ;
#63172=ORIENTED_EDGE ( 'NONE', *, *, #4457, .F. ) ;
#63175=VECTOR ( 'NONE', #33825, 1000.000000000000000 ) ;
#63179=CARTESIAN_POINT ( 'NONE',  ( 95.00000000000000000, -206.9400435732949575, 88.01562500173429271 ) ) ;
#63185=VERTEX_POINT ( 'NONE', #73411 ) ;
#63189=ADVANCED_FACE ( 'NONE', ( #9154 ), #16511, .F. ) ;
#63197=CARTESIAN_POINT ( 'NONE',  ( -92.35000000000003695, 90.00000000000004263, 86.50750000000000739 ) ) ;
#63202=DIRECTION ( 'NONE',  ( 1.000000000000000000, 0.000000000000000000, 0.000000000000000000 ) ) ;
#63203=CARTESIAN_POINT ( 'NONE',  ( -97.30629616937497417, -211.3315407142195852, 87.79072916753381151 ) ) ;
#63209=CARTESIAN_POINT ( 'NONE',  ( -93.84685191531248449, -208.0026889286704943, 76.73114583420047552 ) ) ;
#63212=CIRCLE ( 'NONE', #48792, 3.299999999999983391 ) ;
#63216=CARTESIAN_POINT ( 'NONE',  ( 96.32499999999998863, 87.70503267997126784, 80.13104166840095388 ) ) ;
#63217=CARTESIAN_POINT ( 'NONE',  ( -97.30629616937501680, 90.00000000000004263, 77.57781250086713953 ) ) ;
#63219=CARTESIAN_POINT ( 'NONE',  ( 12.75000000000000000, -120.0000000000000000, 127.5000000000000000 ) ) ;
#63222=EDGE_LOOP ( 'NONE', ( #33395, #9278, #31328, #48171 ) ) ;
#63229=CARTESIAN_POINT ( 'NONE',  ( -97.64999999950704535, 89.99996796756893502, 85.63541623677065218 ) ) ;
#63230=CARTESIAN_POINT ( 'NONE',  ( -97.64999999999996305, -209.9999999999999716, 90.00000000000000000 ) ) ;
#63234=CARTESIAN_POINT ( 'NONE',  ( -93.67500000000003979, 87.70503267997129626, 80.76604166840097321 ) ) ;
#63243=LINE ( 'NONE', #17728, #36689 ) ;
#63244=ORIENTED_EDGE ( 'NONE', *, *, #47311, .F. ) ;
#63245=EDGE_CURVE ( 'NONE', #15433, #10724, #57353, .T. ) ;
#63246=CARTESIAN_POINT ( 'NONE',  ( 95.00000000000000000, -212.6630814284392557, 89.16656250086712987 ) ) ;
#63249=CARTESIAN_POINT ( 'NONE',  ( -97.64999999980591383, 89.99998015682162134, 84.36502760998403971 ) ) ;
#63264=ORIENTED_EDGE ( 'NONE', *, *, #21387, .T. ) ;
#63270=CARTESIAN_POINT ( 'NONE',  ( 96.15314808468748708, 88.00268892867053694, 84.77447916753381207 ) ) ;
#63272=CARTESIAN_POINT ( 'NONE',  ( 92.69370383062501162, -211.3315407142195852, 83.34572916753380412 ) ) ;
#63278=DIRECTION ( 'NONE',  ( -1.000000000000000000, -0.000000000000000000, -0.000000000000000000 ) ) ;
#63282=CARTESIAN_POINT ( 'NONE',  ( -92.69370383062498320, -209.9999999999999716, 84.24531250086714351 ) ) ;
#63284=CARTESIAN_POINT ( 'NONE',  ( -93.84685191531252713, 88.00268892867056536, 81.75822916753382685 ) ) ;
#63286=CARTESIAN_POINT ( 'NONE',  ( 96.15314808468748708, 91.99731107132950569, 85.62114583420046188 ) ) ;
#63287=CARTESIAN_POINT ( 'NONE',  ( -93.84685191531254134, 91.99731107132950569, 86.25614583420048120 ) ) ;
#63288=ORIENTED_EDGE ( 'NONE', *, *, #65022, .F. ) ;
#63293=CARTESIAN_POINT ( 'NONE',  ( -94.99999999999997158, -212.6630814284392557, 85.99156250086714692 ) ) ;
#63295=CARTESIAN_POINT ( 'NONE',  ( -97.64999999954994792, 89.99996890530464100, 88.81037122970319331 ) ) ;
#63299=ORIENTED_EDGE ( 'NONE', *, *, #6983, .T. ) ;
#63300=CARTESIAN_POINT ( 'NONE',  ( -93.67500000000003979, 92.29496732002878900, 78.99333333333332519 ) ) ;
#63302=CARTESIAN_POINT ( 'NONE',  ( -94.70223316838999494, -207.6384304500494977, 74.83035915144985495 ) ) ;
#63307=( BOUNDED_CURVE ( )  B_SPLINE_CURVE ( 2, ( #4826, #72825, #67955, #55928, #22846, #27728, #50652, #38646, #28093 ),
 .UNSPECIFIED., .F., .F. ) 
 B_SPLINE_CURVE_WITH_KNOTS ( ( 3, 2, 2, 2, 3 ),
 ( 0.2540073681295598185, 0.2540075594730126229, 0.2610633250139296480, 0.2681190905548467285, 0.2751748541917909407 ),
 .UNSPECIFIED. ) 
 CURVE ( )  GEOMETRIC_REPRESENTATION_ITEM ( )  RATIONAL_B_SPLINE_CURVE ( ( 0.9999927337532719118, 0.9999963667781075483, 1.000000000000000000, 0.8660254037844387076, 1.000000000000000000, 0.8660254037844387076, 1.000000000000000000, 0.8660254037844387076, 1.000000000000000000 ) ) 
 REPRESENTATION_ITEM ( '' )  );
#63310=CARTESIAN_POINT ( 'NONE',  ( -93.84685191531254134, 91.99731107132950569, 77.36614583420046642 ) ) ;
#63317=FACE_OUTER_BOUND ( 'NONE', #40882, .T. ) ;
#63323=CARTESIAN_POINT ( 'NONE',  ( 97.30629616937498838, 88.66845928578035796, 78.63614583420046245 ) ) ;
#63325=CARTESIAN_POINT ( 'NONE',  ( -96.15314808468745866, -211.9973110713294489, 81.01739583420049939 ) ) ;
#63328=CARTESIAN_POINT ( 'NONE',  ( -92.35000000000003695, 90.00000000000004263, 82.77687500173431090 ) ) ;
#63329=CARTESIAN_POINT ( 'NONE',  ( 97.64999999954044085, -209.9999506483753180, 87.22187670868780174 ) ) ;
#63330=CARTESIAN_POINT ( 'NONE',  ( 96.32499999999998863, -212.2949673200287179, 78.86104166840097207 ) ) ;
#63331=VECTOR ( 'NONE', #46144, 1000.000000000000000 ) ;
#63333=CARTESIAN_POINT ( 'NONE',  ( -97.30629616937501680, 91.33154071421968467, 75.14364583420049826 ) ) ;
#63334=CARTESIAN_POINT ( 'NONE',  ( 95.00000000000000000, -207.3369185715606307, 75.51406250086714067 ) ) ;
#63340=ORIENTED_EDGE ( 'NONE', *, *, #33689, .F. ) ;
#63345=CARTESIAN_POINT ( 'NONE',  ( -96.32499999999996021, -212.2949673200287179, 77.40583333333331950 ) ) ;
#63349=ORIENTED_EDGE ( 'NONE', *, *, #47963, .T. ) ;
#63350=CARTESIAN_POINT ( 'NONE',  ( 96.15314808468748708, 91.99731107132950569, 83.23989583420049598 ) ) ;
#63352=CARTESIAN_POINT ( 'NONE',  ( 93.67500000000001137, -207.7050326799711968, 75.28916666666665947 ) ) ;
#63365=FACE_OUTER_BOUND ( 'NONE', #29565, .T. ) ;
#63368=CARTESIAN_POINT ( 'NONE',  ( -93.67499999999998295, -212.2949673200287179, 80.13104166840095388 ) ) ;
#63372=CARTESIAN_POINT ( 'NONE',  ( 97.64999999999999147, 90.00000000000002842, 78.96687500173429441 ) ) ;
#63373=CARTESIAN_POINT ( 'NONE',  ( -97.65000000000001990, 90.00000000000004263, 79.91937500173429498 ) ) ;
#63375=CARTESIAN_POINT ( 'NONE',  ( 92.69370383062498320, 88.66845928578037217, 78.42447916753380355 ) ) ;
#63381=DIRECTION ( 'NONE',  ( -0.000000000000000000, -0.000000000000000000, 1.000000000000000000 ) ) ;
#63383=DIRECTION ( 'NONE',  ( -0.000000000000000000, -0.000000000000000000, 1.000000000000000000 ) ) ;
#63384=EDGE_LOOP ( 'NONE', ( #47433, #26447, #30968, #21730 ) ) ;
#63388=CIRCLE ( 'NONE', #30938, 23.50000000000000355 ) ;
#63391=DIRECTION ( 'NONE',  ( 4.476705744456278560E-17, -1.000000000000000000, 8.723836835350694626E-17 ) ) ;
#63393=FACE_OUTER_BOUND ( 'NONE', #22187, .T. ) ;
#63394=CARTESIAN_POINT ( 'NONE',  ( -93.84685191531247028, -211.9973110713294489, 76.67822916753381435 ) ) ;
#63396=EDGE_LOOP ( 'NONE', ( #44705, #25039, #26764, #1242 ) ) ;
#63400=CARTESIAN_POINT ( 'NONE',  ( 93.84685191531248449, 88.00268892867053694, 75.77864583420047495 ) ) ;
#63401=CARTESIAN_POINT ( 'NONE',  ( 95.00000000000000000, -209.9999999999999716, 90.00000000000000000 ) ) ;
#63403=EDGE_CURVE ( 'NONE', #56237, #21161, #41980, .T. ) ;
#63410=CARTESIAN_POINT ( 'NONE',  ( 92.69370383062498320, 90.00000000000002842, 85.99156250086716113 ) ) ;
#63419=CARTESIAN_POINT ( 'NONE',  ( -95.00000000000002842, 87.33691857156074434, 80.27656250086714351 ) ) ;
#63436=CARTESIAN_POINT ( 'NONE',  ( 96.15314808468748708, -208.0026889286704943, 80.69989583420047552 ) ) ;
#63437=EDGE_CURVE ( 'NONE', #59366, #29381, #62643, .T. ) ;
#63441=CARTESIAN_POINT ( 'NONE',  ( 92.34999999999999432, 90.00000000000002842, 83.72937500173429726 ) ) ;
#63444=CARTESIAN_POINT ( 'NONE',  ( 93.67500000000001137, -207.7050326799711968, 86.08416666666666117 ) ) ;
#63449=CARTESIAN_POINT ( 'NONE',  ( -92.69370383062502583, 91.33154071421968467, 88.90197916753382401 ) ) ;
#63451=CARTESIAN_POINT ( 'NONE',  ( -96.32500000000001705, 87.70503267997129626, 83.75583333333332803 ) ) ;
#63452=CARTESIAN_POINT ( 'NONE',  ( 92.35000000000002274, -211.5299782133524502, 77.43229166840096411 ) ) ;
#63453=CARTESIAN_POINT ( 'NONE',  ( 97.64999999999997726, 91.52997821335252127, 77.67041666666665378 ) ) ;
#63457=CARTESIAN_POINT ( 'NONE',  ( -97.64999999999996305, -208.4700217866474645, 83.04145833506764518 ) ) ;
#63458=ORIENTED_EDGE ( 'NONE', *, *, #36098, .F. ) ;
#63459=CARTESIAN_POINT ( 'NONE',  ( -92.35000000000005116, 88.47002178664754979, 88.43895833506762472 ) ) ;
#63460=CARTESIAN_POINT ( 'NONE',  ( -92.69370383062505425, 88.66845928578038638, 81.17614583420049712 ) ) ;
#63462=CARTESIAN_POINT ( 'NONE',  ( 94.99999999999998579, 87.33691857156068750, 89.32531250086715602 ) ) ;
#63468=CARTESIAN_POINT ( 'NONE',  ( -97.65000000000001990, 90.00000000000004263, 86.18999999999999773 ) ) ;
#63469=CARTESIAN_POINT ( 'NONE',  ( -92.93550210798947830, 91.06393496763725182, 74.79348190356850523 ) ) ;
#63472=CARTESIAN_POINT ( 'NONE',  ( -96.15314808468745866, -211.9973110713294489, 78.31864583420048120 ) ) ;
#63477=ORIENTED_EDGE ( 'NONE', *, *, #45249, .T. ) ;
#63478=CARTESIAN_POINT ( 'NONE',  ( 92.35000000019411459, -210.0000198431783929, 84.36502760998391182 ) ) ;
#63481=CARTESIAN_POINT ( 'NONE',  ( -93.84685191531248449, -208.0026889286704943, 77.36614583420046642 ) ) ;
#63486=ORIENTED_EDGE ( 'NONE', *, *, #48411, .F. ) ;
#63493=CARTESIAN_POINT ( 'NONE',  ( 96.15314808468748708, 88.00268892867053694, 85.40947916753380298 ) ) ;
#63513=( BOUNDED_CURVE ( )  B_SPLINE_CURVE ( 2, ( #56923, #5430, #45654, #53760, #28325, #191, #22714 ),
 .UNSPECIFIED., .F., .F. ) 
 B_SPLINE_CURVE_WITH_KNOTS ( ( 3, 2, 2, 3 ),
 ( 0.000000000000000000, 0.006944444444444406762, 0.01388888888888881352, 0.02083333333333322115 ),
 .UNSPECIFIED. ) 
 CURVE ( )  GEOMETRIC_REPRESENTATION_ITEM ( )  RATIONAL_B_SPLINE_CURVE ( ( 1.000000000000000000, 0.8660254037844387076, 1.000000000000000000, 0.8660254037844387076, 1.000000000000000000, 0.8660254037844408170, 0.9999999999999978906 ) ) 
 REPRESENTATION_ITEM ( '' )  );
#63523=CARTESIAN_POINT ( 'NONE',  ( 93.84685191531251292, -211.9973110713294489, 84.82739583420048746 ) ) ;
#63527=CARTESIAN_POINT ( 'NONE',  ( -92.34999999999989484, -208.4700217866475214, 85.92541666666664923 ) ) ;
#63529=CARTESIAN_POINT ( 'NONE',  ( -92.34999999999999432, -208.4700217866474645, 79.65479166840096070 ) ) ;
#63530=CARTESIAN_POINT ( 'NONE',  ( 93.84685191531249870, -208.0026889286704943, 74.93197916753379673 ) ) ;
#63532=CARTESIAN_POINT ( 'NONE',  ( 96.15314808468748708, -208.0026889286704943, 83.23989583420049598 ) ) ;
#63544=CARTESIAN_POINT ( 'NONE',  ( 96.32499999999998863, -212.2949673200287179, 85.84604166840097150 ) ) ;
#63563=CARTESIAN_POINT ( 'NONE',  ( -93.67500000000003979, 87.70503267997129626, 88.30666666666665776 ) ) ;
#63564=ORIENTED_EDGE ( 'NONE', *, *, #58490, .F. ) ;
#63568=CARTESIAN_POINT ( 'NONE',  ( -97.30629616937497417, -208.6684592857803011, 87.68489583420047495 ) ) ;
#63574=CARTESIAN_POINT ( 'NONE',  ( -93.84685191531247028, -211.9973110713294489, 75.88447916753381151 ) ) ;
#63582=CARTESIAN_POINT ( 'NONE',  ( -97.65000000000001990, 88.47002178664754979, 85.05229166840096866 ) ) ;
#63583=ADVANCED_FACE ( 'NONE', ( #66244 ), #35792, .F. ) ;
#63589=CARTESIAN_POINT ( 'NONE',  ( -92.69370383062504004, 90.00000000000004263, 77.89531250086714920 ) ) ;
#63593=VERTEX_POINT ( 'NONE', #24897 ) ;
#63594=CARTESIAN_POINT ( 'NONE',  ( 92.34999999999999432, 90.00000000000002842, 79.28437500173430408 ) ) ;
#63596=EDGE_CURVE ( 'NONE', #11817, #26794, #39273, .T. ) ;
#63597=CARTESIAN_POINT ( 'NONE',  ( -97.64999999999996305, -209.9999999999999716, 81.10999999999999943 ) ) ;
#63603=CARTESIAN_POINT ( 'NONE',  ( -93.84685191531248449, -208.0026889286704943, 76.25489583420049655 ) ) ;
#63617=CARTESIAN_POINT ( 'NONE',  ( 97.64999999999999147, 90.00000000000002842, 81.42749999999999488 ) ) ;
#63622=CARTESIAN_POINT ( 'NONE',  ( 95.00000000000000000, -212.6630814284392557, 84.72156250086713669 ) ) ;
#63626=AXIS2_PLACEMENT_3D ( 'NONE', #54985, #50072, #62506 ) ;
#63632=CARTESIAN_POINT ( 'NONE',  ( -97.30629616937501680, 88.66845928578038638, 81.59947916753381492 ) ) ;
#63633=VERTEX_POINT ( 'NONE', #27852 ) ;
#63639=CARTESIAN_POINT ( 'NONE',  ( 93.08933536981345469, 88.26122129797421678, 74.95660481729451874 ) ) ;
#63640=ORIENTED_EDGE ( 'NONE', *, *, #23420, .T. ) ;
#63642=CARTESIAN_POINT ( 'NONE',  ( 92.69370383062498320, 90.00000000000002842, 86.46781250086714010 ) ) ;
#63645=CARTESIAN_POINT ( 'NONE',  ( 97.30629616937498838, -209.9999999999999716, 82.34031250086714238 ) ) ;
#63653=CARTESIAN_POINT ( 'NONE',  ( -92.35000000000005116, 88.47002178664754979, 79.46958333333331836 ) ) ;
#63656=CARTESIAN_POINT ( 'NONE',  ( -92.69370383062498320, -208.6684592857803011, 84.93322916753379559 ) ) ;
#63657=CARTESIAN_POINT ( 'NONE',  ( -95.00000000000002842, 87.33691857156074434, 81.07031250086716057 ) ) ;
#63659=CARTESIAN_POINT ( 'NONE',  ( 96.15314808468748708, 88.00268892867053694, 86.04447916753380809 ) ) ;
#63660=ORIENTED_EDGE ( 'NONE', *, *, #19411, .F. ) ;
#63666=CARTESIAN_POINT ( 'NONE',  ( -97.30629616937497417, -211.3315407142195852, 87.79072916753379729 ) ) ;
#63671=CARTESIAN_POINT ( 'NONE',  ( -92.35000000000553655, 89.99999459739531460, 81.50687481489494246 ) ) ;
#63675=ADVANCED_FACE ( 'NONE', ( #26370 ), #49300, .F. ) ;
#63677=CARTESIAN_POINT ( 'NONE',  ( -92.35000000000005116, 91.52997821335253548, 78.94041666666666401 ) ) ;
#63679=CARTESIAN_POINT ( 'NONE',  ( -95.43397055421739594, -207.6412937382899031, 74.84690984288805282 ) ) ;
#63685=CARTESIAN_POINT ( 'NONE',  ( -92.69370383062502583, 91.33154071421968467, 79.85322916753379729 ) ) ;
#63691=CARTESIAN_POINT ( 'NONE',  ( 95.00000000000000000, -206.9400435732949575, 84.20562500173429044 ) ) ;
#63693=CARTESIAN_POINT ( 'NONE',  ( -92.69370383062498320, -211.3315407142195852, 84.98614583420047097 ) ) ;
#63696=CARTESIAN_POINT ( 'NONE',  ( 94.99999999999998579, 92.66308142843932671, 77.57781250086715374 ) ) ;
#63697=CARTESIAN_POINT ( 'NONE',  ( -94.99999999999997158, -207.3369185715606307, 77.57781250086715374 ) ) ;
#63704=EDGE_CURVE ( 'NONE', #66690, #70972, #85, .T. ) ;
#63708=CARTESIAN_POINT ( 'NONE',  ( 93.84685191531251292, -211.9973110713294489, 78.31864583420048120 ) ) ;
#63711=ORIENTED_EDGE ( 'NONE', *, *, #18562, .T. ) ;
#63714=CARTESIAN_POINT ( 'NONE',  ( 92.35000000000000853, -209.9999999999999716, 83.65000000000000568 ) ) ;
#63717=VERTEX_POINT ( 'NONE', #45542 ) ;
#63718=CARTESIAN_POINT ( 'NONE',  ( 97.64999999999999147, -209.9999998456624155, 79.60187500750917877 ) ) ;
#63721=CARTESIAN_POINT ( 'NONE',  ( 94.99999999999998579, 87.33691857156068750, 83.61031250086716682 ) ) ;
#63731=B_SPLINE_CURVE_WITH_KNOTS ( 'NONE', 3,
 ( #72010, #20520, #43478, #66396, #37821, #60752, #9229, #32151, #15624, #61494, #26889, #15243, #73120, #3624, #11096, #26523, #38177, #45319 ),
 .UNSPECIFIED., .F., .F.,
 ( 4, 2, 2, 2, 2, 2, 2, 2, 4 ),
 ( -0.004093595874563257103, -0.003575961937392224069, -0.003058328000221191036, -0.002540694063050158436, -0.002023060125879125402, -0.001505426188708092368, -0.0009877922515370597678, -0.0004701583143660267340, 4.747562280500629978E-05 ),
 .UNSPECIFIED. ) ;
#63733=CARTESIAN_POINT ( 'NONE',  ( -97.64999999999996305, -208.4700217866474645, 75.42145833506764063 ) ) ;
#63736=CARTESIAN_POINT ( 'NONE',  ( 93.67500000000001137, -212.2949673200287179, 87.01020833506763097 ) ) ;
#63740=CARTESIAN_POINT ( 'NONE',  ( -92.34999999999999432, -211.5299782133524502, 80.18395833506764347 ) ) ;
#63741=ORIENTED_EDGE ( 'NONE', *, *, #14406, .T. ) ;
#63744=CARTESIAN_POINT ( 'NONE',  ( 93.67499999999998295, 92.29496732002878900, 78.54354166840096241 ) ) ;
#63745=CARTESIAN_POINT ( 'NONE',  ( -92.35000000000005116, 91.52997821335253548, 78.38479166840096468 ) ) ;
#63746=( BOUNDED_CURVE ( )  B_SPLINE_CURVE ( 2, ( #20025, #65918, #14394, #37343, #60282, #8761, #54621 ),
 .UNSPECIFIED., .F., .F. ) 
 B_SPLINE_CURVE_WITH_KNOTS ( ( 3, 2, 2, 3 ),
 ( 0.7499999999999996669, 0.7569444444444439757, 0.7638888888888883955, 0.7708333333333328152 ),
 .UNSPECIFIED. ) 
 CURVE ( )  GEOMETRIC_REPRESENTATION_ITEM ( )  RATIONAL_B_SPLINE_CURVE ( ( 1.000000000000006439, 0.8660254037844322683, 1.000000000000000000, 0.8660254037844387076, 1.000000000000000000, 0.8660254037844493658, 0.9999999999999893419 ) ) 
 REPRESENTATION_ITEM ( '' )  );
#63747=ORIENTED_EDGE ( 'NONE', *, *, #50910, .T. ) ;
#63748=CARTESIAN_POINT ( 'NONE',  ( 93.84685191531248449, 88.00268892867053694, 79.11239583420048405 ) ) ;
#63749=DIRECTION ( 'NONE',  ( 1.000000000000000000, 0.000000000000000000, 0.000000000000000000 ) ) ;
#63750=PRODUCT_DEFINITION ( 'UNKNOWN', '', #60394, #59703 ) ;
#63752=ADVANCED_FACE ( 'NONE', ( #74084 ), #52269, .F. ) ;
#63753=CARTESIAN_POINT ( 'NONE',  ( -93.67500000000003979, 92.29496732002878900, 86.69270833506763552 ) ) ;
#63754=VECTOR ( 'NONE', #20278, 1000.000000000000000 ) ;
#63758=CARTESIAN_POINT ( 'NONE',  ( 97.64999999999999147, 90.00000000000002842, 78.25249999999999773 ) ) ;
#63769=DIRECTION ( 'NONE',  ( 1.000000000000000000, 0.000000000000000000, 0.000000000000000000 ) ) ;
#63770=CARTESIAN_POINT ( 'NONE',  ( -92.69370383062498320, -208.6684592857803011, 78.10697916753383652 ) ) ;
#63778=LINE ( 'NONE', #59233, #36074 ) ;
#63781=DIRECTION ( 'NONE',  ( -0.000000000000000000, -0.000000000000000000, 1.000000000000000000 ) ) ;
#63782=ADVANCED_FACE ( 'NONE', ( #18063 ), #50387, .F. ) ;
#63783=CARTESIAN_POINT ( 'NONE',  ( 100.0010000000000474, -65.00000000000002842, -90.00000000000000000 ) ) ;
#63785=CARTESIAN_POINT ( 'NONE',  ( 94.99999999999998579, 87.33691857156068750, 88.05531250086714579 ) ) ;
#63787=LINE ( 'NONE', #57393, #2606 ) ;
#63792=CARTESIAN_POINT ( 'NONE',  ( -95.00000000000002842, 92.66308142843932671, 76.14906250086716000 ) ) ;
#63794=EDGE_CURVE ( 'NONE', #74237, #41316, #35359, .T. ) ;
#63795=CARTESIAN_POINT ( 'NONE',  ( 92.69370383062501162, -211.3315407142195852, 87.15572916753380639 ) ) ;
#63798=CARTESIAN_POINT ( 'NONE',  ( -92.34999999999999432, -210.0000000024460576, 75.15687493084206494 ) ) ;
#63807=CARTESIAN_POINT ( 'NONE',  ( 93.84685191531249870, -208.0026889286704943, 83.34572916753383254 ) ) ;
#63808=DIRECTION ( 'NONE',  ( 1.000000000000000000, 0.000000000000000000, 0.000000000000000000 ) ) ;
#63810=CARTESIAN_POINT ( 'NONE',  ( -97.64999999999996305, -208.4700217866474645, 77.32645833506762756 ) ) ;
#63812=CARTESIAN_POINT ( 'NONE',  ( -94.99999999999997158, -209.9999999999999716, 90.00000000000000000 ) ) ;
#63813=CARTESIAN_POINT ( 'NONE',  ( 92.35000000000002274, -211.5299782133524502, 86.24291666666665890 ) ) ;
#63820=CARTESIAN_POINT ( 'NONE',  ( -92.69370383062504004, 90.00000000000004263, 86.94406250086716170 ) ) ;
#63823=CARTESIAN_POINT ( 'NONE',  ( 97.65000000000000568, -208.4700217866474645, 78.38479166840096468 ) ) ;
#63824=CARTESIAN_POINT ( 'NONE',  ( 93.67500000000001137, -212.2949673200287179, 76.85020833506763438 ) ) ;
#63825=CARTESIAN_POINT ( 'NONE',  ( 94.99999999999998579, 93.05995642670504253, 79.68124999999999147 ) ) ;
#63826=EDGE_CURVE ( 'NONE', #20056, #14688, #15623, .T. ) ;
#63827=ORIENTED_EDGE ( 'NONE', *, *, #3407, .F. ) ;
#63828=CARTESIAN_POINT ( 'NONE',  ( -94.99999999999997158, -213.0599564267049857, 88.33312500173428816 ) ) ;
#63832=CARTESIAN_POINT ( 'NONE',  ( -97.65000000000001990, 90.00000000000004263, 88.80937500173430976 ) ) ;
#63833=CARTESIAN_POINT ( 'NONE',  ( -96.15314808468752972, 91.99731107132950569, 82.71072916753381321 ) ) ;
#63834=CARTESIAN_POINT ( 'NONE',  ( 92.69370383062498320, 91.33154071421968467, 75.61989583420047722 ) ) ;
#63841=CARTESIAN_POINT ( 'NONE',  ( -93.07889023459844680, 91.30563282057288177, 74.79348190356849102 ) ) ;
#63842=EDGE_LOOP ( 'NONE', ( #68946, #50365 ) ) ;
#63845=CARTESIAN_POINT ( 'NONE',  ( -92.69370383062498320, -209.9999999999999716, 75.35531250086714294 ) ) ;
#63849=LINE ( 'NONE', #5600, #16946 ) ;
#63854=CARTESIAN_POINT ( 'NONE',  ( -92.69370383062498320, -211.3315407142195852, 87.52614583420049144 ) ) ;
#63856=CARTESIAN_POINT ( 'NONE',  ( -15.70000000000000284, -120.0000000000000000, -85.59999999999999432 ) ) ;
#63864=CARTESIAN_POINT ( 'NONE',  ( 97.65000000000000568, -208.4700217866474645, 86.00479166840096923 ) ) ;
#63865=CARTESIAN_POINT ( 'NONE',  ( 97.30629616937498838, 88.66845928578035796, 84.19239583420048234 ) ) ;
#63884=CARTESIAN_POINT ( 'NONE',  ( -92.34999999999999432, -209.9999999999999716, 90.00000000000000000 ) ) ;
#63886=CARTESIAN_POINT ( 'NONE',  ( 94.99999999999998579, 93.05995642670504253, 77.14124999999999943 ) ) ;
#63888=CARTESIAN_POINT ( 'NONE',  ( -97.64995975554930396, 88.46999855150308179, 77.43229327564789344 ) ) ;
#63890=CARTESIAN_POINT ( 'NONE',  ( 97.30629616937498838, -208.6684592857803011, 86.99697916753382287 ) ) ;
#63901=CARTESIAN_POINT ( 'NONE',  ( 95.00000000000000000, -212.6630814284392557, 78.53031250086715431 ) ) ;
#63913=CARTESIAN_POINT ( 'NONE',  ( 92.35000000000002274, -211.5299782133524502, 86.32229166840097889 ) ) ;
#63914=CARTESIAN_POINT ( 'NONE',  ( 94.99999999999998579, 86.94004357329500010, 88.88875000000000171 ) ) ;
#63921=CARTESIAN_POINT ( 'NONE',  ( 94.99999999999998579, 93.05995642670504253, 86.11062500173430578 ) ) ;
#63930=CARTESIAN_POINT ( 'NONE',  ( 92.35000000021533140, 90.00002100773845370, 79.91868729553033290 ) ) ;
#63932=CARTESIAN_POINT ( 'NONE',  ( -95.00000000000002842, 93.05995642670501411, 87.30124999999999602 ) ) ;
#63933=ORIENTED_EDGE ( 'NONE', *, *, #62083, .T. ) ;
#63938=CARTESIAN_POINT ( 'NONE',  ( -94.99999999999997158, -207.3369185715606307, 83.13406250086714522 ) ) ;
#63944=CARTESIAN_POINT ( 'NONE',  ( -96.15314808468747287, -208.0026889286704943, 75.56697916753381605 ) ) ;
#63950=CARTESIAN_POINT ( 'NONE',  ( 2.500000000000034639, 90.00000000000000000, -310.0000000000000000 ) ) ;
#63954=CARTESIAN_POINT ( 'NONE',  ( -97.30629616937501680, 91.33154071421968467, 80.06489583420047040 ) ) ;
#63957=EDGE_CURVE ( 'NONE', #52806, #58070, #7929, .T. ) ;
#63959=( BOUNDED_CURVE ( )  B_SPLINE_CURVE ( 2, ( #63930, #40246, #23692, #46626, #33859, #57545, #69556 ),
 .UNSPECIFIED., .F., .F. ) 
 B_SPLINE_CURVE_WITH_KNOTS ( ( 3, 2, 2, 3 ),
 ( 0.6350190250571090544, 0.6420746642202955767, 0.6491304297611778518, 0.6561861948910822084 ),
 .UNSPECIFIED. ) 
 CURVE ( )  GEOMETRIC_REPRESENTATION_ITEM ( )  RATIONAL_B_SPLINE_CURVE ( ( 0.9999952007766099715, 0.8660278034391145630, 1.000000000000000000, 0.8660254037844387076, 1.000000000000000000, 0.8660254037844387076, 1.000000000000000000 ) ) 
 REPRESENTATION_ITEM ( '' )  );
#63963=DIRECTION ( 'NONE',  ( -0.000000000000000000, -0.000000000000000000, 1.000000000000000000 ) ) ;
#63968=CARTESIAN_POINT ( 'NONE',  ( -97.64999999969894873, 90.00002455906438570, 87.53856274002211535 ) ) ;
#63969=CARTESIAN_POINT ( 'NONE',  ( -96.15314808468745866, -211.9973110713294489, 75.93739583420048689 ) ) ;
#63970=CARTESIAN_POINT ( 'NONE',  ( -95.00000000000002842, 90.00000000000004263, 90.00000000000000000 ) ) ;
#63981=CARTESIAN_POINT ( 'NONE',  ( 97.30629616937498838, -211.3315407142195852, 84.82739583420048746 ) ) ;
#63982=CARTESIAN_POINT ( 'NONE',  ( -95.00000000000002842, 93.05995642670504253, 82.30062500173427509 ) ) ;
#63984=ADVANCED_FACE ( 'NONE', ( #24439 ), #42113, .F. ) ;
#63990=CARTESIAN_POINT ( 'NONE',  ( -96.15314808468752972, 91.99731107132950569, 81.44072916753381719 ) ) ;
#63991=ADVANCED_FACE ( 'NONE', ( #43600 ), #66519, .F. ) ;
#63992=AXIS2_PLACEMENT_3D ( 'NONE', #35487, #35847, #951 ) ;
#63993=EDGE_LOOP ( 'NONE', ( #28864, #4361, #49193, #20604 ) ) ;
#64010=CARTESIAN_POINT ( 'NONE',  ( 97.30629616937498838, -211.3315407142195852, 81.01739583420048518 ) ) ;
#64014=CARTESIAN_POINT ( 'NONE',  ( -94.26002770235174921, -212.5681771730648109, 75.00000000000000000 ) ) ;
#64017=CARTESIAN_POINT ( 'NONE',  ( -92.35000000000003695, 90.00000000000004263, 79.52249999999999375 ) ) ;
#64019=CARTESIAN_POINT ( 'NONE',  ( -93.84685191531248449, -208.0026889286704943, 85.62114583420046188 ) ) ;
#64020=CARTESIAN_POINT ( 'NONE',  ( -92.69370383062502583, 88.66845928578038638, 82.44614583420049314 ) ) ;
#64022=ADVANCED_FACE ( 'NONE', ( #72506 ), #16782, .F. ) ;
#64023=CARTESIAN_POINT ( 'NONE',  ( 96.15314808468748708, 88.00268892867053694, 84.77447916753381207 ) ) ;
#64026=DIRECTION ( 'NONE',  ( -0.000000000000000000, -0.000000000000000000, 1.000000000000000000 ) ) ;
#64031=CARTESIAN_POINT ( 'NONE',  ( -93.84685191531248449, -208.0026889286704943, 84.98614583420047097 ) ) ;
#64036=FACE_OUTER_BOUND ( 'NONE', #55382, .T. ) ;
#64039=CARTESIAN_POINT ( 'NONE',  ( -92.35000000000005116, 88.47002178664754979, 77.56458333333333144 ) ) ;
#64040=CARTESIAN_POINT ( 'NONE',  ( 95.00000000000000000, -213.0599564267049857, 88.88875000000000171 ) ) ;
#64042=CARTESIAN_POINT ( 'NONE',  ( -92.69370383062502583, 88.66845928578038638, 89.27239583420048064 ) ) ;
#64050=EDGE_CURVE ( 'NONE', #45116, #27941, #61741, .T. ) ;
#64056=DIRECTION ( 'NONE',  ( -0.000000000000000000, -0.000000000000000000, 1.000000000000000000 ) ) ;
#64058=CARTESIAN_POINT ( 'NONE',  ( -93.84685191531247028, -211.9973110713294489, 86.83822916753382515 ) ) ;
#64062=CARTESIAN_POINT ( 'NONE',  ( 92.69370383062498320, 90.00000000000002842, 77.73656250086715147 ) ) ;
#64063=CARTESIAN_POINT ( 'NONE',  ( -96.15314808468747287, -208.0026889286704943, 75.72572916753382799 ) ) ;
#64065=ORIENTED_EDGE ( 'NONE', *, *, #39730, .T. ) ;
#64073=CARTESIAN_POINT ( 'NONE',  ( 95.00000000000000000, -207.3369185715606307, 76.78406250086712248 ) ) ;
#64074=ORIENTED_EDGE ( 'NONE', *, *, #24556, .T. ) ;
#64080=ADVANCED_FACE ( 'NONE', ( #5142 ), #28044, .F. ) ;
#64082=EDGE_CURVE ( 'NONE', #39726, #30760, #31182, .T. ) ;
#64084=ORIENTED_EDGE ( 'NONE', *, *, #7974, .F. ) ;
#64088=CARTESIAN_POINT ( 'NONE',  ( 97.64999999999996305, -211.0554082285335937, 75.04099707143595310 ) ) ;
#64092=CARTESIAN_POINT ( 'NONE',  ( 97.30629616937498838, 88.66845928578037217, 82.44614583420049314 ) ) ;
#64094=CARTESIAN_POINT ( 'NONE',  ( 92.35000000000002274, -208.4700217866474645, 75.34208333333333485 ) ) ;
#64098=ORIENTED_EDGE ( 'NONE', *, *, #33594, .T. ) ;
#64103=CARTESIAN_POINT ( 'NONE',  ( 92.35000000000000853, -211.5299782133524218, 82.51229166840094820 ) ) ;
#64104=CARTESIAN_POINT ( 'NONE',  ( -94.99999999999997158, -209.9999999999999716, 90.00000000000000000 ) ) ;
#64106=CARTESIAN_POINT ( 'NONE',  ( 92.35000000000005116, 91.52997821335254969, 77.88208333333332689 ) ) ;
#64107=CARTESIAN_POINT ( 'NONE',  ( -97.64999999999994884, -211.5299782133524502, 79.97229166840095615 ) ) ;
#64111=CARTESIAN_POINT ( 'NONE',  ( 96.32499999999997442, 92.29496732002878900, 79.70770833506762187 ) ) ;
#64112=CARTESIAN_POINT ( 'NONE',  ( -96.32500000000001705, 87.70503267997129626, 76.85020833506763438 ) ) ;
#64115=CARTESIAN_POINT ( 'NONE',  ( 94.99999999999998579, 92.66308142843935514, 79.48281250086715488 ) ) ;
#64116=VECTOR ( 'NONE', #46393, 1000.000000000000000 ) ;
#64119=CARTESIAN_POINT ( 'NONE',  ( 92.35000000000000853, -211.5299782133524218, 79.33729166840096525 ) ) ;
#64120=CARTESIAN_POINT ( 'NONE',  ( -89.99999999999992895, -116.0000000000000000, -40.00000000000002132 ) ) ;
#64130=B_SPLINE_CURVE_WITH_KNOTS ( 'NONE', 3,
 ( #20508, #38160, #56199, #20122, #49803, #44178, #14861, #66017 ),
 .UNSPECIFIED., .F., .F.,
 ( 4, 2, 2, 4 ),
 ( 0.001653806717455073069, 0.002539064216007527134, 0.002981692965283746360, 0.003424321714559965153 ),
 .UNSPECIFIED. ) ;
#64133=CARTESIAN_POINT ( 'NONE',  ( -96.32499999999996021, -207.7050326799711968, 75.92416666666666458 ) ) ;
#64134=CARTESIAN_POINT ( 'NONE',  ( -94.99999999999997158, -207.3369185715606307, 76.30781250086715772 ) ) ;
#64138=CARTESIAN_POINT ( 'NONE',  ( -97.40333747838421630, -210.8453944377615414, 74.93511027845802630 ) ) ;
#64145=CARTESIAN_POINT ( 'NONE',  ( -93.67499999999998295, -212.2949673200287179, 76.24166666666666003 ) ) ;
#64146=DIRECTION ( 'NONE',  ( -0.000000000000000000, -0.000000000000000000, 1.000000000000000000 ) ) ;
#64148=CARTESIAN_POINT ( 'NONE',  ( 97.30629616937498838, 90.00000000000002842, 86.30906250086715659 ) ) ;
#64149=CARTESIAN_POINT ( 'NONE',  ( -97.30629616937495996, -209.9999999999999716, 85.35656250086715602 ) ) ;
#64153=CARTESIAN_POINT ( 'NONE',  ( -94.99999999999997158, -206.9400435732949575, 81.58624999999999261 ) ) ;
#64154=CARTESIAN_POINT ( 'NONE',  ( -96.15314808468752972, 91.99731107132950569, 76.20197916753380696 ) ) ;
#64156=CARTESIAN_POINT ( 'NONE',  ( 92.69370383062501162, -211.3315407142195852, 88.42572916753380241 ) ) ;
#64168=ORIENTED_EDGE ( 'NONE', *, *, #11949, .F. ) ;
#64172=CARTESIAN_POINT ( 'NONE',  ( 93.84685191531249870, -208.0026889286704943, 80.17072916753382117 ) ) ;
#64176=CARTESIAN_POINT ( 'NONE',  ( 92.34999999999999432, 90.00000000000002842, 83.01499999999998636 ) ) ;
#64177=( BOUNDED_CURVE ( )  B_SPLINE_CURVE ( 2, ( #12922, #46414, #40786, #68979, #63345, #30222, #35857 ),
 .UNSPECIFIED., .F., .F. ) 
 B_SPLINE_CURVE_WITH_KNOTS ( ( 3, 2, 2, 3 ),
 ( 0.8125000000000002220, 0.8194444444444446418, 0.8263888888888889506, 0.8333333333333334814 ),
 .UNSPECIFIED. ) 
 CURVE ( )  GEOMETRIC_REPRESENTATION_ITEM ( )  RATIONAL_B_SPLINE_CURVE ( ( 0.9999999999999956701, 0.8660254037844430375, 1.000000000000000000, 0.8660254037844387076, 1.000000000000000000, 0.8660254037844365982, 1.000000000000002220 ) ) 
 REPRESENTATION_ITEM ( '' )  );
#64181=CARTESIAN_POINT ( 'NONE',  ( 93.67500000000001137, -212.2949673200287179, 85.66083333333332916 ) ) ;
#64184=VERTEX_POINT ( 'NONE', #14117 ) ;
#64188=CARTESIAN_POINT ( 'NONE',  ( -97.30629616937501680, 91.33154071421968467, 85.93864583420048575 ) ) ;
#64190=DIRECTION ( 'NONE',  ( -0.000000000000000000, -0.000000000000000000, 1.000000000000000000 ) ) ;
#64191=CARTESIAN_POINT ( 'NONE',  ( 96.15314808468748708, -208.0026889286704943, 88.79614583420047325 ) ) ;
#64192=CARTESIAN_POINT ( 'NONE',  ( 96.32499999999997442, 92.29496732002878900, 79.62833333333333030 ) ) ;
#64195=CARTESIAN_POINT ( 'NONE',  ( -96.32499999999996021, -212.2949673200287179, 88.28020833506764120 ) ) ;
#64201=CARTESIAN_POINT ( 'NONE',  ( 97.30629616937498838, 88.66845928578037217, 89.43114583420049257 ) ) ;
#64211=CARTESIAN_POINT ( 'NONE',  ( -97.64998530214684536, 91.52998669916203767, 81.77145774807789280 ) ) ;
#64214=ORIENTED_EDGE ( 'NONE', *, *, #40858, .T. ) ;
#64215=CARTESIAN_POINT ( 'NONE',  ( 97.64999999999999147, -210.0000000255706709, 84.04687500080852658 ) ) ;
#64218=ORIENTED_EDGE ( 'NONE', *, *, #10256, .F. ) ;
#64219=CARTESIAN_POINT ( 'NONE',  ( -96.15314808468747287, -208.0026889286704943, 87.15572916753382060 ) ) ;
#64229=CARTESIAN_POINT ( 'NONE',  ( 94.99999999999998579, 92.66308142843932671, 80.59406250086715318 ) ) ;
#64232=FACE_OUTER_BOUND ( 'NONE', #51301, .T. ) ;
#64242=CARTESIAN_POINT ( 'NONE',  ( -97.30629616937501680, 90.00000000000004263, 85.19781250086714408 ) ) ;
#64244=EDGE_CURVE ( 'NONE', #16870, #71356, #55745, .T. ) ;
#64250=CARTESIAN_POINT ( 'NONE',  ( 93.67500000000001137, -207.7050326799711968, 76.00354166840097037 ) ) ;
#64255=CARTESIAN_POINT ( 'NONE',  ( 96.15314808468750130, -211.9973110713294489, 81.75822916753382685 ) ) ;
#64256=EDGE_CURVE ( 'NONE', #57167, #43311, #13346, .T. ) ;
#64258=EDGE_LOOP ( 'NONE', ( #14033, #52153, #60977, #57162, #73960 ) ) ;
#64262=CARTESIAN_POINT ( 'NONE',  ( -92.35000000000003695, 90.00000000000004263, 90.00000000000000000 ) ) ;
#64266=CARTESIAN_POINT ( 'NONE',  ( 97.30629616937498838, -208.6684592857803011, 78.10697916753383652 ) ) ;
#64277=CARTESIAN_POINT ( 'NONE',  ( 95.00000000000000000, -206.9400435732949575, 82.30062500173428930 ) ) ;
#64278=CARTESIAN_POINT ( 'NONE',  ( 97.64999999999997726, 91.52997821335252127, 89.73541666666666572 ) ) ;
#64289=CARTESIAN_POINT ( 'NONE',  ( 96.32499999999997442, 92.29496732002878900, 84.78770833506763438 ) ) ;
#64291=ORIENTED_EDGE ( 'NONE', *, *, #56987, .T. ) ;
#64298=LINE ( 'NONE', #53373, #18119 ) ;
#64300=CARTESIAN_POINT ( 'NONE',  ( -97.65000000000001990, 91.52997821335253548, 88.67708333333332860 ) ) ;
#64305=CARTESIAN_POINT ( 'NONE',  ( -97.30629616937497417, -211.3315407142195852, 82.07572916753380809 ) ) ;
#64308=CARTESIAN_POINT ( 'NONE',  ( 92.48632958231168288, -210.0000000000000284, 74.91808492278046572 ) ) ;
#64310=CARTESIAN_POINT ( 'NONE',  ( -97.30629616937497417, -211.3315407142195852, 75.72572916753381378 ) ) ;
#64317=EDGE_CURVE ( 'NONE', #25333, #23675, #70411, .T. ) ;
#64318=CARTESIAN_POINT ( 'NONE',  ( -95.00000000000002842, 87.33691857156074434, 78.37156250086714238 ) ) ;
#64321=B_SPLINE_CURVE_WITH_KNOTS ( 'NONE', 3,
 ( #6128, #11729, #34672, #6489, #57623, #12844, #47442, #29029, #63639, #29759, #64369, #18855, #35418, #46704, #52709, #1622, #51595, #29390 ),
 .UNSPECIFIED., .F., .F.,
 ( 4, 2, 2, 2, 2, 2, 2, 2, 4 ),
 ( -0.004093595874563310012, -0.003575961937392308637, -0.003058328000221307262, -0.002540694063050305887, -0.002023060125879304512, -0.001505426188708303137, -0.0009877922515373017617, -0.0004701583143663003866, 4.747562280470098844E-05 ),
 .UNSPECIFIED. ) ;
#64327=CARTESIAN_POINT ( 'NONE',  ( -92.34999999999999432, -209.9999999999999716, 90.00000000000000000 ) ) ;
#64330=CARTESIAN_POINT ( 'NONE',  ( -92.69370383062498320, -208.6684592857803011, 75.56697916753383026 ) ) ;
#64342=CARTESIAN_POINT ( 'NONE',  ( -92.35000000000003695, 90.00000000000004263, 86.50750000000000739 ) ) ;
#64350=CARTESIAN_POINT ( 'NONE',  ( 92.69370383062501162, -208.6684592857803295, 86.41489583420047893 ) ) ;
#64351=CARTESIAN_POINT ( 'NONE',  ( 96.15314808468748708, -208.0026889286704943, 87.68489583420048916 ) ) ;
#64354=CARTESIAN_POINT ( 'NONE',  ( 92.69370383062501162, -209.9999999999999716, 89.16656250086715829 ) ) ;
#64357=VERTEX_POINT ( 'NONE', #33170 ) ;
#64358=CARTESIAN_POINT ( 'NONE',  ( -95.00000000000002842, 87.33691857156074434, 80.43531250086715545 ) ) ;
#64361=CARTESIAN_POINT ( 'NONE',  ( -97.64999999999996305, -209.9999999999999716, 87.53937500173429953 ) ) ;
#64369=CARTESIAN_POINT ( 'NONE',  ( 93.46017751755557867, 87.90457393955796306, 74.96680960279266515 ) ) ;
#64370=ADVANCED_FACE ( 'NONE', ( #50472 ), #21901, .F. ) ;
#64375=CARTESIAN_POINT ( 'NONE',  ( 92.69370383062501162, -211.3315407142195852, 80.80572916753382628 ) ) ;
#64378=CARTESIAN_POINT ( 'NONE',  ( -92.35000000000003695, 90.00000000000004263, 90.00000000000000000 ) ) ;
#64385=CARTESIAN_POINT ( 'NONE',  ( -94.99999999999997158, -212.6630814284392557, 84.72156250086713669 ) ) ;
#64386=CARTESIAN_POINT ( 'NONE',  ( -97.30629616937501680, 90.00000000000004263, 84.08656250086716000 ) ) ;
#64389=CARTESIAN_POINT ( 'NONE',  ( 92.69370383062498320, 90.00000000000002842, 81.38781250086714181 ) ) ;
#64391=( BOUNDED_CURVE ( )  B_SPLINE_CURVE ( 2, ( #34174, #57117, #50715, #51092, #12343, #35283, #58210, #69139, #11239 ),
 .UNSPECIFIED., .F., .F. ) 
 B_SPLINE_CURVE_WITH_KNOTS ( ( 3, 2, 2, 2, 3 ),
 ( 0.3386766260338262002, 0.3386767459623536980, 0.3457325115032360840, 0.3527882770441184701, 0.3598440426530882807 ),
 .UNSPECIFIED. ) 
 CURVE ( )  GEOMETRIC_REPRESENTATION_ITEM ( )  RATIONAL_B_SPLINE_CURVE ( ( 0.9999954456811669390, 0.9999977228018773756, 1.000000000000000000, 0.8660254037844387076, 1.000000000000000000, 0.8660254037844387076, 1.000000000000000000, 0.8660254037844387076, 1.000000000000000000 ) ) 
 REPRESENTATION_ITEM ( '' )  );
#64398=CARTESIAN_POINT ( 'NONE',  ( -97.30629616937497417, -211.3315407142195852, 86.52072916753381548 ) ) ;
#64406=CARTESIAN_POINT ( 'NONE',  ( 97.64999999999999147, -209.9999999999999716, 89.04749999999999943 ) ) ;
#64407=CARTESIAN_POINT ( 'NONE',  ( -93.84685191531252713, 88.00268892867056536, 87.31447916753380412 ) ) ;
#64408=CARTESIAN_POINT ( 'NONE',  ( 95.04693102382854875, 87.35041560265749183, 75.00000002508419072 ) ) ;
#64409=DIRECTION ( 'NONE',  ( -0.8571673007021122226, 1.049727191138618572E-16, 0.5150380749100542666 ) ) ;
#64412=CARTESIAN_POINT ( 'NONE',  ( -94.99999999999997158, -206.9400435732949575, 78.41125000000000966 ) ) ;
#64414=CARTESIAN_POINT ( 'NONE',  ( -92.69370383062504004, 90.00000000000004263, 75.99031250086714806 ) ) ;
#64417=CLOSED_SHELL ( 'NONE', ( #16153, #53742, #2069, #73600, #43163, #43987, #39548, #73495, #20540, #72125, #1818, #20373, #15801, #20689, #10679, #72284, #16282, #43622, #26925, #30445, #15173, #50486, #3923, #61815, #11457, #827, #10784, #34099, #17586, #1888, #34747, #47978, #68144, #28174, #60532, #48950, #68515, #806, #19198, #17477, #16908, #59152, #67641, #40912, #39928, #74071, #19173, #5214, #59519, #1940, #68928, #44811, #20828, #61740, #53205, #39847, #23490, #56575, #28867, #56389, #58331, #26383, #15616, #46484, #34869, #33973, #41740, #58295, #32227, #46041, #27781, #57289, #70874, #1986, #14869, #59224, #13597, #41361, #58076, #48392, #39926, #1185, #38441, #63984, #65223, #74162, #10588, #57168, #45916, #73669, #27244, #35877, #40659, #15079, #66460, #69595, #68593, #26582, #46537, #12078, #23025, #52205, #46927, #38906, #15555, #10091, #21394, #67398, #63583, #42796, #45952, #17301, #64080, #42512, #18322, #50404, #61904, #36940, #69264, #63991, #28249, #71527, #18267, #28963, #27752, #62477, #3757, #56970, #7804, #60714, #17379, #57718, #33779, #60366, #42549, #57436, #24960, #68915, #2953, #34214, #31118, #54151, #31081, #38288, #25783, #54575, #19848, #58449, #64507, #9869, #60546, #32072, #68609, #13902, #51585, #2455, #31384, #46358, #44851, #30818, #31585, #49573, #30209, #71994, #37706, #23948, #74268, #46881, #38626, #38811, #42458, #68999, #11144, #10509, #72467, #9607, #57546, #64370, #19918, #3511, #20249, #16324, #24551, #65982, #51028, #46170, #23417, #2226, #39293, #7554, #63675, #60305, #25533, #31615, #17155, #63782, #13924, #4600, #556, #62706, #56510, #70031, #38255, #51174, #65770, #32483, #14001, #63752, #51843, #8938, #52218, #70764, #71102, #36341, #33780, #57053, #206, #60953, #15305, #26032, #19757, #61531, #53921, #12294, #13919, #7742, #31966, #466, #12552, #41444, #1265, #69597, #56450, #51406, #54920, #50927, #57787, #5617, #21579, #65534, #69585, #1967, #3613, #59651, #20785, #39837, #35485, #24204, #64022, #3033, #69172, #32259, #6899, #17990, #13596, #73332, #19768, #72902, #40754, #5694, #9650, #61948, #221, #33518, #55269, #63189, #10247, #37860, #45874, #2866, #14276, #65526, #53873 ) ) ;
#64421=CARTESIAN_POINT ( 'NONE',  ( -97.30629616937497417, -211.3315407142195852, 87.31447916753381833 ) ) ;
#64426=CARTESIAN_POINT ( 'NONE',  ( -97.30629616937497417, -211.3315407142195852, 77.15447916753382174 ) ) ;
#64430=CARTESIAN_POINT ( 'NONE',  ( -92.35000000000003695, 89.99999413691148220, 82.77687479895028844 ) ) ;
#64434=CARTESIAN_POINT ( 'NONE',  ( -92.69370383062504004, 89.06968786819598449, 74.84209103131394158 ) ) ;
#64435=CARTESIAN_POINT ( 'NONE',  ( 92.69370383062501162, -209.9999999999999716, 78.21281250086714465 ) ) ;
#64453=ORIENTED_EDGE ( 'NONE', *, *, #64597, .F. ) ;
#64454=CARTESIAN_POINT ( 'NONE',  ( 96.15314808468748708, 91.99731107132950569, 80.69989583420047552 ) ) ;
#64455=LINE ( 'NONE', #12926, #73181 ) ;
#64457=ORIENTED_EDGE ( 'NONE', *, *, #12546, .T. ) ;
#64464=CARTESIAN_POINT ( 'NONE',  ( 97.64999999999999147, 90.00000000000002842, 90.00000000000000000 ) ) ;
#64470=CARTESIAN_POINT ( 'NONE',  ( -97.64999999999996305, -209.9999999999999716, 78.01437500173430806 ) ) ;
#64471=DIRECTION ( 'NONE',  ( 1.000000000000000000, 0.000000000000000000, 0.000000000000000000 ) ) ;
#64473=CARTESIAN_POINT ( 'NONE',  ( 96.32499999999997442, 92.29496732002878900, 76.53270833506762472 ) ) ;
#64474=CARTESIAN_POINT ( 'NONE',  ( -92.35000000000003695, 90.00000000000004263, 76.42687500173430237 ) ) ;
#64476=CARTESIAN_POINT ( 'NONE',  ( 93.84685191531248449, 88.00268892867053694, 81.65239583420049030 ) ) ;
#64477=CARTESIAN_POINT ( 'NONE',  ( 96.32499999999998863, 87.70503267997126784, 75.60666666666665492 ) ) ;
#64485=ORIENTED_EDGE ( 'NONE', *, *, #44654, .F. ) ;
#64487=ORIENTED_EDGE ( 'NONE', *, *, #67054, .F. ) ;
#64492=CARTESIAN_POINT ( 'NONE',  ( -97.64999999999996305, -209.9999999999999716, 76.03000000000000114 ) ) ;
#64493=CARTESIAN_POINT ( 'NONE',  ( -96.15314808468745866, -211.9973110713294489, 78.47739583420049314 ) ) ;
#64501=CARTESIAN_POINT ( 'NONE',  ( 7.103376864691351012E-17, -120.0000000000000000, -85.59999999999999432 ) ) ;
#64502=DIRECTION ( 'NONE',  ( 1.000000000000000000, 0.000000000000000000, 0.000000000000000000 ) ) ;
#64506=CARTESIAN_POINT ( 'NONE',  ( 92.34999999999999432, 89.99997747911952217, 86.26937578065384571 ) ) ;
#64507=ADVANCED_FACE ( 'NONE', ( #8439 ), #2471, .F. ) ;
#64512=CARTESIAN_POINT ( 'NONE',  ( 93.84685191531248449, 91.99731107132950569, 82.71072916753381321 ) ) ;
#64513=CARTESIAN_POINT ( 'NONE',  ( -97.30629616937495996, -209.9999999999999716, 87.89656250086714806 ) ) ;
#64514=CARTESIAN_POINT ( 'NONE',  ( 92.35001655588500569, 91.52998777189721125, 79.23145767387346439 ) ) ;
#64517=CARTESIAN_POINT ( 'NONE',  ( -93.67499999999998295, -212.2949673200287179, 81.32166666666667254 ) ) ;
#64518=CARTESIAN_POINT ( 'NONE',  ( -96.15314808468751551, 88.00268892867056536, 75.14364583420046984 ) ) ;
#64519=CARTESIAN_POINT ( 'NONE',  ( 92.69370383062501162, -208.6684592857803011, 87.68489583420047495 ) ) ;
#64520=ORIENTED_EDGE ( 'NONE', *, *, #43256, .F. ) ;
#64523=ORIENTED_EDGE ( 'NONE', *, *, #50647, .T. ) ;
#64530=VERTEX_POINT ( 'NONE', #44874 ) ;
#64534=CARTESIAN_POINT ( 'NONE',  ( 97.30629616937498838, -208.6684592857803295, 81.91697916753383879 ) ) ;
#64539=CARTESIAN_POINT ( 'NONE',  ( 92.35000000000006537, -211.5299782133524786, 76.71791666666666742 ) ) ;
#64540=DIRECTION ( 'NONE',  ( 1.000000000000000000, 0.000000000000000000, 0.000000000000000000 ) ) ;
#64541=CARTESIAN_POINT ( 'NONE',  ( 95.00000000000000000, -206.9400435732949575, 83.49125000000000796 ) ) ;
#64543=VERTEX_POINT ( 'NONE', #27567 ) ;
#64544=ORIENTED_EDGE ( 'NONE', *, *, #5463, .T. ) ;
#64546=CARTESIAN_POINT ( 'NONE',  ( -92.35000000000003695, 90.00000000000004263, 75.07749999999998636 ) ) ;
#64549=CARTESIAN_POINT ( 'NONE',  ( -92.69370383062502583, 91.33154071421968467, 87.63197916753382799 ) ) ;
#64552=CARTESIAN_POINT ( 'NONE',  ( 97.30629616937498838, -209.9999999999999716, 89.32531250086714181 ) ) ;
#64553=CARTESIAN_POINT ( 'NONE',  ( 96.32499999999997442, 92.29496732002878900, 77.72333333333332916 ) ) ;
#64555=CARTESIAN_POINT ( 'NONE',  ( -96.32499999999996021, -207.7050326799711968, 89.33854166840096411 ) ) ;
#64557=CARTESIAN_POINT ( 'NONE',  ( -93.67499999999998295, -212.2949673200287179, 85.13166666666666060 ) ) ;
#64559=CARTESIAN_POINT ( 'NONE',  ( -95.00000000000002842, 93.05995642670501411, 85.47562500173431488 ) ) ;
#64560=CARTESIAN_POINT ( 'NONE',  ( 97.30629616937498838, 88.66845928578037217, 75.30239583420048177 ) ) ;
#64562=CARTESIAN_POINT ( 'NONE',  ( 2.499999999999979572, -90.00000000000000000, -280.0000000000000000 ) ) ;
#64565=FACE_OUTER_BOUND ( 'NONE', #16921, .T. ) ;
#64568=CARTESIAN_POINT ( 'NONE',  ( -93.84685191531248449, -208.0026889286704943, 74.82614583420047438 ) ) ;
#64574=CARTESIAN_POINT ( 'NONE',  ( -93.84685191531247028, -211.9973110713294489, 88.10822916753382117 ) ) ;
#64583=CARTESIAN_POINT ( 'NONE',  ( 93.67499999999998295, 92.29496732002878900, 86.71916666666666629 ) ) ;
#64587=CARTESIAN_POINT ( 'NONE',  ( 94.99999999999998579, 87.33691857156068750, 82.81656250086712134 ) ) ;
#64594=DIRECTION ( 'NONE',  ( -0.000000000000000000, -0.000000000000000000, 1.000000000000000000 ) ) ;
#64596=( BOUNDED_CURVE ( )  B_SPLINE_CURVE ( 2, ( #28705, #52001, #29804, #64412, #12150, #41471, #24190 ),
 .UNSPECIFIED., .F., .F. ) 
 B_SPLINE_CURVE_WITH_KNOTS ( ( 3, 2, 2, 3 ),
 ( 0.7499999999999996669, 0.7569444444444439757, 0.7638888888888883955, 0.7708333333333328152 ),
 .UNSPECIFIED. ) 
 CURVE ( )  GEOMETRIC_REPRESENTATION_ITEM ( )  RATIONAL_B_SPLINE_CURVE ( ( 1.000000000000006439, 0.8660254037844322683, 1.000000000000000000, 0.8660254037844387076, 1.000000000000000000, 0.8660254037844493658, 0.9999999999999893419 ) ) 
 REPRESENTATION_ITEM ( '' )  );
#64597=EDGE_CURVE ( 'NONE', #35941, #48178, #23318, .T. ) ;
#64598=CARTESIAN_POINT ( 'NONE',  ( 96.32499999999998863, -207.7050326799711968, 85.42270833506762528 ) ) ;
#64600=CARTESIAN_POINT ( 'NONE',  ( -93.84685191531252713, 88.00268892867056536, 86.67947916753381321 ) ) ;
#64616=CARTESIAN_POINT ( 'NONE',  ( 93.84685191531251292, -211.9973110713294489, 81.01739583420049939 ) ) ;
#64622=DIRECTION ( 'NONE',  ( -0.000000000000000000, -0.000000000000000000, 1.000000000000000000 ) ) ;
#64624=CARTESIAN_POINT ( 'NONE',  ( 97.30629616937498838, -209.9999999999999716, 78.05406250086716113 ) ) ;
#64626=ORIENTED_EDGE ( 'NONE', *, *, #37215, .T. ) ;
#64636=DIRECTION ( 'NONE',  ( -0.000000000000000000, -0.000000000000000000, 1.000000000000000000 ) ) ;
#64637=CARTESIAN_POINT ( 'NONE',  ( 92.35000000000000853, -209.9999999999999716, 83.72937500173429726 ) ) ;
#64638=CARTESIAN_POINT ( 'NONE',  ( 92.34999999999999432, 90.00000000000002842, 88.73000000000000398 ) ) ;
#64644=CARTESIAN_POINT ( 'NONE',  ( -96.15314808468752972, 91.99731107132950569, 87.15572916753382060 ) ) ;
#64646=CARTESIAN_POINT ( 'NONE',  ( 92.34999999999999432, 88.47002178664753558, 86.32229166840097889 ) ) ;
#64652=ORIENTED_EDGE ( 'NONE', *, *, #52908, .F. ) ;
#64660=CARTESIAN_POINT ( 'NONE',  ( -97.65000000000001990, 91.52997821335253548, 89.31208333333333371 ) ) ;
#64665=ORIENTED_EDGE ( 'NONE', *, *, #8653, .T. ) ;
#64666=CARTESIAN_POINT ( 'NONE',  ( 95.00000000000000000, -213.0599564267049857, 85.07875000000001364 ) ) ;
#64667=CARTESIAN_POINT ( 'NONE',  ( -92.69370383062498320, -208.6684592857803011, 81.75822916753381264 ) ) ;
#64681=CARTESIAN_POINT ( 'NONE',  ( -97.64999999996709334, -209.9999916080759306, 86.90410584369134028 ) ) ;
#64683=CARTESIAN_POINT ( 'NONE',  ( -96.15314808468752972, 91.99731107132950569, 89.69572916753382685 ) ) ;
#64687=AXIS2_PLACEMENT_3D ( 'NONE', #5485, #58436, #23493 ) ;
#64694=CARTESIAN_POINT ( 'NONE',  ( 95.04693102382874770, -212.6495843973424940, 75.00000002508419072 ) ) ;
#64696=CARTESIAN_POINT ( 'NONE',  ( -93.33920801875063944, -211.6002412367801071, 74.80065669543250806 ) ) ;
#64700=EDGE_CURVE ( 'NONE', #43660, #46588, #6501, .T. ) ;
#64703=CARTESIAN_POINT ( 'NONE',  ( 93.67500000000001137, -212.2949673200287179, 88.20083333333332121 ) ) ;
#64708=CIRCLE ( 'NONE', #29918, 3.299999999999969624 ) ;
#64717=CARTESIAN_POINT ( 'NONE',  ( 92.69370383062501162, -208.6684592857803295, 85.77989583420048803 ) ) ;
#64718=CARTESIAN_POINT ( 'NONE',  ( 97.30629616937498838, -208.6684592857803295, 86.99697916753382287 ) ) ;
#64720=CARTESIAN_POINT ( 'NONE',  ( 96.15314808468748708, -208.0026889286704943, 89.58989583420049030 ) ) ;
#64723=ORIENTED_EDGE ( 'NONE', *, *, #8347, .F. ) ;
#64724=CARTESIAN_POINT ( 'NONE',  ( -93.84685191531254134, 91.99731107132950569, 80.06489583420048461 ) ) ;
#64725=VERTEX_POINT ( 'NONE', #57997 ) ;
#64728=( BOUNDED_CURVE ( )  B_SPLINE_CURVE ( 2, ( #73743, #45579, #63234, #50064, #4614, #50812, #28254, #45199, #6095 ),
 .UNSPECIFIED., .F., .F. ) 
 B_SPLINE_CURVE_WITH_KNOTS ( ( 3, 2, 2, 2, 3 ),
 ( 0.5715170088666297055, 0.5785727743523534361, 0.5856285398932350450, 0.5926843054341167649, 0.5926843883797354717 ),
 .UNSPECIFIED. ) 
 CURVE ( )  GEOMETRIC_REPRESENTATION_ITEM ( )  RATIONAL_B_SPLINE_CURVE ( ( 1.000000000000000000, 0.8660254037844387076, 1.000000000000000000, 0.8660254037844387076, 1.000000000000000000, 0.8660254037844387076, 1.000000000000000000, 0.9999984250318816326, 0.9999968501007930888 ) ) 
 REPRESENTATION_ITEM ( '' )  );
#64735=EDGE_LOOP ( 'NONE', ( #24791, #37515, #38855, #6767 ) ) ;
#64741=AXIS2_PLACEMENT_3D ( 'NONE', #48780, #2225, #71328 ) ;
#64745=CARTESIAN_POINT ( 'NONE',  ( 93.84685191531249870, -208.0026889286704943, 81.91697916753381037 ) ) ;
#64751=EDGE_CURVE ( 'NONE', #24954, #16487, #71902, .T. ) ;
#64754=CARTESIAN_POINT ( 'NONE',  ( -92.69370383062498320, -209.9999999999999716, 82.97531250086714749 ) ) ;
#64756=CARTESIAN_POINT ( 'NONE',  ( -97.30629616937501680, 91.33154071421968467, 84.03364583420049883 ) ) ;
#64758=CARTESIAN_POINT ( 'NONE',  ( 97.30629616937498838, 88.66845928578037217, 80.38239583420049428 ) ) ;
#64759=VERTEX_POINT ( 'NONE', #24888 ) ;
#64760=DIRECTION ( 'NONE',  ( -0.000000000000000000, -0.000000000000000000, 1.000000000000000000 ) ) ;
#64762=CARTESIAN_POINT ( 'NONE',  ( -92.34999999999999432, -211.5299782133524218, 83.35895833506764063 ) ) ;
#64765=CARTESIAN_POINT ( 'NONE',  ( -94.99999999999997158, -207.3369185715606307, 81.86406250086713499 ) ) ;
#64770=CARTESIAN_POINT ( 'NONE',  ( 97.64999999999999147, 90.00000000000002842, 78.88750000000000284 ) ) ;
#64775=ORIENTED_EDGE ( 'NONE', *, *, #7744, .F. ) ;
#64780=CARTESIAN_POINT ( 'NONE',  ( -97.30629616937501680, 91.33154071421968467, 88.31989583420046586 ) ) ;
#64788=CARTESIAN_POINT ( 'NONE',  ( -95.00000000000002842, 92.66308142843932671, 74.87906250086713555 ) ) ;
#64791=CARTESIAN_POINT ( 'NONE',  ( 92.35000000000000853, -208.4700217866474645, 84.31145833506762699 ) ) ;
#64793=CARTESIAN_POINT ( 'NONE',  ( -96.15314808468747287, -208.0026889286704943, 86.52072916753382970 ) ) ;
#64799=EDGE_CURVE ( 'NONE', #4573, #9802, #69977, .T. ) ;
#64800=DIRECTION ( 'NONE',  ( -0.000000000000000000, -0.000000000000000000, 1.000000000000000000 ) ) ;
#64802=CARTESIAN_POINT ( 'NONE',  ( -97.30629616937497417, -208.6684592857803295, 77.68364583420047609 ) ) ;
#64803=CARTESIAN_POINT ( 'NONE',  ( 94.99999999999998579, 93.05995642670504253, 88.57124999999999204 ) ) ;
#64805=CARTESIAN_POINT ( 'NONE',  ( 97.64999999999999147, 89.99999996655866141, 87.85687500050293863 ) ) ;
#64806=CARTESIAN_POINT ( 'NONE',  ( -94.99999999999997158, -209.9999999999999716, 90.00000000000000000 ) ) ;
#64811=CARTESIAN_POINT ( 'NONE',  ( 97.30629616937498838, -208.6684592857803011, 76.04322916753380923 ) ) ;
#64820=ORIENTED_EDGE ( 'NONE', *, *, #9020, .F. ) ;
#64828=( BOUNDED_CURVE ( )  B_SPLINE_CURVE ( 2, ( #19769, #66398, #55477, #31786, #8872, #2544, #3988, #71641, #43840 ),
 .UNSPECIFIED., .F., .F. ) 
 B_SPLINE_CURVE_WITH_KNOTS ( ( 3, 2, 2, 2, 3 ),
 ( 0.4021785743327777052, 0.4021786358302963382, 0.4092344013711782802, 0.4162901669120601666, 0.4233457466685772164 ),
 .UNSPECIFIED. ) 
 CURVE ( )  GEOMETRIC_REPRESENTATION_ITEM ( )  RATIONAL_B_SPLINE_CURVE ( ( 0.9999976645954666843, 0.9999988322875555946, 1.000000000000000000, 0.8660254037844387076, 1.000000000000000000, 0.8660254037844387076, 1.000000000000000000, 0.8660289314505905667, 0.9999929448534692344 ) ) 
 REPRESENTATION_ITEM ( '' )  );
#64829=CARTESIAN_POINT ( 'NONE',  ( 94.99999999999998579, 92.66308142843935514, 80.75281250086715090 ) ) ;
#64831=CARTESIAN_POINT ( 'NONE',  ( 93.67500000000001137, -207.7050326799711968, 75.92416666666666458 ) ) ;
#64840=CARTESIAN_POINT ( 'NONE',  ( -95.67252605959640732, 92.31128197830616955, 74.85222950654855367 ) ) ;
#64843=EDGE_CURVE ( 'NONE', #4256, #36714, #3709, .T. ) ;
#64844=CARTESIAN_POINT ( 'NONE',  ( -92.34999999999992326, 88.47002178664760663, 78.19958333333332234 ) ) ;
#64846=CARTESIAN_POINT ( 'NONE',  ( -97.64999999999996305, -209.9999999999999716, 78.64937500173429896 ) ) ;
#64849=CARTESIAN_POINT ( 'NONE',  ( 96.32499999999998863, 87.70503267997126784, 75.05104166840095559 ) ) ;
#64850=CARTESIAN_POINT ( 'NONE',  ( -97.65000000000001990, 90.00000000000004263, 76.10937500173430692 ) ) ;
#64852=CARTESIAN_POINT ( 'NONE',  ( 97.30629616937498838, 91.33154071421968467, 76.83697916753382628 ) ) ;
#64855=CARTESIAN_POINT ( 'NONE',  ( 95.00000000000000000, -209.9999999999999716, 90.00000000000000000 ) ) ;
#64856=CARTESIAN_POINT ( 'NONE',  ( 97.65000000000000568, -211.5299782133524218, 77.64395833506762301 ) ) ;
#64860=ORIENTED_EDGE ( 'NONE', *, *, #17808, .T. ) ;
#64871=CARTESIAN_POINT ( 'NONE',  ( -94.99999999999997158, -212.6630814284392557, 78.53031250086715431 ) ) ;
#64887=CARTESIAN_POINT ( 'NONE',  ( -92.34999999999999432, -208.4700217866474645, 77.74979166840097378 ) ) ;
#64888=LINE ( 'NONE', #28243, #47831 ) ;
#64890=EDGE_CURVE ( 'NONE', #45343, #66667, #49654, .T. ) ;
#64891=CARTESIAN_POINT ( 'NONE',  ( 96.15314808468748708, 91.99731107132950569, 84.50989583420049200 ) ) ;
#64892=CARTESIAN_POINT ( 'NONE',  ( -96.15314808468747287, -208.0026889286704943, 85.25072916753381946 ) ) ;
#64896=CARTESIAN_POINT ( 'NONE',  ( -92.34999999999999432, -209.9999999999999716, 80.15749999999999886 ) ) ;
#64897=CARTESIAN_POINT ( 'NONE',  ( -92.69370383062505425, 91.33154071421968467, 77.94822916753381037 ) ) ;
#64898=CARTESIAN_POINT ( 'NONE',  ( 97.30629616937498838, -208.6684592857803011, 87.47322916753381605 ) ) ;
#64910=CARTESIAN_POINT ( 'NONE',  ( 93.84685191531249870, -208.0026889286704943, 82.07572916753382231 ) ) ;
#64912=CARTESIAN_POINT ( 'NONE',  ( 95.00000000000000000, -209.9999999999999716, 90.00000000000000000 ) ) ;
#64916=CARTESIAN_POINT ( 'NONE',  ( 95.00000000000000000, -213.0599564267049857, 85.71374999999997613 ) ) ;
#64919=ORIENTED_EDGE ( 'NONE', *, *, #28240, .T. ) ;
#64924=DIRECTION ( 'NONE',  ( -1.000000000000000000, 0.000000000000000000, 0.000000000000000000 ) ) ;
#64929=CARTESIAN_POINT ( 'NONE',  ( -97.30629616937501680, 88.66845928578038638, 87.31447916753381833 ) ) ;
#64932=CARTESIAN_POINT ( 'NONE',  ( -92.34999999999998010, 88.47002178664759242, 83.91458333333333997 ) ) ;
#64933=CARTESIAN_POINT ( 'NONE',  ( 92.69370383062501162, -211.3315407142195852, 87.15572916753380639 ) ) ;
#64936=ORIENTED_EDGE ( 'NONE', *, *, #14016, .T. ) ;
#64937=CARTESIAN_POINT ( 'NONE',  ( -97.64999999999996305, -209.9999999999999716, 88.80937500173430976 ) ) ;
#64938=EDGE_LOOP ( 'NONE', ( #69242, #27531, #17142, #36810, #57003 ) ) ;
#64941=CARTESIAN_POINT ( 'NONE',  ( -95.00000000000002842, 86.94004357329504273, 85.79312500173431033 ) ) ;
#64942=CARTESIAN_POINT ( 'NONE',  ( 97.30629616937498838, 88.66845928578037217, 88.79614583420050167 ) ) ;
#64945=CARTESIAN_POINT ( 'NONE',  ( -97.64999999989191792, -209.9999848944890175, 78.64888723590522090 ) ) ;
#64948=VERTEX_POINT ( 'NONE', #25629 ) ;
#64950=CARTESIAN_POINT ( 'NONE',  ( -92.35000000000553655, 89.99999459739531460, 81.50687481489494246 ) ) ;
#64957=CARTESIAN_POINT ( 'NONE',  ( -92.69370383062498320, -208.6684592857803011, 86.36197916753383197 ) ) ;
#64958=ORIENTED_EDGE ( 'NONE', *, *, #62312, .F. ) ;
#64969=CARTESIAN_POINT ( 'NONE',  ( 92.69370383062498320, 91.33154071421968467, 89.74864583420048803 ) ) ;
#64971=CARTESIAN_POINT ( 'NONE',  ( 94.99999999999998579, 92.66308142843932671, 81.22906250086714408 ) ) ;
#64973=CARTESIAN_POINT ( 'NONE',  ( -97.65000000000001990, 90.00000000000004263, 88.09499999999999886 ) ) ;
#64985=CARTESIAN_POINT ( 'NONE',  ( -92.69370383062504004, 90.00000000000004263, 84.88031250086713442 ) ) ;
#64990=DIRECTION ( 'NONE',  ( 1.000000000000000000, 0.000000000000000000, 0.000000000000000000 ) ) ;
#64994=DIRECTION ( 'NONE',  ( -1.343011723336883198E-16, 1.000000000000000000, 0.000000000000000000 ) ) ;
#64996=CARTESIAN_POINT ( 'NONE',  ( 92.69370383062501162, -211.3315407142195852, 82.23447916753383424 ) ) ;
#64997=EDGE_LOOP ( 'NONE', ( #8790, #66254, #65116, #61955 ) ) ;
#64998=ORIENTED_EDGE ( 'NONE', *, *, #10383, .T. ) ;
#64999=CARTESIAN_POINT ( 'NONE',  ( -96.32499999999996021, -207.7050326799711968, 86.08416666666666117 ) ) ;
#65002=CARTESIAN_POINT ( 'NONE',  ( 92.69370383062501162, -209.9999999999999716, 75.03781250086713328 ) ) ;
#65004=CARTESIAN_POINT ( 'NONE',  ( 97.30629616937498838, -211.3315407142195852, 81.17614583420048291 ) ) ;
#65016=CARTESIAN_POINT ( 'NONE',  ( -92.35000000000000853, 91.52997821335252127, 82.75041666666666629 ) ) ;
#65017=VERTEX_POINT ( 'NONE', #62073 ) ;
#65019=CARTESIAN_POINT ( 'NONE',  ( 95.00000000000000000, -206.9400435732949575, 82.93562500173429441 ) ) ;
#65021=CARTESIAN_POINT ( 'NONE',  ( 97.64999999999999147, 90.00000000000002842, 87.77749999999998920 ) ) ;
#65022=EDGE_CURVE ( 'NONE', #47168, #64184, #5318, .T. ) ;
#65029=CARTESIAN_POINT ( 'NONE',  ( -97.30629616937501680, 88.66845928578038638, 88.58447916753382856 ) ) ;
#65030=CARTESIAN_POINT ( 'NONE',  ( 96.15314808468748708, 88.00268892867053694, 84.13947916753380696 ) ) ;
#65032=CARTESIAN_POINT ( 'NONE',  ( 92.34999999999999432, 90.00000000000002842, 87.53937500173429953 ) ) ;
#65044=CARTESIAN_POINT ( 'NONE',  ( -97.65000000000001990, 90.00000000000004263, 83.65000000000000568 ) ) ;
#65046=CARTESIAN_POINT ( 'NONE',  ( -97.64999999953499810, 89.99996900126896548, 83.09538598081491045 ) ) ;
#65047=( BOUNDED_CURVE ( )  B_SPLINE_CURVE ( 2, ( #30567, #20411, #26411, #53512, #71151, #48964, #2048, #19292, #65541 ),
 .UNSPECIFIED., .F., .F. ) 
 B_SPLINE_CURVE_WITH_KNOTS ( ( 3, 2, 2, 2, 3 ),
 ( 0.4868478063952913493, 0.4939035878641909738, 0.5009593534051074437, 0.5080151189460238026, 0.5080151867278726030 ),
 .UNSPECIFIED. ) 
 CURVE ( )  GEOMETRIC_REPRESENTATION_ITEM ( )  RATIONAL_B_SPLINE_CURVE ( ( 1.000000000000000000, 0.8660254037844387076, 1.000000000000000000, 0.8660254037844387076, 1.000000000000000000, 0.8660254037844387076, 1.000000000000000000, 0.9999987129609425596, 0.9999974259466133386 ) ) 
 REPRESENTATION_ITEM ( '' )  );
#65051=CARTESIAN_POINT ( 'NONE',  ( -97.30629616937495996, -209.9999999999999716, 83.92781250086714806 ) ) ;
#65060=CARTESIAN_POINT ( 'NONE',  ( 92.35000000010803944, 90.00001510551041406, 78.64888723592453346 ) ) ;
#65062=CARTESIAN_POINT ( 'NONE',  ( 97.30629616937498838, -210.2956651733038314, 74.79348190356851944 ) ) ;
#65065=CARTESIAN_POINT ( 'NONE',  ( -97.30629616937501680, 90.00000000000004263, 75.67281250086713840 ) ) ;
#65068=( BOUNDED_SURFACE ( )  B_SPLINE_SURFACE ( 1, 2, ( 
 ( #56294, #27712, #22075, #62700, #22827, #46123, #17540, #67944, #39371, #57037, #45770, #62313, #69057, #10797, #33724, #70139, #19011, #69411, #6996, #35939, #6634, #17914, #13000, #64156, #12636, #19385, #7741, #47230, #23555, #41583, #41966, #35568, #47971, #24662, #58499, #58884, #42335, #64519, #40857, #29546, #12268, #64898, #46483, #69779, #7379, #30295, #29921, #63795, #53237, #57774, #52120, #35199, #41217, #52483, #666, #1776, #13376, #58137, #47592, #6279, #1036, #52871, #29178, #65267, #23931, #13740, #53601, #46867, #36308, #25030, #59248, #70499, #30659, #2140, #18282, #1411, #70884, #24303, #18640, #49801, #26511, #65635, #8105, #48699, #14107, #31030, #53989, #71622, #21225, #71242, #48335, #25769, #49440, #72721, #61100, #2525, #71999, #44176, #67102, #36678, #14485, #25409, #60372, #37057, #59625, #55079, #19749, #26871, #72368, #3612, #20118, #43460, #54713, #66742, #3974, #37443, #42698, #43083, #66015, #20867, #60006, #15228, #9215, #8490, #31404, #43822, #54353, #8855, #66383, #37806, #31769, #2875, #14858, #3242, #26130, #49068, #20506, #60739, #32134, #38158, #9598, #32513, #55458, #38539, #27233, #10703, #15608, #23109, #50165, #217, #11436, #38909, #51291, #57311, #22741, #16724, #62978, #74222, #33247, #56197, #68603, #32875, #61476, #28731, #5458, #44557, #9957, #27625, #67478, #55826, #4343, #50548, #46039, #73100, #21607, #4719, #28354, #51670, #40026, #15968, #50922, #61845, #10329, #73474, #67852, #21983, #39284, #44928, #16344, #34002, #62216, #5823, #45683, #56949, #33632, #22359, #56584, #17091, #5086, #27986, #73844, #45305, #68223, #34371, #39660, #62599, #11080, #18919, #40767, #575, #69325, #69698, #30573, #17817, #63708, #18194, #64435, #47507, #7653, #23469, #12177, #46778, #58413, #35115, #30207, #58051, #53149, #6911, #1689, #6192, #41137, #47147, #6552, #29094, #24217, #945, #23836, #53516, #41862, #29826, #34752, #52784, #24575, #64073, #59162, #35842, #12548, #70055, #2054, #1328, #52030, #57693, #18556, #70413, #41495, #35482, #36219, #64811, #13289, #12909, #24940, #68967, #17453, #29454, #40383, #58793, #7293, #63334, #11794, #46399, #52398, #13653, #65181, #37351, #14399, #49983, #72903, #48249, #65920, #19299, #25322, #8021, #73288, #25681, #39096 ),
 ( #55637, #61290, #4527, #16159, #48615, #36586, #8399, #54265, #67292, #30939, #27427, #21406, #21795, #19662, #53886, #71156, #71529, #10511, #42610, #65545, #20029, #44366, #50364, #62034, #2433, #14020, #42988, #9777, #36964, #10142, #59911, #33062, #32692, #56008, #59535, #4154, #27051, #31316, #2793, #15791, #38727, #61656, #33435, #44747, #67668, #56399, #4908, #47870, #70794, #42247, #69155, #57136, #6017, #63890, #11614, #39473, #51111, #56770, #34937, #16526, #39849, #57504, #28919, #5645, #10900, #34556, #27806, #22175, #62419, #11261, #74037, #45115, #51854, #57872, #5275, #400, #50734, #33820, #22932, #73660, #35306, #28176, #12362, #23651, #22548, #58233, #28540, #68038, #51478, #45492, #40957, #46221, #68423, #18014, #63523, #17643, #62799, #23294, #45868, #6377, #69513, #37, #16912, #34191, #68794, #40575, #17274, #29279, #11999, #52220, #40208, #63155, #764, #46584, #42791, #7097, #30018, #30387, #2238, #59717, #19843, #12725, #52965, #58981, #70597, #1504, #42426, #24393, #65364, #19115, #13829, #18370, #53332, #59347, #47326, #41313, #36400, #13099, #36035, #65727, #31128, #42063, #46959, #64996, #36770, #7471, #71337, #48065, #1869, #7836, #14206, #13472, #64255, #70228, #35658, #8197, #69872, #18735, #30748, #53696, #24753, #58597, #25133, #6733, #1135, #41675, #64616, #47687, #24034, #70977, #54081, #19476, #2616, #29640, #25494, #48428, #52583, #37160, #20214, #44661, #55921, #8950, #21318, #27335, #67203, #61200, #32974, #44276, #3335, #26228, #38639, #2971, #31497, #73203, #49897, #14581, #54441, #72092, #37530, #25859, #48791, #20601, #67575, #43182, #71712, #49167, #72817, #21704, #10056, #66108, #20962, #16073, #60104, #15703, #60470, #43553, #15318, #9687, #37898, #31867, #66833, #8583, #54806, #66472, #14959, #60826, #9308, #32610, #61571, #32229, #55551, #55179, #3705, #26600, #49530, #72458, #43915, #38257, #4436, #4070, #50270, #26967, #63073, #28453, #5922, #17187, #62321, #10808, #34466, #33340, #61941, #46134, #68703, #22086, #10424, #33734, #45026, #56303, #4821, #56681, #17548, #50644, #27721, #5182, #40120, #23204, #28830, #73569, #11173, #40481, #39009, #67950, #51384, #28087, #74323, #22458, #16439, #69064, #51025, #39379, #73947, #45398, #11532, #68325, #16820 ) ),
 .UNSPECIFIED., .F., .F., .F. ) 
 B_SPLINE_SURFACE_WITH_KNOTS ( ( 2, 2 ),
 ( 3, 2, 2, 2, 2, 2, 2, 2, 2, 2, 2, 2, 2, 2, 2, 2, 2, 2, 2, 2, 2, 2, 2, 2, 2, 2, 2, 2, 2, 2, 2, 2, 2, 2, 2, 2, 2, 2, 2, 2, 2, 2, 2, 2, 2, 2, 2, 2, 2, 2, 2, 2, 2, 2, 2, 2, 2, 2, 2, 2, 2, 2, 2, 2, 2, 2, 2, 2, 2, 2, 2, 2, 2, 2, 2, 2, 2, 2, 2, 2, 2, 2, 2, 2, 2, 2, 2, 2, 2, 2, 2, 2, 2, 2, 2, 2, 2, 2, 2, 2, 2, 2, 2, 2, 2, 2, 2, 2, 2, 2, 2, 2, 2, 2, 2, 2, 2, 2, 2, 2, 2, 2, 2, 2, 2, 2, 2, 2, 2, 2, 2, 2, 2, 2, 2, 2, 2, 2, 2, 2, 2, 2, 3 ),
 ( 0.000000000000000000, 1.000000000000000000 ),
 ( 0.000000000000000000, 0.006944444444444444059, 0.01388888888888888812, 0.02083333333333333218, 0.02777777777777777624, 0.03472222222222222376, 0.04166666666666666435, 0.04861111111111111188, 0.05555555555555555247, 0.06250000000000000000, 0.06944444444444444753, 0.07638888888888889506, 0.08333333333333332871, 0.09027777777777777624, 0.09722222222222222376, 0.1041666666666666713, 0.1111111111111111049, 0.1180555555555555525, 0.1250000000000000000, 0.1319444444444444475, 0.1388888888888888951, 0.1458333333333333426, 0.1527777777777777901, 0.1597222222222222099, 0.1666666666666666574, 0.1736111111111111049, 0.1805555555555555525, 0.1875000000000000000, 0.1944444444444444475, 0.2013888888888888951, 0.2083333333333333426, 0.2152777777777777901, 0.2222222222222222099, 0.2291666666666666574, 0.2361111111111111049, 0.2430555555555555525, 0.2500000000000000000, 0.2569444444444444198, 0.2638888888888888951, 0.2708333333333333148, 0.2777777777777777901, 0.2847222222222222099, 0.2916666666666666852, 0.2986111111111111049, 0.3055555555555555802, 0.3125000000000000000, 0.3194444444444444198, 0.3263888888888888951, 0.3333333333333333148, 0.3402777777777777901, 0.3472222222222222099, 0.3541666666666666852, 0.3611111111111111049, 0.3680555555555555802, 0.3750000000000000000, 0.3819444444444444198, 0.3888888888888888951, 0.3958333333333333148, 0.4027777777777777901, 0.4097222222222222099, 0.4166666666666666852, 0.4236111111111111049, 0.4305555555555555802, 0.4375000000000000000, 0.4444444444444444198, 0.4513888888888888951, 0.4583333333333333148, 0.4652777777777777901, 0.4722222222222222099, 0.4791666666666666852, 0.4861111111111111049, 0.4930555555555555802, 0.5000000000000000000, 0.5069444444444444198, 0.5138888888888888395, 0.5208333333333333703, 0.5277777777777777901, 0.5347222222222222099, 0.5416666666666666297, 0.5486111111111111605, 0.5555555555555555802, 0.5625000000000000000, 0.5694444444444444198, 0.5763888888888888395, 0.5833333333333333703, 0.5902777777777777901, 0.5972222222222222099, 0.6041666666666666297, 0.6111111111111111605, 0.6180555555555555802, 0.6250000000000000000, 0.6319444444444444198, 0.6388888888888888395, 0.6458333333333333703, 0.6527777777777777901, 0.6597222222222222099, 0.6666666666666666297, 0.6736111111111111605, 0.6805555555555555802, 0.6875000000000000000, 0.6944444444444444198, 0.7013888888888888395, 0.7083333333333333703, 0.7152777777777777901, 0.7222222222222222099, 0.7291666666666666297, 0.7361111111111111605, 0.7430555555555555802, 0.7500000000000000000, 0.7569444444444444198, 0.7638888888888888395, 0.7708333333333333703, 0.7777777777777777901, 0.7847222222222222099, 0.7916666666666666297, 0.7986111111111111605, 0.8055555555555555802, 0.8125000000000000000, 0.8194444444444444198, 0.8263888888888888395, 0.8333333333333333703, 0.8402777777777777901, 0.8472222222222222099, 0.8541666666666666297, 0.8611111111111111605, 0.8680555555555555802, 0.8750000000000000000, 0.8819444444444444198, 0.8888888888888888395, 0.8958333333333333703, 0.9027777777777777901, 0.9097222222222222099, 0.9166666666666666297, 0.9236111111111111605, 0.9305555555555555802, 0.9375000000000000000, 0.9444444444444444198, 0.9513888888888888395, 0.9583333333333333703, 0.9652777777777777901, 0.9722222222222222099, 0.9791666666666666297, 0.9842227634901432598 ),
 .UNSPECIFIED. ) 
 GEOMETRIC_REPRESENTATION_ITEM ( )  RATIONAL_B_SPLINE_SURFACE ( (
 ( 1.000000000000000000, 0.8660254037844387076, 1.000000000000000000, 0.8660254037844387076, 1.000000000000000000, 0.8660254037844387076, 1.000000000000000000, 0.8660254037844387076, 1.000000000000000000, 0.8660254037844387076, 1.000000000000000000, 0.8660254037844387076, 1.000000000000000000, 0.8660254037844387076, 1.000000000000000000, 0.8660254037844387076, 1.000000000000000000, 0.8660254037844387076, 1.000000000000000000, 0.8660254037844387076, 1.000000000000000000, 0.8660254037844387076, 1.000000000000000000, 0.8660254037844387076, 1.000000000000000000, 0.8660254037844387076, 1.000000000000000000, 0.8660254037844387076, 1.000000000000000000, 0.8660254037844387076, 1.000000000000000000, 0.8660254037844387076, 1.000000000000000000, 0.8660254037844387076, 1.000000000000000000, 0.8660254037844387076, 1.000000000000000000, 0.8660254037844387076, 1.000000000000000000, 0.8660254037844387076, 1.000000000000000000, 0.8660254037844387076, 1.000000000000000000, 0.8660254037844387076, 1.000000000000000000, 0.8660254037844387076, 1.000000000000000000, 0.8660254037844387076, 1.000000000000000000, 0.8660254037844387076, 1.000000000000000000, 0.8660254037844387076, 1.000000000000000000, 0.8660254037844387076, 1.000000000000000000, 0.8660254037844387076, 1.000000000000000000, 0.8660254037844387076, 1.000000000000000000, 0.8660254037844387076, 1.000000000000000000, 0.8660254037844387076, 1.000000000000000000, 0.8660254037844387076, 1.000000000000000000, 0.8660254037844387076, 1.000000000000000000, 0.8660254037844387076, 1.000000000000000000, 0.8660254037844387076, 1.000000000000000000, 0.8660254037844387076, 1.000000000000000000, 0.8660254037844387076, 1.000000000000000000, 0.8660254037844387076, 1.000000000000000000, 0.8660254037844387076, 1.000000000000000000, 0.8660254037844387076, 1.000000000000000000, 0.8660254037844387076, 1.000000000000000000, 0.8660254037844387076, 1.000000000000000000, 0.8660254037844387076, 1.000000000000000000, 0.8660254037844387076, 1.000000000000000000, 0.8660254037844387076, 1.000000000000000000, 0.8660254037844387076, 1.000000000000000000, 0.8660254037844387076, 1.000000000000000000, 0.8660254037844387076, 1.000000000000000000, 0.8660254037844387076, 1.000000000000000000, 0.8660254037844387076, 1.000000000000000000, 0.8660254037844387076, 1.000000000000000000, 0.8660254037844387076, 1.000000000000000000, 0.8660254037844387076, 1.000000000000000000, 0.8660254037844387076, 1.000000000000000000, 0.8660254037844387076, 1.000000000000000000, 0.8660254037844387076, 1.000000000000000000, 0.8660254037844387076, 1.000000000000000000, 0.8660254037844387076, 1.000000000000000000, 0.8660254037844387076, 1.000000000000000000, 0.8660254037844387076, 1.000000000000000000, 0.8660254037844387076, 1.000000000000000000, 0.8660254037844387076, 1.000000000000000000, 0.8660254037844387076, 1.000000000000000000, 0.8660254037844387076, 1.000000000000000000, 0.8660254037844387076, 1.000000000000000000, 0.8660254037844387076, 1.000000000000000000, 0.8660254037844387076, 1.000000000000000000, 0.8660254037844387076, 1.000000000000000000, 0.8660254037844387076, 1.000000000000000000, 0.8660254037844387076, 1.000000000000000000, 0.8660254037844387076, 1.000000000000000000, 0.8660254037844387076, 1.000000000000000000, 0.8660254037844387076, 1.000000000000000000, 0.8660254037844387076, 1.000000000000000000, 0.8660254037844387076, 1.000000000000000000, 0.8660254037844387076, 1.000000000000000000, 0.8660254037844387076, 1.000000000000000000, 0.8660254037844387076, 1.000000000000000000, 0.8660254037844387076, 1.000000000000000000, 0.8660254037844387076, 1.000000000000000000, 0.8660254037844387076, 1.000000000000000000, 0.8660254037844387076, 1.000000000000000000, 0.8660254037844387076, 1.000000000000000000, 0.8660254037844387076, 1.000000000000000000, 0.8660254037844387076, 1.000000000000000000, 0.8660254037844387076, 1.000000000000000000, 0.8660254037844387076, 1.000000000000000000, 0.8660254037844387076, 1.000000000000000000, 0.8660254037844387076, 1.000000000000000000, 0.8660254037844387076, 1.000000000000000000, 0.8660254037844387076, 1.000000000000000000, 0.8660254037844387076, 1.000000000000000000, 0.8660254037844387076, 1.000000000000000000, 0.8660254037844387076, 1.000000000000000000, 0.8660254037844387076, 1.000000000000000000, 0.8660254037844387076, 1.000000000000000000, 0.8660254037844387076, 1.000000000000000000, 0.8660254037844387076, 1.000000000000000000, 0.8660254037844387076, 1.000000000000000000, 0.8660254037844387076, 1.000000000000000000, 0.8660254037844387076, 1.000000000000000000, 0.8660254037844387076, 1.000000000000000000, 0.8660254037844387076, 1.000000000000000000, 0.8660254037844387076, 1.000000000000000000, 0.8660254037844387076, 1.000000000000000000, 0.8660254037844387076, 1.000000000000000000, 0.8660254037844387076, 1.000000000000000000, 0.8660254037844387076, 1.000000000000000000, 0.8660254037844387076, 1.000000000000000000, 0.8660254037844387076, 1.000000000000000000, 0.8660254037844387076, 1.000000000000000000, 0.8660254037844387076, 1.000000000000000000, 0.8660254037844387076, 1.000000000000000000, 0.8660254037844387076, 1.000000000000000000, 0.8660254037844387076, 1.000000000000000000, 0.8660254037844387076, 1.000000000000000000, 0.8660254037844387076, 1.000000000000000000, 0.8660254037844387076, 1.000000000000000000, 0.8660254037844387076, 1.000000000000000000, 0.8660254037844387076, 1.000000000000000000, 0.8660254037844387076, 1.000000000000000000, 0.8660254037844387076, 1.000000000000000000, 0.8660254037844387076, 1.000000000000000000, 0.8660254037844387076, 1.000000000000000000, 0.8660254037844387076, 1.000000000000000000, 0.8660254037844387076, 1.000000000000000000, 0.8660254037844387076, 1.000000000000000000, 0.8660254037844387076, 1.000000000000000000, 0.8660254037844387076, 1.000000000000000000, 0.8660254037844387076, 1.000000000000000000, 0.8660254037844387076, 1.000000000000000000, 0.8660254037844387076, 1.000000000000000000, 0.8660254037844387076, 1.000000000000000000, 0.8660254037844387076, 1.000000000000000000, 0.8660254037844387076, 1.000000000000000000, 0.8660254037844387076, 1.000000000000000000, 0.8660254037844387076, 1.000000000000000000, 0.8660254037844387076, 1.000000000000000000, 0.8660254037844387076, 1.000000000000000000, 0.8660254037844387076, 1.000000000000000000, 0.8660254037844387076, 1.000000000000000000, 0.9024560516293040902, 0.9469512977404621612),
 ( 1.000000000000000000, 0.8660254037844387076, 1.000000000000000000, 0.8660254037844387076, 1.000000000000000000, 0.8660254037844387076, 1.000000000000000000, 0.8660254037844387076, 1.000000000000000000, 0.8660254037844387076, 1.000000000000000000, 0.8660254037844387076, 1.000000000000000000, 0.8660254037844387076, 1.000000000000000000, 0.8660254037844387076, 1.000000000000000000, 0.8660254037844387076, 1.000000000000000000, 0.8660254037844387076, 1.000000000000000000, 0.8660254037844387076, 1.000000000000000000, 0.8660254037844387076, 1.000000000000000000, 0.8660254037844387076, 1.000000000000000000, 0.8660254037844387076, 1.000000000000000000, 0.8660254037844387076, 1.000000000000000000, 0.8660254037844387076, 1.000000000000000000, 0.8660254037844387076, 1.000000000000000000, 0.8660254037844387076, 1.000000000000000000, 0.8660254037844387076, 1.000000000000000000, 0.8660254037844387076, 1.000000000000000000, 0.8660254037844387076, 1.000000000000000000, 0.8660254037844387076, 1.000000000000000000, 0.8660254037844387076, 1.000000000000000000, 0.8660254037844387076, 1.000000000000000000, 0.8660254037844387076, 1.000000000000000000, 0.8660254037844387076, 1.000000000000000000, 0.8660254037844387076, 1.000000000000000000, 0.8660254037844387076, 1.000000000000000000, 0.8660254037844387076, 1.000000000000000000, 0.8660254037844387076, 1.000000000000000000, 0.8660254037844387076, 1.000000000000000000, 0.8660254037844387076, 1.000000000000000000, 0.8660254037844387076, 1.000000000000000000, 0.8660254037844387076, 1.000000000000000000, 0.8660254037844387076, 1.000000000000000000, 0.8660254037844387076, 1.000000000000000000, 0.8660254037844387076, 1.000000000000000000, 0.8660254037844387076, 1.000000000000000000, 0.8660254037844387076, 1.000000000000000000, 0.8660254037844387076, 1.000000000000000000, 0.8660254037844387076, 1.000000000000000000, 0.8660254037844387076, 1.000000000000000000, 0.8660254037844387076, 1.000000000000000000, 0.8660254037844387076, 1.000000000000000000, 0.8660254037844387076, 1.000000000000000000, 0.8660254037844387076, 1.000000000000000000, 0.8660254037844387076, 1.000000000000000000, 0.8660254037844387076, 1.000000000000000000, 0.8660254037844387076, 1.000000000000000000, 0.8660254037844387076, 1.000000000000000000, 0.8660254037844387076, 1.000000000000000000, 0.8660254037844387076, 1.000000000000000000, 0.8660254037844387076, 1.000000000000000000, 0.8660254037844387076, 1.000000000000000000, 0.8660254037844387076, 1.000000000000000000, 0.8660254037844387076, 1.000000000000000000, 0.8660254037844387076, 1.000000000000000000, 0.8660254037844387076, 1.000000000000000000, 0.8660254037844387076, 1.000000000000000000, 0.8660254037844387076, 1.000000000000000000, 0.8660254037844387076, 1.000000000000000000, 0.8660254037844387076, 1.000000000000000000, 0.8660254037844387076, 1.000000000000000000, 0.8660254037844387076, 1.000000000000000000, 0.8660254037844387076, 1.000000000000000000, 0.8660254037844387076, 1.000000000000000000, 0.8660254037844387076, 1.000000000000000000, 0.8660254037844387076, 1.000000000000000000, 0.8660254037844387076, 1.000000000000000000, 0.8660254037844387076, 1.000000000000000000, 0.8660254037844387076, 1.000000000000000000, 0.8660254037844387076, 1.000000000000000000, 0.8660254037844387076, 1.000000000000000000, 0.8660254037844387076, 1.000000000000000000, 0.8660254037844387076, 1.000000000000000000, 0.8660254037844387076, 1.000000000000000000, 0.8660254037844387076, 1.000000000000000000, 0.8660254037844387076, 1.000000000000000000, 0.8660254037844387076, 1.000000000000000000, 0.8660254037844387076, 1.000000000000000000, 0.8660254037844387076, 1.000000000000000000, 0.8660254037844387076, 1.000000000000000000, 0.8660254037844387076, 1.000000000000000000, 0.8660254037844387076, 1.000000000000000000, 0.8660254037844387076, 1.000000000000000000, 0.8660254037844387076, 1.000000000000000000, 0.8660254037844387076, 1.000000000000000000, 0.8660254037844387076, 1.000000000000000000, 0.8660254037844387076, 1.000000000000000000, 0.8660254037844387076, 1.000000000000000000, 0.8660254037844387076, 1.000000000000000000, 0.8660254037844387076, 1.000000000000000000, 0.8660254037844387076, 1.000000000000000000, 0.8660254037844387076, 1.000000000000000000, 0.8660254037844387076, 1.000000000000000000, 0.8660254037844387076, 1.000000000000000000, 0.8660254037844387076, 1.000000000000000000, 0.8660254037844387076, 1.000000000000000000, 0.8660254037844387076, 1.000000000000000000, 0.8660254037844387076, 1.000000000000000000, 0.8660254037844387076, 1.000000000000000000, 0.8660254037844387076, 1.000000000000000000, 0.8660254037844387076, 1.000000000000000000, 0.8660254037844387076, 1.000000000000000000, 0.8660254037844387076, 1.000000000000000000, 0.8660254037844387076, 1.000000000000000000, 0.8660254037844387076, 1.000000000000000000, 0.8660254037844387076, 1.000000000000000000, 0.8660254037844387076, 1.000000000000000000, 0.8660254037844387076, 1.000000000000000000, 0.8660254037844387076, 1.000000000000000000, 0.8660254037844387076, 1.000000000000000000, 0.8660254037844387076, 1.000000000000000000, 0.8660254037844387076, 1.000000000000000000, 0.8660254037844387076, 1.000000000000000000, 0.8660254037844387076, 1.000000000000000000, 0.8660254037844387076, 1.000000000000000000, 0.8660254037844387076, 1.000000000000000000, 0.8660254037844387076, 1.000000000000000000, 0.8660254037844387076, 1.000000000000000000, 0.8660254037844387076, 1.000000000000000000, 0.8660254037844387076, 1.000000000000000000, 0.8660254037844387076, 1.000000000000000000, 0.8660254037844387076, 1.000000000000000000, 0.8660254037844387076, 1.000000000000000000, 0.8660254037844387076, 1.000000000000000000, 0.8660254037844387076, 1.000000000000000000, 0.8660254037844387076, 1.000000000000000000, 0.8660254037844387076, 1.000000000000000000, 0.8660254037844387076, 1.000000000000000000, 0.8660254037844387076, 1.000000000000000000, 0.8660254037844387076, 1.000000000000000000, 0.8660254037844387076, 1.000000000000000000, 0.8660254037844387076, 1.000000000000000000, 0.8660254037844387076, 1.000000000000000000, 0.8660254037844387076, 1.000000000000000000, 0.8660254037844387076, 1.000000000000000000, 0.8660254037844387076, 1.000000000000000000, 0.8660254037844387076, 1.000000000000000000, 0.8660254037844387076, 1.000000000000000000, 0.8660254037844387076, 1.000000000000000000, 0.9024560516293040902, 0.9469512977404621612) ) ) 
 REPRESENTATION_ITEM ( '' )  SURFACE ( )  );
#65076=CARTESIAN_POINT ( 'NONE',  ( -97.64999999999994884, -208.4700217866474645, 89.31208333333333371 ) ) ;
#65078=CARTESIAN_POINT ( 'NONE',  ( 100.0010000000000190, -123.9999999999999858, 39.99999999999996447 ) ) ;
#65079=AXIS2_PLACEMENT_3D ( 'NONE', #58083, #23498, #40413 ) ;
#65084=CARTESIAN_POINT ( 'NONE',  ( -92.35000000000003695, 90.00000000000004263, 84.60249999999999204 ) ) ;
#65091=VERTEX_POINT ( 'NONE', #79 ) ;
#65092=CARTESIAN_POINT ( 'NONE',  ( 92.69370383062501162, -208.6684592857803295, 85.14489583420045449 ) ) ;
#65093=CARTESIAN_POINT ( 'NONE',  ( 92.69370383062501162, -211.3315407142195852, 88.58447916753382856 ) ) ;
#65096=CARTESIAN_POINT ( 'NONE',  ( 92.69370383062501162, -211.3315407142195852, 88.58447916753382856 ) ) ;
#65099=EDGE_CURVE ( 'NONE', #51207, #58350, #10937, .T. ) ;
#65100=CARTESIAN_POINT ( 'NONE',  ( -94.99999999999997158, -213.0599564267049857, 80.63375000000000625 ) ) ;
#65102=CARTESIAN_POINT ( 'NONE',  ( -96.15314808468752972, 91.99731107132950569, 79.53572916753381605 ) ) ;
#65104=EDGE_CURVE ( 'NONE', #25068, #19568, #10688, .T. ) ;
#65116=ORIENTED_EDGE ( 'NONE', *, *, #56436, .F. ) ;
#65117=VERTEX_POINT ( 'NONE', #61701 ) ;
#65119=CARTESIAN_POINT ( 'NONE',  ( 93.84685191531249870, -208.0026889286704943, 78.74197916753381321 ) ) ;
#65120=CARTESIAN_POINT ( 'NONE',  ( -92.35000000000017906, 91.52997821335260653, 83.38541666666667140 ) ) ;
#65129=CARTESIAN_POINT ( 'NONE',  ( -97.30629616937497417, -208.6684592857803011, 80.06489583420047040 ) ) ;
#65131=CARTESIAN_POINT ( 'NONE',  ( -96.15314808468751551, 88.00268892867056536, 77.84239583420048803 ) ) ;
#65135=CARTESIAN_POINT ( 'NONE',  ( 92.69370383062498320, 88.66845928578037217, 80.17072916753379275 ) ) ;
#65140=CARTESIAN_POINT ( 'NONE',  ( 94.99999999999998579, 86.94004357329502852, 77.53812500173428646 ) ) ;
#65143=CARTESIAN_POINT ( 'NONE',  ( -92.69370383062498320, -211.3315407142195852, 81.65239583420047609 ) ) ;
#65150=EDGE_CURVE ( 'NONE', #48479, #21836, #49347, .T. ) ;
#65153=CARTESIAN_POINT ( 'NONE',  ( -94.46769236096046995, 86.73322217287214642, 74.92222617501695936 ) ) ;
#65155=CARTESIAN_POINT ( 'NONE',  ( -97.30629616937501680, 88.66845928578038638, 83.98072916753380923 ) ) ;
#65158=CARTESIAN_POINT ( 'NONE',  ( 92.34999999999999432, 88.47002178664752137, 81.24229166840096639 ) ) ;
#65161=CARTESIAN_POINT ( 'NONE',  ( -93.84685191531252713, 88.00268892867056536, 76.51947916753380241 ) ) ;
#65165=CARTESIAN_POINT ( 'NONE',  ( -94.99999999999997158, -206.9400435732949575, 79.12562500173429214 ) ) ;
#65166=CARTESIAN_POINT ( 'NONE',  ( -96.15314808468747287, -208.0026889286704943, 87.79072916753381151 ) ) ;
#65169=CARTESIAN_POINT ( 'NONE',  ( 93.84685191531248449, 91.99731107132950569, 75.09072916753380866 ) ) ;
#65171=CARTESIAN_POINT ( 'NONE',  ( -97.30629616937495996, -209.9999999999999716, 77.10156250086714635 ) ) ;
#65174=FACE_OUTER_BOUND ( 'NONE', #53151, .T. ) ;
#65179=SHAPE_REPRESENTATION ( 'housing', ( #43395 ), #14652 ) ;
#65181=CARTESIAN_POINT ( 'NONE',  ( 96.15314808468750130, -211.9973110713294489, 75.24947916753380639 ) ) ;
#65199=CARTESIAN_POINT ( 'NONE',  ( 92.69370383062498320, 90.00000000000002842, 78.37156250086715659 ) ) ;
#65210=CARTESIAN_POINT ( 'NONE',  ( -93.41453557521646189, 91.70561969393801860, 74.79912739178801928 ) ) ;
#65211=DIRECTION ( 'NONE',  ( 1.000000000000000000, 0.000000000000000000, 0.000000000000000000 ) ) ;
#65215=CARTESIAN_POINT ( 'NONE',  ( -92.34999999999999432, -209.9999999999999716, 77.06187500173429328 ) ) ;
#65216=EDGE_CURVE ( 'NONE', #52827, #45343, #28564, .T. ) ;
#65217=CARTESIAN_POINT ( 'NONE',  ( -96.15314808468752972, 91.99731107132950569, 88.42572916753381662 ) ) ;
#65220=CARTESIAN_POINT ( 'NONE',  ( 92.34999999999999432, 88.47002178664753558, 77.43229166840096411 ) ) ;
#65221=CARTESIAN_POINT ( 'NONE',  ( -93.67500000000003979, 92.29496732002878900, 77.16770833506762983 ) ) ;
#65223=ADVANCED_FACE ( 'NONE', ( #805 ), #68827, .F. ) ;
#65224=CARTESIAN_POINT ( 'NONE',  ( 93.84685191531248449, 88.00268892867053694, 77.84239583420048803 ) ) ;
#65226=CARTESIAN_POINT ( 'NONE',  ( 97.64999999999999147, 90.00000000000002842, 90.00000000000000000 ) ) ;
#65227=CARTESIAN_POINT ( 'NONE',  ( 96.32499999999998863, -207.7050326799711968, 77.16770833506762983 ) ) ;
#65243=AXIS2_PLACEMENT_3D ( 'NONE', #14746, #14384, #30924 ) ;
#65245=AXIS2_PLACEMENT_3D ( 'NONE', #62631, #5852, #17119 ) ;
#65256=DIRECTION ( 'NONE',  ( 0.4565542962317865050, 0.000000000000000000, 0.8896955516311735312 ) ) ;
#65257=CARTESIAN_POINT ( 'NONE',  ( 97.64999999999999147, 90.00000000000002842, 90.00000000000000000 ) ) ;
#65258=EDGE_CURVE ( 'NONE', #44809, #30760, #30427, .T. ) ;
#65259=CARTESIAN_POINT ( 'NONE',  ( 92.69370383062498320, 90.00000000000002842, 83.45156250086715488 ) ) ;
#65260=CARTESIAN_POINT ( 'NONE',  ( -93.84685191531247028, -211.9973110713294489, 88.10822916753382117 ) ) ;
#65261=CARTESIAN_POINT ( 'NONE',  ( 92.35000000000000853, -209.9999999999999716, 90.00000000000000000 ) ) ;
#65263=CARTESIAN_POINT ( 'NONE',  ( -97.64999999999984936, -211.5299782133525071, 81.16291666666667481 ) ) ;
#65264=CARTESIAN_POINT ( 'NONE',  ( -93.67499999999998295, -212.2949673200287179, 80.68666666666665321 ) ) ;
#65265=CARTESIAN_POINT ( 'NONE',  ( -97.30629616937501680, 88.66845928578038638, 75.72572916753381378 ) ) ;
#65267=CARTESIAN_POINT ( 'NONE',  ( 95.00000000000000000, -207.3369185715606307, 86.30906250086715659 ) ) ;
#65273=( BOUNDED_CURVE ( )  B_SPLINE_CURVE ( 2, ( #18603, #17502, #69740, #40816, #63753, #29141, #47556 ),
 .UNSPECIFIED., .F., .F. ) 
 B_SPLINE_CURVE_WITH_KNOTS ( ( 3, 2, 2, 3 ),
 ( 0.1693384224419976214, 0.1763941385220586799, 0.1834499040629413436, 0.1905056698837213069 ),
 .UNSPECIFIED. ) 
 CURVE ( )  GEOMETRIC_REPRESENTATION_ITEM ( )  RATIONAL_B_SPLINE_CURVE ( ( 0.9999981216929294536, 0.8660263429445574923, 1.000000000000000000, 0.8660254037844387076, 1.000000000000000000, 0.8660254037844387076, 1.000000000000000000 ) ) 
 REPRESENTATION_ITEM ( '' )  );
#65278=CARTESIAN_POINT ( 'NONE',  ( -97.65000000000001990, 88.47002178664754979, 79.33729166840096525 ) ) ;
#65282=CARTESIAN_POINT ( 'NONE',  ( 92.69370383062501162, -208.6684592857803295, 79.58864583420049144 ) ) ;
#65284=FACE_OUTER_BOUND ( 'NONE', #32159, .T. ) ;
#65287=CARTESIAN_POINT ( 'NONE',  ( 94.99999999999998579, 86.94004357329502852, 76.82374999999998977 ) ) ;
#65288=VECTOR ( 'NONE', #59800, 1000.000000000000000 ) ;
#65291=CARTESIAN_POINT ( 'NONE',  ( 92.35000000000002274, -208.4700217866474645, 80.42208333333331893 ) ) ;
#65299=CARTESIAN_POINT ( 'NONE',  ( -97.30629616937501680, 88.66845928578038638, 82.86947916753382515 ) ) ;
#65302=CARTESIAN_POINT ( 'NONE',  ( 97.64999999999997726, 88.47002178664753558, 75.65958333333333030 ) ) ;
#65304=CARTESIAN_POINT ( 'NONE',  ( -97.64999999999994884, -208.4700217866474645, 88.12145833506762926 ) ) ;
#65306=ORIENTED_EDGE ( 'NONE', *, *, #58490, .T. ) ;
#65310=CARTESIAN_POINT ( 'NONE',  ( -92.35000000000003695, 90.00000000000004263, 84.68187500173429783 ) ) ;
#65312=CARTESIAN_POINT ( 'NONE',  ( 93.84685191531248449, 91.99731107132950569, 85.25072916753381946 ) ) ;
#65316=DIRECTION ( 'NONE',  ( 1.000000000000000000, 0.000000000000000000, 0.000000000000000000 ) ) ;
#65323=FACE_OUTER_BOUND ( 'NONE', #69966, .T. ) ;
#65327=CARTESIAN_POINT ( 'NONE',  ( -92.69370383062498320, -208.6684592857803011, 89.53697916753382913 ) ) ;
#65330=ORIENTED_EDGE ( 'NONE', *, *, #8212, .F. ) ;
#65334=CARTESIAN_POINT ( 'NONE',  ( 97.30629616937498838, 90.00000000000002842, 88.84906250086716284 ) ) ;
#65335=CARTESIAN_POINT ( 'NONE',  ( 94.99999999999998579, 90.00000000000002842, 75.00000000000000000 ) ) ;
#65336=CARTESIAN_POINT ( 'NONE',  ( 97.30629616937498838, 91.33154071421968467, 82.39322916753381776 ) ) ;
#65337=DIRECTION ( 'NONE',  ( 0.8571673007021122226, 0.000000000000000000, 0.5150380749100542666 ) ) ;
#65339=CARTESIAN_POINT ( 'NONE',  ( -97.64999999999997726, 91.52997821335256390, 85.50208333333331723 ) ) ;
#65344=AXIS2_PLACEMENT_3D ( 'NONE', #45043, #16463, #39399 ) ;
#65351=CARTESIAN_POINT ( 'NONE',  ( -92.69370383062505425, 88.66845928578038638, 86.73239583420047438 ) ) ;
#65361=CARTESIAN_POINT ( 'NONE',  ( 92.34999999999999432, 90.00000000000002842, 82.37999999999999545 ) ) ;
#65364=CARTESIAN_POINT ( 'NONE',  ( 96.15314808468750130, -211.9973110713294489, 83.02822916753380866 ) ) ;
#65365=ORIENTED_EDGE ( 'NONE', *, *, #11964, .T. ) ;
#65370=EDGE_CURVE ( 'NONE', #11290, #57825, #19296, .T. ) ;
#65375=CARTESIAN_POINT ( 'NONE',  ( 92.69370383062501162, -209.9999999999999716, 79.00656250086716170 ) ) ;
#65383=CARTESIAN_POINT ( 'NONE',  ( -93.67500000000003979, 92.29496732002878900, 82.80333333333332746 ) ) ;
#65385=CARTESIAN_POINT ( 'NONE',  ( 92.35000000000002274, -211.5299782133524502, 82.51229166840094820 ) ) ;
#65386=CARTESIAN_POINT ( 'NONE',  ( 93.67499999999999716, 87.70503267997126784, 86.29583333333333428 ) ) ;
#65388=DIRECTION ( 'NONE',  ( 0.000000000000000000, 0.000000000000000000, -1.000000000000000000 ) ) ;
#65390=CARTESIAN_POINT ( 'NONE',  ( -94.95306897617113862, 87.35041560265752025, 75.00000002508417651 ) ) ;
#65394=CARTESIAN_POINT ( 'NONE',  ( -92.69370383062505425, 91.33154071421968467, 86.99697916753382287 ) ) ;
#65397=CARTESIAN_POINT ( 'NONE',  ( 94.99999999999998579, 92.66308142843935514, 80.59406250086715318 ) ) ;
#65400=CARTESIAN_POINT ( 'NONE',  ( 94.99999999999998579, 86.94004357329500010, 85.79312500173431033 ) ) ;
#65409=LINE ( 'NONE', #31172, #37288 ) ;
#65410=CARTESIAN_POINT ( 'NONE',  ( 1.243286885786405054E-17, -120.0000000000000000, -80.00000000000001421 ) ) ;
#65412=CARTESIAN_POINT ( 'NONE',  ( -96.32500000000001705, 87.70503267997129626, 83.75583333333332803 ) ) ;
#65414=DIRECTION ( 'NONE',  ( -0.000000000000000000, -0.000000000000000000, 1.000000000000000000 ) ) ;
#65419=CARTESIAN_POINT ( 'NONE',  ( -97.30629616937495996, -209.9999999999999716, 82.65781250086713783 ) ) ;
#65423=CARTESIAN_POINT ( 'NONE',  ( 92.34999999999999432, 90.00000000000002842, 89.44437500173430067 ) ) ;
#65430=CARTESIAN_POINT ( 'NONE',  ( 97.64999999997402824, 89.99998827382246702, 82.77687459617033028 ) ) ;
#65432=CARTESIAN_POINT ( 'NONE',  ( -92.69370383062504004, 90.00000000000004263, 75.35531250086714294 ) ) ;
#65446=CARTESIAN_POINT ( 'NONE',  ( -92.34999999999999432, -208.4700217866474645, 86.56041666666665435 ) ) ;
#65447=EDGE_CURVE ( 'NONE', #44202, #17922, #36264, .T. ) ;
#65450=ORIENTED_EDGE ( 'NONE', *, *, #5244, .T. ) ;
#65462=CARTESIAN_POINT ( 'NONE',  ( 92.69370383062501162, -211.3315407142195852, 83.34572916753381833 ) ) ;
#65463=CARTESIAN_POINT ( 'NONE',  ( 97.30629616937498838, -209.9999999999999716, 88.84906250086716284 ) ) ;
#65466=CARTESIAN_POINT ( 'NONE',  ( 97.30629616937498838, -208.6684592857803011, 88.90197916753382401 ) ) ;
#65472=CARTESIAN_POINT ( 'NONE',  ( -96.15314808468751551, 88.00268892867056536, 75.93739583420048689 ) ) ;
#65477=VERTEX_POINT ( 'NONE', #39429 ) ;
#65478=CARTESIAN_POINT ( 'NONE',  ( 96.32499999999998863, -207.7050326799711968, 84.78770833506763438 ) ) ;
#65481=EDGE_CURVE ( 'NONE', #52479, #66194, #5549, .T. ) ;
#65483=( BOUNDED_CURVE ( )  B_SPLINE_CURVE ( 2, ( #30569, #52780, #59531, #19294, #53145, #47505, #46395 ),
 .UNSPECIFIED., .F., .F. ) 
 B_SPLINE_CURVE_WITH_KNOTS ( ( 3, 2, 2, 3 ),
 ( 0.06350193517735455706, 0.07055765540882334708, 0.07761342094970608008, 0.08466915177892317401 ),
 .UNSPECIFIED. ) 
 CURVE ( )  GEOMETRIC_REPRESENTATION_ITEM ( )  RATIONAL_B_SPLINE_CURVE ( ( 0.9999982793443398243, 0.8660262641177934873, 1.000000000000000000, 0.8660254037844387076, 1.000000000000000000, 0.8660260628881689682, 0.9999986817990245136 ) ) 
 REPRESENTATION_ITEM ( '' )  );
#65488=CARTESIAN_POINT ( 'NONE',  ( 97.30629616937498838, -211.3315407142195852, 78.47739583420047893 ) ) ;
#65498=CARTESIAN_POINT ( 'NONE',  ( -96.15314808468747287, -208.0026889286704943, 82.55197916753380127 ) ) ;
#65499=CARTESIAN_POINT ( 'NONE',  ( -97.30629616937501680, 91.33154071421968467, 78.95364583420048632 ) ) ;
#65501=CARTESIAN_POINT ( 'NONE',  ( 97.30629616937498838, 88.66845928578037217, 81.01739583420048518 ) ) ;
#65509=CARTESIAN_POINT ( 'NONE',  ( -92.69370383062498320, -209.9999999999999716, 81.70531250086713726 ) ) ;
#65516=CARTESIAN_POINT ( 'NONE',  ( -95.00000000000002842, 86.94004357329504273, 76.18874999999999886 ) ) ;
#65518=CARTESIAN_POINT ( 'NONE',  ( -97.30629616937501680, 91.33154071421968467, 83.87489583420047268 ) ) ;
#65519=CARTESIAN_POINT ( 'NONE',  ( -96.44578755843112106, -208.0396902886533894, 74.86947676125085138 ) ) ;
#65524=CARTESIAN_POINT ( 'NONE',  ( -97.30629616937501680, 91.33154071421968467, 74.98489583420048632 ) ) ;
#65526=ADVANCED_FACE ( 'NONE', ( #21753 ), #22129, .T. ) ;
#65532=CARTESIAN_POINT ( 'NONE',  ( 93.67499999999999716, 87.70503267997126784, 86.29583333333333428 ) ) ;
#65533=CARTESIAN_POINT ( 'NONE',  ( -94.99999999999997158, -212.6630814284392557, 81.70531250086715147 ) ) ;
#65534=ADVANCED_FACE ( 'NONE', ( #73247 ), #50694, .F. ) ;
#65541=CARTESIAN_POINT ( 'NONE',  ( -97.64999999993850111, -209.9999881787635729, 81.82400613094797848 ) ) ;
#65543=CARTESIAN_POINT ( 'NONE',  ( 15.70000000000000284, -120.0000000000000000, -90.00000000000000000 ) ) ;
#65545=CARTESIAN_POINT ( 'NONE',  ( 97.30629616937498838, -211.3315407142195852, 88.79614583420050167 ) ) ;
#65551=ORIENTED_EDGE ( 'NONE', *, *, #49158, .T. ) ;
#65557=EDGE_CURVE ( 'NONE', #47974, #5670, #38686, .T. ) ;
#65559=ORIENTED_EDGE ( 'NONE', *, *, #64597, .T. ) ;
#65570=CARTESIAN_POINT ( 'NONE',  ( 92.69370383062498320, 91.33154071421968467, 81.49364583420047836 ) ) ;
#65575=ORIENTED_EDGE ( 'NONE', *, *, #50937, .F. ) ;
#65581=CARTESIAN_POINT ( 'NONE',  ( -97.64999999990722301, -209.9999861897314304, 80.55392363651652943 ) ) ;
#65585=DIRECTION ( 'NONE',  ( 1.000000000000000000, 0.000000000000000000, 0.000000000000000000 ) ) ;
#65586=CARTESIAN_POINT ( 'NONE',  ( -93.67499999999998295, -212.2949673200287179, 76.95604166840095672 ) ) ;
#65587=CARTESIAN_POINT ( 'NONE',  ( -92.69370383062504004, 90.00000000000004263, 88.84906250086716284 ) ) ;
#65588=CARTESIAN_POINT ( 'NONE',  ( 93.67499999999999716, 87.70503267997126784, 77.48520833506763950 ) ) ;
#65589=CARTESIAN_POINT ( 'NONE',  ( -92.35000000000003695, 90.00000000000004263, 77.69687500173431260 ) ) ;
#65591=CARTESIAN_POINT ( 'NONE',  ( 94.99999999999998579, 87.33691857156068750, 76.62531250086715318 ) ) ;
#65620=CARTESIAN_POINT ( 'NONE',  ( -92.35000000000000853, -208.4700217866474929, 87.19541666666667368 ) ) ;
#65622=CARTESIAN_POINT ( 'NONE',  ( -92.35000000000000853, -209.9999996502046429, 77.69687501385436690 ) ) ;
#65627=CARTESIAN_POINT ( 'NONE',  ( 92.69370383062498320, 91.33154071421968467, 84.03364583420049883 ) ) ;
#65628=CARTESIAN_POINT ( 'NONE',  ( -92.69370383062498320, -209.9999999999999716, 86.30906250086715659 ) ) ;
#65629=CARTESIAN_POINT ( 'NONE',  ( 97.65000000000000568, -211.5299782133524218, 83.99395833506763154 ) ) ;
#65632=CARTESIAN_POINT ( 'NONE',  ( -94.99999999999997158, -206.9400435732949575, 82.85625000000000284 ) ) ;
#65633=LINE ( 'NONE', #55823, #46195 ) ;
#65635=CARTESIAN_POINT ( 'NONE',  ( 95.00000000000000000, -212.6630814284392557, 85.35656250086714181 ) ) ;
#65641=VERTEX_POINT ( 'NONE', #64215 ) ;
#65642=CARTESIAN_POINT ( 'NONE',  ( 92.35000000000000853, -209.9999999999999716, 84.28499999999999659 ) ) ;
#65645=CARTESIAN_POINT ( 'NONE',  ( 92.69370383062501162, -209.9999999999999716, 77.73656250086715147 ) ) ;
#65651=CARTESIAN_POINT ( 'NONE',  ( -93.09170270117142820, -211.8387227684682159, 74.99954709728268654 ) ) ;
#65652=CARTESIAN_POINT ( 'NONE',  ( 97.64999999999997726, -208.4700217866474645, 82.11541666666666117 ) ) ;
#65658=DIRECTION ( 'NONE',  ( -0.000000000000000000, -0.000000000000000000, -1.000000000000000000 ) ) ;
#65659=CARTESIAN_POINT ( 'NONE',  ( -92.69370383062502583, 91.33154071421968467, 83.18697916753382060 ) ) ;
#65661=AXIS2_PLACEMENT_3D ( 'NONE', #8092, #24285, #18623 ) ;
#65663=CARTESIAN_POINT ( 'NONE',  ( 94.15631797925330204, 85.30516711421525144, 74.84535815546860249 ) ) ;
#65666=CARTESIAN_POINT ( 'NONE',  ( -92.34999999999999432, -208.4700217866474645, 86.00479166840096923 ) ) ;
#65671=ORIENTED_EDGE ( 'NONE', *, *, #1649, .F. ) ;
#65672=CARTESIAN_POINT ( 'NONE',  ( -96.32500000000001705, 87.70503267997129626, 86.37520833506764006 ) ) ;
#65674=CARTESIAN_POINT ( 'NONE',  ( 96.15314808468748708, 88.00268892867053694, 87.47322916753381605 ) ) ;
#65675=VECTOR ( 'NONE', #69862, 1000.000000000000000 ) ;
#65676=DIRECTION ( 'NONE',  ( -1.000000000000000000, 0.000000000000000000, 0.000000000000000000 ) ) ;
#65677=DIRECTION ( 'NONE',  ( -0.000000000000000000, -0.000000000000000000, 1.000000000000000000 ) ) ;
#65678=CARTESIAN_POINT ( 'NONE',  ( 97.64999999999999147, -209.9999999999999716, 90.00000000000000000 ) ) ;
#65680=ORIENTED_EDGE ( 'NONE', *, *, #36155, .T. ) ;
#65686=EDGE_CURVE ( 'NONE', #59366, #22794, #63849, .T. ) ;
#65692=CARTESIAN_POINT ( 'NONE',  ( -96.15314808468745866, -211.9973110713294489, 82.92239583420048632 ) ) ;
#65702=CARTESIAN_POINT ( 'NONE',  ( 92.69370383062498320, 90.00000000000002842, 80.11781250086713158 ) ) ;
#65706=CARTESIAN_POINT ( 'NONE',  ( 95.99319914654111585, 92.13398380010835353, 74.81432998548488911 ) ) ;
#65709=( BOUNDED_CURVE ( )  B_SPLINE_CURVE ( 2, ( #16933, #10917, #56416, #68810, #39871, #28199, #33842, #28558, #28942 ),
 .UNSPECIFIED., .F., .F. ) 
 B_SPLINE_CURVE_WITH_KNOTS ( ( 3, 2, 2, 2, 3 ),
 ( 0.8255245790564498254, 0.8325803338241194451, 0.8396360993650018312, 0.8466918649058842172, 0.8466920362367558184 ),
 .UNSPECIFIED. ) 
 CURVE ( )  GEOMETRIC_REPRESENTATION_ITEM ( )  RATIONAL_B_SPLINE_CURVE ( ( 1.000000000000000000, 0.8660254037844387076, 1.000000000000000000, 0.8660254037844387076, 1.000000000000000000, 0.8660254037844387076, 1.000000000000000000, 0.9999967467762058693, 0.9999934937104038024 ) ) 
 REPRESENTATION_ITEM ( '' )  );
#65710=EDGE_CURVE ( 'NONE', #16558, #11817, #11363, .T. ) ;
#65714=CARTESIAN_POINT ( 'NONE',  ( -92.34999999999999432, -209.9999999999999716, 90.00000000000000000 ) ) ;
#65716=CARTESIAN_POINT ( 'NONE',  ( -92.69370383062505425, 88.66845928578038638, 86.09739583420048348 ) ) ;
#65722=ORIENTED_EDGE ( 'NONE', *, *, #5398, .T. ) ;
#65725=DIRECTION ( 'NONE',  ( -0.000000000000000000, -0.000000000000000000, 1.000000000000000000 ) ) ;
#65727=CARTESIAN_POINT ( 'NONE',  ( 97.30629616937498838, -211.3315407142195852, 82.44614583420049314 ) ) ;
#65736=CARTESIAN_POINT ( 'NONE',  ( 95.46326757314950839, -212.8430781844920432, 74.72378867588406592 ) ) ;
#65738=CARTESIAN_POINT ( 'NONE',  ( 94.99999999999998579, 86.94004357329502852, 79.36374999999996760 ) ) ;
#65746=CARTESIAN_POINT ( 'NONE',  ( 97.64999999999997726, -208.4700217866474645, 84.73479166840097321 ) ) ;
#65747=CARTESIAN_POINT ( 'NONE',  ( 97.64999999999997726, 88.47002178664753558, 85.18458333333332178 ) ) ;
#65748=VERTEX_POINT ( 'NONE', #30348 ) ;
#65752=ORIENTED_EDGE ( 'NONE', *, *, #60190, .F. ) ;
#65753=CARTESIAN_POINT ( 'NONE',  ( -92.69370383062505425, 88.66845928578038638, 86.25614583420048120 ) ) ;
#65754=CARTESIAN_POINT ( 'NONE',  ( 92.69370383062498320, 91.33154071421968467, 80.06489583420047040 ) ) ;
#65755=ORIENTED_EDGE ( 'NONE', *, *, #12961, .T. ) ;
#65757=CARTESIAN_POINT ( 'NONE',  ( 93.67499999999998295, 92.29496732002878900, 81.71854166840095957 ) ) ;
#65761=CARTESIAN_POINT ( 'NONE',  ( -93.67499999999998295, -212.2949673200287179, 86.40166666666667084 ) ) ;
#65764=VERTEX_POINT ( 'NONE', #13433 ) ;
#65769=CARTESIAN_POINT ( 'NONE',  ( -92.35000000000003695, 90.00000000000004263, 84.60249999999999204 ) ) ;
#65770=ADVANCED_FACE ( 'NONE', ( #71299, #60067, #59301, #42752, #65323 ), #54040, .F. ) ;
#65776=CARTESIAN_POINT ( 'NONE',  ( -93.84685191531248449, -208.0026889286704943, 80.54114583420046358 ) ) ;
#65793=CARTESIAN_POINT ( 'NONE',  ( -97.30629616937501680, 88.66845928578038638, 89.21947916753381946 ) ) ;
#65802=CARTESIAN_POINT ( 'NONE',  ( -94.99999999999997158, -213.0599564267049857, 84.52312500173428589 ) ) ;
#65805=CARTESIAN_POINT ( 'NONE',  ( 92.35000000000009379, -211.5299782133524502, 78.62291666666668277 ) ) ;
#65806=CARTESIAN_POINT ( 'NONE',  ( -2.499999999999965361, 90.00000000000000000, -310.0000000000000000 ) ) ;
#65807=CARTESIAN_POINT ( 'NONE',  ( -97.64999999999996305, -209.9999999999999716, 89.36499999999999488 ) ) ;
#65813=CARTESIAN_POINT ( 'NONE',  ( 92.35000000003358878, -210.0000076551254153, 78.01464417100928017 ) ) ;
#65816=VECTOR ( 'NONE', #53591, 1000.000000000000000 ) ;
#65824=CARTESIAN_POINT ( 'NONE',  ( 96.15314808468750130, -211.9973110713294489, 80.32947916753380468 ) ) ;
#65825=CARTESIAN_POINT ( 'NONE',  ( 97.30629616937498838, -211.3315407142195852, 88.16114583420048234 ) ) ;
#65827=CARTESIAN_POINT ( 'NONE',  ( 93.84685191531251292, -211.9973110713294489, 88.00239583420048461 ) ) ;
#65831=CARTESIAN_POINT ( 'NONE',  ( -92.69370383062502583, 91.33154071421968467, 78.74197916753382742 ) ) ;
#65845=VECTOR ( 'NONE', #46668, 1000.000000000000000 ) ;
#65851=CARTESIAN_POINT ( 'NONE',  ( 93.84685191531249870, -208.0026889286704943, 78.10697916753380809 ) ) ;
#65853=FACE_OUTER_BOUND ( 'NONE', #2434, .T. ) ;
#65854=ORIENTED_EDGE ( 'NONE', *, *, #34629, .T. ) ;
#65856=CARTESIAN_POINT ( 'NONE',  ( -96.32499999999996021, -212.2949673200287179, 78.75520833506763552 ) ) ;
#65860=CARTESIAN_POINT ( 'NONE',  ( -94.99999999999997158, -213.0599564267049857, 75.55375000000000796 ) ) ;
#65862=CARTESIAN_POINT ( 'NONE',  ( -97.64999999999996305, -209.9999999999999716, 88.80937500173430976 ) ) ;
#65865=CARTESIAN_POINT ( 'NONE',  ( -94.99999999999997158, -207.3369185715606307, 79.95906250086713385 ) ) ;
#65866=CARTESIAN_POINT ( 'NONE',  ( -92.69370383062502583, 91.33154071421968467, 77.47197916753381719 ) ) ;
#65868=CARTESIAN_POINT ( 'NONE',  ( 93.84685191531248449, 91.99731107132950569, 81.91697916753381037 ) ) ;
#65872=CARTESIAN_POINT ( 'NONE',  ( -92.69370383062498320, -211.3315407142195852, 88.00239583420047040 ) ) ;
#65874=CARTESIAN_POINT ( 'NONE',  ( -94.99999999999997158, -213.0599564267049857, 76.82374999999998977 ) ) ;
#65877=CARTESIAN_POINT ( 'NONE',  ( -96.15314808468747287, -208.0026889286704943, 82.55197916753380127 ) ) ;
#65889=CARTESIAN_POINT ( 'NONE',  ( -96.32500000000001705, 92.29496732002878900, 75.28916666666665947 ) ) ;
#65891=CARTESIAN_POINT ( 'NONE',  ( -92.69370383062504004, 90.00000000000004263, 84.88031250086713442 ) ) ;
#65894=DIRECTION ( 'NONE',  ( -1.000000000000000000, -0.000000000000000000, -0.000000000000000000 ) ) ;
#65895=ORIENTED_EDGE ( 'NONE', *, *, #18109, .F. ) ;
#65899=EDGE_CURVE ( 'NONE', #14594, #42482, #34975, .T. ) ;
#65907=CARTESIAN_POINT ( 'NONE',  ( -97.30629616937495996, -209.9999999999999716, 83.45156250086715488 ) ) ;
#65913=CARTESIAN_POINT ( 'NONE',  ( 94.99999999999998579, 87.33691857156068750, 75.35531250086715715 ) ) ;
#65915=CARTESIAN_POINT ( 'NONE',  ( -93.67500000000003979, 87.70503267997129626, 88.94166666666666288 ) ) ;
#65918=CARTESIAN_POINT ( 'NONE',  ( -97.65000000000009095, 91.52997821335249284, 78.51708333333334622 ) ) ;
#65920=CARTESIAN_POINT ( 'NONE',  ( 93.84685191531249870, -208.0026889286704943, 74.93197916753379673 ) ) ;
#65922=VECTOR ( 'NONE', #15448, 1000.000000000000000 ) ;
#65923=CARTESIAN_POINT ( 'NONE',  ( 97.64999999999999147, 90.00000000000002842, 87.22187500173430408 ) ) ;
#65925=( BOUNDED_CURVE ( )  B_SPLINE_CURVE ( 2, ( #38699, #34529, #28897, #57476, #5990, #17617, #7811 ),
 .UNSPECIFIED., .F., .F. ) 
 B_SPLINE_CURVE_WITH_KNOTS ( ( 3, 2, 2, 3 ),
 ( 0.3958333333333330373, 0.4027777777777774570, 0.4097222222222218768, 0.4166666666666662966 ),
 .UNSPECIFIED. ) 
 CURVE ( )  GEOMETRIC_REPRESENTATION_ITEM ( )  RATIONAL_B_SPLINE_CURVE ( ( 1.000000000000005329, 0.8660254037844333785, 1.000000000000000000, 0.8660254037844387076, 1.000000000000000000, 0.8660254037844462571, 0.9999999999999924505 ) ) 
 REPRESENTATION_ITEM ( '' )  );
#65937=DIRECTION ( 'NONE',  ( 1.000000000000000000, 0.000000000000000000, 0.000000000000000000 ) ) ;
#65940=CARTESIAN_POINT ( 'NONE',  ( 94.99999999999998579, 87.33691857156068750, 81.07031250086716057 ) ) ;
#65944=VECTOR ( 'NONE', #6060, 1000.000000000000000 ) ;
#65951=VECTOR ( 'NONE', #68356, 1000.000000000000000 ) ;
#65955=CARTESIAN_POINT ( 'NONE',  ( -96.44578755843129159, 91.96030971134661058, 74.86947676125078033 ) ) ;
#65958=CARTESIAN_POINT ( 'NONE',  ( -93.67500000000003979, 87.70503267997129626, 78.14666666666667538 ) ) ;
#65964=CARTESIAN_POINT ( 'NONE',  ( -97.64999999999994884, -208.4700217866474645, 76.69145833506763665 ) ) ;
#65965=CARTESIAN_POINT ( 'NONE',  ( -92.69370383062504004, 90.00000000000004263, 88.21406250086714351 ) ) ;
#65967=CARTESIAN_POINT ( 'NONE',  ( 92.34999999999999432, 88.47002178664753558, 76.16229166840095388 ) ) ;
#65968=CARTESIAN_POINT ( 'NONE',  ( -95.00000000000002842, 92.66308142843932671, 88.21406250086714351 ) ) ;
#65969=AXIS2_PLACEMENT_3D ( 'NONE', #20514, #14867, #54723 ) ;
#65971=CARTESIAN_POINT ( 'NONE',  ( 96.15314808468748708, 88.00268892867053694, 77.94822916753382458 ) ) ;
#65975=CARTESIAN_POINT ( 'NONE',  ( -92.35000000000003695, 90.00000000000004263, 78.33187500173430351 ) ) ;
#65978=CARTESIAN_POINT ( 'NONE',  ( -92.34999999999999432, -209.9999999999999716, 87.77749999999998920 ) ) ;
#65981=EDGE_LOOP ( 'NONE', ( #63086, #62070, #60651, #13402 ) ) ;
#65982=ADVANCED_FACE ( 'NONE', ( #57655 ), #16307, .F. ) ;
#65984=CARTESIAN_POINT ( 'NONE',  ( 93.67500000000001137, -207.7050326799711968, 82.90916666666666401 ) ) ;
#65985=CARTESIAN_POINT ( 'NONE',  ( 92.35000000001612364, -210.0000060634596082, 88.17456390440206349 ) ) ;
#65987=CARTESIAN_POINT ( 'NONE',  ( -95.00000000000002842, 86.94004357329504273, 76.26812500173430465 ) ) ;
#65988=CARTESIAN_POINT ( 'NONE',  ( -94.99999999999997158, -207.3369185715606307, 75.03781250086714749 ) ) ;
#65997=CARTESIAN_POINT ( 'NONE',  ( -96.32500000000001705, 92.29496732002878900, 79.09916666666666174 ) ) ;
#65998=CARTESIAN_POINT ( 'NONE',  ( 97.64999999999999147, 90.00000000000002842, 90.00000000000000000 ) ) ;
#66004=CARTESIAN_POINT ( 'NONE',  ( 97.30629616937498838, 88.66845928578035796, 83.08114583420048405 ) ) ;
#66005=CARTESIAN_POINT ( 'NONE',  ( -96.15314808468747287, -208.0026889286704943, 83.98072916753382344 ) ) ;
#66006=DIRECTION ( 'NONE',  ( -0.000000000000000000, -0.000000000000000000, 1.000000000000000000 ) ) ;
#66009=CARTESIAN_POINT ( 'NONE',  ( -97.64999999999994884, -211.5299782133524502, 78.62291666666668277 ) ) ;
#66015=CARTESIAN_POINT ( 'NONE',  ( 93.84685191531251292, -211.9973110713294489, 83.39864583420047950 ) ) ;
#66016=ORIENTED_EDGE ( 'NONE', *, *, #3433, .T. ) ;
#66017=CARTESIAN_POINT ( 'NONE',  ( 96.66135172262724495, 88.39919842643632819, 74.79754476654878204 ) ) ;
#66023=CARTESIAN_POINT ( 'NONE',  ( 95.00000000000000000, -212.6630814284392557, 79.16531250086715943 ) ) ;
#66027=CARTESIAN_POINT ( 'NONE',  ( -95.00000000000002842, 90.00000000000004263, 90.00000000000000000 ) ) ;
#66030=CARTESIAN_POINT ( 'NONE',  ( 95.00000000000000000, -206.9400435732949575, 80.31624999999998238 ) ) ;
#66040=CARTESIAN_POINT ( 'NONE',  ( -96.15314808468751551, 88.00268892867056536, 84.82739583420048746 ) ) ;
#66045=CARTESIAN_POINT ( 'NONE',  ( -92.34999999999999432, -210.0000000255707278, 84.04687500080852658 ) ) ;
#66048=CARTESIAN_POINT ( 'NONE',  ( -97.64999999999994884, -208.4700217866474645, 87.48645833506763836 ) ) ;
#66052=CARTESIAN_POINT ( 'NONE',  ( -93.67500000000003979, 87.70503267997129626, 87.75104166840095843 ) ) ;
#66055=CARTESIAN_POINT ( 'NONE',  ( 94.99999999999998579, 92.66308142843935514, 88.37281250086715545 ) ) ;
#66057=CARTESIAN_POINT ( 'NONE',  ( -95.00000000000002842, 86.94004357329504273, 85.79312500173431033 ) ) ;
#66060=DIRECTION ( 'NONE',  ( -0.000000000000000000, -0.000000000000000000, 1.000000000000000000 ) ) ;
#66069=ORIENTED_EDGE ( 'NONE', *, *, #26060, .F. ) ;
#66076=CARTESIAN_POINT ( 'NONE',  ( -92.34999999999999432, -209.9999999999999716, 83.33250000000001023 ) ) ;
#66077=CARTESIAN_POINT ( 'NONE',  ( -96.15314808468747287, -208.0026889286704943, 85.88572916753381037 ) ) ;
#66086=CARTESIAN_POINT ( 'NONE',  ( 93.84685191531248449, 91.99731107132950569, 79.37697916753380412 ) ) ;
#66087=LINE ( 'NONE', #55151, #53262 ) ;
#66088=CARTESIAN_POINT ( 'NONE',  ( 0.000000000000000000, 0.000000000000000000, -80.00000000000000000 ) ) ;
#66090=CARTESIAN_POINT ( 'NONE',  ( 93.86969025972511815, 92.14422361751726953, 74.86230178910948041 ) ) ;
#66094=VERTEX_POINT ( 'NONE', #24178 ) ;
#66095=VECTOR ( 'NONE', #9665, 1000.000000000000000 ) ;
#66096=CARTESIAN_POINT ( 'NONE',  ( -92.69370383062505425, 88.66845928578038638, 82.92239583420045790 ) ) ;
#66102=CARTESIAN_POINT ( 'NONE',  ( -97.64999999996706492, -209.9999916046304520, 84.99910573338409847 ) ) ;
#66108=CARTESIAN_POINT ( 'NONE',  ( 97.30629616937498838, -208.6684592857803011, 78.74197916753382742 ) ) ;
#66116=ORIENTED_EDGE ( 'NONE', *, *, #69780, .T. ) ;
#66118=CARTESIAN_POINT ( 'NONE',  ( 92.69370383062501162, -209.9999999999999716, 75.19656250086714522 ) ) ;
#66129=CARTESIAN_POINT ( 'NONE',  ( 93.67500000000001137, -212.2949673200287179, 79.39020833506762642 ) ) ;
#66130=CARTESIAN_POINT ( 'NONE',  ( 92.34999999999999432, 88.47002178664753558, 84.97291666666666288 ) ) ;
#66131=ORIENTED_EDGE ( 'NONE', *, *, #58726, .T. ) ;
#66136=CARTESIAN_POINT ( 'NONE',  ( -96.15314808468751551, 88.00268892867056536, 89.27239583420049485 ) ) ;
#66138=CARTESIAN_POINT ( 'NONE',  ( 92.69370383062498320, 90.00000000000002842, 80.75281250086715090 ) ) ;
#66140=CARTESIAN_POINT ( 'NONE',  ( 92.34999999999999432, 90.00000000000002842, 82.45937500173430124 ) ) ;
#66150=CARTESIAN_POINT ( 'NONE',  ( -93.67500000000003979, 92.29496732002878900, 84.07333333333333769 ) ) ;
#66152=ORIENTED_EDGE ( 'NONE', *, *, #23887, .T. ) ;
#66155=CARTESIAN_POINT ( 'NONE',  ( 97.64999999999997726, 88.47002178664753558, 88.43895833506762472 ) ) ;
#66157=( BOUNDED_CURVE ( )  B_SPLINE_CURVE ( 2, ( #40531, #44709, #6340, #62378, #39058, #67625, #69118 ),
 .UNSPECIFIED., .F., .F. ) 
 B_SPLINE_CURVE_WITH_KNOTS ( ( 3, 2, 2, 3 ),
 ( 0.6041666666666670737, 0.6111111111111116045, 0.6180555555555559133, 0.6250000000000003331 ),
 .UNSPECIFIED. ) 
 CURVE ( )  GEOMETRIC_REPRESENTATION_ITEM ( )  RATIONAL_B_SPLINE_CURVE ( ( 0.9999999999999914513, 0.8660254037844472563, 1.000000000000000000, 0.8660254037844387076, 1.000000000000000000, 0.8660254037844322683, 1.000000000000006439 ) ) 
 REPRESENTATION_ITEM ( '' )  );
#66158=DIRECTION ( 'NONE',  ( 1.000000000000000000, 0.000000000000000000, 0.000000000000000000 ) ) ;
#66159=CARTESIAN_POINT ( 'NONE',  ( -94.99999999999997158, -207.3369185715606307, 79.32406250086714294 ) ) ;
#66164=CYLINDRICAL_SURFACE ( 'NONE', #46557, 2.649999999999985700 ) ;
#66170=CARTESIAN_POINT ( 'NONE',  ( 93.84685191531248449, 88.00268892867053694, 87.20864583420046756 ) ) ;
#66171=CARTESIAN_POINT ( 'NONE',  ( 92.35000000006145626, -209.9999881787626919, 81.82400613091914465 ) ) ;
#66173=CARTESIAN_POINT ( 'NONE',  ( -97.64999999992174651, -209.9999869687493685, 79.28395951166956479 ) ) ;
#66174=CARTESIAN_POINT ( 'NONE',  ( -97.65000000000001990, 90.00000000000004263, 81.74500000000000455 ) ) ;
#66175=CARTESIAN_POINT ( 'NONE',  ( -96.15314808468752972, 91.99731107132950569, 74.93197916753379673 ) ) ;
#66178=CARTESIAN_POINT ( 'NONE',  ( 92.35000000000009379, -208.4700217866474361, 75.34208333333333485 ) ) ;
#66183=CARTESIAN_POINT ( 'NONE',  ( -94.99999999999997158, -213.0599564267049857, 87.61875000000000568 ) ) ;
#66188=CARTESIAN_POINT ( 'NONE',  ( 97.64998213368573943, -211.5299885284737513, 78.27895762153872283 ) ) ;
#66189=CARTESIAN_POINT ( 'NONE',  ( -95.00000000000002842, 93.05995642670504253, 84.76125000000000398 ) ) ;
#66192=AXIS2_PLACEMENT_3D ( 'NONE', #15653, #49847, #72764 ) ;
#66194=VERTEX_POINT ( 'NONE', #64770 ) ;
#66203=CARTESIAN_POINT ( 'NONE',  ( 92.69370383062501162, -211.3315407142195852, 80.17072916753380696 ) ) ;
#66204=CARTESIAN_POINT ( 'NONE',  ( 97.30629616937498838, -209.9999999999999716, 85.03906250086714635 ) ) ;
#66206=CARTESIAN_POINT ( 'NONE',  ( 97.30629616937498838, -211.3315407142195852, 85.62114583420047609 ) ) ;
#66212=CARTESIAN_POINT ( 'NONE',  ( -95.00000000000002842, 92.66308142843932671, 76.94281250086714863 ) ) ;
#66228=CARTESIAN_POINT ( 'NONE',  ( 95.00000000000000000, -212.6630814284392557, 79.64156250086713840 ) ) ;
#66238=CARTESIAN_POINT ( 'NONE',  ( -97.30629616937501680, 90.00000000000004263, 79.64156250086715261 ) ) ;
#66242=CARTESIAN_POINT ( 'NONE',  ( 92.69370383062498320, 90.00000000000002842, 76.94281250086713442 ) ) ;
#66244=FACE_OUTER_BOUND ( 'NONE', #18983, .T. ) ;
#66248=CARTESIAN_POINT ( 'NONE',  ( -92.69370383062498320, -209.9999999999999716, 84.24531250086714351 ) ) ;
#66254=ORIENTED_EDGE ( 'NONE', *, *, #15216, .T. ) ;
#66257=CARTESIAN_POINT ( 'NONE',  ( 23.49955575014745435, 0.001194404164629722436, -64.00000000000000000 ) ) ;
#66261=CARTESIAN_POINT ( 'NONE',  ( -92.69370383062502583, 91.33154071421968467, 86.83822916753381094 ) ) ;
#66266=DIRECTION ( 'NONE',  ( 0.4565542962317865050, 0.000000000000000000, 0.8896955516311735312 ) ) ;
#66275=CARTESIAN_POINT ( 'NONE',  ( -96.15314808468745866, -211.9973110713294489, 81.65239583420049030 ) ) ;
#66277=CARTESIAN_POINT ( 'NONE',  ( 92.34999999999999432, 90.00000000000002842, 76.10937500173430692 ) ) ;
#66290=VERTEX_POINT ( 'NONE', #49670 ) ;
#66293=DIRECTION ( 'NONE',  ( -1.000000000000000000, -0.000000000000000000, -0.000000000000000000 ) ) ;
#66295=EDGE_CURVE ( 'NONE', #14366, #64530, #25284, .T. ) ;
#66305=CARTESIAN_POINT ( 'NONE',  ( -2.500000000000020428, -90.00000000000000000, -310.0000000000000000 ) ) ;
#66311=CARTESIAN_POINT ( 'NONE',  ( 97.30629616937498838, 88.66845928578037217, 78.00114583420049996 ) ) ;
#66314=CARTESIAN_POINT ( 'NONE',  ( -92.35000000000005116, 91.52997821335253548, 87.90979166840097037 ) ) ;
#66317=EDGE_LOOP ( 'NONE', ( #62420, #54653, #57648, #70188 ) ) ;
#66318=CARTESIAN_POINT ( 'NONE',  ( 97.30629616937498838, 91.33154071421968467, 89.37822916753381719 ) ) ;
#66322=CARTESIAN_POINT ( 'NONE',  ( 97.64999999999999147, -209.9999999999999716, 74.52187500173430124 ) ) ;
#66323=VECTOR ( 'NONE', #41172, 1000.000000000000000 ) ;
#66328=LINE ( 'NONE', #43020, #7835 ) ;
#66331=CARTESIAN_POINT ( 'NONE',  ( -96.32499999999996021, -207.7050326799711968, 76.00354166840097037 ) ) ;
#66336=CARTESIAN_POINT ( 'NONE',  ( 96.15314808468748708, 91.99731107132950569, 86.25614583420048120 ) ) ;
#66337=CARTESIAN_POINT ( 'NONE',  ( -92.69370383062502583, 88.66845928578038638, 89.27239583420048064 ) ) ;
#66338=VERTEX_POINT ( 'NONE', #14363 ) ;
#66339=CARTESIAN_POINT ( 'NONE',  ( 92.69370383062498320, 88.66845928578037217, 75.24947916753383481 ) ) ;
#66346=CARTESIAN_POINT ( 'NONE',  ( -93.67499999999998295, -212.2949673200287179, 87.67166666666666686 ) ) ;
#66355=CARTESIAN_POINT ( 'NONE',  ( -96.15314808468745866, -211.9973110713294489, 75.93739583420048689 ) ) ;
#66356=VERTEX_POINT ( 'NONE', #60611 ) ;
#66357=CARTESIAN_POINT ( 'NONE',  ( -93.84685191531254134, 91.99731107132950569, 81.17614583420048291 ) ) ;
#66367=DIRECTION ( 'NONE',  ( -0.000000000000000000, -0.000000000000000000, 1.000000000000000000 ) ) ;
#66369=( BOUNDED_CURVE ( )  B_SPLINE_CURVE ( 2, ( #51103, #5638, #6010, #21787, #28536, #29, #28914 ),
 .UNSPECIFIED., .F., .F. ) 
 B_SPLINE_CURVE_WITH_KNOTS ( ( 3, 2, 2, 3 ),
 ( 0.8333333333333334814, 0.8402777777777779011, 0.8472222222222222099, 0.8541666666666666297 ),
 .UNSPECIFIED. ) 
 CURVE ( )  GEOMETRIC_REPRESENTATION_ITEM ( )  RATIONAL_B_SPLINE_CURVE ( ( 0.9999999999999978906, 0.8660254037844408170, 1.000000000000000000, 0.8660254037844387076, 1.000000000000000000, 0.8660254037844387076, 1.000000000000000000 ) ) 
 REPRESENTATION_ITEM ( '' )  );
#66370=CARTESIAN_POINT ( 'NONE',  ( 96.15314808468748708, 88.00268892867053694, 81.75822916753382685 ) ) ;
#66371=CARTESIAN_POINT ( 'NONE',  ( -92.69370383062498320, -208.6684592857803295, 82.55197916753380127 ) ) ;
#66372=DIRECTION ( 'NONE',  ( 1.000000000000000000, 0.000000000000000000, 0.000000000000000000 ) ) ;
#66375=CARTESIAN_POINT ( 'NONE',  ( -92.34999999999999432, -208.4700217866474645, 77.03541666666666288 ) ) ;
#66377=DIRECTION ( 'NONE',  ( -0.000000000000000000, -0.000000000000000000, 1.000000000000000000 ) ) ;
#66383=CARTESIAN_POINT ( 'NONE',  ( 96.15314808468750130, -211.9973110713294489, 82.86947916753379673 ) ) ;
#66393=CARTESIAN_POINT ( 'NONE',  ( 97.30629616937498838, -209.9999999999999716, 79.95906250086714806 ) ) ;
#66396=CARTESIAN_POINT ( 'NONE',  ( -97.44941226940133561, 89.32071446497062084, 74.93153462041256319 ) ) ;
#66397=CARTESIAN_POINT ( 'NONE',  ( 96.15314808468748708, 91.99731107132950569, 85.77989583420048803 ) ) ;
#66398=CARTESIAN_POINT ( 'NONE',  ( -92.35000000000003695, 90.00001154861327279, 83.41187540116096955 ) ) ;
#66399=CARTESIAN_POINT ( 'NONE',  ( 97.64999999999999147, -209.9999999999999716, 80.79249999999998977 ) ) ;
#66400=ORIENTED_EDGE ( 'NONE', *, *, #35957, .T. ) ;
#66403=ORIENTED_EDGE ( 'NONE', *, *, #6000, .F. ) ;
#66405=CARTESIAN_POINT ( 'NONE',  ( 97.65000000000000568, -211.5299782133523934, 87.08958333333333712 ) ) ;
#66409=CARTESIAN_POINT ( 'NONE',  ( -96.15314808468751551, 88.00268892867056536, 83.55739583420049144 ) ) ;
#66415=CARTESIAN_POINT ( 'NONE',  ( -93.67499999999998295, -212.2949673200287179, 86.48104166840096241 ) ) ;
#66419=CARTESIAN_POINT ( 'NONE',  ( -93.67500000000003979, 87.70503267997129626, 83.94104166840097037 ) ) ;
#66421=VERTEX_POINT ( 'NONE', #62473 ) ;
#66422=CARTESIAN_POINT ( 'NONE',  ( 92.69370383062498320, 91.33154071421968467, 87.20864583420049598 ) ) ;
#66424=CARTESIAN_POINT ( 'NONE',  ( 2.500000000000034639, 90.00000000000000000, -310.0000000000000000 ) ) ;
#66430=DIRECTION ( 'NONE',  ( -0.000000000000000000, -0.000000000000000000, 1.000000000000000000 ) ) ;
#66434=DIRECTION ( 'NONE',  ( 1.000000000000000000, 0.000000000000000000, 0.000000000000000000 ) ) ;
#66435=LINE ( 'NONE', #25462, #18009 ) ;
#66437=CARTESIAN_POINT ( 'NONE',  ( -97.30629616937495996, -209.9999999999999716, 85.99156250086716113 ) ) ;
#66439=FACE_OUTER_BOUND ( 'NONE', #70557, .T. ) ;
#66443=CARTESIAN_POINT ( 'NONE',  ( 93.67500000000001137, -207.7050326799711968, 82.98854166840096980 ) ) ;
#66444=CARTESIAN_POINT ( 'NONE',  ( 97.30629616937498838, 88.66845928578035796, 77.84239583420047381 ) ) ;
#66454=CARTESIAN_POINT ( 'NONE',  ( 96.32499999999998863, 87.70503267997126784, 76.95604166840095672 ) ) ;
#66456=CARTESIAN_POINT ( 'NONE',  ( -96.15314808468752972, 91.99731107132950569, 83.18697916753382060 ) ) ;
#66460=ADVANCED_FACE ( 'NONE', ( #10953 ), #68094, .F. ) ;
#66470=CARTESIAN_POINT ( 'NONE',  ( 93.67499999999999716, 87.70503267997126784, 83.20020833506764291 ) ) ;
#66472=CARTESIAN_POINT ( 'NONE',  ( 97.30629616937498838, -211.3315407142195852, 78.00114583420049996 ) ) ;
#66481=CARTESIAN_POINT ( 'NONE',  ( 97.30629616937498838, -210.9303121318039871, 74.84209103131395580 ) ) ;
#66494=CARTESIAN_POINT ( 'NONE',  ( 97.64999999999997726, -208.4700217866474645, 79.01979166840095559 ) ) ;
#66495=CARTESIAN_POINT ( 'NONE',  ( 96.32499999999998863, 87.70503267997126784, 86.40166666666667084 ) ) ;
#66498=CARTESIAN_POINT ( 'NONE',  ( 96.32499999999997442, 92.29496732002878900, 80.97770833506763211 ) ) ;
#66502=CARTESIAN_POINT ( 'NONE',  ( -95.00000000000002842, 92.66308142843932671, 85.83281250086717762 ) ) ;
#66503=CARTESIAN_POINT ( 'NONE',  ( 94.99999999999998579, 92.66308142843935514, 82.49906250086714010 ) ) ;
#66510=CIRCLE ( 'NONE', #40109, 15.70000000000000284 ) ;
#66517=CARTESIAN_POINT ( 'NONE',  ( 92.34999999999999432, 91.52997821335252127, 88.75645833506762017 ) ) ;
#66519=CYLINDRICAL_SURFACE ( 'NONE', #38380, 2.649999999999985700 ) ;
#66520=CARTESIAN_POINT ( 'NONE',  ( -92.69370383062498320, -211.3315407142195852, 81.01739583420048518 ) ) ;
#66531=CARTESIAN_POINT ( 'NONE',  ( 97.30629616937498838, 88.66845928578035796, 88.00239583420047040 ) ) ;
#66535=CARTESIAN_POINT ( 'NONE',  ( 96.37670920697048871, -212.2908000246596316, 75.00000000000000000 ) ) ;
#66549=CARTESIAN_POINT ( 'NONE',  ( -92.34999999999999432, -211.5299782133524502, 88.35958333333333314 ) ) ;
#66555=CARTESIAN_POINT ( 'NONE',  ( 97.64999999999449187, -210.0000054026048701, 81.50687481489494246 ) ) ;
#66564=ORIENTED_EDGE ( 'NONE', *, *, #47311, .T. ) ;
#66566=CARTESIAN_POINT ( 'NONE',  ( 92.69370383062501162, -209.9999999999999716, 80.75281250086715090 ) ) ;
#66567=CARTESIAN_POINT ( 'NONE',  ( 96.15314808468750130, -211.9973110713294489, 83.66322916753382799 ) ) ;
#66568=AXIS2_PLACEMENT_3D ( 'NONE', #31678, #48245, #32040 ) ;
#66570=CARTESIAN_POINT ( 'NONE',  ( 97.30629616937498838, -209.9999999999999716, 87.57906250086715261 ) ) ;
#66575=CARTESIAN_POINT ( 'NONE',  ( -95.00000000000002842, 87.33691857156074434, 77.89531250086714920 ) ) ;
#66578=CYLINDRICAL_SURFACE ( 'NONE', #25670, 2.649999999999985700 ) ;
#66580=EDGE_LOOP ( 'NONE', ( #69537, #1178, #475, #74149 ) ) ;
#66587=( BOUNDED_CURVE ( )  B_SPLINE_CURVE ( 2, ( #8095, #25013, #47217, #47955, #18995, #41949, #2863, #64887, #65622 ),
 .UNSPECIFIED., .F., .F. ) 
 B_SPLINE_CURVE_WITH_KNOTS ( ( 3, 2, 2, 2, 3 ),
 ( 0.7620226289501886852, 0.7620226784190389235, 0.7690784439599557265, 0.7761342095008724185, 0.7831899741104385582 ),
 .UNSPECIFIED. ) 
 CURVE ( )  GEOMETRIC_REPRESENTATION_ITEM ( )  RATIONAL_B_SPLINE_CURVE ( ( 0.9999981213880371200, 0.9999990606874329391, 1.000000000000000000, 0.8660254037844387076, 1.000000000000000000, 0.8660254037844387076, 1.000000000000000000, 0.8660254037844387076, 1.000000000000000000 ) ) 
 REPRESENTATION_ITEM ( '' )  );
#66588=CARTESIAN_POINT ( 'NONE',  ( 96.32499999999998863, -212.2949673200287179, 81.40104166840096411 ) ) ;
#66592=CARTESIAN_POINT ( 'NONE',  ( 96.66078690017491226, -211.6002465100980032, 74.64190636928354650 ) ) ;
#66599=CARTESIAN_POINT ( 'NONE',  ( -97.30629616937501680, 88.66845928578038638, 80.32947916753381890 ) ) ;
#66602=CARTESIAN_POINT ( 'NONE',  ( 94.99999999999998579, 92.66308142843935514, 78.05406250086714692 ) ) ;
#66605=CARTESIAN_POINT ( 'NONE',  ( -92.69370383062498320, -209.9999999999999716, 89.32531250086714181 ) ) ;
#66609=CARTESIAN_POINT ( 'NONE',  ( -96.15314808468747287, -208.0026889286704943, 80.64697916753381435 ) ) ;
#66621=CARTESIAN_POINT ( 'NONE',  ( -95.00000000000002842, 87.33691857156074434, 85.35656250086714181 ) ) ;
#66634=FACE_OUTER_BOUND ( 'NONE', #54314, .T. ) ;
#66635=CARTESIAN_POINT ( 'NONE',  ( -97.64999999954994792, 89.99996890530464100, 88.81037122970319331 ) ) ;
#66636=CARTESIAN_POINT ( 'NONE',  ( -96.15314808468745866, -211.9973110713294489, 82.28739583420048120 ) ) ;
#66637=CARTESIAN_POINT ( 'NONE',  ( -97.64999999999996305, -209.9999999999999716, 86.90437500173429441 ) ) ;
#66646=CARTESIAN_POINT ( 'NONE',  ( 97.64999999999999147, -209.9999999999999716, 79.52249999999999375 ) ) ;
#66651=CARTESIAN_POINT ( 'NONE',  ( 96.32499999999997442, 92.29496732002878900, 78.35833333333333428 ) ) ;
#66667=VERTEX_POINT ( 'NONE', #1929 ) ;
#66668=CARTESIAN_POINT ( 'NONE',  ( 96.15314808468748708, 91.99731107132950569, 76.88989583420048746 ) ) ;
#66676=CARTESIAN_POINT ( 'NONE',  ( 97.30629616937498838, 91.33154071421968467, 86.83822916753381094 ) ) ;
#66677=ORIENTED_EDGE ( 'NONE', *, *, #49611, .T. ) ;
#66678=AXIS2_PLACEMENT_3D ( 'NONE', #21314, #4430, #20956 ) ;
#66679=CARTESIAN_POINT ( 'NONE',  ( 92.35000000000002274, -208.4700217866474645, 74.78645833506763552 ) ) ;
#66687=DIRECTION ( 'NONE',  ( 1.000000000000000000, 0.000000000000000000, 0.000000000000000000 ) ) ;
#66688=CARTESIAN_POINT ( 'NONE',  ( -94.99999999999997158, -206.9400435732949575, 75.31562500173430408 ) ) ;
#66689=CARTESIAN_POINT ( 'NONE',  ( -97.30629616937501680, 90.00000000000004263, 87.89656250086714806 ) ) ;
#66690=VERTEX_POINT ( 'NONE', #46643 ) ;
#66691=CARTESIAN_POINT ( 'NONE',  ( 97.30629616937498838, 88.66845928578037217, 87.36739583420047950 ) ) ;
#66692=CARTESIAN_POINT ( 'NONE',  ( -93.84685191531252713, 88.00268892867056536, 86.67947916753381321 ) ) ;
#66694=CARTESIAN_POINT ( 'NONE',  ( 97.64999999999999147, -210.0000001167898631, 84.68187499741277691 ) ) ;
#66695=CARTESIAN_POINT ( 'NONE',  ( 92.34999999999999432, 90.00000000000002842, 82.37999999999999545 ) ) ;
#66697=CARTESIAN_POINT ( 'NONE',  ( 93.67499999999998295, 92.29496732002878900, 82.35354166840096468 ) ) ;
#66708=CARTESIAN_POINT ( 'NONE',  ( -97.65000000000001990, 88.47002178664754979, 79.89291666666666458 ) ) ;
#66711=CARTESIAN_POINT ( 'NONE',  ( 95.00000000000000000, -206.9400435732949575, 75.87125000000000341 ) ) ;
#66712=CARTESIAN_POINT ( 'NONE',  ( 95.00000000000000000, -206.9400435732949575, 88.01562500173432113 ) ) ;
#66713=CARTESIAN_POINT ( 'NONE',  ( -100.0000000000000142, 95.00000000000002842, 90.00000000000000000 ) ) ;
#66715=CARTESIAN_POINT ( 'NONE',  ( 92.35000000000002274, 88.47002178664752137, 84.33791666666667197 ) ) ;
#66717=CARTESIAN_POINT ( 'NONE',  ( -95.00000000000002842, 92.66308142843932671, 83.13406250086714522 ) ) ;
#66725=CARTESIAN_POINT ( 'NONE',  ( -97.65000000000001990, 90.00000000000004263, 90.00000000000000000 ) ) ;
#66729=CARTESIAN_POINT ( 'NONE',  ( 96.15314808468748708, 88.00268892867053694, 81.12322916753382174 ) ) ;
#66731=CARTESIAN_POINT ( 'NONE',  ( -97.30629616937497417, -211.3315407142195852, 82.23447916753383424 ) ) ;
#66735=CARTESIAN_POINT ( 'NONE',  ( -97.64999999999996305, -209.9999999999999716, 78.57000000000000739 ) ) ;
#66736=DIRECTION ( 'NONE',  ( 1.000000000000000000, 0.000000000000000000, 0.000000000000000000 ) ) ;
#66741=CARTESIAN_POINT ( 'NONE',  ( -97.30629616937501680, 91.33154071421968467, 78.31864583420050963 ) ) ;
#66742=CARTESIAN_POINT ( 'NONE',  ( 97.30629616937498838, -208.6684592857803011, 83.66322916753379957 ) ) ;
#66752=CARTESIAN_POINT ( 'NONE',  ( 97.30629616937498838, -208.6684592857803295, 78.74197916753381321 ) ) ;
#66756=CARTESIAN_POINT ( 'NONE',  ( 92.69370383062498320, 88.66845928578037217, 85.40947916753380298 ) ) ;
#66757=CARTESIAN_POINT ( 'NONE',  ( 95.73180504966225612, 87.36255141571184879, 75.02735117824596500 ) ) ;
#66758=CARTESIAN_POINT ( 'NONE',  ( 93.67500000000001137, -212.2949673200287179, 81.85083333333332689 ) ) ;
#66759=ORIENTED_EDGE ( 'NONE', *, *, #54841, .T. ) ;
#66764=CARTESIAN_POINT ( 'NONE',  ( -97.64999999999996305, -209.9999999999999716, 85.55499999999999261 ) ) ;
#66770=CARTESIAN_POINT ( 'NONE',  ( -93.67499999999998295, -207.7050326799711968, 86.69270833506763552 ) ) ;
#66774=CARTESIAN_POINT ( 'NONE',  ( -97.65000000000001990, 88.47002178664754979, 83.78229166840095843 ) ) ;
#66776=CARTESIAN_POINT ( 'NONE',  ( 94.99999999999998579, 87.33691857156068750, 82.34031250086714238 ) ) ;
#66780=EDGE_CURVE ( 'NONE', #64543, #24878, #306, .T. ) ;
#66797=CARTESIAN_POINT ( 'NONE',  ( -94.99999999999997158, -213.0599564267049857, 83.17374999999999829 ) ) ;
#66799=( BOUNDED_CURVE ( )  B_SPLINE_CURVE ( 2, ( #72731, #4727, #44186, #11446, #34379, #3980, #55833 ),
 .UNSPECIFIED., .F., .F. ) 
 B_SPLINE_CURVE_WITH_KNOTS ( ( 3, 2, 2, 3 ),
 ( 0.4166666666666662966, 0.4236111111111106609, 0.4305555555555550806, 0.4374999999999994449 ),
 .UNSPECIFIED. ) 
 CURVE ( )  GEOMETRIC_REPRESENTATION_ITEM ( )  RATIONAL_B_SPLINE_CURVE ( ( 1.000000000000007550, 0.8660254037844311581, 1.000000000000000000, 0.8660254037844387076, 1.000000000000000000, 0.8660254037844493658, 0.9999999999999893419 ) ) 
 REPRESENTATION_ITEM ( '' )  );
#66800=CARTESIAN_POINT ( 'NONE',  ( -94.99999999999997158, -212.6630814284392557, 83.61031250086716682 ) ) ;
#66809=CARTESIAN_POINT ( 'NONE',  ( 94.99999999999998579, 92.66308142843932671, 78.05406250086714692 ) ) ;
#66811=CARTESIAN_POINT ( 'NONE',  ( 97.64999999999999147, 89.99999989488613039, 86.58687499784845443 ) ) ;
#66813=CARTESIAN_POINT ( 'NONE',  ( 94.21072067537627959, 92.27861417635780583, 74.85481846778738202 ) ) ;
#66816=CARTESIAN_POINT ( 'NONE',  ( -92.69370383062498320, -210.0000000000000568, 74.79348190356851944 ) ) ;
#66820=CARTESIAN_POINT ( 'NONE',  ( -97.30629616937501680, 88.66845928578038638, 84.61572916753380014 ) ) ;
#66827=CARTESIAN_POINT ( 'NONE',  ( 95.00000000000000000, -209.9999999999999716, 75.00000000000000000 ) ) ;
#66832=DIRECTION ( 'NONE',  ( 1.000000000000000000, 0.000000000000000000, 0.000000000000000000 ) ) ;
#66833=CARTESIAN_POINT ( 'NONE',  ( 96.15314808468748708, -208.0026889286704943, 78.15989583420049769 ) ) ;
#66840=DIRECTION ( 'NONE',  ( -1.000000000000000000, -0.000000000000000000, -0.000000000000000000 ) ) ;
#66844=CARTESIAN_POINT ( 'NONE',  ( 96.15314808468748708, -208.0026889286704943, 77.52489583420047836 ) ) ;
#66847=ORIENTED_EDGE ( 'NONE', *, *, #8676, .F. ) ;
#66853=CARTESIAN_POINT ( 'NONE',  ( 93.67500000000001137, -207.7050326799711968, 79.81354166840095843 ) ) ;
#66854=CARTESIAN_POINT ( 'NONE',  ( 96.32499999999998863, 87.70503267997126784, 84.49666666666666970 ) ) ;
#66858=CARTESIAN_POINT ( 'NONE',  ( -92.91683521821995839, -211.0005890871206589, 74.79348190356851944 ) ) ;
#66860=CARTESIAN_POINT ( 'NONE',  ( 93.67499999999998295, 92.29496732002878900, 84.25854166840096582 ) ) ;
#66861=CARTESIAN_POINT ( 'NONE',  ( -97.30629616937501680, 88.66845928578038638, 83.50447916753383026 ) ) ;
#66862=CARTESIAN_POINT ( 'NONE',  ( 93.84685191531248449, 88.00268892867053694, 81.49364583420047836 ) ) ;
#66870=CARTESIAN_POINT ( 'NONE',  ( 93.67499999999999716, 87.70503267997126784, 79.94583333333332575 ) ) ;
#66874=CARTESIAN_POINT ( 'NONE',  ( 94.99999999999998579, 93.05995642670504253, 88.01562500173429271 ) ) ;
#66876=DIRECTION ( 'NONE',  ( 1.000000000000000000, 0.000000000000000000, 0.000000000000000000 ) ) ;
#66877=CARTESIAN_POINT ( 'NONE',  ( -93.84685191531247028, -211.9973110713294489, 80.32947916753380468 ) ) ;
#66884=CARTESIAN_POINT ( 'NONE',  ( 95.00000000000000000, -209.9999999999999716, 90.00000000000000000 ) ) ;
#66888=CARTESIAN_POINT ( 'NONE',  ( 97.30629616937498838, 88.66845928578035796, 86.73239583420047438 ) ) ;
#66899=CARTESIAN_POINT ( 'NONE',  ( 97.65000000000006253, -208.4700217866474929, 75.13041666666666174 ) ) ;
#66900=DIRECTION ( 'NONE',  ( 1.000000000000000000, 0.000000000000000000, 0.000000000000000000 ) ) ;
#66902=EDGE_CURVE ( 'NONE', #1787, #45691, #72394, .T. ) ;
#66906=CARTESIAN_POINT ( 'NONE',  ( -97.64999999999994884, -208.4700217866474645, 84.23208333333333542 ) ) ;
#66907=LINE ( 'NONE', #72895, #54879 ) ;
#66914=DIRECTION ( 'NONE',  ( 0.000000000000000000, 0.000000000000000000, 1.000000000000000000 ) ) ;
#66917=CARTESIAN_POINT ( 'NONE',  ( 97.30629616937498838, -211.3315407142195852, 82.28739583420048120 ) ) ;
#66918=CARTESIAN_POINT ( 'NONE',  ( 93.84685191531251292, -211.9973110713294489, 83.55739583420049144 ) ) ;
#66921=CARTESIAN_POINT ( 'NONE',  ( 95.00000000000000000, -207.3369185715606307, 87.73781250086715033 ) ) ;
#66926=CARTESIAN_POINT ( 'NONE',  ( -95.00000000000002842, 92.66308142843932671, 76.30781250086715772 ) ) ;
#66944=CARTESIAN_POINT ( 'NONE',  ( 97.30629616937498838, -211.3315407142195852, 75.30239583420048177 ) ) ;
#66955=CARTESIAN_POINT ( 'NONE',  ( -93.84685191531254134, 91.99731107132950569, 74.98489583420048632 ) ) ;
#66957=CARTESIAN_POINT ( 'NONE',  ( 96.15314808468748708, 88.00268892867053694, 77.78947916753381264 ) ) ;
#66966=CARTESIAN_POINT ( 'NONE',  ( -93.84685191531247028, -211.9973110713294489, 80.32947916753380468 ) ) ;
#66968=CARTESIAN_POINT ( 'NONE',  ( -2.499999999999965361, 90.00000000000000000, -90.00000000000000000 ) ) ;
#66971=VERTEX_POINT ( 'NONE', #61627 ) ;
#66972=DIRECTION ( 'NONE',  ( -1.000000000000000000, -1.343011723336883198E-16, -0.000000000000000000 ) ) ;
#66975=CARTESIAN_POINT ( 'NONE',  ( 95.29776683160980610, -207.6384304500494409, 74.83035915144985495 ) ) ;
#66977=CARTESIAN_POINT ( 'NONE',  ( -97.30629616937501680, 90.00000000000004263, 80.75281250086715090 ) ) ;
#66981=ORIENTED_EDGE ( 'NONE', *, *, #15067, .T. ) ;
#66988=DIRECTION ( 'NONE',  ( 1.343011723336883198E-16, -1.000000000000000000, 0.000000000000000000 ) ) ;
#66990=CARTESIAN_POINT ( 'NONE',  ( -92.69370383062498320, -209.9999999999999716, 81.86406250086714920 ) ) ;
#67000=AXIS2_PLACEMENT_3D ( 'NONE', #26525, #54733, #43481 ) ;
#67009=( BOUNDED_CURVE ( )  B_SPLINE_CURVE ( 2, ( #72988, #55718, #4235, #9115, #27129, #50059, #60636, #43716, #66637, #9480, #32404 ),
 .UNSPECIFIED., .F., .F. ) 
 B_SPLINE_CURVE_WITH_KNOTS ( ( 3, 2, 2, 2, 2, 3 ),
 ( 0.1481709449582802873, 0.1481710763592573865, 0.1552268419001741062, 0.1622826074410907982, 0.1693383729820075179, 0.1693384224428226559 ),
 .UNSPECIFIED. ) 
 CURVE ( )  GEOMETRIC_REPRESENTATION_ITEM ( )  RATIONAL_B_SPLINE_CURVE ( ( 0.9999950100198486957, 0.9999975049634587387, 1.000000000000000000, 0.8660254037844387076, 1.000000000000000000, 0.8660254037844387076, 1.000000000000000000, 0.8660254037844387076, 1.000000000000000000, 0.9999990608400038949, 0.9999981216931748129 ) ) 
 REPRESENTATION_ITEM ( '' )  );
#67024=ORIENTED_EDGE ( 'NONE', *, *, #55840, .T. ) ;
#67025=CARTESIAN_POINT ( 'NONE',  ( 97.30629616937498838, 90.00000000000002842, 78.05406250086716113 ) ) ;
#67026=DIRECTION ( 'NONE',  ( 1.000000000000000000, 0.000000000000000000, 0.000000000000000000 ) ) ;
#67035=CARTESIAN_POINT ( 'NONE',  ( 93.84685191531248449, 91.99731107132950569, 87.63197916753379957 ) ) ;
#67037=CARTESIAN_POINT ( 'NONE',  ( 92.69370383062501162, -211.3315407142195852, 84.61572916753380014 ) ) ;
#67041=FACE_OUTER_BOUND ( 'NONE', #68313, .T. ) ;
#67042=CARTESIAN_POINT ( 'NONE',  ( -92.35000000000006537, 90.00000034979574082, 77.69687501385438111 ) ) ;
#67047=CARTESIAN_POINT ( 'NONE',  ( -96.15314808468747287, -208.0026889286704943, 87.63197916753379957 ) ) ;
#67048=CARTESIAN_POINT ( 'NONE',  ( -92.69370383062502583, 91.33154071421968467, 84.45697916753383083 ) ) ;
#67050=CARTESIAN_POINT ( 'NONE',  ( 92.69370383062498320, 91.33154071421968467, 87.68489583420047495 ) ) ;
#67051=CARTESIAN_POINT ( 'NONE',  ( -93.84685191531252713, 88.00268892867056536, 87.31447916753380412 ) ) ;
#67054=EDGE_CURVE ( 'NONE', #5282, #14250, #43956, .T. ) ;
#67068=CARTESIAN_POINT ( 'NONE',  ( -97.65000000000001990, 88.47002178664754979, 81.79791666666666572 ) ) ;
#67072=CARTESIAN_POINT ( 'NONE',  ( 92.35000000005783249, -210.0000112241611703, 75.47473230081648410 ) ) ;
#67074=CARTESIAN_POINT ( 'NONE',  ( 97.64999999999999147, -209.9999999999999716, 76.98250000000000171 ) ) ;
#67080=CARTESIAN_POINT ( 'NONE',  ( -92.69370383062504004, 90.00000000000004263, 80.43531250086714124 ) ) ;
#67090=CARTESIAN_POINT ( 'NONE',  ( 92.69370383062498320, 91.33154071421968467, 80.22364583420048234 ) ) ;
#67093=CARTESIAN_POINT ( 'NONE',  ( -92.69370383062498320, -209.9999999999999716, 83.76906250086716454 ) ) ;
#67094=CARTESIAN_POINT ( 'NONE',  ( 97.64999999999990621, 90.00000071509185773, 85.31687502647973531 ) ) ;
#67097=CARTESIAN_POINT ( 'NONE',  ( -92.34999999999999432, -209.9999999999999716, 78.88750000000000284 ) ) ;
#67098=FACE_OUTER_BOUND ( 'NONE', #24067, .T. ) ;
#67101=CARTESIAN_POINT ( 'NONE',  ( -95.00000000000002842, 92.66308142843932671, 77.57781250086715374 ) ) ;
#67102=CARTESIAN_POINT ( 'NONE',  ( 93.84685191531249870, -208.0026889286704943, 84.45697916753380241 ) ) ;
#67103=ORIENTED_EDGE ( 'NONE', *, *, #18608, .T. ) ;
#67104=CARTESIAN_POINT ( 'NONE',  ( -95.00000000000002842, 90.00000000000004263, 90.00000000000000000 ) ) ;
#67117=CARTESIAN_POINT ( 'NONE',  ( 95.00000000000000000, -212.6630814284392557, 75.99031250086716227 ) ) ;
#67122=CARTESIAN_POINT ( 'NONE',  ( 97.30629616937498838, 90.00000000000002842, 86.94406250086716170 ) ) ;
#67123=CARTESIAN_POINT ( 'NONE',  ( 92.34999999999999432, 90.00001557635631855, 80.55437446300187787 ) ) ;
#67124=CARTESIAN_POINT ( 'NONE',  ( 95.00000000000000000, -206.9400435732949575, 77.14124999999999943 ) ) ;
#67133=CARTESIAN_POINT ( 'NONE',  ( -97.64999999993855795, 90.00001182123732235, 81.82400613091868991 ) ) ;
#67140=CARTESIAN_POINT ( 'NONE',  ( -96.32499999999996021, -212.2949673200287179, 85.10520833506762983 ) ) ;
#67141=ORIENTED_EDGE ( 'NONE', *, *, #46529, .T. ) ;
#67144=CARTESIAN_POINT ( 'NONE',  ( -97.65000000000001990, 90.00000000000004263, 83.09437500173430635 ) ) ;
#67147=CARTESIAN_POINT ( 'NONE',  ( 97.30629616937498838, 91.33154071421968467, 81.91697916753381037 ) ) ;
#67149=CARTESIAN_POINT ( 'NONE',  ( -97.64999999999994884, 88.47002178664749295, 76.08291666666664810 ) ) ;
#67150=AXIS2_PLACEMENT_3D ( 'NONE', #43385, #60301, #53905 ) ;
#67166=CARTESIAN_POINT ( 'NONE',  ( -97.65000000000001990, 88.47002178664754979, 79.97229166840095615 ) ) ;
#67168=CARTESIAN_POINT ( 'NONE',  ( -92.69370383062498320, -211.3315407142195852, 79.90614583420048689 ) ) ;
#67171=VERTEX_POINT ( 'NONE', #47658 ) ;
#67172=VECTOR ( 'NONE', #35701, 1000.000000000000000 ) ;
#67177=CARTESIAN_POINT ( 'NONE',  ( -92.35000000000395914, -210.0000045800647115, 76.42687486209126746 ) ) ;
#67178=CARTESIAN_POINT ( 'NONE',  ( 97.30629616937498838, 90.00000000000002842, 77.89531250086714920 ) ) ;
#67183=CARTESIAN_POINT ( 'NONE',  ( 96.73972734126401463, 91.51405112163766375, 74.79348190356853365 ) ) ;
#67189=CARTESIAN_POINT ( 'NONE',  ( -92.35000000018069954, 89.99996905681452120, 78.33187387208522523 ) ) ;
#67191=CARTESIAN_POINT ( 'NONE',  ( -96.15314808468752972, 91.99731107132950569, 84.45697916753380241 ) ) ;
#67198=CARTESIAN_POINT ( 'NONE',  ( -95.00000000000002842, 90.00000000000004263, 75.00000000000000000 ) ) ;
#67202=CARTESIAN_POINT ( 'NONE',  ( -92.34999999999999432, -209.9999999999999716, 84.60249999999999204 ) ) ;
#67203=CARTESIAN_POINT ( 'NONE',  ( 96.15314808468748708, -208.0026889286704943, 80.06489583420048461 ) ) ;
#67211=CARTESIAN_POINT ( 'NONE',  ( 97.64999999999999147, -209.9999999999999716, 76.98250000000000171 ) ) ;
#67213=CARTESIAN_POINT ( 'NONE',  ( 92.69370383062501162, -208.6684592857803011, 75.77864583420048916 ) ) ;
#67219=VERTEX_POINT ( 'NONE', #31835 ) ;
#67225=ORIENTED_EDGE ( 'NONE', *, *, #18099, .T. ) ;
#67227=CARTESIAN_POINT ( 'NONE',  ( 96.32499999999998863, -212.2949673200287179, 78.86104166840097207 ) ) ;
#67228=CARTESIAN_POINT ( 'NONE',  ( 92.34999999999999432, 88.47002178664753558, 80.52791666666665549 ) ) ;
#67233=CARTESIAN_POINT ( 'NONE',  ( -93.14543241548911112, -211.3788240028428618, 74.79348190356847681 ) ) ;
#67236=CARTESIAN_POINT ( 'NONE',  ( 96.32499999999997442, 92.29496732002878900, 84.15270833506762926 ) ) ;
#67237=( BOUNDED_CURVE ( )  B_SPLINE_CURVE ( 2, ( #62572, #50134, #61069, #11054, #20838, #9562, #67072 ),
 .UNSPECIFIED., .F., .F. ) 
 B_SPLINE_CURVE_WITH_KNOTS ( ( 3, 2, 2, 3 ),
 ( 0.9101937466091534201, 0.9172495203147084109, 0.9243052858555913520, 0.9313609857393206903 ),
 .UNSPECIFIED. ) 
 CURVE ( )  GEOMETRIC_REPRESENTATION_ITEM ( )  RATIONAL_B_SPLINE_CURVE ( ( 1.000000000000000000, 0.8660254037844387076, 1.000000000000000000, 0.8660254037844387076, 1.000000000000000000, 0.8660266504798650455, 0.9999975066323494310 ) ) 
 REPRESENTATION_ITEM ( '' )  );
#67238=CARTESIAN_POINT ( 'NONE',  ( -95.00000000000002842, 92.66308142843932671, 84.56281250086716739 ) ) ;
#67239=CARTESIAN_POINT ( 'NONE',  ( 93.84685191531248449, 91.99731107132950569, 78.74197916753381321 ) ) ;
#67248=CARTESIAN_POINT ( 'NONE',  ( -92.69370383062498320, -211.3315407142195852, 81.65239583420049030 ) ) ;
#67253=EDGE_CURVE ( 'NONE', #3617, #37865, #13444, .T. ) ;
#67255=CARTESIAN_POINT ( 'NONE',  ( 94.99999999999998579, 86.94004357329500010, 88.33312500173428816 ) ) ;
#67257=CARTESIAN_POINT ( 'NONE',  ( -96.15314808468747287, -208.0026889286704943, 79.37697916753380412 ) ) ;
#67260=CARTESIAN_POINT ( 'NONE',  ( 92.34999999999999432, 91.52997821335252127, 88.75645833506762017 ) ) ;
#67262=DIRECTION ( 'NONE',  ( -0.000000000000000000, -0.000000000000000000, 1.000000000000000000 ) ) ;
#67270=CARTESIAN_POINT ( 'NONE',  ( 96.15314808468748708, 91.99731107132950569, 89.43114583420047836 ) ) ;
#67283=CARTESIAN_POINT ( 'NONE',  ( -93.67499999999998295, -212.2949673200287179, 85.76666666666665151 ) ) ;
#67289=CARTESIAN_POINT ( 'NONE',  ( 97.64999999999999147, -209.9999999999999716, 77.61749999999999261 ) ) ;
#67292=CARTESIAN_POINT ( 'NONE',  ( 96.15314808468750130, -211.9973110713294489, 89.37822916753381719 ) ) ;
#67293=EDGE_CURVE ( 'NONE', #14612, #23771, #40563, .T. ) ;
#67296=ORIENTED_EDGE ( 'NONE', *, *, #41071, .F. ) ;
#67301=CARTESIAN_POINT ( 'NONE',  ( 97.30629616937498838, -211.3315407142195852, 79.11239583420046984 ) ) ;
#67302=CARTESIAN_POINT ( 'NONE',  ( 97.30629616937498838, -211.3315407142195852, 85.62114583420047609 ) ) ;
#67304=CARTESIAN_POINT ( 'NONE',  ( 93.84685191531249870, -208.0026889286704943, 85.25072916753381946 ) ) ;
#67314=CARTESIAN_POINT ( 'NONE',  ( 93.67500000000001137, -212.2949673200287179, 88.91520833506763211 ) ) ;
#67316=ORIENTED_EDGE ( 'NONE', *, *, #20092, .F. ) ;
#67321=ORIENTED_EDGE ( 'NONE', *, *, #17552, .T. ) ;
#67327=DIRECTION ( 'NONE',  ( 0.000000000000000000, 0.000000000000000000, -1.000000000000000000 ) ) ;
#67328=ORIENTED_EDGE ( 'NONE', *, *, #4074, .F. ) ;
#67329=AXIS2_PLACEMENT_3D ( 'NONE', #33778, #27380, #55595 ) ;
#67335=CARTESIAN_POINT ( 'NONE',  ( -93.67500000000003979, 92.29496732002878900, 89.78833333333332689 ) ) ;
#67337=CARTESIAN_POINT ( 'NONE',  ( 97.30629616937498838, 88.66845928578037217, 78.47739583420047893 ) ) ;
#67338=ORIENTED_EDGE ( 'NONE', *, *, #57672, .T. ) ;
#67339=CARTESIAN_POINT ( 'NONE',  ( 97.64999999981932888, 89.99996905681224746, 78.33187387208513996 ) ) ;
#67340=CARTESIAN_POINT ( 'NONE',  ( -93.84685191531248449, -208.0026889286704943, 88.16114583420046813 ) ) ;
#67341=ORIENTED_EDGE ( 'NONE', *, *, #3316, .F. ) ;
#67344=CARTESIAN_POINT ( 'NONE',  ( 92.35000000019410038, 89.99998015720535705, 86.27002759516707897 ) ) ;
#67345=CARTESIAN_POINT ( 'NONE',  ( -92.69370383062498320, -208.6684592857803295, 81.12322916753380753 ) ) ;
#67353=CARTESIAN_POINT ( 'NONE',  ( 95.99319914654141428, -207.8660161998918454, 74.81432998548488911 ) ) ;
#67354=CARTESIAN_POINT ( 'NONE',  ( -92.69370383062504004, 90.00000000000004263, 80.43531250086714124 ) ) ;
#67357=ORIENTED_EDGE ( 'NONE', *, *, #62949, .T. ) ;
#67366=CARTESIAN_POINT ( 'NONE',  ( -92.69370383062498320, -211.3315407142195852, 78.63614583420049087 ) ) ;
#67370=EDGE_CURVE ( 'NONE', #7767, #29135, #72263, .T. ) ;
#67371=CARTESIAN_POINT ( 'NONE',  ( -97.65000000000001990, 90.00000000000004263, 88.73000000000000398 ) ) ;
#67387=CARTESIAN_POINT ( 'NONE',  ( 93.84685191531249870, -208.0026889286704943, 88.26697916753380468 ) ) ;
#67388=CARTESIAN_POINT ( 'NONE',  ( -92.35000000045951651, -209.9999506483816560, 87.22187670868756015 ) ) ;
#67398=ADVANCED_FACE ( 'NONE', ( #68296 ), #45372, .F. ) ;
#67399=EDGE_CURVE ( 'NONE', #53082, #50665, #5530, .T. ) ;
#67400=ORIENTED_EDGE ( 'NONE', *, *, #63794, .F. ) ;
#67403=CARTESIAN_POINT ( 'NONE',  ( 94.99999999999998579, 87.33691857156068750, 77.89531250086714920 ) ) ;
#67404=LINE ( 'NONE', #5389, #11951 ) ;
#67411=CARTESIAN_POINT ( 'NONE',  ( 97.30629616937498838, 88.66845928578037217, 88.00239583420047040 ) ) ;
#67414=CARTESIAN_POINT ( 'NONE',  ( 92.69370383062501162, -209.9999999999999716, 84.56281250086713897 ) ) ;
#67415=EDGE_CURVE ( 'NONE', #35038, #35410, #26572, .T. ) ;
#67419=DIRECTION ( 'NONE',  ( -0.000000000000000000, -0.000000000000000000, 1.000000000000000000 ) ) ;
#67422=CARTESIAN_POINT ( 'NONE',  ( 94.99999999999998579, 90.00000000000002842, 90.00000000000000000 ) ) ;
#67424=CARTESIAN_POINT ( 'NONE',  ( -97.30629616937497417, -211.3315407142195852, 89.06072916753379332 ) ) ;
#67425=CARTESIAN_POINT ( 'NONE',  ( -96.15314808468751551, 88.00268892867056536, 87.36739583420049371 ) ) ;
#67426=VECTOR ( 'NONE', #1086, 1000.000000000000000 ) ;
#67428=CARTESIAN_POINT ( 'NONE',  ( 96.15314808468748708, 88.00268892867053694, 86.67947916753381321 ) ) ;
#67429=CARTESIAN_POINT ( 'NONE',  ( -97.30629616937501680, 91.33154071421968467, 89.58989583420047609 ) ) ;
#67430=ORIENTED_EDGE ( 'NONE', *, *, #60291, .T. ) ;
#67431=CARTESIAN_POINT ( 'NONE',  ( 93.67500000000001137, -212.2949673200287179, 84.47020833506762472 ) ) ;
#67435=CARTESIAN_POINT ( 'NONE',  ( -93.84685191531248449, -208.0026889286704943, 89.43114583420047836 ) ) ;
#67436=CARTESIAN_POINT ( 'NONE',  ( -92.34999999999999432, -209.9999999999999716, 82.06250000000000000 ) ) ;
#67440=VERTEX_POINT ( 'NONE', #38227 ) ;
#67444=CARTESIAN_POINT ( 'NONE',  ( -97.65000000000001990, 91.52997821335253548, 80.42208333333331893 ) ) ;
#67450=DIRECTION ( 'NONE',  ( -0.000000000000000000, -0.000000000000000000, 1.000000000000000000 ) ) ;
#67451=( BOUNDED_CURVE ( )  B_SPLINE_CURVE ( 2, ( #26443, #38094, #30961, #25342, #71923, #43754, #36983 ),
 .UNSPECIFIED., .F., .F. ) 
 B_SPLINE_CURVE_WITH_KNOTS ( ( 3, 2, 2, 3 ),
 ( 0.3125000000000001665, 0.3194444444444445308, 0.3263888888888890061, 0.3333333333333333703 ),
 .UNSPECIFIED. ) 
 CURVE ( )  GEOMETRIC_REPRESENTATION_ITEM ( )  RATIONAL_B_SPLINE_CURVE ( ( 0.9999999999999967804, 0.8660254037844419273, 1.000000000000000000, 0.8660254037844387076, 1.000000000000000000, 0.8660254037844375974, 1.000000000000001110 ) ) 
 REPRESENTATION_ITEM ( '' )  );
#67452=CARTESIAN_POINT ( 'NONE',  ( -92.34999999999999432, -208.4700217866474645, 79.57541666666666913 ) ) ;
#67454=CARTESIAN_POINT ( 'NONE',  ( -97.30629616937501680, 88.66845928578038638, 81.44072916753381719 ) ) ;
#67456=DIRECTION ( 'NONE',  ( 1.000000000000000000, 0.000000000000000000, 0.000000000000000000 ) ) ;
#67460=DIRECTION ( 'NONE',  ( -0.000000000000000000, -0.000000000000000000, 1.000000000000000000 ) ) ;
#67465=( BOUNDED_CURVE ( )  B_SPLINE_CURVE ( 2, ( #9912, #4670, #73800, #33960, #27577, #50506, #21940, #56908, #15181 ),
 .UNSPECIFIED., .F., .F. ) 
 B_SPLINE_CURVE_WITH_KNOTS ( ( 3, 2, 2, 2, 3 ),
 ( 0.5715170088694363493, 0.5785727743551949409, 0.5856285398961110777, 0.5926843054370272146, 0.5926843883826560244 ),
 .UNSPECIFIED. ) 
 CURVE ( )  GEOMETRIC_REPRESENTATION_ITEM ( )  RATIONAL_B_SPLINE_CURVE ( ( 1.000000000000000000, 0.8660254037844387076, 1.000000000000000000, 0.8660254037844387076, 1.000000000000000000, 0.8660254037844387076, 1.000000000000000000, 0.9999984250316910073, 0.9999968501004118382 ) ) 
 REPRESENTATION_ITEM ( '' )  );
#67466=CARTESIAN_POINT ( 'NONE',  ( 97.30629616937498838, 91.33154071421968467, 80.64697916753382856 ) ) ;
#67468=CARTESIAN_POINT ( 'NONE',  ( -97.30629616937497417, -211.3315407142195852, 84.13947916753383538 ) ) ;
#67473=CARTESIAN_POINT ( 'NONE',  ( -92.34999999999999432, -208.4700217866474645, 78.94041666666666401 ) ) ;
#67477=CARTESIAN_POINT ( 'NONE',  ( -96.15314808468751551, 88.00268892867056536, 78.47739583420049314 ) ) ;
#67478=CARTESIAN_POINT ( 'NONE',  ( 92.69370383062501162, -209.9999999999999716, 80.75281250086715090 ) ) ;
#67485=CARTESIAN_POINT ( 'NONE',  ( -96.32499999999996021, -207.7050326799711968, 76.00354166840097037 ) ) ;
#67493=CARTESIAN_POINT ( 'NONE',  ( 93.84685191531251292, -211.9973110713294489, 76.57239583420049200 ) ) ;
#67496=ORIENTED_EDGE ( 'NONE', *, *, #47466, .T. ) ;
#67499=CARTESIAN_POINT ( 'NONE',  ( 92.69370383062498320, 88.66845928578037217, 86.04447916753382231 ) ) ;
#67501=CARTESIAN_POINT ( 'NONE',  ( 95.00000000000000000, -213.0599564267049857, 78.72875000000001933 ) ) ;
#67503=VERTEX_POINT ( 'NONE', #41197 ) ;
#67512=FACE_OUTER_BOUND ( 'NONE', #43386, .T. ) ;
#67514=CARTESIAN_POINT ( 'NONE',  ( -96.32499999999996021, -207.7050326799711968, 82.35354166840096468 ) ) ;
#67518=CARTESIAN_POINT ( 'NONE',  ( 96.32499999999997442, 92.29496732002878900, 84.15270833506762926 ) ) ;
#67519=CARTESIAN_POINT ( 'NONE',  ( -96.32500000000001705, 92.29496732002878900, 82.98854166840096980 ) ) ;
#67521=CARTESIAN_POINT ( 'NONE',  ( 92.69370383062498320, 91.33154071421968467, 84.03364583420049883 ) ) ;
#67523=CARTESIAN_POINT ( 'NONE',  ( -97.64999999999996305, -211.5299782133524218, 82.51229166840094820 ) ) ;
#67527=DIRECTION ( 'NONE',  ( -1.000000000000000000, -1.343011723336883198E-16, -0.000000000000000000 ) ) ;
#67537=CARTESIAN_POINT ( 'NONE',  ( 97.64999999999999147, -209.9999999999999716, 90.00000000000000000 ) ) ;
#67541=CARTESIAN_POINT ( 'NONE',  ( -94.99999999999997158, -207.3369185715606307, 79.48281250086715488 ) ) ;
#67545=CARTESIAN_POINT ( 'NONE',  ( -97.64999999953586496, -210.0000309672219601, 77.38038495123339544 ) ) ;
#67550=CARTESIAN_POINT ( 'NONE',  ( 97.30629616937498838, 91.33154071421968467, 76.04322916753380923 ) ) ;
#67554=FACE_OUTER_BOUND ( 'NONE', #414, .T. ) ;
#67555=CARTESIAN_POINT ( 'NONE',  ( -90.00000000000002842, 95.00000000000002842, -79.99999999999998579 ) ) ;
#67563=CARTESIAN_POINT ( 'NONE',  ( -93.67500000000003979, 87.70503267997129626, 78.22604166840096696 ) ) ;
#67566=CARTESIAN_POINT ( 'NONE',  ( -95.00000000000002842, 87.33691857156074434, 84.08656250086714579 ) ) ;
#67568=CARTESIAN_POINT ( 'NONE',  ( -97.65000000000001990, 90.00000000000004263, 90.00000000000000000 ) ) ;
#67569=VERTEX_POINT ( 'NONE', #34434 ) ;
#67570=CARTESIAN_POINT ( 'NONE',  ( 94.99999999999998579, 90.00000000000002842, 90.00000000000000000 ) ) ;
#67575=CARTESIAN_POINT ( 'NONE',  ( 93.84685191531251292, -211.9973110713294489, 79.11239583420048405 ) ) ;
#67578=( BOUNDED_CURVE ( )  B_SPLINE_CURVE ( 2, ( #7274, #35822, #7635, #64791, #1670, #63691, #24923, #70777, #35103 ),
 .UNSPECIFIED., .F., .F. ) 
 B_SPLINE_CURVE_WITH_KNOTS ( ( 3, 2, 2, 2, 3 ),
 ( 0.3386766260338262002, 0.3386767459623536425, 0.3457325115032360840, 0.3527882770441184701, 0.3598440426530883918 ),
 .UNSPECIFIED. ) 
 CURVE ( )  GEOMETRIC_REPRESENTATION_ITEM ( )  RATIONAL_B_SPLINE_CURVE ( ( 0.9999954456811690484, 0.9999977228018784858, 1.000000000000000000, 0.8660254037844387076, 1.000000000000000000, 0.8660254037844387076, 1.000000000000000000, 0.8660254037844387076, 1.000000000000000000 ) ) 
 REPRESENTATION_ITEM ( '' )  );
#67579=ORIENTED_EDGE ( 'NONE', *, *, #16530, .T. ) ;
#67582=CARTESIAN_POINT ( 'NONE',  ( 96.73972734126404305, -208.4859488783623362, 74.79348190356850523 ) ) ;
#67583=CARTESIAN_POINT ( 'NONE',  ( -92.35000000000003695, 90.00000000000004263, 90.00000000000000000 ) ) ;
#67588=CARTESIAN_POINT ( 'NONE',  ( 93.67500000000001137, -207.7050326799711968, 87.35416666666665719 ) ) ;
#67596=CARTESIAN_POINT ( 'NONE',  ( 26.50000000000000355, -120.0000000000000000, -64.00000000000000000 ) ) ;
#67599=CARTESIAN_POINT ( 'NONE',  ( 97.64999999999997726, -208.4700217866474645, 80.28979166840098003 ) ) ;
#67600=CARTESIAN_POINT ( 'NONE',  ( 93.67499999999999716, 87.70503267997126784, 82.48583333333333201 ) ) ;
#67604=CARTESIAN_POINT ( 'NONE',  ( -92.34999999999999432, -208.4700217866474645, 82.82979166840095786 ) ) ;
#67607=CARTESIAN_POINT ( 'NONE',  ( -95.00000000000002842, 92.66308142843932671, 85.19781250086714408 ) ) ;
#67608=CARTESIAN_POINT ( 'NONE',  ( 92.69370383062498320, 88.66845928578037217, 79.53572916753380184 ) ) ;
#67614=EDGE_LOOP ( 'NONE', ( #14768, #25149, #55113, #44663 ) ) ;
#67616=CARTESIAN_POINT ( 'NONE',  ( -92.69370383062498320, -208.6684592857803011, 80.48822916753383083 ) ) ;
#67620=ORIENTED_EDGE ( 'NONE', *, *, #38020, .T. ) ;
#67621=CYLINDRICAL_SURFACE ( 'NONE', #59997, 2.649999999999985700 ) ;
#67625=CARTESIAN_POINT ( 'NONE',  ( 92.34999999999990905, 88.47002178664757821, 80.52791666666665549 ) ) ;
#67627=CARTESIAN_POINT ( 'NONE',  ( -92.69370383062498320, -209.9999999999999716, 75.35531250086714294 ) ) ;
#67628=ORIENTED_EDGE ( 'NONE', *, *, #65150, .T. ) ;
#67629=CARTESIAN_POINT ( 'NONE',  ( -92.35000000000003695, 90.00000000000004263, 86.50750000000000739 ) ) ;
#67634=CARTESIAN_POINT ( 'NONE',  ( -97.64999999999993463, 88.47002178664749295, 81.16291666666667481 ) ) ;
#67636=VECTOR ( 'NONE', #66293, 1000.000000000000000 ) ;
#67638=CARTESIAN_POINT ( 'NONE',  ( 92.69370383062498320, 90.00000000000002842, 87.73781250086713612 ) ) ;
#67641=ADVANCED_FACE ( 'NONE', ( #40835 ), #52462, .F. ) ;
#67646=CARTESIAN_POINT ( 'NONE',  ( 97.64999999997402824, 89.99998827382246702, 82.77687459617033028 ) ) ;
#67654=CARTESIAN_POINT ( 'NONE',  ( 97.64999999999999147, -209.9999999999999716, 82.06250000000000000 ) ) ;
#67658=CARTESIAN_POINT ( 'NONE',  ( -92.34999999999999432, -208.4700217866474645, 84.02041666666667652 ) ) ;
#67668=CARTESIAN_POINT ( 'NONE',  ( 96.15314808468750130, -211.9973110713294489, 87.47322916753381605 ) ) ;
#67676=( BOUNDED_CURVE ( )  B_SPLINE_CURVE ( 2, ( #1792, #47606, #69070, #13016, #35950, #57790, #18293 ),
 .UNSPECIFIED., .F., .F. ) 
 B_SPLINE_CURVE_WITH_KNOTS ( ( 3, 2, 2, 3 ),
 ( 0.5833333333333329263, 0.5902777777777776791, 0.5972222222222223209, 0.6041666666666670737 ),
 .UNSPECIFIED. ) 
 CURVE ( )  GEOMETRIC_REPRESENTATION_ITEM ( )  RATIONAL_B_SPLINE_CURVE ( ( 1.000000000000008660, 0.8660254037844301589, 1.000000000000000000, 0.8660254037844387076, 1.000000000000000000, 0.8660254037844301589, 1.000000000000008660 ) ) 
 REPRESENTATION_ITEM ( '' )  );
#67677=CARTESIAN_POINT ( 'NONE',  ( 93.84685191531249870, -208.0026889286704943, 78.74197916753381321 ) ) ;
#67679=CARTESIAN_POINT ( 'NONE',  ( 96.15314808468750130, -211.9973110713294489, 82.39322916753381776 ) ) ;
#67689=CARTESIAN_POINT ( 'NONE',  ( -96.32500000000001705, 87.70503267997129626, 77.40583333333331950 ) ) ;
#67708=CARTESIAN_POINT ( 'NONE',  ( -99.99999999999998579, -124.0000000000000142, -40.00000000000002132 ) ) ;
#67709=CARTESIAN_POINT ( 'NONE',  ( -97.30629616937501680, 91.33154071421968467, 77.04864583420048518 ) ) ;
#67711=CARTESIAN_POINT ( 'NONE',  ( 96.15314808468748708, 91.99731107132950569, 77.36614583420046642 ) ) ;
#67712=ORIENTED_EDGE ( 'NONE', *, *, #45247, .T. ) ;
#67714=CARTESIAN_POINT ( 'NONE',  ( -97.30629616937495996, -209.9999999999999716, 85.19781250086714408 ) ) ;
#67719=CARTESIAN_POINT ( 'NONE',  ( -97.30629616937497417, -208.6684592857803295, 80.69989583420046131 ) ) ;
#67730=CARTESIAN_POINT ( 'NONE',  ( 94.99999999999998579, 93.05995642670504253, 84.76125000000000398 ) ) ;
#67731=DIRECTION ( 'NONE',  ( -1.000000000000000000, 0.000000000000000000, 0.000000000000000000 ) ) ;
#67732=CARTESIAN_POINT ( 'NONE',  ( -92.69370383062504004, 90.00000000000004263, 82.34031250086714238 ) ) ;
#67742=CARTESIAN_POINT ( 'NONE',  ( -92.35000000000005116, 91.52997821335254969, 89.73541666666663730 ) ) ;
#67743=CARTESIAN_POINT ( 'NONE',  ( 92.35000000000000853, -209.9999999999999716, 88.80937500173430976 ) ) ;
#67744=CARTESIAN_POINT ( 'NONE',  ( -93.84685191531247028, -211.9973110713294489, 79.85322916753381151 ) ) ;
#67750=CARTESIAN_POINT ( 'NONE',  ( -92.34999999999998010, 91.52997821335249284, 88.46541666666664128 ) ) ;
#67764=DIRECTION ( 'NONE',  ( 1.000000000000000000, 0.000000000000000000, 0.000000000000000000 ) ) ;
#67765=VERTEX_POINT ( 'NONE', #41939 ) ;
#67766=VECTOR ( 'NONE', #18744, 1000.000000000000000 ) ;
#67767=CARTESIAN_POINT ( 'NONE',  ( 95.00000000000000000, -212.6630814284392557, 87.26156250086714294 ) ) ;
#67769=ORIENTED_EDGE ( 'NONE', *, *, #41592, .T. ) ;
#67776=EDGE_LOOP ( 'NONE', ( #2925, #41549, #1962, #68569 ) ) ;
#67781=CARTESIAN_POINT ( 'NONE',  ( 94.99999999999998579, 92.66308142843935514, 76.94281250086714863 ) ) ;
#67787=CARTESIAN_POINT ( 'NONE',  ( 94.99999999999998579, 87.33691857156068750, 87.89656250086713385 ) ) ;
#67789=CARTESIAN_POINT ( 'NONE',  ( 96.15314808468748708, -208.0026889286704943, 84.35114583420048007 ) ) ;
#67792=CARTESIAN_POINT ( 'NONE',  ( -92.34999999999999432, -209.9999999999999716, 90.00000000000000000 ) ) ;
#67798=CARTESIAN_POINT ( 'NONE',  ( -97.30629616937497417, -208.6684592857803011, 88.31989583420046586 ) ) ;
#67799=CARTESIAN_POINT ( 'NONE',  ( -95.00000000000002842, 92.66308142843932671, 87.10281250086715943 ) ) ;
#67801=CARTESIAN_POINT ( 'NONE',  ( 92.69370383062498320, 91.33154071421968467, 88.95489583420048518 ) ) ;
#67802=CARTESIAN_POINT ( 'NONE',  ( -95.00000000000002842, 87.33691857156074434, 84.72156250086713669 ) ) ;
#67804=CARTESIAN_POINT ( 'NONE',  ( 95.00000000000000000, -213.0599564267049857, 84.52312500173428589 ) ) ;
#67805=CARTESIAN_POINT ( 'NONE',  ( -95.00000000000002842, 90.00000000000004263, 90.00000000000000000 ) ) ;
#67815=EDGE_CURVE ( 'NONE', #49448, #69189, #13355, .T. ) ;
#67817=EDGE_CURVE ( 'NONE', #16386, #23771, #4340, .T. ) ;
#67818=CARTESIAN_POINT ( 'NONE',  ( -97.65000000000001990, 88.47002178664754979, 83.06791666666664753 ) ) ;
#67820=CARTESIAN_POINT ( 'NONE',  ( -95.00000000000002842, 90.00000000000004263, 90.00000000000000000 ) ) ;
#67828=CARTESIAN_POINT ( 'NONE',  ( -92.69370383062504004, 90.00000000000004263, 82.97531250086714749 ) ) ;
#67832=CARTESIAN_POINT ( 'NONE',  ( -23.50044424985255276, 0.001194404164626844313, -80.00000000000000000 ) ) ;
#67835=CARTESIAN_POINT ( 'NONE',  ( -92.35000000000003695, 90.00000000000004263, 82.06250000000000000 ) ) ;
#67836=CYLINDRICAL_SURFACE ( 'NONE', #16613, 2.649999999999985700 ) ;
#67840=CIRCLE ( 'NONE', #39081, 15.70000000000000284 ) ;
#67841=CARTESIAN_POINT ( 'NONE',  ( 97.30629616937498838, 90.00000000000002842, 81.86406250086714920 ) ) ;
#67842=CARTESIAN_POINT ( 'NONE',  ( -97.30629616937497417, -211.3315407142195852, 80.32947916753381890 ) ) ;
#67844=VERTEX_POINT ( 'NONE', #10680 ) ;
#67846=CARTESIAN_POINT ( 'NONE',  ( -92.34999999999999432, -209.9999999999999716, 75.07749999999998636 ) ) ;
#67847=CARTESIAN_POINT ( 'NONE',  ( 97.64999999999999147, -209.9999733970770137, 78.96687592183759818 ) ) ;
#67849=EDGE_CURVE ( 'NONE', #47502, #26794, #73455, .T. ) ;
#67851=CARTESIAN_POINT ( 'NONE',  ( -96.15314808468752972, 91.99731107132950569, 77.63072916753381492 ) ) ;
#67852=CARTESIAN_POINT ( 'NONE',  ( 96.15314808468748708, -208.0026889286704943, 79.90614583420047268 ) ) ;
#67856=AXIS2_PLACEMENT_3D ( 'NONE', #29153, #1008, #63039 ) ;
#67857=CARTESIAN_POINT ( 'NONE',  ( -94.99999999999997158, -206.9400435732949575, 88.01562500173432113 ) ) ;
#67858=VECTOR ( 'NONE', #62066, 1000.000000000000000 ) ;
#67866=CARTESIAN_POINT ( 'NONE',  ( 97.30629616937498838, -211.3315407142195852, 75.46114583420049371 ) ) ;
#67867=EDGE_LOOP ( 'NONE', ( #56736, #41546, #5937, #24490 ) ) ;
#67869=CARTESIAN_POINT ( 'NONE',  ( -97.64999999993850111, -209.9999881787635729, 81.82400613094797848 ) ) ;
#67870=CARTESIAN_POINT ( 'NONE',  ( 97.30629616937498838, 88.66845928578037217, 86.89114583420050053 ) ) ;
#67872=CARTESIAN_POINT ( 'NONE',  ( 97.64999999999997726, -211.5299782133524502, 76.92958333333332632 ) ) ;
#67884=CARTESIAN_POINT ( 'NONE',  ( -92.35000000005462084, -210.0000170173125014, 88.49187441316038871 ) ) ;
#67888=CARTESIAN_POINT ( 'NONE',  ( -93.67499999999998295, -207.7050326799711968, 84.15270833506762926 ) ) ;
#67893=CARTESIAN_POINT ( 'NONE',  ( 96.32499999999997442, 92.29496732002878900, 83.51770833506763836 ) ) ;
#67894=CARTESIAN_POINT ( 'NONE',  ( -95.00000000000002842, 86.94004357329504273, 78.17312500173430578 ) ) ;
#67895=( BOUNDED_CURVE ( )  B_SPLINE_CURVE ( 2, ( #6281, #23557, #46486, #56677, #28447, #22078, #45394, #45022, #51380 ),
 .UNSPECIFIED., .F., .F. ) 
 B_SPLINE_CURVE_WITH_KNOTS ( ( 3, 2, 2, 2, 3 ),
 ( 0.6138516023186938453, 0.6209073675976484186, 0.6279631331385308046, 0.6350188986794130797, 0.6350190250571088324 ),
 .UNSPECIFIED. ) 
 CURVE ( )  GEOMETRIC_REPRESENTATION_ITEM ( )  RATIONAL_B_SPLINE_CURVE ( ( 1.000000000000000000, 0.8660254037844387076, 1.000000000000000000, 0.8660254037844387076, 1.000000000000000000, 0.8660254037844387076, 1.000000000000000000, 0.9999976003453262541, 0.9999952007766141904 ) ) 
 REPRESENTATION_ITEM ( '' )  );
#67897=CARTESIAN_POINT ( 'NONE',  ( 93.84685191531248449, 88.00268892867053694, 82.92239583420048632 ) ) ;
#67898=CARTESIAN_POINT ( 'NONE',  ( -93.67500000000003979, 87.70503267997129626, 76.24166666666666003 ) ) ;
#67899=DIRECTION ( 'NONE',  ( 1.343011723336883198E-16, -1.000000000000000000, 0.000000000000000000 ) ) ;
#67915=CARTESIAN_POINT ( 'NONE',  ( -94.99999999999997158, -207.3369185715606307, 82.02281250086714692 ) ) ;
#67918=CARTESIAN_POINT ( 'NONE',  ( -96.15314808468751551, 88.00268892867056536, 88.47864583420047779 ) ) ;
#67925=CARTESIAN_POINT ( 'NONE',  ( 93.84685191531248449, 91.99731107132950569, 75.56697916753381605 ) ) ;
#67927=CARTESIAN_POINT ( 'NONE',  ( 94.99999999999998579, 86.94004357329502852, 78.17312500173430578 ) ) ;
#67929=CARTESIAN_POINT ( 'NONE',  ( -96.32499999999996021, -207.7050326799711968, 76.63854166840096127 ) ) ;
#67930=CARTESIAN_POINT ( 'NONE',  ( -93.26027265873587169, -208.4859488783624215, 74.79348190356851944 ) ) ;
#67931=EDGE_CURVE ( 'NONE', #22766, #47765, #59909, .T. ) ;
#67936=CARTESIAN_POINT ( 'NONE',  ( 95.00000000000000000, -206.9400435732949575, 79.12562500173429214 ) ) ;
#67938=CARTESIAN_POINT ( 'NONE',  ( -92.69370383062498320, -211.3315407142195852, 89.43114583420049257 ) ) ;
#67942=CARTESIAN_POINT ( 'NONE',  ( -93.84685191531254134, 91.99731107132950569, 78.63614583420047666 ) ) ;
#67944=CARTESIAN_POINT ( 'NONE',  ( 97.30629616937498838, -211.3315407142195852, 89.27239583420048064 ) ) ;
#67949=CARTESIAN_POINT ( 'NONE',  ( -94.99999999999997158, -206.9400435732949575, 84.76125000000000398 ) ) ;
#67950=CARTESIAN_POINT ( 'NONE',  ( 97.30629616937498838, -211.3315407142195852, 75.46114583420049371 ) ) ;
#67953=CARTESIAN_POINT ( 'NONE',  ( 92.69370383062501162, -209.9999999999999716, 89.64281250086713726 ) ) ;
#67955=CARTESIAN_POINT ( 'NONE',  ( -97.64999999999996305, -209.9999999999999716, 85.63437500173431260 ) ) ;
#67958=CARTESIAN_POINT ( 'NONE',  ( 92.35000000000000853, -209.9999999999999716, 81.82437500173429612 ) ) ;
#67959=CARTESIAN_POINT ( 'NONE',  ( 93.67500000000001137, -207.7050326799711968, 89.89416666666666345 ) ) ;
#67962=CARTESIAN_POINT ( 'NONE',  ( -97.47814808468751835, 90.00000000000004263, 89.90078125043358170 ) ) ;
#67964=ORIENTED_EDGE ( 'NONE', *, *, #63403, .T. ) ;
#67972=CARTESIAN_POINT ( 'NONE',  ( 96.32499999999998863, -207.7050326799711968, 75.26270833506764291 ) ) ;
#67973=CARTESIAN_POINT ( 'NONE',  ( 92.34999999999999432, 90.00000000000002842, 81.10999999999999943 ) ) ;
#67976=ORIENTED_EDGE ( 'NONE', *, *, #829, .T. ) ;
#67977=CARTESIAN_POINT ( 'NONE',  ( -92.35000000000000853, -210.0000058630848798, 82.77687479895044476 ) ) ;
#67981=CARTESIAN_POINT ( 'NONE',  ( -96.15314808468751551, 88.00268892867056536, 86.09739583420049769 ) ) ;
#67982=CARTESIAN_POINT ( 'NONE',  ( 97.30629616937498838, 91.33154071421968467, 79.85322916753379729 ) ) ;
#67986=FACE_OUTER_BOUND ( 'NONE', #48976, .T. ) ;
#67988=CARTESIAN_POINT ( 'NONE',  ( -97.64999999999986358, -208.4700217866474361, 77.88208333333332689 ) ) ;
#67991=CARTESIAN_POINT ( 'NONE',  ( -94.99999999999997158, -207.3369185715606307, 78.05406250086714692 ) ) ;
#67995=CARTESIAN_POINT ( 'NONE',  ( 92.52185191531251007, -209.9999999999999716, 89.90078125043358170 ) ) ;
#67996=EDGE_LOOP ( 'NONE', ( #4541, #64098, #27588, #13354 ) ) ;
#67999=EDGE_LOOP ( 'NONE', ( #49644, #31748, #11644, #314 ) ) ;
#68000=CARTESIAN_POINT ( 'NONE',  ( -94.99999999999997158, -207.3369185715606307, 77.41906250086714181 ) ) ;
#68010=CARTESIAN_POINT ( 'NONE',  ( 92.69370383062498320, 90.00000000000002842, 83.29281250086714294 ) ) ;
#68013=CARTESIAN_POINT ( 'NONE',  ( 97.64999999999999147, -209.9999999999999716, 86.50750000000000739 ) ) ;
#68020=CARTESIAN_POINT ( 'NONE',  ( -92.35000000000016485, 91.52997821335260653, 75.76541666666668107 ) ) ;
#68028=CARTESIAN_POINT ( 'NONE',  ( -92.34999999999999432, -208.4700217866474645, 84.65541666666666742 ) ) ;
#68029=AXIS2_PLACEMENT_3D ( 'NONE', #42730, #73135, #8526 ) ;
#68035=DIRECTION ( 'NONE',  ( -0.000000000000000000, -0.000000000000000000, 1.000000000000000000 ) ) ;
#68038=CARTESIAN_POINT ( 'NONE',  ( 95.00000000000000000, -207.3369185715606307, 85.19781250086714408 ) ) ;
#68044=CARTESIAN_POINT ( 'NONE',  ( 97.30629616937498838, -209.9999999999999716, 79.80031250086713612 ) ) ;
#68046=CARTESIAN_POINT ( 'NONE',  ( 93.84685191531249870, -208.0026889286704943, 83.34572916753383254 ) ) ;
#68050=VERTEX_POINT ( 'NONE', #57290 ) ;
#68053=CARTESIAN_POINT ( 'NONE',  ( 15.70000000000000284, -120.0000000000000000, -85.59999999999999432 ) ) ;
#68068=CARTESIAN_POINT ( 'NONE',  ( 92.69370383062501162, -209.9999999999999716, 75.67281250086713840 ) ) ;
#68078=CARTESIAN_POINT ( 'NONE',  ( -92.69370383062504004, 89.06968786819598449, 74.84209103131394158 ) ) ;
#68082=CARTESIAN_POINT ( 'NONE',  ( 92.69370383062498320, 90.00000000000002842, 75.03781250086713328 ) ) ;
#68085=CARTESIAN_POINT ( 'NONE',  ( 93.67499999999998295, 92.29496732002878900, 75.28916666666665947 ) ) ;
#68086=CARTESIAN_POINT ( 'NONE',  ( -92.69370383062498320, -211.3315407142195852, 84.82739583420045903 ) ) ;
#68089=EDGE_CURVE ( 'NONE', #52810, #67503, #69675, .T. ) ;
#68091=CARTESIAN_POINT ( 'NONE',  ( 92.35000000000000853, -209.9999999999999716, 88.09499999999999886 ) ) ;
#68092=CARTESIAN_POINT ( 'NONE',  ( -93.84685191531248449, -208.0026889286704943, 78.00114583420048575 ) ) ;
#68094=CYLINDRICAL_SURFACE ( 'NONE', #21156, 2.649999999999999467 ) ;
#68100=CARTESIAN_POINT ( 'NONE',  ( 94.68886060456939902, -207.6265741463516861, 74.84415580543368662 ) ) ;
#68102=CARTESIAN_POINT ( 'NONE',  ( -96.15314808468752972, 91.99731107132950569, 81.91697916753381037 ) ) ;
#68107=DIRECTION ( 'NONE',  ( 0.000000000000000000, 0.000000000000000000, -1.000000000000000000 ) ) ;
#68112=CARTESIAN_POINT ( 'NONE',  ( -93.67500000000003979, 92.29496732002878900, 87.24833333333333485 ) ) ;
#68113=CARTESIAN_POINT ( 'NONE',  ( -97.30629616937497417, -211.3315407142195852, 78.42447916753380355 ) ) ;
#68115=( BOUNDED_CURVE ( )  B_SPLINE_CURVE ( 2, ( #56541, #38496, #10292, #5418, #44518, #61436, #68179 ),
 .UNSPECIFIED., .F., .F. ) 
 B_SPLINE_CURVE_WITH_KNOTS ( ( 3, 2, 2, 3 ),
 ( 0.2083333333333331483, 0.2152777777777775681, 0.2222222222222219323, 0.2291666666666663521 ),
 .UNSPECIFIED. ) 
 CURVE ( )  GEOMETRIC_REPRESENTATION_ITEM ( )  RATIONAL_B_SPLINE_CURVE ( ( 1.000000000000003775, 0.8660254037844349329, 1.000000000000000000, 0.8660254037844387076, 1.000000000000000000, 0.8660254037844445918, 0.9999999999999941158 ) ) 
 REPRESENTATION_ITEM ( '' )  );
#68119=CARTESIAN_POINT ( 'NONE',  ( 92.35003715139256997, 91.52999966271907795, 76.69145685134850510 ) ) ;
#68122=CARTESIAN_POINT ( 'NONE',  ( 92.35000000046409241, 89.99996903277681781, 77.38038495127642591 ) ) ;
#68128=CARTESIAN_POINT ( 'NONE',  ( -94.95306897617113862, 87.35041560265752025, 75.00000002508417651 ) ) ;
#68130=CARTESIAN_POINT ( 'NONE',  ( 96.15314808468748708, -208.0026889286704943, 86.89114583420047211 ) ) ;
#68131=CARTESIAN_POINT ( 'NONE',  ( -96.32500000000001705, 92.29496732002878900, 77.82916666666665151 ) ) ;
#68135=ORIENTED_EDGE ( 'NONE', *, *, #7793, .F. ) ;
#68143=EDGE_CURVE ( 'NONE', #23740, #53644, #3272, .T. ) ;
#68144=ADVANCED_FACE ( 'NONE', ( #43255 ), #27033, .F. ) ;
#68150=CARTESIAN_POINT ( 'NONE',  ( 97.64999999999999147, 90.00000000000002842, 87.14249999999999829 ) ) ;
#68152=FACE_OUTER_BOUND ( 'NONE', #70047, .T. ) ;
#68154=ORIENTED_EDGE ( 'NONE', *, *, #24846, .T. ) ;
#68157=CARTESIAN_POINT ( 'NONE',  ( 97.30629616937498838, 91.33154071421968467, 86.20322916753382003 ) ) ;
#68159=CARTESIAN_POINT ( 'NONE',  ( 92.69370383062501162, -211.3315407142195852, 85.25072916753379104 ) ) ;
#68162=CARTESIAN_POINT ( 'NONE',  ( -96.32500000000001705, 92.29496732002878900, 77.90854166840097150 ) ) ;
#68166=CARTESIAN_POINT ( 'NONE',  ( -96.15314808468747287, -208.0026889286704943, 86.36197916753381776 ) ) ;
#68167=CARTESIAN_POINT ( 'NONE',  ( -95.00000000000002842, 87.33691857156074434, 86.78531250086716398 ) ) ;
#68170=CARTESIAN_POINT ( 'NONE',  ( 92.69370383062498320, 88.66845928578037217, 85.25072916753379104 ) ) ;
#68171=CARTESIAN_POINT ( 'NONE',  ( -96.15314808468752972, 91.99731107132950569, 85.09197916753380753 ) ) ;
#68179=CARTESIAN_POINT ( 'NONE',  ( -92.35000000000003695, 90.00000000000004263, 86.50750000000000739 ) ) ;
#68183=DIRECTION ( 'NONE',  ( 0.000000000000000000, -0.000000000000000000, -1.000000000000000000 ) ) ;
#68187=EDGE_LOOP ( 'NONE', ( #61216, #17312, #27003, #2191 ) ) ;
#68188=AXIS2_PLACEMENT_3D ( 'NONE', #54863, #27389, #50331 ) ;
#68191=CARTESIAN_POINT ( 'NONE',  ( -92.35000000000005116, 88.47002178664754979, 79.46958333333333258 ) ) ;
#68194=CARTESIAN_POINT ( 'NONE',  ( -92.35000000000000853, 88.47002178664756400, 78.83458333333334167 ) ) ;
#68195=CARTESIAN_POINT ( 'NONE',  ( -100.0000000000000142, 95.00000000000002842, 90.00000000000000000 ) ) ;
#68201=CARTESIAN_POINT ( 'NONE',  ( -97.30629616937501680, 91.33154071421968467, 78.15989583420048348 ) ) ;
#68210=CARTESIAN_POINT ( 'NONE',  ( -96.15314808468745866, -211.9973110713294489, 88.63739583420048973 ) ) ;
#68215=CARTESIAN_POINT ( 'NONE',  ( 94.99999999999998579, 92.66308142843932671, 76.30781250086715772 ) ) ;
#68216=CARTESIAN_POINT ( 'NONE',  ( -92.69370383062498320, -211.3315407142195852, 81.17614583420049712 ) ) ;
#68220=CARTESIAN_POINT ( 'NONE',  ( -97.64999999999994884, -208.4700217866474645, 75.34208333333333485 ) ) ;
#68222=CARTESIAN_POINT ( 'NONE',  ( -92.69370383062505425, 91.33154071421968467, 77.47197916753381719 ) ) ;
#68223=CARTESIAN_POINT ( 'NONE',  ( 93.84685191531251292, -211.9973110713294489, 78.95364583420047211 ) ) ;
#68242=CARTESIAN_POINT ( 'NONE',  ( 92.69370383062501162, -211.3315407142195852, 75.88447916753382572 ) ) ;
#68246=CARTESIAN_POINT ( 'NONE',  ( 93.84685191531248449, 88.00268892867053694, 84.82739583420048746 ) ) ;
#68248=CARTESIAN_POINT ( 'NONE',  ( 93.67500000000001137, -207.7050326799711968, 79.73416666666666686 ) ) ;
#68262=DIRECTION ( 'NONE',  ( -0.000000000000000000, -0.000000000000000000, -1.000000000000000000 ) ) ;
#68264=CARTESIAN_POINT ( 'NONE',  ( -97.64999999999994884, -208.4700217866474645, 84.31145833506762699 ) ) ;
#68268=CARTESIAN_POINT ( 'NONE',  ( 92.34999999999999432, 91.52997821335252127, 81.77145833506763495 ) ) ;
#68269=CARTESIAN_POINT ( 'NONE',  ( -95.00000000000002842, 93.05995642670501411, 79.12562500173429214 ) ) ;
#68271=VERTEX_POINT ( 'NONE', #18 ) ;
#68272=CARTESIAN_POINT ( 'NONE',  ( 93.84685191531248449, 91.99731107132950569, 83.34572916753383254 ) ) ;
#68273=CARTESIAN_POINT ( 'NONE',  ( -92.35000000000000853, 88.47002178664759242, 76.29458333333333542 ) ) ;
#68274=CARTESIAN_POINT ( 'NONE',  ( -94.99999999999997158, -213.0599564267049857, 82.61812500173428475 ) ) ;
#68286=CARTESIAN_POINT ( 'NONE',  ( 95.00000000000000000, -209.9999999999999716, 90.00000000000000000 ) ) ;
#68288=CARTESIAN_POINT ( 'NONE',  ( -2.499999999999970690, 73.00000000000001421, -251.7000000000000455 ) ) ;
#68290=CARTESIAN_POINT ( 'NONE',  ( -92.69370383062498320, -211.3315407142195852, 81.81114583420048803 ) ) ;
#68293=CARTESIAN_POINT ( 'NONE',  ( -92.69370383062502583, 88.66845928578038638, 87.36739583420047950 ) ) ;
#68296=FACE_OUTER_BOUND ( 'NONE', #3413, .T. ) ;
#68297=CARTESIAN_POINT ( 'NONE',  ( -96.53982248241459274, -212.0954260604656270, 74.96680960279337569 ) ) ;
#68299=CARTESIAN_POINT ( 'NONE',  ( 92.69370383062498320, 88.66845928578035796, 76.36072916753381890 ) ) ;
#68303=CARTESIAN_POINT ( 'NONE',  ( -93.67499999999998295, -207.7050326799711968, 78.99333333333332519 ) ) ;
#68308=CARTESIAN_POINT ( 'NONE',  ( 93.84685191531248449, 91.99731107132950569, 89.69572916753382685 ) ) ;
#68311=DIRECTION ( 'NONE',  ( -0.000000000000000000, -0.000000000000000000, 1.000000000000000000 ) ) ;
#68313=EDGE_LOOP ( 'NONE', ( #61130, #57215, #29985 ) ) ;
#68314=CARTESIAN_POINT ( 'NONE',  ( -93.09170270117147084, 88.16127723153179829, 74.99954709728268654 ) ) ;
#68315=CARTESIAN_POINT ( 'NONE',  ( -96.15314808468752972, 91.99731107132950569, 80.64697916753381435 ) ) ;
#68319=EDGE_LOOP ( 'NONE', ( #70628, #61408, #7187, #7591 ) ) ;
#68325=CARTESIAN_POINT ( 'NONE',  ( 97.30629616937497417, -210.9303297190751891, 74.84209033237941355 ) ) ;
#68330=VECTOR ( 'NONE', #26724, 1000.000000000000000 ) ;
#68333=( BOUNDED_SURFACE ( )  B_SPLINE_SURFACE ( 1, 2, ( 
 ( #70565, #64969, #20186, #31838, #59688, #36007, #13802, #37132, #71311, #25099, #3306, #30724, #13446, #58955, #36369, #59314, #70948, #19453, #65334, #8171, #54050, #2587, #60078, #48398, #19816, #42765, #37823, #61495, #3987, #49819, #22376, #72381, #73494, #44196, #15986, #3625, #38928, #55476, #62236, #73867, #5106, #61123, #22002, #72741, #49457, #21624, #56220, #44947, #9612, #21240, #32531, #32892, #26890, #4357, #67122, #67870, #15625, #50185, #38558, #55846, #9973, #60753, #16361, #27254, #56602, #4739, #61863, #39304, #73121, #44577, #43839, #67499, #9230, #10348, #33263, #27641, #66397, #14878, #20884, #28003, #32152, #50566, #55098, #66756, #15244, #10727, #33649, #50943, #26524, #38178, #52412, #45320, #16743, #52802, #68246, #57329, #62620, #1345, #18211, #17839, #40789, #17473, #39679, #23855, #5841, #29113, #34020, #28750, #40401, #58067, #51688, #234, #12194, #11097, #593, #23131, #6571, #63721, #46054, #52048, #69341, #23486, #69714, #963, #63350, #29475, #68983, #11815, #68625, #56968, #74240, #46799, #34770, #5478, #28376, #57706, #41152, #46418, #51306, #64092, #40039, #12566, #58430, #11456, #6214, #35135, #22763, #35504, #34389, #6924, #29846, #45698, #17109, #62997, #30958, #8040, #24590, #65570, #70432, #59183, #41885, #25340, #54643, #59934, #43003, #65940, #18938, #42629, #54286, #70071, #30588, #64829, #64454, #8421, #2458, #48635, #70816, #7309, #53909, #13306, #7672, #53536, #2075, #8784, #36606, #31335, #19681, #14038, #48266, #71176, #2810, #14421, #36239, #1705, #24957, #36980, #42270, #24237, #47893, #12925, #19313, #25701, #71555, #37369, #31700, #20052, #60308, #47163, #18573, #41514, #30229, #35860, #13674, #58813, #53170, #47529, #65199, #59555, #26441, #60666, #56128, #62143, #67025, #66311, #44105, #67403, #27164, #55383, #38837, #38092, #49367, #73403, #61776, #71921, #27547, #50482, #33181, #4644, #15530, #38469, #21529, #3538, #21158, #67781, #66668, #15154, #61405, #55757, #43390, #39214, #16268, #14787, #44490, #3902, #9888, #50094, #10627, #72300, #20798, #15903, #33553, #61022, #10257, #48992, #72651, #9522, #32444, #3173, #9147, #21913, #26803, #73022, #37735, #44859, #49727, #26065, #20437, #32070, #43752, #55007, #32805, #4270, #12752, #47348, #36060, #51222, #40978 ),
 ( #1530, #45609, #58620, #70253, #53352, #64278, #41337, #56880, #24410, #28282, #18037, #74150, #7126, #13499, #18760, #1892, #24779, #22662, #41698, #13122, #27920, #63914, #68536, #22287, #64638, #35678, #7497, #29660, #39584, #30042, #12383, #35329, #58258, #6754, #42084, #69895, #59004, #52991, #30407, #47708, #70624, #19138, #65021, #52610, #33934, #1162, #56513, #24059, #5016, #46983, #45229, #18390, #50849, #73775, #68150, #16642, #62531, #11007, #5388, #14977, #3725, #19502, #49556, #25886, #32256, #20623, #42449, #19869, #66495, #59740, #65386, #37919, #20985, #48816, #25160, #2993, #26250, #60489, #14230, #72114, #71363, #8224, #55204, #43577, #30773, #60850, #9330, #26623, #42818, #31521, #49189, #65747, #37185, #3357, #36422, #66130, #60126, #72481, #54832, #48449, #43207, #8970, #14605, #43937, #66854, #54459, #59369, #8608, #71734, #7858, #53719, #2262, #20237, #31893, #2637, #48086, #31153, #70998, #13853, #54106, #36794, #25517, #37557, #27745, #44299, #22864, #39030, #11198, #45802, #15726, #10077, #56707, #28473, #27358, #5209, #61229, #10448, #50294, #73227, #15340, #21340, #22484, #67600, #39403, #26988, #62350, #4464, #34124, #38284, #51409, #33000, #45426, #21727, #72840, #45047, #28109, #68353, #55944, #44683, #16093, #56327, #61968, #50668, #33366, #16849, #4844, #73596, #22107, #67973, #16467, #9712, #39780, #10833, #5578, #51046, #33754, #62729, #73969, #57071, #67228, #54470, #32630, #55575, #4094, #49923, #38661, #61593, #51788, #58921, #24693, #6311, #57433, #337, #23230, #58532, #63825, #64192, #23965, #13031, #1445, #68725, #40143, #1807, #17210, #29214, #11554, #63097, #41614, #41253, #12666, #40889, #34490, #47266, #52152, #52516, #5950, #46901, #18671, #24330, #12298, #52904, #697, #69444, #70169, #7029, #28859, #23588, #18310, #34873, #35598, #40506, #29954, #64553, #63453, #35970, #46156, #1070, #6667, #69089, #17574, #17947, #7411, #11927, #57808, #46518, #30326, #53270, #35236, #58169, #29573, #69809, #59654, #31061, #3639, #53637, #54745, #25437, #71654, #59283, #20150, #36708, #43491, #55111, #60767, #42364, #3273, #54019, #30690, #2910, #37472, #26162, #65302, #2557, #13773, #14138, #8137, #60040, #48365, #49099, #71277, #31437, #19781, #37089, #42729, #41998, #72025, #65663 ) ),
 .UNSPECIFIED., .F., .F., .F. ) 
 B_SPLINE_SURFACE_WITH_KNOTS ( ( 2, 2 ),
 ( 3, 2, 2, 2, 2, 2, 2, 2, 2, 2, 2, 2, 2, 2, 2, 2, 2, 2, 2, 2, 2, 2, 2, 2, 2, 2, 2, 2, 2, 2, 2, 2, 2, 2, 2, 2, 2, 2, 2, 2, 2, 2, 2, 2, 2, 2, 2, 2, 2, 2, 2, 2, 2, 2, 2, 2, 2, 2, 2, 2, 2, 2, 2, 2, 2, 2, 2, 2, 2, 2, 2, 2, 2, 2, 2, 2, 2, 2, 2, 2, 2, 2, 2, 2, 2, 2, 2, 2, 2, 2, 2, 2, 2, 2, 2, 2, 2, 2, 2, 2, 2, 2, 2, 2, 2, 2, 2, 2, 2, 2, 2, 2, 2, 2, 2, 2, 2, 2, 2, 2, 2, 2, 2, 2, 2, 2, 2, 2, 2, 2, 2, 2, 2, 2, 2, 2, 2, 2, 2, 2, 2, 2, 2, 3 ),
 ( 0.000000000000000000, 1.000000000000000000 ),
 ( 0.000000000000000000, 0.006944444444444444059, 0.01388888888888888812, 0.02083333333333333218, 0.02777777777777777624, 0.03472222222222222376, 0.04166666666666666435, 0.04861111111111111188, 0.05555555555555555247, 0.06250000000000000000, 0.06944444444444444753, 0.07638888888888889506, 0.08333333333333332871, 0.09027777777777777624, 0.09722222222222222376, 0.1041666666666666713, 0.1111111111111111049, 0.1180555555555555525, 0.1250000000000000000, 0.1319444444444444475, 0.1388888888888888951, 0.1458333333333333426, 0.1527777777777777901, 0.1597222222222222099, 0.1666666666666666574, 0.1736111111111111049, 0.1805555555555555525, 0.1875000000000000000, 0.1944444444444444475, 0.2013888888888888951, 0.2083333333333333426, 0.2152777777777777901, 0.2222222222222222099, 0.2291666666666666574, 0.2361111111111111049, 0.2430555555555555525, 0.2500000000000000000, 0.2569444444444444198, 0.2638888888888888951, 0.2708333333333333148, 0.2777777777777777901, 0.2847222222222222099, 0.2916666666666666852, 0.2986111111111111049, 0.3055555555555555802, 0.3125000000000000000, 0.3194444444444444198, 0.3263888888888888951, 0.3333333333333333148, 0.3402777777777777901, 0.3472222222222222099, 0.3541666666666666852, 0.3611111111111111049, 0.3680555555555555802, 0.3750000000000000000, 0.3819444444444444198, 0.3888888888888888951, 0.3958333333333333148, 0.4027777777777777901, 0.4097222222222222099, 0.4166666666666666852, 0.4236111111111111049, 0.4305555555555555802, 0.4375000000000000000, 0.4444444444444444198, 0.4513888888888888951, 0.4583333333333333148, 0.4652777777777777901, 0.4722222222222222099, 0.4791666666666666852, 0.4861111111111111049, 0.4930555555555555802, 0.5000000000000000000, 0.5069444444444444198, 0.5138888888888888395, 0.5208333333333333703, 0.5277777777777777901, 0.5347222222222222099, 0.5416666666666666297, 0.5486111111111111605, 0.5555555555555555802, 0.5625000000000000000, 0.5694444444444444198, 0.5763888888888888395, 0.5833333333333333703, 0.5902777777777777901, 0.5972222222222222099, 0.6041666666666666297, 0.6111111111111111605, 0.6180555555555555802, 0.6250000000000000000, 0.6319444444444444198, 0.6388888888888888395, 0.6458333333333333703, 0.6527777777777777901, 0.6597222222222222099, 0.6666666666666666297, 0.6736111111111111605, 0.6805555555555555802, 0.6875000000000000000, 0.6944444444444444198, 0.7013888888888888395, 0.7083333333333333703, 0.7152777777777777901, 0.7222222222222222099, 0.7291666666666666297, 0.7361111111111111605, 0.7430555555555555802, 0.7500000000000000000, 0.7569444444444444198, 0.7638888888888888395, 0.7708333333333333703, 0.7777777777777777901, 0.7847222222222222099, 0.7916666666666666297, 0.7986111111111111605, 0.8055555555555555802, 0.8125000000000000000, 0.8194444444444444198, 0.8263888888888888395, 0.8333333333333333703, 0.8402777777777777901, 0.8472222222222222099, 0.8541666666666666297, 0.8611111111111111605, 0.8680555555555555802, 0.8750000000000000000, 0.8819444444444444198, 0.8888888888888888395, 0.8958333333333333703, 0.9027777777777777901, 0.9097222222222222099, 0.9166666666666666297, 0.9236111111111111605, 0.9305555555555555802, 0.9375000000000000000, 0.9444444444444444198, 0.9513888888888888395, 0.9583333333333333703, 0.9652777777777777901, 0.9722222222222222099, 0.9791666666666666297, 0.9842226772312639982, 0.9940649040035766104 ),
 .UNSPECIFIED. ) 
 GEOMETRIC_REPRESENTATION_ITEM ( )  RATIONAL_B_SPLINE_SURFACE ( (
 ( 1.000000000000000000, 0.8660254037844387076, 1.000000000000000000, 0.8660254037844387076, 1.000000000000000000, 0.8660254037844387076, 1.000000000000000000, 0.8660254037844387076, 1.000000000000000000, 0.8660254037844387076, 1.000000000000000000, 0.8660254037844387076, 1.000000000000000000, 0.8660254037844387076, 1.000000000000000000, 0.8660254037844387076, 1.000000000000000000, 0.8660254037844387076, 1.000000000000000000, 0.8660254037844387076, 1.000000000000000000, 0.8660254037844387076, 1.000000000000000000, 0.8660254037844387076, 1.000000000000000000, 0.8660254037844387076, 1.000000000000000000, 0.8660254037844387076, 1.000000000000000000, 0.8660254037844387076, 1.000000000000000000, 0.8660254037844387076, 1.000000000000000000, 0.8660254037844387076, 1.000000000000000000, 0.8660254037844387076, 1.000000000000000000, 0.8660254037844387076, 1.000000000000000000, 0.8660254037844387076, 1.000000000000000000, 0.8660254037844387076, 1.000000000000000000, 0.8660254037844387076, 1.000000000000000000, 0.8660254037844387076, 1.000000000000000000, 0.8660254037844387076, 1.000000000000000000, 0.8660254037844387076, 1.000000000000000000, 0.8660254037844387076, 1.000000000000000000, 0.8660254037844387076, 1.000000000000000000, 0.8660254037844387076, 1.000000000000000000, 0.8660254037844387076, 1.000000000000000000, 0.8660254037844387076, 1.000000000000000000, 0.8660254037844387076, 1.000000000000000000, 0.8660254037844387076, 1.000000000000000000, 0.8660254037844387076, 1.000000000000000000, 0.8660254037844387076, 1.000000000000000000, 0.8660254037844387076, 1.000000000000000000, 0.8660254037844387076, 1.000000000000000000, 0.8660254037844387076, 1.000000000000000000, 0.8660254037844387076, 1.000000000000000000, 0.8660254037844387076, 1.000000000000000000, 0.8660254037844387076, 1.000000000000000000, 0.8660254037844387076, 1.000000000000000000, 0.8660254037844387076, 1.000000000000000000, 0.8660254037844387076, 1.000000000000000000, 0.8660254037844387076, 1.000000000000000000, 0.8660254037844387076, 1.000000000000000000, 0.8660254037844387076, 1.000000000000000000, 0.8660254037844387076, 1.000000000000000000, 0.8660254037844387076, 1.000000000000000000, 0.8660254037844387076, 1.000000000000000000, 0.8660254037844387076, 1.000000000000000000, 0.8660254037844387076, 1.000000000000000000, 0.8660254037844387076, 1.000000000000000000, 0.8660254037844387076, 1.000000000000000000, 0.8660254037844387076, 1.000000000000000000, 0.8660254037844387076, 1.000000000000000000, 0.8660254037844387076, 1.000000000000000000, 0.8660254037844387076, 1.000000000000000000, 0.8660254037844387076, 1.000000000000000000, 0.8660254037844387076, 1.000000000000000000, 0.8660254037844387076, 1.000000000000000000, 0.8660254037844387076, 1.000000000000000000, 0.8660254037844387076, 1.000000000000000000, 0.8660254037844387076, 1.000000000000000000, 0.8660254037844387076, 1.000000000000000000, 0.8660254037844387076, 1.000000000000000000, 0.8660254037844387076, 1.000000000000000000, 0.8660254037844387076, 1.000000000000000000, 0.8660254037844387076, 1.000000000000000000, 0.8660254037844387076, 1.000000000000000000, 0.8660254037844387076, 1.000000000000000000, 0.8660254037844387076, 1.000000000000000000, 0.8660254037844387076, 1.000000000000000000, 0.8660254037844387076, 1.000000000000000000, 0.8660254037844387076, 1.000000000000000000, 0.8660254037844387076, 1.000000000000000000, 0.8660254037844387076, 1.000000000000000000, 0.8660254037844387076, 1.000000000000000000, 0.8660254037844387076, 1.000000000000000000, 0.8660254037844387076, 1.000000000000000000, 0.8660254037844387076, 1.000000000000000000, 0.8660254037844387076, 1.000000000000000000, 0.8660254037844387076, 1.000000000000000000, 0.8660254037844387076, 1.000000000000000000, 0.8660254037844387076, 1.000000000000000000, 0.8660254037844387076, 1.000000000000000000, 0.8660254037844387076, 1.000000000000000000, 0.8660254037844387076, 1.000000000000000000, 0.8660254037844387076, 1.000000000000000000, 0.8660254037844387076, 1.000000000000000000, 0.8660254037844387076, 1.000000000000000000, 0.8660254037844387076, 1.000000000000000000, 0.8660254037844387076, 1.000000000000000000, 0.8660254037844387076, 1.000000000000000000, 0.8660254037844387076, 1.000000000000000000, 0.8660254037844387076, 1.000000000000000000, 0.8660254037844387076, 1.000000000000000000, 0.8660254037844387076, 1.000000000000000000, 0.8660254037844387076, 1.000000000000000000, 0.8660254037844387076, 1.000000000000000000, 0.8660254037844387076, 1.000000000000000000, 0.8660254037844387076, 1.000000000000000000, 0.8660254037844387076, 1.000000000000000000, 0.8660254037844387076, 1.000000000000000000, 0.8660254037844387076, 1.000000000000000000, 0.8660254037844387076, 1.000000000000000000, 0.8660254037844387076, 1.000000000000000000, 0.8660254037844387076, 1.000000000000000000, 0.8660254037844387076, 1.000000000000000000, 0.8660254037844387076, 1.000000000000000000, 0.8660254037844387076, 1.000000000000000000, 0.8660254037844387076, 1.000000000000000000, 0.8660254037844387076, 1.000000000000000000, 0.8660254037844387076, 1.000000000000000000, 0.8660254037844387076, 1.000000000000000000, 0.8660254037844387076, 1.000000000000000000, 0.8660254037844387076, 1.000000000000000000, 0.8660254037844387076, 1.000000000000000000, 0.8660254037844387076, 1.000000000000000000, 0.8660254037844387076, 1.000000000000000000, 0.8660254037844387076, 1.000000000000000000, 0.8660254037844387076, 1.000000000000000000, 0.8660254037844387076, 1.000000000000000000, 0.8660254037844387076, 1.000000000000000000, 0.8660254037844387076, 1.000000000000000000, 0.8660254037844387076, 1.000000000000000000, 0.8660254037844387076, 1.000000000000000000, 0.8660254037844387076, 1.000000000000000000, 0.8660254037844387076, 1.000000000000000000, 0.8660254037844387076, 1.000000000000000000, 0.8660254037844387076, 1.000000000000000000, 0.8660254037844387076, 1.000000000000000000, 0.8660254037844387076, 1.000000000000000000, 0.8660254037844387076, 1.000000000000000000, 0.8660254037844387076, 1.000000000000000000, 0.8660254037844387076, 1.000000000000000000, 0.8660254037844387076, 1.000000000000000000, 0.8660254037844387076, 1.000000000000000000, 0.8660254037844387076, 1.000000000000000000, 0.8660254037844387076, 1.000000000000000000, 0.8660254037844387076, 1.000000000000000000, 0.8660254037844387076, 1.000000000000000000, 0.9024577157650908177, 0.9469497795711379062, 0.9469497795711379062, 0.9469497795711379062),
 ( 1.000000000000000000, 0.8660254037844387076, 1.000000000000000000, 0.8660254037844387076, 1.000000000000000000, 0.8660254037844387076, 1.000000000000000000, 0.8660254037844387076, 1.000000000000000000, 0.8660254037844387076, 1.000000000000000000, 0.8660254037844387076, 1.000000000000000000, 0.8660254037844387076, 1.000000000000000000, 0.8660254037844387076, 1.000000000000000000, 0.8660254037844387076, 1.000000000000000000, 0.8660254037844387076, 1.000000000000000000, 0.8660254037844387076, 1.000000000000000000, 0.8660254037844387076, 1.000000000000000000, 0.8660254037844387076, 1.000000000000000000, 0.8660254037844387076, 1.000000000000000000, 0.8660254037844387076, 1.000000000000000000, 0.8660254037844387076, 1.000000000000000000, 0.8660254037844387076, 1.000000000000000000, 0.8660254037844387076, 1.000000000000000000, 0.8660254037844387076, 1.000000000000000000, 0.8660254037844387076, 1.000000000000000000, 0.8660254037844387076, 1.000000000000000000, 0.8660254037844387076, 1.000000000000000000, 0.8660254037844387076, 1.000000000000000000, 0.8660254037844387076, 1.000000000000000000, 0.8660254037844387076, 1.000000000000000000, 0.8660254037844387076, 1.000000000000000000, 0.8660254037844387076, 1.000000000000000000, 0.8660254037844387076, 1.000000000000000000, 0.8660254037844387076, 1.000000000000000000, 0.8660254037844387076, 1.000000000000000000, 0.8660254037844387076, 1.000000000000000000, 0.8660254037844387076, 1.000000000000000000, 0.8660254037844387076, 1.000000000000000000, 0.8660254037844387076, 1.000000000000000000, 0.8660254037844387076, 1.000000000000000000, 0.8660254037844387076, 1.000000000000000000, 0.8660254037844387076, 1.000000000000000000, 0.8660254037844387076, 1.000000000000000000, 0.8660254037844387076, 1.000000000000000000, 0.8660254037844387076, 1.000000000000000000, 0.8660254037844387076, 1.000000000000000000, 0.8660254037844387076, 1.000000000000000000, 0.8660254037844387076, 1.000000000000000000, 0.8660254037844387076, 1.000000000000000000, 0.8660254037844387076, 1.000000000000000000, 0.8660254037844387076, 1.000000000000000000, 0.8660254037844387076, 1.000000000000000000, 0.8660254037844387076, 1.000000000000000000, 0.8660254037844387076, 1.000000000000000000, 0.8660254037844387076, 1.000000000000000000, 0.8660254037844387076, 1.000000000000000000, 0.8660254037844387076, 1.000000000000000000, 0.8660254037844387076, 1.000000000000000000, 0.8660254037844387076, 1.000000000000000000, 0.8660254037844387076, 1.000000000000000000, 0.8660254037844387076, 1.000000000000000000, 0.8660254037844387076, 1.000000000000000000, 0.8660254037844387076, 1.000000000000000000, 0.8660254037844387076, 1.000000000000000000, 0.8660254037844387076, 1.000000000000000000, 0.8660254037844387076, 1.000000000000000000, 0.8660254037844387076, 1.000000000000000000, 0.8660254037844387076, 1.000000000000000000, 0.8660254037844387076, 1.000000000000000000, 0.8660254037844387076, 1.000000000000000000, 0.8660254037844387076, 1.000000000000000000, 0.8660254037844387076, 1.000000000000000000, 0.8660254037844387076, 1.000000000000000000, 0.8660254037844387076, 1.000000000000000000, 0.8660254037844387076, 1.000000000000000000, 0.8660254037844387076, 1.000000000000000000, 0.8660254037844387076, 1.000000000000000000, 0.8660254037844387076, 1.000000000000000000, 0.8660254037844387076, 1.000000000000000000, 0.8660254037844387076, 1.000000000000000000, 0.8660254037844387076, 1.000000000000000000, 0.8660254037844387076, 1.000000000000000000, 0.8660254037844387076, 1.000000000000000000, 0.8660254037844387076, 1.000000000000000000, 0.8660254037844387076, 1.000000000000000000, 0.8660254037844387076, 1.000000000000000000, 0.8660254037844387076, 1.000000000000000000, 0.8660254037844387076, 1.000000000000000000, 0.8660254037844387076, 1.000000000000000000, 0.8660254037844387076, 1.000000000000000000, 0.8660254037844387076, 1.000000000000000000, 0.8660254037844387076, 1.000000000000000000, 0.8660254037844387076, 1.000000000000000000, 0.8660254037844387076, 1.000000000000000000, 0.8660254037844387076, 1.000000000000000000, 0.8660254037844387076, 1.000000000000000000, 0.8660254037844387076, 1.000000000000000000, 0.8660254037844387076, 1.000000000000000000, 0.8660254037844387076, 1.000000000000000000, 0.8660254037844387076, 1.000000000000000000, 0.8660254037844387076, 1.000000000000000000, 0.8660254037844387076, 1.000000000000000000, 0.8660254037844387076, 1.000000000000000000, 0.8660254037844387076, 1.000000000000000000, 0.8660254037844387076, 1.000000000000000000, 0.8660254037844387076, 1.000000000000000000, 0.8660254037844387076, 1.000000000000000000, 0.8660254037844387076, 1.000000000000000000, 0.8660254037844387076, 1.000000000000000000, 0.8660254037844387076, 1.000000000000000000, 0.8660254037844387076, 1.000000000000000000, 0.8660254037844387076, 1.000000000000000000, 0.8660254037844387076, 1.000000000000000000, 0.8660254037844387076, 1.000000000000000000, 0.8660254037844387076, 1.000000000000000000, 0.8660254037844387076, 1.000000000000000000, 0.8660254037844387076, 1.000000000000000000, 0.8660254037844387076, 1.000000000000000000, 0.8660254037844387076, 1.000000000000000000, 0.8660254037844387076, 1.000000000000000000, 0.8660254037844387076, 1.000000000000000000, 0.8660254037844387076, 1.000000000000000000, 0.8660254037844387076, 1.000000000000000000, 0.8660254037844387076, 1.000000000000000000, 0.8660254037844387076, 1.000000000000000000, 0.8660254037844387076, 1.000000000000000000, 0.8660254037844387076, 1.000000000000000000, 0.8660254037844387076, 1.000000000000000000, 0.8660254037844387076, 1.000000000000000000, 0.8660254037844387076, 1.000000000000000000, 0.8660254037844387076, 1.000000000000000000, 0.8660254037844387076, 1.000000000000000000, 0.8660254037844387076, 1.000000000000000000, 0.8660254037844387076, 1.000000000000000000, 0.8660254037844387076, 1.000000000000000000, 0.8660254037844387076, 1.000000000000000000, 0.8660254037844387076, 1.000000000000000000, 0.8660254037844387076, 1.000000000000000000, 0.8660254037844387076, 1.000000000000000000, 0.8660254037844387076, 1.000000000000000000, 0.8660254037844387076, 1.000000000000000000, 0.8660254037844387076, 1.000000000000000000, 0.8660254037844387076, 1.000000000000000000, 0.8660254037844387076, 1.000000000000000000, 0.8660254037844387076, 1.000000000000000000, 0.8660254037844387076, 1.000000000000000000, 0.9024577157650908177, 0.9469497795711379062, 0.9469497795711379062, 0.9469497795711379062) ) ) 
 REPRESENTATION_ITEM ( '' )  SURFACE ( )  );
#68338=CARTESIAN_POINT ( 'NONE',  ( 93.67500000000001137, -212.2949673200287179, 89.47083333333333144 ) ) ;
#68352=CARTESIAN_POINT ( 'NONE',  ( 97.64999999999997726, -211.5299782133524502, 78.27895833506762813 ) ) ;
#68353=CARTESIAN_POINT ( 'NONE',  ( 92.34999999999999432, 90.00000000000002842, 81.74500000000000455 ) ) ;
#68354=EDGE_CURVE ( 'NONE', #22408, #39802, #54623, .T. ) ;
#68356=DIRECTION ( 'NONE',  ( -0.000000000000000000, -0.000000000000000000, 1.000000000000000000 ) ) ;
#68361=CARTESIAN_POINT ( 'NONE',  ( -97.65000000000001990, 88.47002178664754979, 88.22729166840096582 ) ) ;
#68362=CARTESIAN_POINT ( 'NONE',  ( -97.30629616937501680, 91.33154071421968467, 82.12864583420048348 ) ) ;
#68363=CARTESIAN_POINT ( 'NONE',  ( 96.15314808468748708, 88.00268892867053694, 77.15447916753380753 ) ) ;
#68365=FACE_OUTER_BOUND ( 'NONE', #72210, .T. ) ;
#68367=DIRECTION ( 'NONE',  ( -0.8571673007021122226, 1.049727191138618572E-16, 0.5150380749100542666 ) ) ;
#68368=VECTOR ( 'NONE', #65414, 1000.000000000000000 ) ;
#68377=CARTESIAN_POINT ( 'NONE',  ( -97.30629616937497417, -211.3315407142195852, 76.99572916753380980 ) ) ;
#68384=CARTESIAN_POINT ( 'NONE',  ( 93.67499999999999716, 87.70503267997126784, 78.04083333333333883 ) ) ;
#68387=CARTESIAN_POINT ( 'NONE',  ( -92.69370383062498320, -211.3315407142195852, 77.20739583420046870 ) ) ;
#68389=CARTESIAN_POINT ( 'NONE',  ( -97.65000000000001990, 90.00000000000004263, 76.66499999999999204 ) ) ;
#68394=CARTESIAN_POINT ( 'NONE',  ( 93.84685191531248449, 91.99731107132950569, 85.09197916753380753 ) ) ;
#68408=CARTESIAN_POINT ( 'NONE',  ( -92.69370383062504004, 90.00000000000004263, 88.69031250086715090 ) ) ;
#68410=CARTESIAN_POINT ( 'NONE',  ( -92.34999999999999432, -208.4700217866474645, 83.38541666666667140 ) ) ;
#68423=CARTESIAN_POINT ( 'NONE',  ( 96.15314808468750130, -211.9973110713294489, 84.93322916753382401 ) ) ;
#68425=AXIS2_PLACEMENT_3D ( 'NONE', #9523, #14039, #59935 ) ;
#68431=CARTESIAN_POINT ( 'NONE',  ( 93.84685191531249870, -208.0026889286704943, 79.37697916753380412 ) ) ;
#68434=CARTESIAN_POINT ( 'NONE',  ( 92.69370383062501162, -208.6684592857803011, 84.66864583420047552 ) ) ;
#68436=CARTESIAN_POINT ( 'NONE',  ( 93.67499999999998295, 92.29496732002878900, 80.44854166840097776 ) ) ;
#68441=CARTESIAN_POINT ( 'NONE',  ( 92.35000000000002274, -208.4700217866474645, 86.21645833506764234 ) ) ;
#68452=ORIENTED_EDGE ( 'NONE', *, *, #74059, .F. ) ;
#68459=ORIENTED_EDGE ( 'NONE', *, *, #23834, .F. ) ;
#68462=CARTESIAN_POINT ( 'NONE',  ( -93.84685191531254134, 91.99731107132950569, 75.61989583420049144 ) ) ;
#68465=ORIENTED_EDGE ( 'NONE', *, *, #24514, .T. ) ;
#68467=CARTESIAN_POINT ( 'NONE',  ( -94.99999999999997158, -212.6630814284392557, 85.99156250086714692 ) ) ;
#68472=CARTESIAN_POINT ( 'NONE',  ( -92.69370383062498320, -209.9999999999999716, 75.99031250086714806 ) ) ;
#68476=CONICAL_SURFACE ( 'NONE', #37235, 2.649999999999999467, 1.029744258676654312 ) ;
#68482=LINE ( 'NONE', #16969, #41145 ) ;
#68484=CARTESIAN_POINT ( 'NONE',  ( -92.69370383062502583, 91.33154071421968467, 81.12322916753382174 ) ) ;
#68487=ORIENTED_EDGE ( 'NONE', *, *, #7586, .F. ) ;
#68490=CARTESIAN_POINT ( 'NONE',  ( 93.67500000000001137, -212.2949673200287179, 86.37520833506764006 ) ) ;
#68491=CARTESIAN_POINT ( 'NONE',  ( 95.04693102382874770, -212.6495843973424940, 75.00000002508419072 ) ) ;
#68494=CARTESIAN_POINT ( 'NONE',  ( -94.99999999999997158, -207.3369185715606307, 79.48281250086715488 ) ) ;
#68513=CARTESIAN_POINT ( 'NONE',  ( 97.30629616937498838, -209.9999999999999716, 87.42031250086714067 ) ) ;
#68515=ADVANCED_FACE ( 'NONE', ( #50200 ), #9248, .F. ) ;
#68520=CARTESIAN_POINT ( 'NONE',  ( 97.65000000000000568, -211.5299782133524218, 85.26395833506762756 ) ) ;
#68523=CARTESIAN_POINT ( 'NONE',  ( 97.65000000000000568, -211.5299782133524502, 82.00958333333333883 ) ) ;
#68524=AXIS2_PLACEMENT_3D ( 'NONE', #65410, #43594, #59389 ) ;
#68525=ORIENTED_EDGE ( 'NONE', *, *, #7793, .T. ) ;
#68533=ORIENTED_EDGE ( 'NONE', *, *, #12632, .T. ) ;
#68536=CARTESIAN_POINT ( 'NONE',  ( 93.67499999999999716, 87.70503267997126784, 88.83583333333334053 ) ) ;
#68538=CYLINDRICAL_SURFACE ( 'NONE', #12911, 2.649999999999985700 ) ;
#68539=ORIENTED_EDGE ( 'NONE', *, *, #51365, .F. ) ;
#68542=CARTESIAN_POINT ( 'NONE',  ( 97.30629616937498838, 90.00000000000002842, 83.61031250086713840 ) ) ;
#68544=CARTESIAN_POINT ( 'NONE',  ( 97.30629616937498838, -208.6684592857803011, 83.66322916753379957 ) ) ;
#68549=DIRECTION ( 'NONE',  ( 1.000000000000000000, 0.000000000000000000, 0.000000000000000000 ) ) ;
#68551=CARTESIAN_POINT ( 'NONE',  ( -93.84685191531247028, -211.9973110713294489, 89.21947916753380525 ) ) ;
#68552=CARTESIAN_POINT ( 'NONE',  ( -92.69370383062504004, 90.00000000000004263, 85.03906250086714635 ) ) ;
#68554=CARTESIAN_POINT ( 'NONE',  ( 92.69370383062498320, 88.66845928578037217, 83.98072916753380923 ) ) ;
#68555=CARTESIAN_POINT ( 'NONE',  ( -93.84685191531252713, 88.00268892867056536, 84.13947916753380696 ) ) ;
#68557=CARTESIAN_POINT ( 'NONE',  ( -97.65000000000001990, 90.00000000000004263, 88.09499999999999886 ) ) ;
#68561=CARTESIAN_POINT ( 'NONE',  ( -93.84685191531247028, -211.9973110713294489, 84.77447916753381207 ) ) ;
#68565=CARTESIAN_POINT ( 'NONE',  ( -97.64996030324549281, 88.46999886771563126, 88.86229325377451005 ) ) ;
#68569=ORIENTED_EDGE ( 'NONE', *, *, #40392, .F. ) ;
#68571=CARTESIAN_POINT ( 'NONE',  ( -93.67500000000003979, 87.70503267997129626, 77.51166666666665606 ) ) ;
#68572=CARTESIAN_POINT ( 'NONE',  ( 1.243286885786405054E-17, -120.0000000000000000, -85.60000000000000853 ) ) ;
#68575=CARTESIAN_POINT ( 'NONE',  ( 97.08316478178002740, -211.0005890871205736, 74.79348190356850523 ) ) ;
#68576=EDGE_CURVE ( 'NONE', #27263, #21733, #46949, .T. ) ;
#68577=CARTESIAN_POINT ( 'NONE',  ( -95.00000000000002842, 86.94004357329504273, 86.42812500173430124 ) ) ;
#68579=( BOUNDED_CURVE ( )  B_SPLINE_CURVE ( 2, ( #19091, #2218, #60445, #60084, #8180, #8562, #31481, #2595, #13079 ),
 .UNSPECIFIED., .F., .F. ) 
 B_SPLINE_CURVE_WITH_KNOTS ( ( 3, 2, 2, 2, 3 ),
 ( 0.8255245790564514907, 0.8325803338241195561, 0.8396360993650018312, 0.8466918649058843283, 0.8466920362367552633 ),
 .UNSPECIFIED. ) 
 CURVE ( )  GEOMETRIC_REPRESENTATION_ITEM ( )  RATIONAL_B_SPLINE_CURVE ( ( 1.000000000000000000, 0.8660254037844387076, 1.000000000000000000, 0.8660254037844387076, 1.000000000000000000, 0.8660254037844387076, 1.000000000000000000, 0.9999967467762187479, 0.9999934937104295596 ) ) 
 REPRESENTATION_ITEM ( '' )  );
#68581=CARTESIAN_POINT ( 'NONE',  ( -95.00000000000002842, 92.66308142843932671, 78.68906250086713783 ) ) ;
#68582=EDGE_CURVE ( 'NONE', #67171, #55390, #13198, .T. ) ;
#68591=CARTESIAN_POINT ( 'NONE',  ( -97.30629616937497417, -208.6684592857803011, 89.11364583420049712 ) ) ;
#68593=ADVANCED_FACE ( 'NONE', ( #67512 ), #34035, .F. ) ;
#68594=CARTESIAN_POINT ( 'NONE',  ( 92.69370383062498320, 91.33154071421968467, 76.41364583420049428 ) ) ;
#68595=CARTESIAN_POINT ( 'NONE',  ( -97.30629616937497417, -208.6684592857803295, 80.22364583420048234 ) ) ;
#68600=CARTESIAN_POINT ( 'NONE',  ( -97.64999999999996305, -209.9999999999999716, 90.00000000000000000 ) ) ;
#68603=CARTESIAN_POINT ( 'NONE',  ( 96.15314808468748708, -208.0026889286704943, 81.17614583420048291 ) ) ;
#68604=ORIENTED_EDGE ( 'NONE', *, *, #33775, .T. ) ;
#68609=ADVANCED_FACE ( 'NONE', ( #63014 ), #50960, .F. ) ;
#68612=DIRECTION ( 'NONE',  ( -1.000000000000000000, -1.343011723336883198E-16, -0.000000000000000000 ) ) ;
#68615=ORIENTED_EDGE ( 'NONE', *, *, #30213, .F. ) ;
#68617=ORIENTED_EDGE ( 'NONE', *, *, #23177, .F. ) ;
#68618=CARTESIAN_POINT ( 'NONE',  ( 97.30629616937498838, -211.3315407142195852, 76.09614583420048461 ) ) ;
#68625=CARTESIAN_POINT ( 'NONE',  ( 96.15314808468748708, 88.00268892867053694, 83.02822916753380866 ) ) ;
#68626=CARTESIAN_POINT ( 'NONE',  ( 96.32499999999998863, -212.2949673200287179, 79.41666666666665719 ) ) ;
#68628=EDGE_CURVE ( 'NONE', #17937, #48269, #21641, .T. ) ;
#68631=ORIENTED_EDGE ( 'NONE', *, *, #28534, .T. ) ;
#68633=CONICAL_SURFACE ( 'NONE', #42232, 2.649999999999999467, 1.029744258676654312 ) ;
#68634=CARTESIAN_POINT ( 'NONE',  ( -92.34999999999999432, -210.0000000024460576, 75.15687493084206494 ) ) ;
#68642=CARTESIAN_POINT ( 'NONE',  ( -97.64999999999994884, -208.4700217866474645, 82.40645833506762585 ) ) ;
#68646=CARTESIAN_POINT ( 'NONE',  ( 93.67499999999999716, 87.70503267997126784, 78.12020833506763040 ) ) ;
#68647=CARTESIAN_POINT ( 'NONE',  ( -95.00000000000002842, 86.94004357329504273, 80.71312500173431204 ) ) ;
#68649=CARTESIAN_POINT ( 'NONE',  ( 92.69370383062498320, 91.33154071421968467, 80.22364583420048234 ) ) ;
#68650=CARTESIAN_POINT ( 'NONE',  ( -92.34999999999999432, -209.9999999999999716, 86.50750000000000739 ) ) ;
#68663=CARTESIAN_POINT ( 'NONE',  ( -97.30629616937497417, -211.3315407142195852, 82.23447916753383424 ) ) ;
#68665=ORIENTED_EDGE ( 'NONE', *, *, #32246, .T. ) ;
#68668=EDGE_CURVE ( 'NONE', #64530, #769, #16000, .T. ) ;
#68674=CARTESIAN_POINT ( 'NONE',  ( 92.69370383062498320, 91.33154071421968467, 74.98489583420048632 ) ) ;
#68684=CARTESIAN_POINT ( 'NONE',  ( 93.84685191531248449, 88.00268892867053694, 87.36739583420049371 ) ) ;
#68685=CARTESIAN_POINT ( 'NONE',  ( -97.30629616937495996, -209.9999999999999716, 88.53156250086716739 ) ) ;
#68687=ORIENTED_EDGE ( 'NONE', *, *, #63403, .F. ) ;
#68689=CARTESIAN_POINT ( 'NONE',  ( -97.30629616937501680, 91.33154071421968467, 78.15989583420048348 ) ) ;
#68692=VECTOR ( 'NONE', #29820, 1000.000000000000000 ) ;
#68700=CARTESIAN_POINT ( 'NONE',  ( -93.67499999999998295, -207.7050326799711968, 84.70833333333332860 ) ) ;
#68703=CARTESIAN_POINT ( 'NONE',  ( 92.69370383062501162, -209.9999999999999716, 76.46656250086715545 ) ) ;
#68706=CARTESIAN_POINT ( 'NONE',  ( 93.84685191531251292, -211.9973110713294489, 85.46239583420047836 ) ) ;
#68713=CARTESIAN_POINT ( 'NONE',  ( 93.67500000000001137, -207.7050326799711968, 89.25916666666667254 ) ) ;
#68721=AXIS2_PLACEMENT_3D ( 'NONE', #41653, #58579, #2220 ) ;
#68723=CARTESIAN_POINT ( 'NONE',  ( 93.67499999999999716, 87.70503267997126784, 87.56583333333333030 ) ) ;
#68724=CARTESIAN_POINT ( 'NONE',  ( 96.32499999999998863, -207.7050326799711968, 77.16770833506762983 ) ) ;
#68725=CARTESIAN_POINT ( 'NONE',  ( 96.32499999999998863, 87.70503267997126784, 79.41666666666665719 ) ) ;
#68726=ORIENTED_EDGE ( 'NONE', *, *, #1312, .T. ) ;
#68732=CARTESIAN_POINT ( 'NONE',  ( 92.35000000019411459, 89.99998015682159291, 84.36502760998348549 ) ) ;
#68734=CARTESIAN_POINT ( 'NONE',  ( -92.69370383062505425, 91.33154071421968467, 81.91697916753383879 ) ) ;
#68735=CARTESIAN_POINT ( 'NONE',  ( 92.69370383062498320, 88.66845928578037217, 78.90072916753381094 ) ) ;
#68736=ORIENTED_EDGE ( 'NONE', *, *, #47473, .T. ) ;
#68737=DIRECTION ( 'NONE',  ( -0.000000000000000000, -0.000000000000000000, 1.000000000000000000 ) ) ;
#68740=CARTESIAN_POINT ( 'NONE',  ( -92.34999999999999432, -209.9999999999999716, 77.61749999999999261 ) ) ;
#68744=CARTESIAN_POINT ( 'NONE',  ( -92.69370383062498320, -209.9999999999999716, 78.53031250086714010 ) ) ;
#68749=CARTESIAN_POINT ( 'NONE',  ( -95.00000000000002842, 90.00000000000004263, 90.00000000000000000 ) ) ;
#68752=CARTESIAN_POINT ( 'NONE',  ( -96.15314808468747287, -208.0026889286704943, 76.20197916753380696 ) ) ;
#68757=CARTESIAN_POINT ( 'NONE',  ( 95.00000000000000000, -206.9400435732949575, 81.58624999999999261 ) ) ;
#68761=CARTESIAN_POINT ( 'NONE',  ( 92.35000000000000853, -208.4700217866474645, 86.21645833506764234 ) ) ;
#68762=CARTESIAN_POINT ( 'NONE',  ( 94.99999999999998579, 92.66308142843932671, 86.30906250086714238 ) ) ;
#68775=CARTESIAN_POINT ( 'NONE',  ( -95.00000000000002842, 87.33691857156074434, 89.16656250086712987 ) ) ;
#68780=CARTESIAN_POINT ( 'NONE',  ( 94.99999999999998579, 86.94004357329502852, 85.71374999999999034 ) ) ;
#68783=( BOUNDED_CURVE ( )  B_SPLINE_CURVE ( 2, ( #17442, #41122, #52766, #17076, #52012, #40369, #62967 ),
 .UNSPECIFIED., .F., .F. ) 
 B_SPLINE_CURVE_WITH_KNOTS ( ( 3, 2, 2, 3 ),
 ( 0.9101937466091533091, 0.9172495203147085219, 0.9243052858555913520, 0.9313609857393202462 ),
 .UNSPECIFIED. ) 
 CURVE ( )  GEOMETRIC_REPRESENTATION_ITEM ( )  RATIONAL_B_SPLINE_CURVE ( ( 1.000000000000000000, 0.8660254037844387076, 1.000000000000000000, 0.8660254037844387076, 1.000000000000000000, 0.8660266504798735943, 0.9999975066323323336 ) ) 
 REPRESENTATION_ITEM ( '' )  );
#68786=CYLINDRICAL_SURFACE ( 'NONE', #15525, 2.649999999999999467 ) ;
#68794=CARTESIAN_POINT ( 'NONE',  ( 96.15314808468750130, -211.9973110713294489, 84.29822916753381890 ) ) ;
#68800=CARTESIAN_POINT ( 'NONE',  ( 92.69370383062501162, -209.9999999999999716, 77.57781250086713953 ) ) ;
#68801=ORIENTED_EDGE ( 'NONE', *, *, #54402, .T. ) ;
#68802=CARTESIAN_POINT ( 'NONE',  ( 96.15314808468748708, -208.0026889286704943, 83.87489583420048689 ) ) ;
#68808=CARTESIAN_POINT ( 'NONE',  ( 92.35000000000000853, -209.9999999999999716, 80.47499999999999432 ) ) ;
#68810=CARTESIAN_POINT ( 'NONE',  ( 95.00000000000000000, -213.0599564267049857, 76.90312500173429555 ) ) ;
#68811=CARTESIAN_POINT ( 'NONE',  ( 97.64999999999997726, -211.5299782133524502, 87.80395833506763381 ) ) ;
#68820=CARTESIAN_POINT ( 'NONE',  ( -92.35000000018064270, -210.0000309433161476, 78.33187387208045038 ) ) ;
#68827=CYLINDRICAL_SURFACE ( 'NONE', #60163, 2.649999999999999467 ) ;
#68829=CARTESIAN_POINT ( 'NONE',  ( -92.35000000000005116, 91.52997821335253548, 86.56041666666665435 ) ) ;
#68832=EDGE_CURVE ( 'NONE', #33969, #73349, #10936, .T. ) ;
#68835=CARTESIAN_POINT ( 'NONE',  ( -92.69370383062498320, -211.3315407142195852, 87.36739583420047950 ) ) ;
#68841=CARTESIAN_POINT ( 'NONE',  ( -92.69370383062498320, -208.6684592857803295, 75.40822916753381833 ) ) ;
#68849=EDGE_CURVE ( 'NONE', #29023, #40438, #57049, .T. ) ;
#68853=CARTESIAN_POINT ( 'NONE',  ( -92.69370383062504004, 90.00000000000004263, 79.16531250086714522 ) ) ;
#68863=DIRECTION ( 'NONE',  ( -1.000000000000000000, 0.000000000000000000, 0.000000000000000000 ) ) ;
#68864=CARTESIAN_POINT ( 'NONE',  ( -97.30629616937497417, -208.6684592857803011, 75.77864583420048916 ) ) ;
#68876=ORIENTED_EDGE ( 'NONE', *, *, #21884, .T. ) ;
#68880=CARTESIAN_POINT ( 'NONE',  ( 97.30629616937498838, -209.9999999999999716, 88.69031250086715090 ) ) ;
#68883=ORIENTED_EDGE ( 'NONE', *, *, #41071, .T. ) ;
#68885=ORIENTED_EDGE ( 'NONE', *, *, #14572, .F. ) ;
#68903=CARTESIAN_POINT ( 'NONE',  ( 94.99999999999998579, 92.66308142843935514, 85.03906250086714635 ) ) ;
#68905=CARTESIAN_POINT ( 'NONE',  ( 95.00000000000000000, -207.3369185715606307, 80.59406250086715318 ) ) ;
#68907=DIRECTION ( 'NONE',  ( 0.000000000000000000, 0.000000000000000000, 1.000000000000000000 ) ) ;
#68914=CARTESIAN_POINT ( 'NONE',  ( -94.99999999999997158, -207.3369185715606307, 84.40406250086712703 ) ) ;
#68915=ADVANCED_FACE ( 'NONE', ( #22814 ), #56658, .F. ) ;
#68916=CARTESIAN_POINT ( 'NONE',  ( -92.69370383062504004, 90.00000000000004263, 81.86406250086714920 ) ) ;
#68918=VECTOR ( 'NONE', #20348, 1000.000000000000000 ) ;
#68919=CARTESIAN_POINT ( 'NONE',  ( 97.30629616937498838, 88.66845928578037217, 84.82739583420045903 ) ) ;
#68920=CARTESIAN_POINT ( 'NONE',  ( -92.69370383062502583, 88.66845928578038638, 86.09739583420048348 ) ) ;
#68926=CARTESIAN_POINT ( 'NONE',  ( -97.30629616937497417, -208.6684592857803295, 86.41489583420047893 ) ) ;
#68927=CARTESIAN_POINT ( 'NONE',  ( -97.64999999999996305, -209.9999999999999716, 81.74500000000000455 ) ) ;
#68928=ADVANCED_FACE ( 'NONE', ( #5526 ), #17160, .F. ) ;
#68932=CARTESIAN_POINT ( 'NONE',  ( 97.65000000000000568, 88.47002178664753558, 89.62958333333334338 ) ) ;
#68936=CARTESIAN_POINT ( 'NONE',  ( -95.00000000000002842, 93.05995642670501411, 79.68124999999999147 ) ) ;
#68937=CARTESIAN_POINT ( 'NONE',  ( 97.65000000000006253, -211.5299782133524502, 88.99458333333333826 ) ) ;
#68946=ORIENTED_EDGE ( 'NONE', *, *, #4506, .T. ) ;
#68947=CARTESIAN_POINT ( 'NONE',  ( -95.00000000000002842, 92.66308142843932671, 76.78406250086712248 ) ) ;
#68951=CARTESIAN_POINT ( 'NONE',  ( -93.33864827736697123, -211.6008015735577033, 74.79754476654878204 ) ) ;
#68953=CARTESIAN_POINT ( 'NONE',  ( -97.64999999980585699, -210.0000198431789897, 84.36502761000342332 ) ) ;
#68955=CARTESIAN_POINT ( 'NONE',  ( -96.15314808468745866, -211.9973110713294489, 89.27239583420049485 ) ) ;
#68958=CARTESIAN_POINT ( 'NONE',  ( 96.15314808468748708, 88.00268892867053694, 76.04322916753382344 ) ) ;
#68960=CARTESIAN_POINT ( 'NONE',  ( -96.15314808468747287, -208.0026889286704943, 80.17072916753382117 ) ) ;
#68963=CARTESIAN_POINT ( 'NONE',  ( 94.99999999999998579, 86.94004357329502852, 87.69812500173429726 ) ) ;
#68966=CARTESIAN_POINT ( 'NONE',  ( -93.84685191531254134, 91.99731107132950569, 76.25489583420049655 ) ) ;
#68967=CARTESIAN_POINT ( 'NONE',  ( 95.00000000000000000, -212.6630814284392557, 75.83156250086715033 ) ) ;
#68971=VERTEX_POINT ( 'NONE', #52853 ) ;
#68972=CARTESIAN_POINT ( 'NONE',  ( -92.34999999999999432, -210.0000000334413528, 87.85687500050293863 ) ) ;
#68978=VERTEX_POINT ( 'NONE', #12614 ) ;
#68979=CARTESIAN_POINT ( 'NONE',  ( -94.99999999999997158, -213.0599564267049857, 77.45874999999999488 ) ) ;
#68983=CARTESIAN_POINT ( 'NONE',  ( 97.30629616937498838, 90.00000000000002842, 83.13406250086715943 ) ) ;
#68986=CARTESIAN_POINT ( 'NONE',  ( 7.103376864691351012E-17, -120.0000000000000000, -64.00000000000000000 ) ) ;
#68990=ORIENTED_EDGE ( 'NONE', *, *, #60700, .F. ) ;
#68993=VECTOR ( 'NONE', #28526, 1000.000000000000000 ) ;
#68995=CARTESIAN_POINT ( 'NONE',  ( -93.67500000000003979, 87.70503267997129626, 87.67166666666666686 ) ) ;
#68999=ADVANCED_FACE ( 'NONE', ( #59604 ), #35186, .F. ) ;
#69003=CARTESIAN_POINT ( 'NONE',  ( -94.99999999999997158, -206.9400435732949575, 82.93562500173429441 ) ) ;
#69009=CARTESIAN_POINT ( 'NONE',  ( 93.67499999999998295, 92.29496732002878900, 79.81354166840095843 ) ) ;
#69010=CARTESIAN_POINT ( 'NONE',  ( -92.35000000000005116, 91.52997821335253548, 79.65479166840096070 ) ) ;
#69011=( BOUNDED_CURVE ( )  B_SPLINE_CURVE ( 2, ( #24934, #2049, #36215, #7286, #24572, #69692, #19293 ),
 .UNSPECIFIED., .F., .F. ) 
 B_SPLINE_CURVE_WITH_KNOTS ( ( 3, 2, 2, 3 ),
 ( 0.9166666666666662966, 0.9236111111111108274, 0.9305555555555551361, 0.9374999999999995559 ),
 .UNSPECIFIED. ) 
 CURVE ( )  GEOMETRIC_REPRESENTATION_ITEM ( )  RATIONAL_B_SPLINE_CURVE ( ( 1.000000000000006439, 0.8660254037844322683, 1.000000000000000000, 0.8660254037844387076, 1.000000000000000000, 0.8660254037844472563, 0.9999999999999914513 ) ) 
 REPRESENTATION_ITEM ( '' )  );
#69013=CARTESIAN_POINT ( 'NONE',  ( 97.30629616937498838, 90.00000000000002842, 81.22906250086715829 ) ) ;
#69014=FACE_OUTER_BOUND ( 'NONE', #57008, .T. ) ;
#69016=AXIS2_PLACEMENT_3D ( 'NONE', #1820, #69821, #52917 ) ;
#69021=CARTESIAN_POINT ( 'NONE',  ( -95.00000000000002842, 93.05995642670504253, 80.31624999999999659 ) ) ;
#69024=VERTEX_POINT ( 'NONE', #53967 ) ;
#69026=CYLINDRICAL_SURFACE ( 'NONE', #52847, 2.649999999999985700 ) ;
#69027=EDGE_CURVE ( 'NONE', #57825, #55546, #2504, .T. ) ;
#69029=DIRECTION ( 'NONE',  ( 1.000000000000000000, 0.000000000000000000, 0.000000000000000000 ) ) ;
#69030=CARTESIAN_POINT ( 'NONE',  ( -97.30629616937497417, -211.3315407142195852, 79.05947916753382287 ) ) ;
#69038=PLANE ( 'NONE',  #20126 ) ;
#69040=CARTESIAN_POINT ( 'NONE',  ( -2.500000000000020428, -90.00000000000000000, -310.0000000000000000 ) ) ;
#69045=LINE ( 'NONE', #16802, #2207 ) ;
#69046=EDGE_CURVE ( 'NONE', #35350, #58563, #46469, .T. ) ;
#69049=CARTESIAN_POINT ( 'NONE',  ( 97.30629616937498838, 91.33154071421968467, 86.36197916753383197 ) ) ;
#69050=CARTESIAN_POINT ( 'NONE',  ( -97.30629616937497417, -208.6684592857803295, 89.74864583420048803 ) ) ;
#69053=CARTESIAN_POINT ( 'NONE',  ( 95.00000000000000000, -213.0599564267049857, 83.25312500173430408 ) ) ;
#69054=CARTESIAN_POINT ( 'NONE',  ( -95.00000000000002842, 87.33691857156074434, 79.00656250086714749 ) ) ;
#69055=CONICAL_SURFACE ( 'NONE', #42587, 2.649999999999999467, 1.029744258676654312 ) ;
#69057=CARTESIAN_POINT ( 'NONE',  ( 92.69370383062501162, -209.9999999999999716, 89.00781250086714635 ) ) ;
#69064=CARTESIAN_POINT ( 'NONE',  ( 92.69370383062501162, -208.6684592857803011, 75.14364583420049826 ) ) ;
#69068=CARTESIAN_POINT ( 'NONE',  ( 97.30629616937498838, -211.3315407142195852, 80.54114583420049200 ) ) ;
#69070=CARTESIAN_POINT ( 'NONE',  ( 93.67499999999998295, 92.29496732002878900, 81.00416666666666288 ) ) ;
#69071=CARTESIAN_POINT ( 'NONE',  ( 92.35000000000006537, 91.52997821335256390, 82.96208333333332519 ) ) ;
#69074=CARTESIAN_POINT ( 'NONE',  ( 97.64999999999997726, -211.5299782133524502, 88.35958333333333314 ) ) ;
#69083=CARTESIAN_POINT ( 'NONE',  ( -96.15314808468751551, 88.00268892867056536, 88.63739583420048973 ) ) ;
#69087=CARTESIAN_POINT ( 'NONE',  ( 92.35000000000002274, -211.5299782133524502, 75.52729166840099140 ) ) ;
#69089=CARTESIAN_POINT ( 'NONE',  ( 93.67499999999999716, 87.70503267997126784, 77.40583333333331950 ) ) ;
#69092=EDGE_LOOP ( 'NONE', ( #11801, #49203, #4086, #13830 ) ) ;
#69094=ORIENTED_EDGE ( 'NONE', *, *, #58037, .F. ) ;
#69095=CARTESIAN_POINT ( 'NONE',  ( -97.65000000000001990, 91.52997821335253548, 88.75645833506762017 ) ) ;
#69097=CARTESIAN_POINT ( 'NONE',  ( -96.15314808468751551, 88.00268892867056536, 80.38239583420048007 ) ) ;
#69099=CARTESIAN_POINT ( 'NONE',  ( 94.99999999999998579, 92.66308142843935514, 89.00781250086716057 ) ) ;
#69104=CARTESIAN_POINT ( 'NONE',  ( 97.64999999999999147, -209.9999999999999716, 85.87249999999998806 ) ) ;
#69110=CARTESIAN_POINT ( 'NONE',  ( -92.69370383062498320, -209.9999999999999716, 77.26031250086714408 ) ) ;
#69118=CARTESIAN_POINT ( 'NONE',  ( 92.34999999999999432, 90.00000000000002842, 80.47499999999999432 ) ) ;
#69120=CARTESIAN_POINT ( 'NONE',  ( -96.15314808468747287, -208.0026889286704943, 75.56697916753381605 ) ) ;
#69122=CARTESIAN_POINT ( 'NONE',  ( -92.35000000000005116, 88.47002178664754979, 76.92958333333332632 ) ) ;
#69130=EDGE_CURVE ( 'NONE', #30791, #26258, #37038, .T. ) ;
#69132=CARTESIAN_POINT ( 'NONE',  ( 97.64999999999324132, -209.9999940177821713, 82.14187520865721126 ) ) ;
#69133=CARTESIAN_POINT ( 'NONE',  ( 92.69370383062498320, 90.00000000000002842, 86.46781250086714010 ) ) ;
#69136=DIRECTION ( 'NONE',  ( -1.000000000000000000, 3.061616997868382648E-16, 0.000000000000000000 ) ) ;
#69139=CARTESIAN_POINT ( 'NONE',  ( -92.35000000000005116, 91.52997821335253548, 84.09979166840098230 ) ) ;
#69154=VECTOR ( 'NONE', #55855, 1000.000000000000000 ) ;
#69155=CARTESIAN_POINT ( 'NONE',  ( 93.84685191531249870, -208.0026889286704943, 87.15572916753382060 ) ) ;
#69160=AXIS2_PLACEMENT_3D ( 'NONE', #27590, #34341, #21192 ) ;
#69165=CARTESIAN_POINT ( 'NONE',  ( 97.30629616937498838, -211.3315407142195852, 82.44614583420049314 ) ) ;
#69169=ORIENTED_EDGE ( 'NONE', *, *, #673, .T. ) ;
#69172=ADVANCED_FACE ( 'NONE', ( #21206 ), #71229, .F. ) ;
#69176=CARTESIAN_POINT ( 'NONE',  ( 92.35000000000002274, -211.5299782133524502, 88.22729166840096582 ) ) ;
#69184=ORIENTED_EDGE ( 'NONE', *, *, #72567, .F. ) ;
#69185=ORIENTED_EDGE ( 'NONE', *, *, #54649, .F. ) ;
#69189=VERTEX_POINT ( 'NONE', #37788 ) ;
#69191=CARTESIAN_POINT ( 'NONE',  ( 97.64999999999999147, -209.9999999999999716, 76.34749999999999659 ) ) ;
#69194=CARTESIAN_POINT ( 'NONE',  ( -95.00000000000002842, 93.05995642670501411, 87.93625000000000114 ) ) ;
#69196=CARTESIAN_POINT ( 'NONE',  ( 97.30629616937498838, 88.66845928578037217, 75.30239583420048177 ) ) ;
#69199=CARTESIAN_POINT ( 'NONE',  ( -93.84685191531248449, -208.0026889286704943, 85.62114583420046188 ) ) ;
#69209=AXIS2_PLACEMENT_3D ( 'NONE', #30882, #19608, #25627 ) ;
#69214=CARTESIAN_POINT ( 'NONE',  ( -95.00000000000002842, 87.33691857156074434, 79.64156250086713840 ) ) ;
#69219=( BOUNDED_CURVE ( )  B_SPLINE_CURVE ( 2, ( #26318, #19933, #14668, #54527, #30838, #59807, #66555 ),
 .UNSPECIFIED., .F., .F. ) 
 B_SPLINE_CURVE_WITH_KNOTS ( ( 3, 2, 2, 3 ),
 ( 0.5080151867253829279, 0.5150708844844119616, 0.5221266500252946807, 0.5291824299508934848 ),
 .UNSPECIFIED. ) 
 CURVE ( )  GEOMETRIC_REPRESENTATION_ITEM ( )  RATIONAL_B_SPLINE_CURVE ( ( 0.9999974259464248227, 0.8660266908235904060, 1.000000000000000000, 0.8660254037844387076, 1.000000000000000000, 0.8660254037844387076, 1.000000000000000000 ) ) 
 REPRESENTATION_ITEM ( '' )  );
#69221=CARTESIAN_POINT ( 'NONE',  ( -94.99999999999997158, -206.9400435732949575, 80.39562500173430237 ) ) ;
#69228=CARTESIAN_POINT ( 'NONE',  ( -94.99999999999997158, -212.6630814284392557, 75.99031250086716227 ) ) ;
#69235=CYLINDRICAL_SURFACE ( 'NONE', #3162, 2.649999999999985700 ) ;
#69240=CARTESIAN_POINT ( 'NONE',  ( 92.69370383062501162, -209.9999999999999716, 85.83281250086714920 ) ) ;
#69242=ORIENTED_EDGE ( 'NONE', *, *, #23834, .T. ) ;
#69246=VERTEX_POINT ( 'NONE', #27969 ) ;
#69247=CARTESIAN_POINT ( 'NONE',  ( 97.64999999999990621, -209.9999992849081139, 85.31687502647973531 ) ) ;
#69249=CARTESIAN_POINT ( 'NONE',  ( -97.30629616937501680, 88.66845928578038638, 80.32947916753381890 ) ) ;
#69264=ADVANCED_FACE ( 'NONE', ( #17075 ), #62966, .F. ) ;
#69266=ORIENTED_EDGE ( 'NONE', *, *, #15067, .F. ) ;
#69268=CARTESIAN_POINT ( 'NONE',  ( 97.30629616937498838, 88.66845928578037217, 86.09739583420048348 ) ) ;
#69270=CARTESIAN_POINT ( 'NONE',  ( 95.00000000000000000, -212.6630814284392557, 82.81656250086713555 ) ) ;
#69278=CARTESIAN_POINT ( 'NONE',  ( -94.99999999999997158, -212.6630814284392557, 82.81656250086713555 ) ) ;
#69281=CARTESIAN_POINT ( 'NONE',  ( -97.30629616937501680, 91.33154071421968467, 82.76364583420048859 ) ) ;
#69284=CARTESIAN_POINT ( 'NONE',  ( 96.15314808468748708, 88.00268892867053694, 83.50447916753381605 ) ) ;
#69285=ORIENTED_EDGE ( 'NONE', *, *, #39482, .F. ) ;
#69286=CARTESIAN_POINT ( 'NONE',  ( -96.32500000000001705, 87.70503267997129626, 78.75520833506763552 ) ) ;
#69288=DIRECTION ( 'NONE',  ( -0.000000000000000000, -0.000000000000000000, 1.000000000000000000 ) ) ;
#69290=CARTESIAN_POINT ( 'NONE',  ( -93.84685191531247028, -211.9973110713294489, 86.04447916753380809 ) ) ;
#69295=ORIENTED_EDGE ( 'NONE', *, *, #2417, .F. ) ;
#69297=CARTESIAN_POINT ( 'NONE',  ( -92.35000000000003695, 90.00000000000004263, 76.34749999999999659 ) ) ;
#69299=CARTESIAN_POINT ( 'NONE',  ( -94.00680085345840098, -207.8660161998918170, 74.81432998548487490 ) ) ;
#69305=CARTESIAN_POINT ( 'NONE',  ( -97.30629616937501680, 91.33154071421968467, 80.06489583420047040 ) ) ;
#69313=CARTESIAN_POINT ( 'NONE',  ( -94.99999999999997158, -207.3369185715606307, 85.19781250086714408 ) ) ;
#69315=CARTESIAN_POINT ( 'NONE',  ( 93.84685191531248449, 91.99731107132950569, 76.36072916753381890 ) ) ;
#69317=CARTESIAN_POINT ( 'NONE',  ( -92.69370383062498320, -209.9999999999999716, 80.59406250086715318 ) ) ;
#69320=CARTESIAN_POINT ( 'NONE',  ( -95.00000000000002842, 93.05995642670504253, 82.93562500173430863 ) ) ;
#69321=CARTESIAN_POINT ( 'NONE',  ( -94.99999999999997158, -206.9400435732949575, 75.23624999999999829 ) ) ;
#69324=CARTESIAN_POINT ( 'NONE',  ( -97.30629616937501680, 91.33154071421968467, 75.77864583420048916 ) ) ;
#69325=CARTESIAN_POINT ( 'NONE',  ( 97.30629616937498838, -209.9999999999999716, 78.53031250086714010 ) ) ;
#69329=CARTESIAN_POINT ( 'NONE',  ( -97.64999999999994884, 91.52997821335257811, 75.34208333333333485 ) ) ;
#69330=VERTEX_POINT ( 'NONE', #68953 ) ;
#69331=CARTESIAN_POINT ( 'NONE',  ( -93.67499999999998295, -207.7050326799711968, 87.96270833506763154 ) ) ;
#69332=VERTEX_POINT ( 'NONE', #34728 ) ;
#69334=CARTESIAN_POINT ( 'NONE',  ( -93.67500000000003979, 92.29496732002878900, 79.07270833506763097 ) ) ;
#69341=CARTESIAN_POINT ( 'NONE',  ( 92.69370383062498320, 90.00000000000002842, 83.45156250086715488 ) ) ;
#69346=ORIENTED_EDGE ( 'NONE', *, *, #64751, .T. ) ;
#69357=CARTESIAN_POINT ( 'NONE',  ( 97.64999999954044085, -209.9999506483753180, 87.22187670868780174 ) ) ;
#69360=ORIENTED_EDGE ( 'NONE', *, *, #65216, .T. ) ;
#69361=CARTESIAN_POINT ( 'NONE',  ( -93.67499999999998295, -212.2949673200287179, 80.76604166840097321 ) ) ;
#69362=EDGE_CURVE ( 'NONE', #13090, #15642, #56180, .T. ) ;
#69367=CARTESIAN_POINT ( 'NONE',  ( 92.34999999999999432, 88.47002178664753558, 79.97229166840095615 ) ) ;
#69368=CARTESIAN_POINT ( 'NONE',  ( -95.00000000000002842, 86.94004357329504273, 78.80812500173429669 ) ) ;
#69371=CARTESIAN_POINT ( 'NONE',  ( 96.15314808468748708, 88.00268892867053694, 80.48822916753381662 ) ) ;
#69372=CARTESIAN_POINT ( 'NONE',  ( -92.34999999999999432, -209.9999999999999716, 82.06250000000000000 ) ) ;
#69387=CARTESIAN_POINT ( 'NONE',  ( -92.69370383062498320, -209.9999999999999716, 76.14906250086716000 ) ) ;
#69392=CARTESIAN_POINT ( 'NONE',  ( 97.64999999999999147, -209.9999999999999716, 90.00000000000000000 ) ) ;
#69400=CARTESIAN_POINT ( 'NONE',  ( 94.99999999999998579, 92.66308142843932671, 88.37281250086715545 ) ) ;
#69407=CARTESIAN_POINT ( 'NONE',  ( -92.69370383062504004, 90.00000000000004263, 81.07031250086714635 ) ) ;
#69411=CARTESIAN_POINT ( 'NONE',  ( 97.30629616937498838, -208.6684592857803011, 88.74322916753379786 ) ) ;
#69412=EDGE_CURVE ( 'NONE', #10724, #65641, #67578, .T. ) ;
#69417=CYLINDRICAL_SURFACE ( 'NONE', #4569, 15.69999999999999929 ) ;
#69422=ORIENTED_EDGE ( 'NONE', *, *, #6000, .T. ) ;
#69425=CARTESIAN_POINT ( 'NONE',  ( 93.84685191531251292, -211.9973110713294489, 81.01739583420049939 ) ) ;
#69429=CARTESIAN_POINT ( 'NONE',  ( 93.67499999999998295, 92.29496732002878900, 82.90916666666666401 ) ) ;
#69430=( BOUNDED_CURVE ( )  B_SPLINE_CURVE ( 2, ( #72600, #21106, #63216, #51545, #34999, #39910, #47391, #47026, #57570 ),
 .UNSPECIFIED., .F., .F. ) 
 B_SPLINE_CURVE_WITH_KNOTS ( ( 3, 2, 2, 2, 3 ),
 ( 0.6138516023186938453, 0.6209073675976485296, 0.6279631331385309156, 0.6350188986794131907, 0.6350190250571090544 ),
 .UNSPECIFIED. ) 
 CURVE ( )  GEOMETRIC_REPRESENTATION_ITEM ( )  RATIONAL_B_SPLINE_CURVE ( ( 1.000000000000000000, 0.8660254037844387076, 1.000000000000000000, 0.8660254037844387076, 1.000000000000000000, 0.8660254037844387076, 1.000000000000000000, 0.9999976003453241447, 0.9999952007766099715 ) ) 
 REPRESENTATION_ITEM ( '' )  );
#69434=CARTESIAN_POINT ( 'NONE',  ( 97.64999999999997726, -211.5299782133524502, 84.54958333333333087 ) ) ;
#69440=CARTESIAN_POINT ( 'NONE',  ( -92.69370383062504004, 90.00000000000004263, 88.84906250086716284 ) ) ;
#69443=CARTESIAN_POINT ( 'NONE',  ( 97.64999999999999147, -209.9999999999999716, 77.06187500173429328 ) ) ;
#69444=CARTESIAN_POINT ( 'NONE',  ( 97.64999999999999147, 90.00000000000002842, 78.25249999999999773 ) ) ;
#69446=CARTESIAN_POINT ( 'NONE',  ( -92.34999999999999432, -211.5299782133524502, 88.43895833506762472 ) ) ;
#69452=CARTESIAN_POINT ( 'NONE',  ( -96.32500000000001705, 87.70503267997129626, 88.28020833506764120 ) ) ;
#69453=CARTESIAN_POINT ( 'NONE',  ( -95.00000000000002842, 92.66308142843932671, 82.02281250086714692 ) ) ;
#69455=CARTESIAN_POINT ( 'NONE',  ( 93.84685191531248449, 88.00268892867053694, 76.41364583420048007 ) ) ;
#69456=ORIENTED_EDGE ( 'NONE', *, *, #43202, .T. ) ;
#69459=VECTOR ( 'NONE', #64146, 1000.000000000000000 ) ;
#69460=CYLINDRICAL_SURFACE ( 'NONE', #25411, 2.649999999999985700 ) ;
#69462=CARTESIAN_POINT ( 'NONE',  ( -92.69370383062504004, 90.27617560457107970, 74.79348190356851944 ) ) ;
#69465=CARTESIAN_POINT ( 'NONE',  ( -93.84685191531247028, -211.9973110713294489, 76.51947916753380241 ) ) ;
#69471=VERTEX_POINT ( 'NONE', #561 ) ;
#69475=CARTESIAN_POINT ( 'NONE',  ( -93.84685191531247028, -211.9973110713294489, 87.47322916753381605 ) ) ;
#69480=VECTOR ( 'NONE', #70405, 1000.000000000000000 ) ;
#69481=VERTEX_POINT ( 'NONE', #13273 ) ;
#69485=CARTESIAN_POINT ( 'NONE',  ( 92.69370383062498320, 88.66845928578035796, 84.61572916753380014 ) ) ;
#69499=CARTESIAN_POINT ( 'NONE',  ( -96.15314808468751551, 88.00268892867056536, 89.11364583420048291 ) ) ;
#69513=CARTESIAN_POINT ( 'NONE',  ( 96.15314808468748708, -208.0026889286704943, 84.50989583420049200 ) ) ;
#69522=EDGE_CURVE ( 'NONE', #1800, #23675, #30189, .T. ) ;
#69524=CARTESIAN_POINT ( 'NONE',  ( 96.15314808468748708, -208.0026889286704943, 80.69989583420047552 ) ) ;
#69528=CARTESIAN_POINT ( 'NONE',  ( 97.64999999999999147, 90.00000000000002842, 79.52249999999999375 ) ) ;
#69537=ORIENTED_EDGE ( 'NONE', *, *, #9865, .F. ) ;
#69539=CARTESIAN_POINT ( 'NONE',  ( 97.64999999999997726, -208.4700217866474645, 87.90979166840095615 ) ) ;
#69547=CARTESIAN_POINT ( 'NONE',  ( 94.99999999999998579, 86.94004357329500010, 85.15812500173430521 ) ) ;
#69549=ORIENTED_EDGE ( 'NONE', *, *, #42139, .F. ) ;
#69551=CARTESIAN_POINT ( 'NONE',  ( -93.67499999999998295, -212.2949673200287179, 78.22604166840096696 ) ) ;
#69555=ORIENTED_EDGE ( 'NONE', *, *, #42130, .F. ) ;
#69556=CARTESIAN_POINT ( 'NONE',  ( 97.64999999999999147, 90.00000015433757028, 79.60187500750917877 ) ) ;
#69558=CARTESIAN_POINT ( 'NONE',  ( -92.35000000000005116, 91.52997821335253548, 88.46541666666665549 ) ) ;
#69560=CARTESIAN_POINT ( 'NONE',  ( 97.30629616937498838, 90.00000000000002842, 75.35531250086714294 ) ) ;
#69563=CARTESIAN_POINT ( 'NONE',  ( -96.15314808468747287, -208.0026889286704943, 84.45697916753380241 ) ) ;
#69568=CARTESIAN_POINT ( 'NONE',  ( 97.64999999999999147, 90.00000000000002842, 81.42749999999999488 ) ) ;
#69569=CARTESIAN_POINT ( 'NONE',  ( -94.99999999999997158, -212.6630814284392557, 77.73656250086713726 ) ) ;
#69576=DIRECTION ( 'NONE',  ( 1.000000000000000000, 0.000000000000000000, 0.000000000000000000 ) ) ;
#69579=CARTESIAN_POINT ( 'NONE',  ( -92.69370383062502583, 88.66845928578038638, 78.47739583420047893 ) ) ;
#69585=ADVANCED_FACE ( 'NONE', ( #66634 ), #19644, .F. ) ;
#69586=CARTESIAN_POINT ( 'NONE',  ( 96.32499999999998863, -207.7050326799711968, 89.23270833506762756 ) ) ;
#69593=CARTESIAN_POINT ( 'NONE',  ( -94.99999999999997158, -212.6630814284392557, 76.62531250086715318 ) ) ;
#69595=ADVANCED_FACE ( 'NONE', ( #20757 ), #20010, .F. ) ;
#69597=ADVANCED_FACE ( 'NONE', ( #43352 ), #2776, .F. ) ;
#69598=FACE_OUTER_BOUND ( 'NONE', #36088, .T. ) ;
#69610=CARTESIAN_POINT ( 'NONE',  ( 92.69370383062501162, -211.3315407142195852, 83.98072916753380923 ) ) ;
#69612=ORIENTED_EDGE ( 'NONE', *, *, #15255, .F. ) ;
#69621=CARTESIAN_POINT ( 'NONE',  ( -97.30629616937501680, 88.66845928578038638, 79.05947916753382287 ) ) ;
#69627=DIRECTION ( 'NONE',  ( -0.000000000000000000, -0.000000000000000000, -1.000000000000000000 ) ) ;
#69628=VERTEX_POINT ( 'NONE', #8003 ) ;
#69631=CARTESIAN_POINT ( 'NONE',  ( 93.67500000000001137, -212.2949673200287179, 80.66020833506763665 ) ) ;
#69632=ORIENTED_EDGE ( 'NONE', *, *, #33959, .T. ) ;
#69634=ORIENTED_EDGE ( 'NONE', *, *, #18280, .T. ) ;
#69635=ORIENTED_EDGE ( 'NONE', *, *, #4954, .T. ) ;
#69637=CARTESIAN_POINT ( 'NONE',  ( 93.84685191531249870, -208.0026889286704943, 81.28197916753380525 ) ) ;
#69640=CARTESIAN_POINT ( 'NONE',  ( -96.32500000000001705, 87.70503267997129626, 84.39083333333333314 ) ) ;
#69641=CARTESIAN_POINT ( 'NONE',  ( 97.64999999999997726, -208.4700217866474929, 78.94041666666664980 ) ) ;
#69642=DIRECTION ( 'NONE',  ( -2.628368902995175337E-16, -1.000000000000000000, 0.000000000000000000 ) ) ;
#69643=CARTESIAN_POINT ( 'NONE',  ( -97.64999999999997726, 88.47002178664750716, 79.25791666666667368 ) ) ;
#69647=CARTESIAN_POINT ( 'NONE',  ( -96.15314808468745866, -211.9973110713294489, 85.30364583420046642 ) ) ;
#69648=CARTESIAN_POINT ( 'NONE',  ( -92.69370383062504004, 90.00000000000004263, 83.76906250086716454 ) ) ;
#69650=CARTESIAN_POINT ( 'NONE',  ( 97.30629616937498838, 88.66845928578037217, 83.55739583420047722 ) ) ;
#69651=( BOUNDED_CURVE ( )  B_SPLINE_CURVE ( 2, ( #68091, #11310, #17327, #28226, #62850, #41010, #449 ),
 .UNSPECIFIED., .F., .F. ) 
 B_SPLINE_CURVE_WITH_KNOTS ( ( 3, 2, 2, 3 ),
 ( 0.1250000000000002220, 0.1319444444444446418, 0.1388888888888890338, 0.1458333333333334536 ),
 .UNSPECIFIED. ) 
 CURVE ( )  GEOMETRIC_REPRESENTATION_ITEM ( )  RATIONAL_B_SPLINE_CURVE ( ( 0.9999999999999956701, 0.8660254037844430375, 1.000000000000000000, 0.8660254037844387076, 1.000000000000000000, 0.8660254037844365982, 1.000000000000002220 ) ) 
 REPRESENTATION_ITEM ( '' )  );
#69657=CARTESIAN_POINT ( 'NONE',  ( 93.67499999999998295, 92.29496732002878900, 87.35416666666665719 ) ) ;
#69658=CARTESIAN_POINT ( 'NONE',  ( -97.30629616937495996, -209.9999999999999716, 85.19781250086714408 ) ) ;
#69663=CARTESIAN_POINT ( 'NONE',  ( 97.64999999999999147, -209.9999999999999716, 90.00000000000000000 ) ) ;
#69666=CARTESIAN_POINT ( 'NONE',  ( -96.32500000000001705, 87.70503267997129626, 76.77083333333332860 ) ) ;
#69668=CARTESIAN_POINT ( 'NONE',  ( -92.69370383062504004, 90.00000000000004263, 88.69031250086715090 ) ) ;
#69674=CARTESIAN_POINT ( 'NONE',  ( -92.69370383062502583, 88.66845928578038638, 79.11239583420046984 ) ) ;
#69675=LINE ( 'NONE', #12525, #33127 ) ;
#69683=CARTESIAN_POINT ( 'NONE',  ( -92.69370383062498320, -208.6684592857803011, 85.09197916753380753 ) ) ;
#69687=CARTESIAN_POINT ( 'NONE',  ( 94.99999999999998579, 87.33691857156068750, 75.99031250086716227 ) ) ;
#69688=CARTESIAN_POINT ( 'NONE',  ( -92.69370383062498320, -209.9999999999999716, 78.05406250086716113 ) ) ;
#69692=CARTESIAN_POINT ( 'NONE',  ( 97.64999999999989200, 91.52997821335259232, 75.76541666666668107 ) ) ;
#69693=FACE_OUTER_BOUND ( 'NONE', #31240, .T. ) ;
#69696=AXIS2_PLACEMENT_3D ( 'NONE', #41861, #31683, #3148 ) ;
#69698=CARTESIAN_POINT ( 'NONE',  ( 97.30629616937498838, -211.3315407142195852, 78.47739583420047893 ) ) ;
#69714=CARTESIAN_POINT ( 'NONE',  ( 93.84685191531248449, 91.99731107132950569, 83.34572916753383254 ) ) ;
#69715=CARTESIAN_POINT ( 'NONE',  ( -97.65000000000001990, 90.00000000000004263, 81.18937500173430521 ) ) ;
#69719=AXIS2_PLACEMENT_3D ( 'NONE', #36291, #18264, #35189 ) ;
#69725=CARTESIAN_POINT ( 'NONE',  ( -97.64999999999996305, -209.9999999999999716, 75.47437500173430180 ) ) ;
#69730=CARTESIAN_POINT ( 'NONE',  ( -92.34999999999999432, -211.5299782133524502, 77.64395833506762301 ) ) ;
#69734=CARTESIAN_POINT ( 'NONE',  ( 92.34999999999999432, 90.00000000000002842, 79.91937500173429498 ) ) ;
#69735=CARTESIAN_POINT ( 'NONE',  ( -95.00000000000002842, 86.94004357329504273, 77.53812500173428646 ) ) ;
#69737=CARTESIAN_POINT ( 'NONE',  ( 96.15314808468748708, 91.99731107132950569, 78.79489583420048859 ) ) ;
#69740=CARTESIAN_POINT ( 'NONE',  ( -96.32500000000001705, 92.29496732002878900, 86.79854166840097207 ) ) ;
#69756=CARTESIAN_POINT ( 'NONE',  ( -96.15314808468745866, -211.9973110713294489, 76.57239583420049200 ) ) ;
#69757=ORIENTED_EDGE ( 'NONE', *, *, #37718, .F. ) ;
#69769=LINE ( 'NONE', #47956, #69459 ) ;
#69771=CARTESIAN_POINT ( 'NONE',  ( 97.30629616937498838, 90.00000000000002842, 88.84906250086716284 ) ) ;
#69772=CARTESIAN_POINT ( 'NONE',  ( -94.99999999999997158, -212.6630814284392557, 88.05531250086714579 ) ) ;
#69773=CARTESIAN_POINT ( 'NONE',  ( 96.32499999999997442, 92.29496732002878900, 79.07270833506763097 ) ) ;
#69776=CARTESIAN_POINT ( 'NONE',  ( 97.64999999989935020, -209.9999769027737671, 83.41187580057901130 ) ) ;
#69777=CARTESIAN_POINT ( 'NONE',  ( -93.67499999999998295, -207.7050326799711968, 82.16833333333332234 ) ) ;
#69778=CARTESIAN_POINT ( 'NONE',  ( -93.84685191531254134, 91.99731107132950569, 77.36614583420046642 ) ) ;
#69779=CARTESIAN_POINT ( 'NONE',  ( 97.30629616937498838, -211.3315407142195852, 87.36739583420047950 ) ) ;
#69780=EDGE_CURVE ( 'NONE', #53082, #63185, #29151, .T. ) ;
#69783=CARTESIAN_POINT ( 'NONE',  ( 95.00000000000000000, -206.9400435732949575, 87.30124999999999602 ) ) ;
#69784=ORIENTED_EDGE ( 'NONE', *, *, #32978, .T. ) ;
#69787=AXIS2_PLACEMENT_3D ( 'NONE', #37859, #68183, #66434 ) ;
#69789=ORIENTED_EDGE ( 'NONE', *, *, #20864, .F. ) ;
#69790=AXIS2_PLACEMENT_3D ( 'NONE', #61184, #10040, #8932 ) ;
#69791=ORIENTED_EDGE ( 'NONE', *, *, #57126, .T. ) ;
#69792=CARTESIAN_POINT ( 'NONE',  ( 95.00000000000000000, -212.6630814284392557, 82.97531250086714749 ) ) ;
#69798=CARTESIAN_POINT ( 'NONE',  ( 96.32499999999998863, -212.2949673200287179, 86.40166666666667084 ) ) ;
#69805=CARTESIAN_POINT ( 'NONE',  ( -93.84685191531252713, 88.00268892867056536, 86.20322916753382003 ) ) ;
#69808=CARTESIAN_POINT ( 'NONE',  ( 92.35000000000000853, -209.9999999999999716, 74.83937500173429669 ) ) ;
#69809=CARTESIAN_POINT ( 'NONE',  ( 93.67499999999999716, 87.70503267997126784, 76.77083333333332860 ) ) ;
#69810=VERTEX_POINT ( 'NONE', #10585 ) ;
#69811=CARTESIAN_POINT ( 'NONE',  ( -97.64999999999996305, -209.9999999999999716, 88.17437500173430465 ) ) ;
#69813=VERTEX_POINT ( 'NONE', #62104 ) ;
#69815=ORIENTED_EDGE ( 'NONE', *, *, #65710, .T. ) ;
#69816=CARTESIAN_POINT ( 'NONE',  ( 93.67499999999999716, 87.70503267997126784, 84.47020833506762472 ) ) ;
#69817=CARTESIAN_POINT ( 'NONE',  ( 96.66077099052519372, 88.39973697852393286, 74.64190534806806454 ) ) ;
#69820=LINE ( 'NONE', #70545, #67426 ) ;
#69821=DIRECTION ( 'NONE',  ( -0.000000000000000000, -0.000000000000000000, 1.000000000000000000 ) ) ;
#69829=ORIENTED_EDGE ( 'NONE', *, *, #5639, .F. ) ;
#69835=CARTESIAN_POINT ( 'NONE',  ( -92.35000000000005116, 91.52997821335253548, 75.20979166840096752 ) ) ;
#69836=EDGE_LOOP ( 'NONE', ( #24323, #24761, #18752, #49650 ) ) ;
#69837=CARTESIAN_POINT ( 'NONE',  ( -96.15314808468747287, -208.0026889286704943, 89.06072916753382174 ) ) ;
#69847=CARTESIAN_POINT ( 'NONE',  ( 92.69370383062498320, 91.33154071421968467, 80.06489583420047040 ) ) ;
#69851=CARTESIAN_POINT ( 'NONE',  ( -92.35000000000003695, 90.00000000000004263, 85.23749999999999716 ) ) ;
#69856=( BOUNDED_CURVE ( )  B_SPLINE_CURVE ( 2, ( #41639, #48391, #58948, #53297, #47655, #70559, #7801 ),
 .UNSPECIFIED., .F., .F. ) 
 B_SPLINE_CURVE_WITH_KNOTS ( ( 3, 2, 2, 3 ),
 ( 0.4791666666666668517, 0.4861111111111112160, 0.4930555555555556357, 0.5000000000000000000 ),
 .UNSPECIFIED. ) 
 CURVE ( )  GEOMETRIC_REPRESENTATION_ITEM ( )  RATIONAL_B_SPLINE_CURVE ( ( 0.9999999999999967804, 0.8660254037844419273, 1.000000000000000000, 0.8660254037844387076, 1.000000000000000000, 0.8660254037844387076, 1.000000000000000000 ) ) 
 REPRESENTATION_ITEM ( '' )  );
#69860=CARTESIAN_POINT ( 'NONE',  ( -92.69370383062504004, 90.00000000000004263, 85.51531250086713953 ) ) ;
#69862=DIRECTION ( 'NONE',  ( -0.000000000000000000, -0.000000000000000000, 1.000000000000000000 ) ) ;
#69868=CARTESIAN_POINT ( 'NONE',  ( 93.67499999999998295, 92.29496732002878900, 85.44916666666665606 ) ) ;
#69869=CARTESIAN_POINT ( 'NONE',  ( 96.32499999999997442, 92.29496732002878900, 77.08833333333332405 ) ) ;
#69872=CARTESIAN_POINT ( 'NONE',  ( 92.69370383062501162, -209.9999999999999716, 81.54656250086715374 ) ) ;
#69882=CARTESIAN_POINT ( 'NONE',  ( 93.84685191531249870, -208.0026889286704943, 78.26572916753382003 ) ) ;
#69890=SURFACE_STYLE_USAGE ( .BOTH. , #12747 ) ;
#69894=CARTESIAN_POINT ( 'NONE',  ( 92.35000000000002274, -208.4700217866474645, 87.48645833506763836 ) ) ;
#69895=CARTESIAN_POINT ( 'NONE',  ( 92.34999999999999432, 88.47002178664753558, 88.14791666666666003 ) ) ;
#69904=CARTESIAN_POINT ( 'NONE',  ( 92.34999999999999432, 90.00000000000002842, 85.63437500173431260 ) ) ;
#69907=CARTESIAN_POINT ( 'NONE',  ( -2.499999999999965361, 90.00000000000000000, -90.00000000000000000 ) ) ;
#69911=ORIENTED_EDGE ( 'NONE', *, *, #42130, .T. ) ;
#69916=CARTESIAN_POINT ( 'NONE',  ( -97.65000000000001990, 90.00000000000004263, 87.45999999999999375 ) ) ;
#69917=EDGE_LOOP ( 'NONE', ( #38594, #4725, #27542, #16935 ) ) ;
#69922=CARTESIAN_POINT ( 'NONE',  ( -97.30629616937497417, -208.6684592857803011, 83.87489583420047268 ) ) ;
#69923=ORIENTED_EDGE ( 'NONE', *, *, #30282, .T. ) ;
#69927=CARTESIAN_POINT ( 'NONE',  ( -96.15314808468745866, -211.9973110713294489, 75.77864583420047495 ) ) ;
#69928=EDGE_CURVE ( 'NONE', #45497, #30067, #26293, .T. ) ;
#69936=CARTESIAN_POINT ( 'NONE',  ( -92.69370383062502583, 91.33154071421968467, 79.21822916753380639 ) ) ;
#69950=CARTESIAN_POINT ( 'NONE',  ( -96.32500000000001705, 92.29496732002878900, 87.43354166840096298 ) ) ;
#69951=CARTESIAN_POINT ( 'NONE',  ( -94.99999999999997158, -212.6630814284392557, 77.26031250086714408 ) ) ;
#69954=EDGE_LOOP ( 'NONE', ( #26324, #37984, #6049, #60661 ) ) ;
#69960=ORIENTED_EDGE ( 'NONE', *, *, #21387, .F. ) ;
#69964=CARTESIAN_POINT ( 'NONE',  ( 93.84685191531249870, -208.0026889286704943, 85.72697916753379843 ) ) ;
#69966=EDGE_LOOP ( 'NONE', ( #72085, #49397, #3178, #19216, #50765, #3645, #38886, #69456, #23972, #1368, #46695, #26588 ) ) ;
#69967=CARTESIAN_POINT ( 'NONE',  ( 95.00000000000000000, -207.3369185715606307, 89.00781250086716057 ) ) ;
#69972=CARTESIAN_POINT ( 'NONE',  ( -93.84685191531252713, 88.00268892867056536, 81.12322916753382174 ) ) ;
#69977=( BOUNDED_CURVE ( )  B_SPLINE_CURVE ( 2, ( #46350, #52724, #70360, #58360, #46722, #70739, #23781 ),
 .UNSPECIFIED., .F., .F. ) 
 B_SPLINE_CURVE_WITH_KNOTS ( ( 3, 2, 2, 3 ),
 ( 0.4791666666666668517, 0.4861111111111112160, 0.4930555555555556357, 0.5000000000000000000 ),
 .UNSPECIFIED. ) 
 CURVE ( )  GEOMETRIC_REPRESENTATION_ITEM ( )  RATIONAL_B_SPLINE_CURVE ( ( 0.9999999999999967804, 0.8660254037844419273, 1.000000000000000000, 0.8660254037844387076, 1.000000000000000000, 0.8660254037844387076, 1.000000000000000000 ) ) 
 REPRESENTATION_ITEM ( '' )  );
#69980=DIRECTION ( 'NONE',  ( 1.000000000000000000, 0.000000000000000000, 0.000000000000000000 ) ) ;
#69990=ORIENTED_EDGE ( 'NONE', *, *, #58583, .T. ) ;
#69991=CARTESIAN_POINT ( 'NONE',  ( 92.69370383062501162, -209.9999999999999716, 83.29281250086714294 ) ) ;
#69997=CARTESIAN_POINT ( 'NONE',  ( 2.499999999999984457, -73.00000000000001421, -255.0000000000000000 ) ) ;
#70001=CARTESIAN_POINT ( 'NONE',  ( -97.30629616937495996, -209.9999999999999716, 83.92781250086714806 ) ) ;
#70002=CARTESIAN_POINT ( 'NONE',  ( -95.00000000000002842, 87.33691857156074434, 82.34031250086714238 ) ) ;
#70004=CARTESIAN_POINT ( 'NONE',  ( 94.99999999999998579, 87.33691857156068750, 81.54656250086715374 ) ) ;
#70012=CARTESIAN_POINT ( 'NONE',  ( -96.15314808468745866, -211.9973110713294489, 85.30364583420046642 ) ) ;
#70016=CARTESIAN_POINT ( 'NONE',  ( 97.64999999999999147, -209.9999999999999716, 84.60249999999999204 ) ) ;
#70017=ORIENTED_EDGE ( 'NONE', *, *, #45772, .T. ) ;
#70021=CARTESIAN_POINT ( 'NONE',  ( -95.00000000000002842, 87.33691857156074434, 87.89656250086713385 ) ) ;
#70029=CARTESIAN_POINT ( 'NONE',  ( -96.15314808468752972, 91.99731107132950569, 76.20197916753380696 ) ) ;
#70031=ADVANCED_FACE ( 'NONE', ( #38995 ), #7911, .T. ) ;
#70033=CARTESIAN_POINT ( 'NONE',  ( 92.48632958231168288, -210.0000000000000284, 74.91808492278046572 ) ) ;
#70038=CARTESIAN_POINT ( 'NONE',  ( -92.69370383062498320, -208.6684592857803011, 85.72697916753381264 ) ) ;
#70044=CARTESIAN_POINT ( 'NONE',  ( 96.15314808468748708, 88.00268892867053694, 75.40822916753381833 ) ) ;
#70045=CARTESIAN_POINT ( 'NONE',  ( -96.15314808468747287, -208.0026889286704943, 75.09072916753380866 ) ) ;
#70047=EDGE_LOOP ( 'NONE', ( #62803, #912, #29288, #1239 ) ) ;
#70050=DIRECTION ( 'NONE',  ( 1.000000000000000000, 0.000000000000000000, 0.000000000000000000 ) ) ;
#70052=AXIS2_PLACEMENT_3D ( 'NONE', #60898, #9016, #4142 ) ;
#70053=AXIS2_PLACEMENT_3D ( 'NONE', #3683, #49514, #32587 ) ;
#70054=CARTESIAN_POINT ( 'NONE',  ( -93.84685191531254134, 91.99731107132950569, 74.98489583420048632 ) ) ;
#70055=CARTESIAN_POINT ( 'NONE',  ( 97.30629616937498838, -211.3315407142195852, 76.57239583420046358 ) ) ;
#70062=CARTESIAN_POINT ( 'NONE',  ( -92.35000000000547971, -210.0000054026037049, 81.50687481489497088 ) ) ;
#70066=CARTESIAN_POINT ( 'NONE',  ( 92.35000000021534561, -209.9999789922616458, 79.91868729553134187 ) ) ;
#70067=VERTEX_POINT ( 'NONE', #14290 ) ;
#70070=( BOUNDED_CURVE ( )  B_SPLINE_CURVE ( 2, ( #23158, #62652, #38961, #5504, #17503, #4768, #22791 ),
 .UNSPECIFIED., .F., .F. ) 
 B_SPLINE_CURVE_WITH_KNOTS ( ( 3, 2, 2, 3 ),
 ( 0.5080151867253831499, 0.5150708844844119616, 0.5221266500252946807, 0.5291824299508944840 ),
 .UNSPECIFIED. ) 
 CURVE ( )  GEOMETRIC_REPRESENTATION_ITEM ( )  RATIONAL_B_SPLINE_CURVE ( ( 0.9999974259464162740, 0.8660266908235946248, 1.000000000000000000, 0.8660254037844387076, 1.000000000000000000, 0.8660254037844387076, 1.000000000000000000 ) ) 
 REPRESENTATION_ITEM ( '' )  );
#70071=CARTESIAN_POINT ( 'NONE',  ( 92.69370383062498320, 91.33154071421968467, 80.85864583420048746 ) ) ;
#70073=LINE ( 'NONE', #12571, #59678 ) ;
#70089=CARTESIAN_POINT ( 'NONE',  ( -92.34999999999999432, -208.4700217866474645, 78.38479166840096468 ) ) ;
#70090=EDGE_LOOP ( 'NONE', ( #57061, #30319, #35746, #61062 ) ) ;
#70093=CARTESIAN_POINT ( 'NONE',  ( 97.64999999999997726, 88.47002178664753558, 80.81895833506764859 ) ) ;
#70094=CARTESIAN_POINT ( 'NONE',  ( -93.67500000000003979, 92.29496732002878900, 75.26270833506764291 ) ) ;
#70097=CARTESIAN_POINT ( 'NONE',  ( 96.15314808468748708, 91.99731107132950569, 80.69989583420047552 ) ) ;
#70099=LINE ( 'NONE', #18600, #44566 ) ;
#70103=ORIENTED_EDGE ( 'NONE', *, *, #19503, .T. ) ;
#70111=EDGE_CURVE ( 'NONE', #65017, #51207, #62323, .T. ) ;
#70115=CARTESIAN_POINT ( 'NONE',  ( -97.30629616937497417, -208.6684592857803011, 77.68364583420047609 ) ) ;
#70116=ORIENTED_EDGE ( 'NONE', *, *, #27410, .F. ) ;
#70128=CARTESIAN_POINT ( 'NONE',  ( -97.64999999999986358, -211.5299782133524502, 76.08291666666664810 ) ) ;
#70129=LINE ( 'NONE', #63783, #65816 ) ;
#70131=CARTESIAN_POINT ( 'NONE',  ( 93.84685191531248449, 88.00268892867053694, 88.00239583420048461 ) ) ;
#70132=CARTESIAN_POINT ( 'NONE',  ( -97.30629616937497417, -211.3315407142195852, 85.40947916753381719 ) ) ;
#70133=CARTESIAN_POINT ( 'NONE',  ( 92.35000000007821086, 90.00001303125209517, 79.28395951162845279 ) ) ;
#70135=CARTESIAN_POINT ( 'NONE',  ( 93.67500000000001137, -212.2949673200287179, 83.20020833506764291 ) ) ;
#70136=CARTESIAN_POINT ( 'NONE',  ( -94.99999999999997158, -213.0599564267049857, 82.53874999999999318 ) ) ;
#70137=CARTESIAN_POINT ( 'NONE',  ( -92.69370383062505425, 91.33154071421968467, 76.04322916753380923 ) ) ;
#70139=CARTESIAN_POINT ( 'NONE',  ( 95.00000000000000000, -207.3369185715606307, 88.84906250086713442 ) ) ;
#70148=ORIENTED_EDGE ( 'NONE', *, *, #35715, .F. ) ;
#70150=CARTESIAN_POINT ( 'NONE',  ( 93.84685191531251292, -211.9973110713294489, 81.65239583420049030 ) ) ;
#70152=DIRECTION ( 'NONE',  ( 1.000000000000000000, 0.000000000000000000, 0.000000000000000000 ) ) ;
#70157=CARTESIAN_POINT ( 'NONE',  ( 92.35000000000002274, -211.5299782133524502, 84.33791666666667197 ) ) ;
#70163=CARTESIAN_POINT ( 'NONE',  ( 99.99999999999998579, 80.00000000000000000, -90.00000000000000000 ) ) ;
#70164=CARTESIAN_POINT ( 'NONE',  ( -97.30629616937501680, 91.33154071421968467, 89.11364583420049712 ) ) ;
#70167=CARTESIAN_POINT ( 'NONE',  ( 97.64999999999999147, -209.9999999999999716, 78.33187500173430351 ) ) ;
#70168=CARTESIAN_POINT ( 'NONE',  ( 92.69370383062501162, -209.9999999999999716, 87.73781250086713612 ) ) ;
#70169=CARTESIAN_POINT ( 'NONE',  ( 97.64999999999997726, 88.47002178664753558, 78.19958333333332234 ) ) ;
#70172=CARTESIAN_POINT ( 'NONE',  ( -97.64999999999994884, -208.4700217866474645, 88.75645833506762017 ) ) ;
#70174=CARTESIAN_POINT ( 'NONE',  ( 95.00000000000000000, -213.0599564267049857, 79.99874999999998693 ) ) ;
#70176=CARTESIAN_POINT ( 'NONE',  ( -97.65000000000001990, 91.52997821335253548, 86.21645833506764234 ) ) ;
#70178=CARTESIAN_POINT ( 'NONE',  ( 93.84685191531248449, 91.99731107132950569, 75.56697916753381605 ) ) ;
#70183=DIRECTION ( 'NONE',  ( 1.000000000000000000, 0.000000000000000000, 0.000000000000000000 ) ) ;
#70186=CARTESIAN_POINT ( 'NONE',  ( -96.32500000000001705, 92.29496732002878900, 81.71854166840095957 ) ) ;
#70188=ORIENTED_EDGE ( 'NONE', *, *, #32172, .F. ) ;
#70196=CARTESIAN_POINT ( 'NONE',  ( -94.99999999999997158, -207.3369185715606307, 89.00781250086716057 ) ) ;
#70199=CARTESIAN_POINT ( 'NONE',  ( 94.99999999999998579, 90.00000000000002842, 90.00000000000000000 ) ) ;
#70202=ORIENTED_EDGE ( 'NONE', *, *, #40937, .F. ) ;
#70206=CARTESIAN_POINT ( 'NONE',  ( 96.15314808468748708, 91.99731107132950569, 81.81114583420047381 ) ) ;
#70209=CARTESIAN_POINT ( 'NONE',  ( -92.35000000000003695, 90.00000000000004263, 80.79249999999998977 ) ) ;
#70213=CARTESIAN_POINT ( 'NONE',  ( 97.65000000000006253, 88.47002178664756400, 83.91458333333333997 ) ) ;
#70217=CARTESIAN_POINT ( 'NONE',  ( -92.69370383062505425, 91.33154071421968467, 84.93322916753379559 ) ) ;
#70218=LINE ( 'NONE', #20203, #11914 ) ;
#70220=CYLINDRICAL_SURFACE ( 'NONE', #18029, 2.649999999999985700 ) ;
#70228=CARTESIAN_POINT ( 'NONE',  ( 95.00000000000000000, -212.6630814284392557, 81.70531250086715147 ) ) ;
#70230=EDGE_CURVE ( 'NONE', #2928, #42628, #21448, .T. ) ;
#70234=EDGE_LOOP ( 'NONE', ( #41226, #26895, #19596, #20989 ) ) ;
#70240=CARTESIAN_POINT ( 'NONE',  ( 96.15314808468750130, -211.9973110713294489, 77.94822916753382458 ) ) ;
#70248=( NAMED_UNIT ( * ) PLANE_ANGLE_UNIT ( ) SI_UNIT ( $, .RADIAN. ) );
#70250=VERTEX_POINT ( 'NONE', #20764 ) ;
#70251=CARTESIAN_POINT ( 'NONE',  ( -97.65000000000001990, 90.00000000000004263, 84.28499999999999659 ) ) ;
#70252=CARTESIAN_POINT ( 'NONE',  ( 92.35000000000000853, -209.9999999999999716, 83.09437500173430635 ) ) ;
#70253=CARTESIAN_POINT ( 'NONE',  ( 94.99999999999998579, 93.05995642670504253, 89.84125000000000227 ) ) ;
#70258=VERTEX_POINT ( 'NONE', #9117 ) ;
#70263=CARTESIAN_POINT ( 'NONE',  ( 93.67499999999999716, 87.70503267997126784, 85.74020833506763495 ) ) ;
#70272=CARTESIAN_POINT ( 'NONE',  ( 92.34999999999999432, 90.00000000000002842, 81.74500000000000455 ) ) ;
#70273=CARTESIAN_POINT ( 'NONE',  ( -96.32500000000001705, 92.29496732002878900, 86.71916666666666629 ) ) ;
#70274=EDGE_CURVE ( 'NONE', #52806, #74080, #59903, .T. ) ;
#70278=( BOUNDED_CURVE ( )  B_SPLINE_CURVE ( 2, ( #43582, #73231, #42821, #61235, #66498, #27362, #14980 ),
 .UNSPECIFIED., .F., .T. ) 
 B_SPLINE_CURVE_WITH_KNOTS ( ( 3, 2, 2, 3 ),
 ( 0.5503499107226623721, 0.5574054777297072771, 0.5644612432705895522, 0.5715170088666294834 ),
 .UNSPECIFIED. ) 
 CURVE ( )  GEOMETRIC_REPRESENTATION_ITEM ( )  RATIONAL_B_SPLINE_CURVE ( ( 0.9999924607068793048, 0.8660291735370716504, 1.000000000000000000, 0.8660254037844387076, 1.000000000000000000, 0.8660254037844387076, 1.000000000000000000 ) ) 
 REPRESENTATION_ITEM ( '' )  );
#70282=CARTESIAN_POINT ( 'NONE',  ( -97.30629616937495996, -209.9999999999999716, 82.02281250086714692 ) ) ;
#70285=DIRECTION ( 'NONE',  ( -1.000000000000000000, 0.000000000000000000, 0.000000000000000000 ) ) ;
#70287=CARTESIAN_POINT ( 'NONE',  ( 96.32499999999997442, 92.29496732002878900, 89.23270833506762756 ) ) ;
#70295=CARTESIAN_POINT ( 'NONE',  ( -97.30629616937501680, 88.66845928578038638, 78.26572916753380582 ) ) ;
#70296=FACE_OUTER_BOUND ( 'NONE', #6566, .T. ) ;
#70298=( BOUNDED_CURVE ( )  B_SPLINE_CURVE ( 2, ( #45564, #62487, #5709, #6085, #22995, #62865, #63594, #57577, #28985 ),
 .UNSPECIFIED., .F., .F. ) 
 B_SPLINE_CURVE_WITH_KNOTS ( ( 3, 2, 2, 2, 3 ),
 ( 0.6561861948910822084, 0.6632419608429419577, 0.6702977263838236777, 0.6773534919247052866, 0.6773535682752295228 ),
 .UNSPECIFIED. ) 
 CURVE ( )  GEOMETRIC_REPRESENTATION_ITEM ( )  RATIONAL_B_SPLINE_CURVE ( ( 1.000000000000000000, 0.8660254037844387076, 1.000000000000000000, 0.8660254037844387076, 1.000000000000000000, 0.8660254037844387076, 1.000000000000000000, 0.9999985502592750874, 0.9999971005499255217 ) ) 
 REPRESENTATION_ITEM ( '' )  );
#70299=VECTOR ( 'NONE', #51716, 1000.000000000000000 ) ;
#70305=CARTESIAN_POINT ( 'NONE',  ( 97.65000000000000568, -211.5299782133524218, 75.10395833506764518 ) ) ;
#70308=CARTESIAN_POINT ( 'NONE',  ( -95.73425683495054272, -214.0859151322042067, 74.64692065633565221 ) ) ;
#70310=DIRECTION ( 'NONE',  ( 1.000000000000000000, 0.000000000000000000, 0.000000000000000000 ) ) ;
#70325=ORIENTED_EDGE ( 'NONE', *, *, #61110, .F. ) ;
#70326=CARTESIAN_POINT ( 'NONE',  ( 92.69370383062501162, -209.9999999999999716, 84.56281250086713897 ) ) ;
#70327=CARTESIAN_POINT ( 'NONE',  ( 97.30629616937498838, -208.6684592857803295, 88.90197916753382401 ) ) ;
#70329=CARTESIAN_POINT ( 'NONE',  ( 93.84685191531251292, -211.9973110713294489, 88.63739583420048973 ) ) ;
#70331=ORIENTED_EDGE ( 'NONE', *, *, #72209, .F. ) ;
#70333=ORIENTED_EDGE ( 'NONE', *, *, #18182, .T. ) ;
#70334=CARTESIAN_POINT ( 'NONE',  ( -97.30629616937501680, 91.33154071421968467, 81.49364583420047836 ) ) ;
#70337=CARTESIAN_POINT ( 'NONE',  ( -97.64999999999996305, -211.5299782133524218, 87.59229166840096070 ) ) ;
#70349=ORIENTED_EDGE ( 'NONE', *, *, #65557, .F. ) ;
#70350=CARTESIAN_POINT ( 'NONE',  ( 92.69370383062501162, -208.6684592857803011, 81.33489583420048064 ) ) ;
#70360=CARTESIAN_POINT ( 'NONE',  ( -93.67500000000003979, 87.70503267997129626, 82.59166666666665435 ) ) ;
#70361=CARTESIAN_POINT ( 'NONE',  ( -97.30629616937497417, -208.6684592857803011, 84.50989583420046358 ) ) ;
#70362=CARTESIAN_POINT ( 'NONE',  ( -92.69370383062502583, 88.66845928578038638, 83.71614583420050337 ) ) ;
#70367=CARTESIAN_POINT ( 'NONE',  ( 97.30629616937498838, 88.66845928578037217, 81.65239583420049030 ) ) ;
#70371=CARTESIAN_POINT ( 'NONE',  ( -97.64999999999996305, -209.9999999999999716, 90.00000000000000000 ) ) ;
#70375=CARTESIAN_POINT ( 'NONE',  ( -92.69370383062498320, -209.9999999999999716, 82.34031250086714238 ) ) ;
#70384=CARTESIAN_POINT ( 'NONE',  ( -92.34999999999996589, -211.5299782133524502, 78.83458333333334167 ) ) ;
#70385=CARTESIAN_POINT ( 'NONE',  ( -92.69370383062502583, 88.66845928578038638, 88.00239583420047040 ) ) ;
#70388=CARTESIAN_POINT ( 'NONE',  ( 92.35000000000002274, -210.0000092897486468, 78.01437532303467037 ) ) ;
#70391=CARTESIAN_POINT ( 'NONE',  ( -97.30629616937501680, 90.00000000000004263, 75.03781250086713328 ) ) ;
#70396=CARTESIAN_POINT ( 'NONE',  ( -92.69370383062498320, -209.9999999999999716, 87.57906250086715261 ) ) ;
#70401=CARTESIAN_POINT ( 'NONE',  ( -97.30629616937497417, -211.3315407142195852, 76.51947916753381662 ) ) ;
#70405=DIRECTION ( 'NONE',  ( -0.000000000000000000, -0.000000000000000000, -1.000000000000000000 ) ) ;
#70411=( BOUNDED_CURVE ( )  B_SPLINE_CURVE ( 2, ( #62902, #39946, #28644, #39574, #51210, #51584, #22651, #62135, #11358 ),
 .UNSPECIFIED., .F., .T. ) 
 B_SPLINE_CURVE_WITH_KNOTS ( ( 3, 2, 2, 2, 3 ),
 ( 0.6138516023217082118, 0.6209073676006977571, 0.6279631331416146711, 0.6350188986825316961, 0.6350190250602294473 ),
 .UNSPECIFIED. ) 
 CURVE ( )  GEOMETRIC_REPRESENTATION_ITEM ( )  RATIONAL_B_SPLINE_CURVE ( ( 1.000000000000000000, 0.8660254037844387076, 1.000000000000000000, 0.8660254037844387076, 1.000000000000000000, 0.8660254037844387076, 1.000000000000000000, 0.9999976003452877293, 0.9999952007765371409 ) ) 
 REPRESENTATION_ITEM ( '' )  );
#70413=CARTESIAN_POINT ( 'NONE',  ( 92.69370383062501162, -208.6684592857803011, 76.25489583420049655 ) ) ;
#70419=LINE ( 'NONE', #52403, #51952 ) ;
#70429=EDGE_LOOP ( 'NONE', ( #41263, #56991, #9051, #36138 ) ) ;
#70430=EDGE_CURVE ( 'NONE', #62638, #5972, #23011, .T. ) ;
#70432=CARTESIAN_POINT ( 'NONE',  ( 93.84685191531248449, 91.99731107132950569, 81.44072916753381719 ) ) ;
#70434=EDGE_CURVE ( 'NONE', #42545, #32709, #28717, .T. ) ;
#70435=CARTESIAN_POINT ( 'NONE',  ( 94.15631797925327362, -214.6948328857846207, 74.84535815546847459 ) ) ;
#70445=CARTESIAN_POINT ( 'NONE',  ( -93.26027265873601380, 91.51405112163766375, 74.79348190356853365 ) ) ;
#70447=DIRECTION ( 'NONE',  ( 1.000000000000000000, 0.000000000000000000, 0.000000000000000000 ) ) ;
#70448=CARTESIAN_POINT ( 'NONE',  ( -97.65000000000009095, 88.47002178664760663, 77.98791666666667766 ) ) ;
#70450=CARTESIAN_POINT ( 'NONE',  ( -96.32499999999996021, -212.2949673200287179, 80.02520833506763154 ) ) ;
#70452=EDGE_CURVE ( 'NONE', #60230, #54767, #64728, .T. ) ;
#70453=CARTESIAN_POINT ( 'NONE',  ( 92.34999999999999432, 91.52997821335252127, 74.78645833506763552 ) ) ;
#70454=CARTESIAN_POINT ( 'NONE',  ( -95.00000000000002842, 86.94004357329504273, 74.99812500173430863 ) ) ;
#70455=VERTEX_POINT ( 'NONE', #33904 ) ;
#70456=CARTESIAN_POINT ( 'NONE',  ( 94.99999999999998579, 92.66308142843935514, 77.57781250086715374 ) ) ;
#70463=EDGE_CURVE ( 'NONE', #69471, #2166, #18613, .T. ) ;
#70467=DIRECTION ( 'NONE',  ( -0.000000000000000000, -0.000000000000000000, 1.000000000000000000 ) ) ;
#70473=CARTESIAN_POINT ( 'NONE',  ( 12.74955575014744547, 0.001194404164628405998, -85.60000000000000853 ) ) ;
#70475=CARTESIAN_POINT ( 'NONE',  ( -97.30629616937497417, -208.6684592857803011, 78.95364583420048632 ) ) ;
#70488=CARTESIAN_POINT ( 'NONE',  ( 97.30629616937498838, 91.33154071421968467, 83.82197916753382572 ) ) ;
#70489=CARTESIAN_POINT ( 'NONE',  ( -92.69370383062498320, -208.6684592857803295, 85.72697916753381264 ) ) ;
#70493=CARTESIAN_POINT ( 'NONE',  ( -94.99999999999997158, -213.0599564267049857, 81.90374999999998806 ) ) ;
#70495=CARTESIAN_POINT ( 'NONE',  ( -96.15314808468751551, 88.00268892867056536, 75.77864583420047495 ) ) ;
#70499=CARTESIAN_POINT ( 'NONE',  ( 92.69370383062501162, -211.3315407142195852, 85.88572916753382458 ) ) ;
#70502=( BOUNDED_CURVE ( )  B_SPLINE_CURVE ( 2, ( #33162, #50463, #61008, #44471, #22273, #9128, #56111 ),
 .UNSPECIFIED., .F., .F. ) 
 B_SPLINE_CURVE_WITH_KNOTS ( ( 3, 2, 2, 3 ),
 ( 0.2499999999999995837, 0.2569444444444442532, 0.2638888888888890061, 0.2708333333333337034 ),
 .UNSPECIFIED. ) 
 CURVE ( )  GEOMETRIC_REPRESENTATION_ITEM ( )  RATIONAL_B_SPLINE_CURVE ( ( 1.000000000000007994, 0.8660254037844307140, 1.000000000000000000, 0.8660254037844387076, 1.000000000000000000, 0.8660254037844311581, 1.000000000000007550 ) ) 
 REPRESENTATION_ITEM ( '' )  );
#70513=DIRECTION ( 'NONE',  ( -0.000000000000000000, -0.000000000000000000, -1.000000000000000000 ) ) ;
#70514=CARTESIAN_POINT ( 'NONE',  ( 96.15314808468748708, -208.0026889286704943, 83.23989583420049598 ) ) ;
#70520=CARTESIAN_POINT ( 'NONE',  ( 92.35000000000002274, -208.4700217866474645, 84.23208333333333542 ) ) ;
#70526=EDGE_CURVE ( 'NONE', #56117, #55837, #19044, .T. ) ;
#70529=CARTESIAN_POINT ( 'NONE',  ( -96.15314808468752972, 91.99731107132950569, 87.15572916753382060 ) ) ;
#70531=B_SPLINE_CURVE_WITH_KNOTS ( 'NONE', 3,
 ( #15459, #38403, #56818, #15842 ),
 .UNSPECIFIED., .F., .F.,
 ( 4, 4 ),
 ( 2.446487931514401995E-06, 1.000000000000000000 ),
 .UNSPECIFIED. ) ;
#70532=CARTESIAN_POINT ( 'NONE',  ( -93.67500000000003979, 87.70503267997129626, 83.86166666666666458 ) ) ;
#70533=CARTESIAN_POINT ( 'NONE',  ( 93.84685191531249870, -208.0026889286704943, 88.26697916753380468 ) ) ;
#70541=CARTESIAN_POINT ( 'NONE',  ( -96.32500000000001705, 87.70503267997129626, 87.64520833506762187 ) ) ;
#70542=CARTESIAN_POINT ( 'NONE',  ( 92.69370383062498320, 91.33154071421968467, 89.11364583420049712 ) ) ;
#70545=CARTESIAN_POINT ( 'NONE',  ( 92.35000000000000853, -209.9999999999999716, 89.90078125043358170 ) ) ;
#70546=CARTESIAN_POINT ( 'NONE',  ( 7.103376864691351012E-17, -120.0000000000000000, -64.00000000000000000 ) ) ;
#70556=CARTESIAN_POINT ( 'NONE',  ( -94.99999999999997158, -207.3369185715606307, 86.46781250086716852 ) ) ;
#70557=EDGE_LOOP ( 'NONE', ( #70333, #68525, #51870, #21303 ) ) ;
#70559=CARTESIAN_POINT ( 'NONE',  ( -97.64999999999996305, -211.5299782133524218, 82.43291666666665662 ) ) ;
#70563=ORIENTED_EDGE ( 'NONE', *, *, #65447, .T. ) ;
#70565=CARTESIAN_POINT ( 'NONE',  ( 92.69370383062498320, 90.00000000000002842, 89.80156250086714920 ) ) ;
#70568=CARTESIAN_POINT ( 'NONE',  ( 97.30629616937498838, 91.33154071421968467, 81.75822916753381264 ) ) ;
#70572=DIRECTION ( 'NONE',  ( 1.000000000000000000, 0.000000000000000000, 0.000000000000000000 ) ) ;
#70578=EDGE_CURVE ( 'NONE', #11224, #13197, #1226, .T. ) ;
#70582=CARTESIAN_POINT ( 'NONE',  ( -92.69370383062504004, 90.00000000000004263, 86.15031250086714465 ) ) ;
#70591=EDGE_LOOP ( 'NONE', ( #4918, #18522, #9992, #50842 ) ) ;
#70597=CARTESIAN_POINT ( 'NONE',  ( 96.15314808468748708, -208.0026889286704943, 83.23989583420049598 ) ) ;
#70605=CARTESIAN_POINT ( 'NONE',  ( 92.69370383062501162, -209.9999999999999716, 75.67281250086713840 ) ) ;
#70607=ORIENTED_EDGE ( 'NONE', *, *, #74295, .T. ) ;
#70608=CARTESIAN_POINT ( 'NONE',  ( 97.30629616937498838, -211.3315407142195852, 79.90614583420048689 ) ) ;
#70623=CARTESIAN_POINT ( 'NONE',  ( 95.00000000000000000, -206.9400435732949575, 84.84062500173429555 ) ) ;
#70624=CARTESIAN_POINT ( 'NONE',  ( 96.32499999999997442, 92.29496732002878900, 87.88333333333332575 ) ) ;
#70628=ORIENTED_EDGE ( 'NONE', *, *, #20184, .F. ) ;
#70630=CARTESIAN_POINT ( 'NONE',  ( -97.30629616937501680, 88.66845928578038638, 89.21947916753381946 ) ) ;
#70631=CARTESIAN_POINT ( 'NONE',  ( 96.15314808468748708, 88.00268892867053694, 85.40947916753380298 ) ) ;
#70633=CARTESIAN_POINT ( 'NONE',  ( 92.34999999999999432, 88.47002178664753558, 86.95729166840096980 ) ) ;
#70635=VERTEX_POINT ( 'NONE', #46667 ) ;
#70637=CARTESIAN_POINT ( 'NONE',  ( -92.35000000000003695, 89.99999998014077107, 85.95187500101400246 ) ) ;
#70644=CARTESIAN_POINT ( 'NONE',  ( -95.00000000000002842, 93.05995642670501411, 84.12625000000001307 ) ) ;
#70650=CARTESIAN_POINT ( 'NONE',  ( -94.99999999999997158, -212.6630814284392557, 82.18156250086714465 ) ) ;
#70651=VERTEX_POINT ( 'NONE', #13190 ) ;
#70665=CARTESIAN_POINT ( 'NONE',  ( -96.15314808468752972, 91.99731107132950569, 75.56697916753381605 ) ) ;
#70667=CARTESIAN_POINT ( 'NONE',  ( 92.35000000000005116, 88.47002178664747873, 76.08291666666664810 ) ) ;
#70673=DIRECTION ( 'NONE',  ( -1.000000000000000000, -4.476705744456277943E-17, 0.000000000000000000 ) ) ;
#70679=CARTESIAN_POINT ( 'NONE',  ( -94.99999999999997158, -213.0599564267049857, 86.98374999999998636 ) ) ;
#70684=CARTESIAN_POINT ( 'NONE',  ( -2.500000000000015543, -73.00000000000001421, -251.7000000000000455 ) ) ;
#70697=EDGE_CURVE ( 'NONE', #47426, #27953, #33990, .T. ) ;
#70698=LINE ( 'NONE', #48158, #22368 ) ;
#70701=CARTESIAN_POINT ( 'NONE',  ( 92.69370383062501162, -208.6684592857803295, 84.50989583420049200 ) ) ;
#70702=CARTESIAN_POINT ( 'NONE',  ( 93.84685191531251292, -211.9973110713294489, 89.27239583420049485 ) ) ;
#70704=ORIENTED_EDGE ( 'NONE', *, *, #15200, .T. ) ;
#70709=CARTESIAN_POINT ( 'NONE',  ( -92.69370383062502583, 88.66845928578038638, 81.81114583420048803 ) ) ;
#70712=CARTESIAN_POINT ( 'NONE',  ( -97.64999999999997726, -209.9999719686937567, 87.53937403222815306 ) ) ;
#70718=DIRECTION ( 'NONE',  ( 1.000000000000000000, 0.000000000000000000, 0.000000000000000000 ) ) ;
#70720=( BOUNDED_CURVE ( )  B_SPLINE_CURVE ( 2, ( #28449, #22080, #11169, #45774, #28826, #39753, #62704 ),
 .UNSPECIFIED., .F., .F. ) 
 B_SPLINE_CURVE_WITH_KNOTS ( ( 3, 2, 2, 3 ),
 ( 0.4374999999999994449, 0.4444444444444441422, 0.4513888888888888951, 0.4583333333333335924 ),
 .UNSPECIFIED. ) 
 CURVE ( )  GEOMETRIC_REPRESENTATION_ITEM ( )  RATIONAL_B_SPLINE_CURVE ( ( 1.000000000000010658, 0.8660254037844280495, 1.000000000000000000, 0.8660254037844387076, 1.000000000000000000, 0.8660254037844333785, 1.000000000000005329 ) ) 
 REPRESENTATION_ITEM ( '' )  );
#70727=ORIENTED_EDGE ( 'NONE', *, *, #62325, .F. ) ;
#70729=CARTESIAN_POINT ( 'NONE',  ( 97.30629616937498838, -208.6684592857803011, 79.85322916753379729 ) ) ;
#70732=DIRECTION ( 'NONE',  ( -0.000000000000000000, -0.000000000000000000, 1.000000000000000000 ) ) ;
#70739=CARTESIAN_POINT ( 'NONE',  ( -97.65000000000001990, 88.47002178664754979, 82.43291666666665662 ) ) ;
#70740=CARTESIAN_POINT ( 'NONE',  ( -97.30629616937495996, -209.9999999999999716, 80.11781250086713158 ) ) ;
#70741=CARTESIAN_POINT ( 'NONE',  ( -97.30629616937501680, 88.66845928578038638, 79.69447916753381378 ) ) ;
#70744=CARTESIAN_POINT ( 'NONE',  ( 96.15314808468748708, 91.99731107132950569, 81.81114583420047381 ) ) ;
#70750=CARTESIAN_POINT ( 'NONE',  ( -92.69370383062498320, -208.6684592857803295, 83.66322916753381378 ) ) ;
#70756=AXIS2_PLACEMENT_3D ( 'NONE', #50581, #73506, #11110 ) ;
#70757=VECTOR ( 'NONE', #2179, 1000.000000000000000 ) ;
#70764=ADVANCED_FACE ( 'NONE', ( #8670 ), #55265, .F. ) ;
#70766=CARTESIAN_POINT ( 'NONE',  ( -97.30629616937501680, 90.00000000000004263, 85.83281250086714920 ) ) ;
#70768=CARTESIAN_POINT ( 'NONE',  ( 23.49955575014745435, 0.001194404164629722436, -64.00000000000000000 ) ) ;
#70769=LINE ( 'NONE', #33041, #3788 ) ;
#70772=CARTESIAN_POINT ( 'NONE',  ( -97.30629616937501680, 90.00000000000004263, 76.30781250086714351 ) ) ;
#70777=CARTESIAN_POINT ( 'NONE',  ( 97.65000000000000568, -208.4700217866474645, 84.09979166840098230 ) ) ;
#70778=CARTESIAN_POINT ( 'NONE',  ( -97.64999999992174651, -209.9999869687493685, 79.28395951166956479 ) ) ;
#70779=CARTESIAN_POINT ( 'NONE',  ( -96.15314808468747287, -208.0026889286704943, 85.25072916753381946 ) ) ;
#70785=CARTESIAN_POINT ( 'NONE',  ( -93.84685191531248449, -208.0026889286704943, 76.88989583420048746 ) ) ;
#70794=CARTESIAN_POINT ( 'NONE',  ( 92.69370383062501162, -209.9999999999999716, 87.26156250086715715 ) ) ;
#70801=CARTESIAN_POINT ( 'NONE',  ( -15.70000000000000284, -120.0000000000000000, -85.59999999999999432 ) ) ;
#70802=EDGE_CURVE ( 'NONE', #11565, #47064, #9463, .T. ) ;
#70816=CARTESIAN_POINT ( 'NONE',  ( 96.15314808468748708, 88.00268892867053694, 80.48822916753381662 ) ) ;
#70818=CARTESIAN_POINT ( 'NONE',  ( -93.67500000000003979, 92.29496732002878900, 87.96270833506763154 ) ) ;
#70826=CARTESIAN_POINT ( 'NONE',  ( -96.90895014231846005, 91.56137061862953885, 74.88237134757150670 ) ) ;
#70827=CARTESIAN_POINT ( 'NONE',  ( 92.34999999999999432, 90.00000000000002842, 78.01437500173430806 ) ) ;
#70831=CARTESIAN_POINT ( 'NONE',  ( -92.34999999999999432, -209.9999999999999716, 78.96687500173429441 ) ) ;
#70834=CARTESIAN_POINT ( 'NONE',  ( 92.34999999999999432, 88.47002178664753558, 76.79729166840095900 ) ) ;
#70835=CARTESIAN_POINT ( 'NONE',  ( -93.67500000000003979, 92.29496732002878900, 76.53270833506762472 ) ) ;
#70838=CARTESIAN_POINT ( 'NONE',  ( 93.84685191531248449, 88.00268892867053694, 75.30239583420048177 ) ) ;
#70839=CARTESIAN_POINT ( 'NONE',  ( 96.32499999999997442, 92.29496732002878900, 82.16833333333332234 ) ) ;
#70857=CARTESIAN_POINT ( 'NONE',  ( -92.35000000000007958, -208.4700217866474077, 75.76541666666668107 ) ) ;
#70858=CARTESIAN_POINT ( 'NONE',  ( -97.30629616937497417, -211.3315407142195852, 75.88447916753382572 ) ) ;
#70870=CARTESIAN_POINT ( 'NONE',  ( -97.64999999996706492, -209.9999916046304520, 84.99910573338409847 ) ) ;
#70874=ADVANCED_FACE ( 'NONE', ( #33430 ), #68786, .F. ) ;
#70876=CARTESIAN_POINT ( 'NONE',  ( 92.69370383062498320, 91.33154071421968467, 84.66864583420047552 ) ) ;
#70877=CARTESIAN_POINT ( 'NONE',  ( -96.15314808468745866, -211.9973110713294489, 87.36739583420049371 ) ) ;
#70879=ORIENTED_EDGE ( 'NONE', *, *, #56467, .T. ) ;
#70881=CARTESIAN_POINT ( 'NONE',  ( -96.32499999999996021, -207.7050326799711968, 80.36916666666665776 ) ) ;
#70882=CARTESIAN_POINT ( 'NONE',  ( -95.00000000000002842, 87.33691857156074434, 75.83156250086715033 ) ) ;
#70884=CARTESIAN_POINT ( 'NONE',  ( 96.15314808468748708, -208.0026889286704943, 85.62114583420046188 ) ) ;
#70894=VECTOR ( 'NONE', #64026, 1000.000000000000000 ) ;
#70897=CARTESIAN_POINT ( 'NONE',  ( 95.00000000000000000, -212.6630814284392557, 79.80031250086715033 ) ) ;
#70900=CARTESIAN_POINT ( 'NONE',  ( 92.34999999999995168, -211.5299782133524502, 80.52791666666665549 ) ) ;
#70903=CARTESIAN_POINT ( 'NONE',  ( 93.67500000000001137, -212.2949673200287179, 86.29583333333333428 ) ) ;
#70912=CARTESIAN_POINT ( 'NONE',  ( -95.00000000000002842, 87.33691857156074434, 82.97531250086716170 ) ) ;
#70918=CARTESIAN_POINT ( 'NONE',  ( -93.67499999999998295, -207.7050326799711968, 88.59770833506763665 ) ) ;
#70922=CARTESIAN_POINT ( 'NONE',  ( -92.35000000000005116, 91.52997821335253548, 84.73479166840097321 ) ) ;
#70923=CARTESIAN_POINT ( 'NONE',  ( 92.69370383062498320, 90.00000000000002842, 86.62656250086715204 ) ) ;
#70935=CARTESIAN_POINT ( 'NONE',  ( 92.34999999999999432, 90.00000000000002842, 78.64937500173429896 ) ) ;
#70938=CARTESIAN_POINT ( 'NONE',  ( -97.65000000000001990, 89.99998767024830215, 75.47437542817787914 ) ) ;
#70939=CARTESIAN_POINT ( 'NONE',  ( -92.69370383062498320, -208.6684592857803011, 86.99697916753382287 ) ) ;
#70943=ORIENTED_EDGE ( 'NONE', *, *, #72943, .T. ) ;
#70948=CARTESIAN_POINT ( 'NONE',  ( 96.15314808468748708, 91.99731107132950569, 88.95489583420049939 ) ) ;
#70950=CARTESIAN_POINT ( 'NONE',  ( 92.69370383062498320, 90.00000000000002842, 82.65781250086713783 ) ) ;
#70954=CARTESIAN_POINT ( 'NONE',  ( -92.35000000053409508, 90.00005320149026034, 78.96687695417308817 ) ) ;
#70958=( BOUNDED_CURVE ( )  B_SPLINE_CURVE ( 2, ( #72329, #64856, #24987, #32100, #48295, #59207, #71581 ),
 .UNSPECIFIED., .F., .F. ) 
 B_SPLINE_CURVE_WITH_KNOTS ( ( 3, 2, 2, 3 ),
 ( 0.7831899741065915244, 0.7902457405788252398, 0.7973015061197076259, 0.8043570860654229993 ),
 .UNSPECIFIED. ) 
 CURVE ( )  GEOMETRIC_REPRESENTATION_ITEM ( )  RATIONAL_B_SPLINE_CURVE ( ( 1.000000000000000000, 0.8660254037844387076, 1.000000000000000000, 0.8660254037844387076, 1.000000000000000000, 0.8660289278581059236, 0.9999929520380603787 ) ) 
 REPRESENTATION_ITEM ( '' )  );
#70964=CARTESIAN_POINT ( 'NONE',  ( -92.69370383062504004, 90.00000000000004263, 87.42031250086714067 ) ) ;
#70966=EDGE_CURVE ( 'NONE', #27457, #5237, #41944, .T. ) ;
#70968=CARTESIAN_POINT ( 'NONE',  ( -94.99999999999997158, -209.9999999999999716, 90.00000000000000000 ) ) ;
#70972=VERTEX_POINT ( 'NONE', #1130 ) ;
#70973=AXIS2_PLACEMENT_3D ( 'NONE', #49975, #14663, #8666 ) ;
#70977=CARTESIAN_POINT ( 'NONE',  ( 92.69370383062501162, -208.6684592857803011, 80.85864583420048746 ) ) ;
#70981=VERTEX_POINT ( 'NONE', #40203 ) ;
#70984=ORIENTED_EDGE ( 'NONE', *, *, #17143, .T. ) ;
#70985=CARTESIAN_POINT ( 'NONE',  ( 95.00000000000000000, -212.6630814284392557, 81.07031250086716057 ) ) ;
#70997=CARTESIAN_POINT ( 'NONE',  ( 92.35000000000002274, -208.4700217866474645, 83.04145833506763097 ) ) ;
#70998=CARTESIAN_POINT ( 'NONE',  ( 94.99999999999998579, 86.94004357329500010, 83.80875000000000341 ) ) ;
#70999=B_SPLINE_CURVE_WITH_KNOTS ( 'NONE', 1,
 ( #22844, #67953 ),
 .UNSPECIFIED., .F., .F.,
 ( 2, 2 ),
 ( 0.000000000000000000, 1.000000000000000000 ),
 .UNSPECIFIED. ) ;
#71005=ORIENTED_EDGE ( 'NONE', *, *, #68668, .F. ) ;
#71006=CARTESIAN_POINT ( 'NONE',  ( -95.00000000000002842, 87.33691857156074434, 87.42031250086715488 ) ) ;
#71007=CARTESIAN_POINT ( 'NONE',  ( 94.99999999999998579, 87.33691857156068750, 80.91156250086714863 ) ) ;
#71009=CARTESIAN_POINT ( 'NONE',  ( 93.67499999999999716, 87.70503267997126784, 87.64520833506762187 ) ) ;
#71023=CARTESIAN_POINT ( 'NONE',  ( -93.67500000000003979, 92.29496732002878900, 85.34333333333333371 ) ) ;
#71029=CARTESIAN_POINT ( 'NONE',  ( -96.15314808468745866, -211.9973110713294489, 82.76364583420047438 ) ) ;
#71035=DIRECTION ( 'NONE',  ( -1.000000000000000000, 0.000000000000000000, 0.000000000000000000 ) ) ;
#71043=CARTESIAN_POINT ( 'NONE',  ( -92.69370383062502583, 91.33154071421968467, 76.67822916753378593 ) ) ;
#71052=CARTESIAN_POINT ( 'NONE',  ( 96.90829729882861443, 88.16127723153182671, 74.99954709728268654 ) ) ;
#71056=CARTESIAN_POINT ( 'NONE',  ( -97.64999999999996305, -209.9999999999999716, 87.45999999999999375 ) ) ;
#71059=ORIENTED_EDGE ( 'NONE', *, *, #50656, .F. ) ;
#71069=ORIENTED_EDGE ( 'NONE', *, *, #70966, .T. ) ;
#71070=CARTESIAN_POINT ( 'NONE',  ( 93.84685191531249870, -208.0026889286704943, 82.55197916753380127 ) ) ;
#71071=CARTESIAN_POINT ( 'NONE',  ( 97.30629616937498838, -209.9999999999999716, 88.21406250086714351 ) ) ;
#71073=CARTESIAN_POINT ( 'NONE',  ( 92.69370383062501162, -209.9999999999999716, 88.53156250086716739 ) ) ;
#71077=CARTESIAN_POINT ( 'NONE',  ( -92.69370383062504004, 90.00000000000004263, 76.14906250086716000 ) ) ;
#71079=VERTEX_POINT ( 'NONE', #40953 ) ;
#71083=CARTESIAN_POINT ( 'NONE',  ( 92.35000000001610942, 89.99999393654047708, 88.17456390440148084 ) ) ;
#71085=EDGE_CURVE ( 'NONE', #42391, #28639, #871, .T. ) ;
#71095=CARTESIAN_POINT ( 'NONE',  ( 92.69370383062501162, -208.6684592857803011, 79.42989583420046529 ) ) ;
#71096=CARTESIAN_POINT ( 'NONE',  ( -97.65000000000001990, 90.00000000000004263, 83.65000000000000568 ) ) ;
#71097=CARTESIAN_POINT ( 'NONE',  ( -95.00000000000002842, 86.94004357329504273, 81.90375000000000227 ) ) ;
#71102=ADVANCED_FACE ( 'NONE', ( #25856, #14954 ), #26226, .F. ) ;
#71106=CARTESIAN_POINT ( 'NONE',  ( -94.99999999999997158, -212.6630814284392557, 79.64156250086713840 ) ) ;
#71107=CARTESIAN_POINT ( 'NONE',  ( -97.30629616937501680, 88.66845928578038638, 79.05947916753382287 ) ) ;
#71110=CARTESIAN_POINT ( 'NONE',  ( 94.99999999999998579, 92.66308142843935514, 82.49906250086714010 ) ) ;
#71115=EDGE_CURVE ( 'NONE', #59392, #24150, #11392, .T. ) ;
#71119=CARTESIAN_POINT ( 'NONE',  ( -92.69370383062498320, -209.9999999999999716, 83.61031250086713840 ) ) ;
#71124=VERTEX_POINT ( 'NONE', #60824 ) ;
#71130=CARTESIAN_POINT ( 'NONE',  ( -97.65000000000001990, 90.00000000000004263, 77.93499999999998806 ) ) ;
#71132=CARTESIAN_POINT ( 'NONE',  ( -97.30629616937501680, 88.66845928578038638, 85.88572916753382458 ) ) ;
#71136=VERTEX_POINT ( 'NONE', #65361 ) ;
#71137=CARTESIAN_POINT ( 'NONE',  ( -97.30629616937501680, 88.66845928578038638, 75.72572916753381378 ) ) ;
#71143=CARTESIAN_POINT ( 'NONE',  ( -96.15314808468747287, -208.0026889286704943, 82.07572916753382231 ) ) ;
#71145=B_SPLINE_CURVE_WITH_KNOTS ( 'NONE', 1,
 ( #50054, #56471 ),
 .UNSPECIFIED., .F., .F.,
 ( 2, 2 ),
 ( 0.000000000000000000, 1.000000000000000000 ),
 .UNSPECIFIED. ) ;
#71146=CARTESIAN_POINT ( 'NONE',  ( 92.69370383062498320, 90.00000000000002842, 75.19656250086714522 ) ) ;
#71151=CARTESIAN_POINT ( 'NONE',  ( -96.32499999999996021, -212.2949673200287179, 81.93020833506763267 ) ) ;
#71156=CARTESIAN_POINT ( 'NONE',  ( 95.00000000000000000, -207.3369185715606307, 89.00781250086716057 ) ) ;
#71163=( BOUNDED_CURVE ( )  B_SPLINE_CURVE ( 2, ( #56221, #44579, #18129, #12477, #21242, #35416, #44197, #67123, #38560 ),
 .UNSPECIFIED., .F., .F. ) 
 B_SPLINE_CURVE_WITH_KNOTS ( ( 3, 2, 2, 2, 3 ),
 ( 0.5715170088666294834, 0.5785727743523534361, 0.5856285398932349340, 0.5926843054341166539, 0.5926843883797353607 ),
 .UNSPECIFIED. ) 
 CURVE ( )  GEOMETRIC_REPRESENTATION_ITEM ( )  RATIONAL_B_SPLINE_CURVE ( ( 1.000000000000000000, 0.8660254037844387076, 1.000000000000000000, 0.8660254037844387076, 1.000000000000000000, 0.8660254037844387076, 1.000000000000000000, 0.9999984250318816326, 0.9999968501007930888 ) ) 
 REPRESENTATION_ITEM ( '' )  );
#71176=CARTESIAN_POINT ( 'NONE',  ( 94.99999999999998579, 87.33691857156068750, 79.80031250086715033 ) ) ;
#71177=FACE_BOUND ( 'NONE', #16907, .T. ) ;
#71178=CARTESIAN_POINT ( 'NONE',  ( -97.64999999998390479, 89.99999393654049129, 88.17456390440148084 ) ) ;
#71193=CARTESIAN_POINT ( 'NONE',  ( -92.34999999999999432, -209.9999999999999716, 75.79187500173429726 ) ) ;
#71194=CARTESIAN_POINT ( 'NONE',  ( -93.84685191531254134, 91.99731107132950569, 88.31989583420048007 ) ) ;
#71196=CARTESIAN_POINT ( 'NONE',  ( 93.67499999999998295, 92.29496732002878900, 76.63854166840096127 ) ) ;
#71197=CARTESIAN_POINT ( 'NONE',  ( -97.65000000000001990, 88.47002178664754979, 74.89229166840097207 ) ) ;
#71199=CARTESIAN_POINT ( 'NONE',  ( 93.84685191531248449, 91.99731107132950569, 75.72572916753382799 ) ) ;
#71203=CARTESIAN_POINT ( 'NONE',  ( 97.65000000000000568, -208.4700217866474645, 77.11479166840095445 ) ) ;
#71211=EDGE_LOOP ( 'NONE', ( #36223, #56636, #20778, #20636 ) ) ;
#71214=CARTESIAN_POINT ( 'NONE',  ( 96.32499999999998863, -207.7050326799711968, 82.80333333333332746 ) ) ;
#71217=CARTESIAN_POINT ( 'NONE',  ( -97.65000000000001990, 88.47002178664754979, 76.16229166840095388 ) ) ;
#71219=CARTESIAN_POINT ( 'NONE',  ( -97.30629616937495996, -209.9999999999999716, 75.19656250086714522 ) ) ;
#71229=PLANE ( 'NONE',  #53687 ) ;
#71230=DIRECTION ( 'NONE',  ( 1.000000000000000000, 0.000000000000000000, 0.000000000000000000 ) ) ;
#71231=CARTESIAN_POINT ( 'NONE',  ( -90.00000000000002842, 85.00000000000002842, 90.00000000000000000 ) ) ;
#71232=DIRECTION ( 'NONE',  ( 0.000000000000000000, 0.000000000000000000, 1.000000000000000000 ) ) ;
#71235=CARTESIAN_POINT ( 'NONE',  ( 96.15314808468748708, 91.99731107132950569, 83.23989583420049598 ) ) ;
#71236=CARTESIAN_POINT ( 'NONE',  ( -93.84685191531247028, -211.9973110713294489, 86.83822916753382515 ) ) ;
#71237=CARTESIAN_POINT ( 'NONE',  ( 92.35004149907325655, -211.5300021728535285, 83.78229332575388355 ) ) ;
#71240=CARTESIAN_POINT ( 'NONE',  ( -96.32499999999996021, -207.7050326799711968, 81.63916666666666799 ) ) ;
#71241=CARTESIAN_POINT ( 'NONE',  ( -92.69370383062504004, 90.00000000000004263, 75.99031250086714806 ) ) ;
#71242=CARTESIAN_POINT ( 'NONE',  ( 97.30629616937498838, -208.6684592857803011, 84.93322916753379559 ) ) ;
#71243=VERTEX_POINT ( 'NONE', #59716 ) ;
#71244=VECTOR ( 'NONE', #62759, 1000.000000000000000 ) ;
#71251=CARTESIAN_POINT ( 'NONE',  ( -96.32500000000001705, 87.70503267997129626, 79.39020833506762642 ) ) ;
#71256=CARTESIAN_POINT ( 'NONE',  ( 97.30629616937498838, -208.6684592857803295, 78.10697916753383652 ) ) ;
#71265=CARTESIAN_POINT ( 'NONE',  ( 93.67500000000001137, -212.2949673200287179, 79.94583333333332575 ) ) ;
#71266=EDGE_LOOP ( 'NONE', ( #35868, #43646, #23994 ) ) ;
#71274=CARTESIAN_POINT ( 'NONE',  ( -95.00000000000002842, 92.66308142843932671, 82.65781250086715204 ) ) ;
#71277=CARTESIAN_POINT ( 'NONE',  ( 94.99999999999998579, 93.05995642670504253, 75.23624999999999829 ) ) ;
#71279=CARTESIAN_POINT ( 'NONE',  ( -94.99999999999997158, -213.0599564267049857, 87.69812500173429726 ) ) ;
#71280=ORIENTED_EDGE ( 'NONE', *, *, #59971, .T. ) ;
#71283=ORIENTED_EDGE ( 'NONE', *, *, #2409, .T. ) ;
#71284=CARTESIAN_POINT ( 'NONE',  ( -97.65000000000001990, 88.47002178664754979, 85.68729166840097378 ) ) ;
#71286=CARTESIAN_POINT ( 'NONE',  ( 93.84685191531248449, 88.00268892867053694, 86.09739583420049769 ) ) ;
#71296=CARTESIAN_POINT ( 'NONE',  ( -92.69370383062498320, -208.6684592857803011, 74.77322916753379900 ) ) ;
#71299=FACE_BOUND ( 'NONE', #63842, .T. ) ;
#71301=CARTESIAN_POINT ( 'NONE',  ( -2.500000000000020428, -90.00000000000000000, -310.0000000000000000 ) ) ;
#71303=DIRECTION ( 'NONE',  ( -0.000000000000000000, -0.000000000000000000, 1.000000000000000000 ) ) ;
#71304=CARTESIAN_POINT ( 'NONE',  ( -94.99999999999997158, -212.6630814284392557, 82.97531250086716170 ) ) ;
#71307=ORIENTED_EDGE ( 'NONE', *, *, #5962, .T. ) ;
#71311=CARTESIAN_POINT ( 'NONE',  ( 96.15314808468748708, 88.00268892867053694, 89.37822916753381719 ) ) ;
#71313=CARTESIAN_POINT ( 'NONE',  ( 92.69370383062498320, 90.00000000000002842, 80.75281250086715090 ) ) ;
#71323=DIRECTION ( 'NONE',  ( -4.476705744456276711E-17, 1.000000000000000000, -0.000000000000000000 ) ) ;
#71326=CARTESIAN_POINT ( 'NONE',  ( -92.69370383062505425, 91.33154071421968467, 86.20322916753380582 ) ) ;
#71328=DIRECTION ( 'NONE',  ( 0.000000000000000000, 0.000000000000000000, 1.000000000000000000 ) ) ;
#71333=CARTESIAN_POINT ( 'NONE',  ( 97.64999999999999147, -210.0000000198592716, 85.95187500101400246 ) ) ;
#71337=CARTESIAN_POINT ( 'NONE',  ( 93.84685191531249870, -208.0026889286704943, 82.07572916753382231 ) ) ;
#71339=EDGE_CURVE ( 'NONE', #26229, #24481, #5178, .T. ) ;
#71344=EDGE_LOOP ( 'NONE', ( #18171, #17748 ) ) ;
#71351=CARTESIAN_POINT ( 'NONE',  ( 96.15314808468748708, -208.0026889286704943, 74.98489583420048632 ) ) ;
#71356=VERTEX_POINT ( 'NONE', #38254 ) ;
#71360=ORIENTED_EDGE ( 'NONE', *, *, #13151, .F. ) ;
#71362=CARTESIAN_POINT ( 'NONE',  ( 97.64999999999997726, -211.5299782133524502, 82.72395833506762131 ) ) ;
#71363=CARTESIAN_POINT ( 'NONE',  ( 96.32499999999998863, 87.70503267997126784, 85.76666666666665151 ) ) ;
#71365=CARTESIAN_POINT ( 'NONE',  ( -92.35000000000003695, 90.00000000000004263, 85.87249999999998806 ) ) ;
#71366=CARTESIAN_POINT ( 'NONE',  ( -93.67500000000003979, 87.70503267997129626, 75.05104166840095559 ) ) ;
#71369=CARTESIAN_POINT ( 'NONE',  ( -93.84685191531254134, 91.99731107132950569, 86.41489583420049314 ) ) ;
#71371=CARTESIAN_POINT ( 'NONE',  ( 93.84685191531248449, 91.99731107132950569, 80.64697916753381435 ) ) ;
#71376=CARTESIAN_POINT ( 'NONE',  ( 92.34999999999999432, 90.00000000000002842, 84.36437500173430237 ) ) ;
#71379=CARTESIAN_POINT ( 'NONE',  ( 93.67500000000001137, -212.2949673200287179, 78.04083333333333883 ) ) ;
#71388=CARTESIAN_POINT ( 'NONE',  ( -96.32500000000001705, 87.70503267997129626, 85.66083333333332916 ) ) ;
#71394=( BOUNDED_CURVE ( )  B_SPLINE_CURVE ( 2, ( #71096, #24512, #47811, #7955, #25618, #65120, #13595 ),
 .UNSPECIFIED., .F., .F. ) 
 B_SPLINE_CURVE_WITH_KNOTS ( ( 3, 2, 2, 3 ),
 ( 0.4166666666666662966, 0.4236111111111106609, 0.4305555555555550806, 0.4374999999999994449 ),
 .UNSPECIFIED. ) 
 CURVE ( )  GEOMETRIC_REPRESENTATION_ITEM ( )  RATIONAL_B_SPLINE_CURVE ( ( 1.000000000000007550, 0.8660254037844311581, 1.000000000000000000, 0.8660254037844387076, 1.000000000000000000, 0.8660254037844493658, 0.9999999999999893419 ) ) 
 REPRESENTATION_ITEM ( '' )  );
#71395=CARTESIAN_POINT ( 'NONE',  ( 92.35000000000000853, -211.5299782133525071, 84.97291666666667709 ) ) ;
#71396=CARTESIAN_POINT ( 'NONE',  ( -97.30629616937497417, -211.3315407142195852, 78.26572916753380582 ) ) ;
#71400=LINE ( 'NONE', #1927, #15257 ) ;
#71409=CARTESIAN_POINT ( 'NONE',  ( -96.15314808468751551, 88.00268892867056536, 89.27239583420049485 ) ) ;
#71417=DIRECTION ( 'NONE',  ( -1.000000000000000000, 0.000000000000000000, 0.000000000000000000 ) ) ;
#71419=CARTESIAN_POINT ( 'NONE',  ( 94.99999999999998579, 86.94004357329502852, 75.63312500173429953 ) ) ;
#71420=CARTESIAN_POINT ( 'NONE',  ( -92.34999999999999432, -209.9999999999999716, 87.14249999999999829 ) ) ;
#71421=FACE_OUTER_BOUND ( 'NONE', #12561, .T. ) ;
#71426=DIRECTION ( 'NONE',  ( 0.000000000000000000, -1.000000000000000000, 0.000000000000000000 ) ) ;
#71428=CARTESIAN_POINT ( 'NONE',  ( -92.35000000000005116, 91.52997821335254969, 84.65541666666669585 ) ) ;
#71437=PLANE ( 'NONE',  #49941 ) ;
#71440=CARTESIAN_POINT ( 'NONE',  ( 97.30629616937498838, -208.6684592857803295, 80.48822916753380241 ) ) ;
#71441=CARTESIAN_POINT ( 'NONE',  ( 97.30629616937498838, -208.6684592857803295, 89.53697916753382913 ) ) ;
#71444=CARTESIAN_POINT ( 'NONE',  ( 93.84685191531249870, -208.0026889286704943, 87.15572916753382060 ) ) ;
#71446=CARTESIAN_POINT ( 'NONE',  ( -97.64999999999996305, -209.9999999999999716, 80.47499999999999432 ) ) ;
#71448=CARTESIAN_POINT ( 'NONE',  ( -97.30629616937501680, 90.00000000000004263, 78.37156250086715659 ) ) ;
#71454=CARTESIAN_POINT ( 'NONE',  ( 97.64999999999999147, 89.99999996655866141, 87.85687500050293863 ) ) ;
#71458=DIRECTION ( 'NONE',  ( 0.000000000000000000, -0.000000000000000000, 1.000000000000000000 ) ) ;
#71459=ORIENTED_EDGE ( 'NONE', *, *, #62659, .T. ) ;
#71460=CARTESIAN_POINT ( 'NONE',  ( 92.35000000000010800, -211.5299782133525071, 86.24291666666667311 ) ) ;
#71464=CARTESIAN_POINT ( 'NONE',  ( 92.69370383062501162, -211.3315407142195852, 79.53572916753380184 ) ) ;
#71469=CARTESIAN_POINT ( 'NONE',  ( 96.90829729882861443, 88.16127723153182671, 74.99954709728268654 ) ) ;
#71470=ORIENTED_EDGE ( 'NONE', *, *, #17095, .F. ) ;
#71471=CARTESIAN_POINT ( 'NONE',  ( -92.34999999999999432, -209.9999999999999716, 78.96687500173429441 ) ) ;
#71476=CARTESIAN_POINT ( 'NONE',  ( -92.34999999999999432, -208.4700217866474645, 88.54479166840097548 ) ) ;
#71478=CARTESIAN_POINT ( 'NONE',  ( -93.84685191531248449, -208.0026889286704943, 79.90614583420047268 ) ) ;
#71479=CARTESIAN_POINT ( 'NONE',  ( -97.30629616937501680, 91.33154071421968467, 79.58864583420047722 ) ) ;
#71480=EDGE_LOOP ( 'NONE', ( #1013, #19023, #51662, #3894 ) ) ;
#71481=CARTESIAN_POINT ( 'NONE',  ( 92.69370383062498320, 90.00000000000002842, 80.11781250086713158 ) ) ;
#71489=CARTESIAN_POINT ( 'NONE',  ( -92.69370383062498320, -211.3315407142195852, 82.28739583420048120 ) ) ;
#71490=CARTESIAN_POINT ( 'NONE',  ( -93.67499999999998295, -212.2949673200287179, 89.57666666666666799 ) ) ;
#71494=ORIENTED_EDGE ( 'NONE', *, *, #58795, .T. ) ;
#71498=CARTESIAN_POINT ( 'NONE',  ( -95.00000000000002842, 86.94004357329504273, 75.55375000000000796 ) ) ;
#71499=CARTESIAN_POINT ( 'NONE',  ( -95.00000000000002842, 90.00000000000004263, 90.00000000000000000 ) ) ;
#71500=CARTESIAN_POINT ( 'NONE',  ( -92.69370383062504004, 90.00000000000004263, 83.61031250086713840 ) ) ;
#71501=CARTESIAN_POINT ( 'NONE',  ( -96.13030974027459763, -207.8557763824826452, 74.86230178910949462 ) ) ;
#71506=ORIENTED_EDGE ( 'NONE', *, *, #3601, .F. ) ;
#71507=CARTESIAN_POINT ( 'NONE',  ( -96.15314808468751551, 88.00268892867056536, 75.14364583420046984 ) ) ;
#71513=CARTESIAN_POINT ( 'NONE',  ( 96.32499999999998863, -207.7050326799711968, 84.70833333333332860 ) ) ;
#71515=CARTESIAN_POINT ( 'NONE',  ( -92.69370383062498320, -208.6684592857803011, 83.82197916753382572 ) ) ;
#71517=DIRECTION ( 'NONE',  ( -1.000000000000000000, 3.061616997868382648E-16, 0.000000000000000000 ) ) ;
#71522=CARTESIAN_POINT ( 'NONE',  ( -96.32500000000001705, 87.70503267997129626, 88.83583333333334053 ) ) ;
#71527=ADVANCED_FACE ( 'NONE', ( #34843 ), #30210, .F. ) ;
#71528=DIRECTION ( 'NONE',  ( 1.000000000000000000, 0.000000000000000000, 0.000000000000000000 ) ) ;
#71529=CARTESIAN_POINT ( 'NONE',  ( 96.15314808468748708, -208.0026889286704943, 88.95489583420049939 ) ) ;
#71530=ORIENTED_EDGE ( 'NONE', *, *, #73825, .F. ) ;
#71532=CARTESIAN_POINT ( 'NONE',  ( 97.64999999999999147, -209.9999999999999716, 87.14249999999999829 ) ) ;
#71545=ORIENTED_EDGE ( 'NONE', *, *, #17552, .F. ) ;
#71555=CARTESIAN_POINT ( 'NONE',  ( 93.84685191531248449, 88.00268892867053694, 79.11239583420048405 ) ) ;
#71570=CARTESIAN_POINT ( 'NONE',  ( -97.65000000000001990, 90.00000000000004263, 77.93499999999998806 ) ) ;
#71572=CARTESIAN_POINT ( 'NONE',  ( -92.34999999999999432, -211.5299782133524502, 76.37395833506761278 ) ) ;
#71573=CARTESIAN_POINT ( 'NONE',  ( -92.69370383062504004, 90.00000000000004263, 87.57906250086715261 ) ) ;
#71574=CARTESIAN_POINT ( 'NONE',  ( 92.34999999999999432, 91.52997821335252127, 77.32645833506762756 ) ) ;
#71575=CARTESIAN_POINT ( 'NONE',  ( -92.69370383062502583, 91.33154071421968467, 88.74322916753379786 ) ) ;
#71577=CARTESIAN_POINT ( 'NONE',  ( 93.84685191531248449, 88.00268892867053694, 77.20739583420048291 ) ) ;
#71581=CARTESIAN_POINT ( 'NONE',  ( 92.35000000046409241, -210.0000309672231253, 77.38038495127494798 ) ) ;
#71582=CARTESIAN_POINT ( 'NONE',  ( -92.35000000000012221, 91.52997821335257811, 89.10041666666667481 ) ) ;
#71584=CARTESIAN_POINT ( 'NONE',  ( -94.99999999999997158, -213.0599564267049857, 79.99874999999998693 ) ) ;
#71585=DIRECTION ( 'NONE',  ( -0.000000000000000000, -0.000000000000000000, 1.000000000000000000 ) ) ;
#71593=CARTESIAN_POINT ( 'NONE',  ( 93.67499999999999716, 87.70503267997126784, 84.39083333333333314 ) ) ;
#71596=EDGE_CURVE ( 'NONE', #7925, #73668, #18077, .T. ) ;
#71607=DIRECTION ( 'NONE',  ( -0.000000000000000000, -0.000000000000000000, 1.000000000000000000 ) ) ;
#71608=CARTESIAN_POINT ( 'NONE',  ( 2.499999999999979572, 90.00000000000000000, -280.0000000000000000 ) ) ;
#71609=EDGE_CURVE ( 'NONE', #56423, #54488, #46645, .T. ) ;
#71612=( BOUNDED_CURVE ( )  B_SPLINE_CURVE ( 2, ( #18003, #6725, #69868, #20212, #72453, #49163, #31123 ),
 .UNSPECIFIED., .F., .F. ) 
 B_SPLINE_CURVE_WITH_KNOTS ( ( 3, 2, 2, 3 ),
 ( 0.2916666666666669072, 0.2986111111111113270, 0.3055555555555557468, 0.3125000000000001665 ),
 .UNSPECIFIED. ) 
 CURVE ( )  GEOMETRIC_REPRESENTATION_ITEM ( )  RATIONAL_B_SPLINE_CURVE ( ( 0.9999999999999956701, 0.8660254037844430375, 1.000000000000000000, 0.8660254037844387076, 1.000000000000000000, 0.8660254037844354880, 1.000000000000003109 ) ) 
 REPRESENTATION_ITEM ( '' )  );
#71613=CARTESIAN_POINT ( 'NONE',  ( 97.30629616937498838, 90.00000000000002842, 85.03906250086714635 ) ) ;
#71615=CARTESIAN_POINT ( 'NONE',  ( -94.99999999999997158, -207.3369185715606307, 82.02281250086714692 ) ) ;
#71618=PLANE ( 'NONE',  #35286 ) ;
#71619=CARTESIAN_POINT ( 'NONE',  ( -94.99999999999997158, -213.0599564267049857, 79.36374999999999602 ) ) ;
#71622=CARTESIAN_POINT ( 'NONE',  ( 95.00000000000000000, -207.3369185715606307, 85.03906250086714635 ) ) ;
#71628=CARTESIAN_POINT ( 'NONE',  ( 97.64999999999999147, -209.9999999999999716, 83.96750000000000114 ) ) ;
#71632=CARTESIAN_POINT ( 'NONE',  ( 93.84685191531249870, -208.0026889286704943, 77.63072916753381492 ) ) ;
#71641=CARTESIAN_POINT ( 'NONE',  ( -97.64995971452408696, 88.46999852781715390, 83.14729327728630892 ) ) ;
#71642=CARTESIAN_POINT ( 'NONE',  ( 93.67500000000001137, -207.7050326799711968, 82.27416666666665890 ) ) ;
#71650=CARTESIAN_POINT ( 'NONE',  ( -95.00000000000002842, 87.33691857156074434, 84.24531250086715772 ) ) ;
#71651=CARTESIAN_POINT ( 'NONE',  ( -94.99999999999997158, -209.9999999999999716, 90.00000000000000000 ) ) ;
#71654=CARTESIAN_POINT ( 'NONE',  ( 97.64999999999997726, 91.52997821335252127, 76.40041666666667197 ) ) ;
#71657=CARTESIAN_POINT ( 'NONE',  ( -92.34999999999999432, -211.5299782133524502, 85.89895833506764689 ) ) ;
#71662=CARTESIAN_POINT ( 'NONE',  ( -95.00000000000002842, 93.05995642670501411, 88.01562500173429271 ) ) ;
#71664=CARTESIAN_POINT ( 'NONE',  ( 97.30629616937498838, 91.33154071421968467, 85.72697916753381264 ) ) ;
#71675=ORIENTED_EDGE ( 'NONE', *, *, #24718, .F. ) ;
#71676=CARTESIAN_POINT ( 'NONE',  ( 93.67499999999999716, 87.70503267997126784, 78.75520833506763552 ) ) ;
#71680=CARTESIAN_POINT ( 'NONE',  ( -94.99999999999997158, -207.3369185715606307, 85.83281250086714920 ) ) ;
#71682=CARTESIAN_POINT ( 'NONE',  ( -95.00000000000002842, 90.00000000000004263, 90.00000000000000000 ) ) ;
#71686=FACE_OUTER_BOUND ( 'NONE', #61352, .T. ) ;
#71688=CARTESIAN_POINT ( 'NONE',  ( 94.99999999999998579, 92.66308142843932671, 76.78406250086712248 ) ) ;
#71690=CARTESIAN_POINT ( 'NONE',  ( 92.35000000003284981, 90.00000839192529156, 86.90410584365271518 ) ) ;
#71698=FACE_OUTER_BOUND ( 'NONE', #37199, .T. ) ;
#71701=CARTESIAN_POINT ( 'NONE',  ( 97.64999999999689351, 89.99999595380309358, 77.06187486178042434 ) ) ;
#71703=CARTESIAN_POINT ( 'NONE',  ( -95.00000000000002842, 92.66308142843932671, 83.76906250086715033 ) ) ;
#71704=DIRECTION ( 'NONE',  ( -0.000000000000000000, -0.000000000000000000, 1.000000000000000000 ) ) ;
#71712=CARTESIAN_POINT ( 'NONE',  ( 92.69370383062501162, -209.9999999999999716, 79.00656250086716170 ) ) ;
#71722=DIRECTION ( 'NONE',  ( -0.000000000000000000, -0.000000000000000000, 1.000000000000000000 ) ) ;
#71723=CARTESIAN_POINT ( 'NONE',  ( 96.15314808468748708, -208.0026889286704943, 76.88989583420048746 ) ) ;
#71728=CARTESIAN_POINT ( 'NONE',  ( -94.99999999999997158, -206.9400435732949575, 82.30062500173427509 ) ) ;
#71733=CARTESIAN_POINT ( 'NONE',  ( 97.64999999999999147, -209.9999999999999716, 84.68187500173429783 ) ) ;
#71734=CARTESIAN_POINT ( 'NONE',  ( 92.34999999999999432, 90.00000000000002842, 84.28499999999999659 ) ) ;
#71740=CARTESIAN_POINT ( 'NONE',  ( -92.69370383062505425, 91.33154071421968467, 88.90197916753382401 ) ) ;
#71742=CARTESIAN_POINT ( 'NONE',  ( 97.30629616937498838, 91.33154071421968467, 82.39322916753381776 ) ) ;
#71744=CARTESIAN_POINT ( 'NONE',  ( 96.32499999999998863, 87.70503267997126784, 82.03604166840096923 ) ) ;
#71746=VERTEX_POINT ( 'NONE', #7534 ) ;
#71751=ORIENTED_EDGE ( 'NONE', *, *, #47134, .F. ) ;
#71755=CARTESIAN_POINT ( 'NONE',  ( -95.00000000000002842, 93.05995642670501411, 84.76125000000000398 ) ) ;
#71757=CYLINDRICAL_SURFACE ( 'NONE', #46785, 2.649999999999985700 ) ;
#71761=CARTESIAN_POINT ( 'NONE',  ( -93.67499999999998295, -212.2949673200287179, 75.05104166840095559 ) ) ;
#71762=CARTESIAN_POINT ( 'NONE',  ( -92.69370383062498320, -211.3315407142195852, 77.84239583420045960 ) ) ;
#71764=CARTESIAN_POINT ( 'NONE',  ( 92.35000000000000853, -209.9999999999999716, 90.00000000000000000 ) ) ;
#71772=CARTESIAN_POINT ( 'NONE',  ( 96.15314808468748708, 91.99731107132950569, 87.52614583420047722 ) ) ;
#71779=CARTESIAN_POINT ( 'NONE',  ( -95.00000000000002842, 92.66308142843932671, 74.87906250086713555 ) ) ;
#71781=CARTESIAN_POINT ( 'NONE',  ( 92.34999999999999432, 90.00000000000002842, 76.03000000000000114 ) ) ;
#71783=CARTESIAN_POINT ( 'NONE',  ( 93.67500000000001137, -207.7050326799711968, 75.28916666666665947 ) ) ;
#71790=CARTESIAN_POINT ( 'NONE',  ( -94.99999999999997158, -213.0599564267049857, 88.25374999999999659 ) ) ;
#71809=CARTESIAN_POINT ( 'NONE',  ( 97.30629616937498838, -211.3315407142195852, 80.38239583420049428 ) ) ;
#71810=CARTESIAN_POINT ( 'NONE',  ( 93.84685191531249870, -208.0026889286704943, 83.98072916753382344 ) ) ;
#71812=CARTESIAN_POINT ( 'NONE',  ( 93.84685191531251292, -211.9973110713294489, 86.09739583420049769 ) ) ;
#71815=VERTEX_POINT ( 'NONE', #24097 ) ;
#71818=CARTESIAN_POINT ( 'NONE',  ( -97.30629616937501680, 91.33154071421968467, 77.04864583420048518 ) ) ;
#71824=ORIENTED_EDGE ( 'NONE', *, *, #5962, .F. ) ;
#71826=CARTESIAN_POINT ( 'NONE',  ( 92.35000000000000853, -209.9999999999999716, 79.20499999999999829 ) ) ;
#71831=( BOUNDED_CURVE ( )  B_SPLINE_CURVE ( 2, ( #2650, #42830, #65761, #62367, #56344, #45065, #60863 ),
 .UNSPECIFIED., .F., .T. ) 
 B_SPLINE_CURVE_WITH_KNOTS ( ( 3, 2, 2, 3 ),
 ( 0.2291666666666663521, 0.2361111111111107719, 0.2430555555555551639, 0.2499999999999995837 ),
 .UNSPECIFIED. ) 
 CURVE ( )  GEOMETRIC_REPRESENTATION_ITEM ( )  RATIONAL_B_SPLINE_CURVE ( ( 1.000000000000005995, 0.8660254037844328234, 1.000000000000000000, 0.8660254037844387076, 1.000000000000000000, 0.8660254037844467012, 0.9999999999999920064 ) ) 
 REPRESENTATION_ITEM ( '' )  );
#71832=CARTESIAN_POINT ( 'NONE',  ( 92.35000000000000853, -209.9999999999999716, 81.18937500173430521 ) ) ;
#71833=ORIENTED_EDGE ( 'NONE', *, *, #19947, .T. ) ;
#71836=CARTESIAN_POINT ( 'NONE',  ( 92.69370383062501162, -211.3315407142195852, 78.26572916753380582 ) ) ;
#71845=CARTESIAN_POINT ( 'NONE',  ( -97.30629616937501680, 90.00000000000004263, 79.00656250086716170 ) ) ;
#71847=CARTESIAN_POINT ( 'NONE',  ( 94.99999999999998579, 92.66308142843935514, 79.32406250086714294 ) ) ;
#71848=VERTEX_POINT ( 'NONE', #59408 ) ;
#71850=CARTESIAN_POINT ( 'NONE',  ( -93.84685191531247028, -211.9973110713294489, 87.94947916753380923 ) ) ;
#71852=CARTESIAN_POINT ( 'NONE',  ( 96.92442009029373651, 88.17815826261617929, 75.00000000000000000 ) ) ;
#71855=CARTESIAN_POINT ( 'NONE',  ( -96.15314808468745866, -211.9973110713294489, 82.12864583420046927 ) ) ;
#71866=CARTESIAN_POINT ( 'NONE',  ( 99.99999999999998579, 95.00000000000001421, -90.00000000000002842 ) ) ;
#71870=CARTESIAN_POINT ( 'NONE',  ( -96.32500000000001705, 87.70503267997129626, 84.47020833506762472 ) ) ;
#71871=CARTESIAN_POINT ( 'NONE',  ( -95.00000000000002842, 87.33691857156074434, 86.62656250086715204 ) ) ;
#71878=DIRECTION ( 'NONE',  ( -0.000000000000000000, -0.000000000000000000, 1.000000000000000000 ) ) ;
#71881=CARTESIAN_POINT ( 'NONE',  ( 94.99999999999998579, 90.00000000000002842, 90.00000000000000000 ) ) ;
#71883=CARTESIAN_POINT ( 'NONE',  ( 97.65000000000006253, 88.47002178664756400, 86.45458333333331780 ) ) ;
#71884=CARTESIAN_POINT ( 'NONE',  ( -93.84685191531247028, -211.9973110713294489, 81.75822916753382685 ) ) ;
#71902=CIRCLE ( 'NONE', #7087, 15.69999999999999929 ) ;
#71918=CARTESIAN_POINT ( 'NONE',  ( -2.500000000000015543, -73.00000000000001421, -204.9999999999999716 ) ) ;
#71919=ORIENTED_EDGE ( 'NONE', *, *, #3942, .T. ) ;
#71921=CARTESIAN_POINT ( 'NONE',  ( 97.30629616937498838, 91.33154071421968467, 77.47197916753381719 ) ) ;
#71923=CARTESIAN_POINT ( 'NONE',  ( -96.32500000000001705, 87.70503267997129626, 85.02583333333332405 ) ) ;
#71931=CARTESIAN_POINT ( 'NONE',  ( 95.00000000000000000, -206.9400435732949575, 74.68062500173429896 ) ) ;
#71935=CARTESIAN_POINT ( 'NONE',  ( 97.64999999999999147, 90.00000000000002842, 83.96750000000000114 ) ) ;
#71936=CARTESIAN_POINT ( 'NONE',  ( -95.78927932462359252, 92.27861417635790531, 74.85481846778735360 ) ) ;
#71938=DIRECTION ( 'NONE',  ( -0.000000000000000000, -0.000000000000000000, 1.000000000000000000 ) ) ;
#71939=CARTESIAN_POINT ( 'NONE',  ( -94.99999999999997158, -209.9999999999999716, 90.00000000000000000 ) ) ;
#71943=CARTESIAN_POINT ( 'NONE',  ( -97.64999999999994884, -211.5299782133524502, 76.79729166840095900 ) ) ;
#71946=CARTESIAN_POINT ( 'NONE',  ( 96.15314808468748708, 91.99731107132950569, 86.89114583420047211 ) ) ;
#71947=CARTESIAN_POINT ( 'NONE',  ( -92.69370383062504004, 90.00000000000004263, 87.42031250086714067 ) ) ;
#71949=CARTESIAN_POINT ( 'NONE',  ( 94.99999999999998579, 87.33691857156068750, 77.26031250086714408 ) ) ;
#71951=CARTESIAN_POINT ( 'NONE',  ( 95.00000000000000000, -213.0599564267049857, 87.61874999999999147 ) ) ;
#71953=CARTESIAN_POINT ( 'NONE',  ( -92.35000000000005116, 89.99998452726650555, 78.33187446658585884 ) ) ;
#71954=CARTESIAN_POINT ( 'NONE',  ( -92.35000000000003695, 90.00000000000004263, 89.04749999999999943 ) ) ;
#71963=CARTESIAN_POINT ( 'NONE',  ( -96.32500000000001705, 92.29496732002878900, 86.16354166840096696 ) ) ;
#71968=AXIS2_PLACEMENT_3D ( 'NONE', #47377, #36089, #13525 ) ;
#71969=EDGE_LOOP ( 'NONE', ( #28288, #56596, #32811, #45514 ) ) ;
#71970=CARTESIAN_POINT ( 'NONE',  ( -96.15314808468751551, 88.00268892867056536, 82.76364583420047438 ) ) ;
#71984=CARTESIAN_POINT ( 'NONE',  ( 96.15314808468748708, 88.00268892867053694, 79.85322916753381151 ) ) ;
#71985=CARTESIAN_POINT ( 'NONE',  ( -96.15314808468745866, -211.9973110713294489, 84.19239583420049655 ) ) ;
#71987=VECTOR ( 'NONE', #57010, 1000.000000000000000 ) ;
#71989=FACE_OUTER_BOUND ( 'NONE', #47735, .T. ) ;
#71991=CARTESIAN_POINT ( 'NONE',  ( -97.64999999999994884, -211.5299782133524502, 79.25791666666665947 ) ) ;
#71994=ADVANCED_FACE ( 'NONE', ( #55214 ), #43948, .F. ) ;
#71999=CARTESIAN_POINT ( 'NONE',  ( 92.69370383062501162, -209.9999999999999716, 84.56281250086713897 ) ) ;
#72007=CARTESIAN_POINT ( 'NONE',  ( 97.30629616937498838, -211.3315407142195852, 76.73114583420048973 ) ) ;
#72010=CARTESIAN_POINT ( 'NONE',  ( -97.51367041768835975, 89.99999999999990052, 74.91808492278043730 ) ) ;
#72013=CARTESIAN_POINT ( 'NONE',  ( 93.67500000000001137, -212.2949673200287179, 81.21583333333333599 ) ) ;
#72020=CARTESIAN_POINT ( 'NONE',  ( -92.69370383062502583, 91.33154071421968467, 83.82197916753382572 ) ) ;
#72021=CARTESIAN_POINT ( 'NONE',  ( -95.00000000000002842, 86.94004357329504273, 81.98312500173430806 ) ) ;
#72025=CARTESIAN_POINT ( 'NONE',  ( 95.53230763903962952, 86.73322217287211799, 74.92222617501700199 ) ) ;
#72029=CARTESIAN_POINT ( 'NONE',  ( -96.32499999999996021, -207.7050326799711968, 85.52854166840096184 ) ) ;
#72034=CARTESIAN_POINT ( 'NONE',  ( -95.00000000000002842, 93.05995642670501411, 83.57062500173429953 ) ) ;
#72036=CARTESIAN_POINT ( 'NONE',  ( 94.99999999999998579, 92.66308142843935514, 87.73781250086715033 ) ) ;
#72042=DIRECTION ( 'NONE',  ( -1.000000000000000000, -0.000000000000000000, -0.000000000000000000 ) ) ;
#72043=FACE_OUTER_BOUND ( 'NONE', #24944, .T. ) ;
#72048=CARTESIAN_POINT ( 'NONE',  ( 99.99999999999998579, 95.00000000000002842, -90.00000000000000000 ) ) ;
#72052=CARTESIAN_POINT ( 'NONE',  ( 92.34999999999999432, 88.47002178664752137, 78.70229166840096013 ) ) ;
#72056=CARTESIAN_POINT ( 'NONE',  ( -96.32499999999996021, -212.2949673200287179, 83.12083333333332291 ) ) ;
#72057=( BOUNDED_CURVE ( )  B_SPLINE_CURVE ( 2, ( #2376, #42194, #53095, #65860, #7235, #13960, #59112 ),
 .UNSPECIFIED., .F., .F. ) 
 B_SPLINE_CURVE_WITH_KNOTS ( ( 3, 2, 2, 3 ),
 ( 0.9374999999999995559, 0.9444444444444441977, 0.9513888888888889506, 0.9583333333333337034 ),
 .UNSPECIFIED. ) 
 CURVE ( )  GEOMETRIC_REPRESENTATION_ITEM ( )  RATIONAL_B_SPLINE_CURVE ( ( 1.000000000000008660, 0.8660254037844301589, 1.000000000000000000, 0.8660254037844387076, 1.000000000000000000, 0.8660254037844322683, 1.000000000000006439 ) ) 
 REPRESENTATION_ITEM ( '' )  );
#72058=CARTESIAN_POINT ( 'NONE',  ( -96.15314808468745866, -211.9973110713294489, 84.19239583420049655 ) ) ;
#72067=CARTESIAN_POINT ( 'NONE',  ( 92.69370383062498320, 88.66845928578035796, 78.90072916753381094 ) ) ;
#72071=CARTESIAN_POINT ( 'NONE',  ( 92.54662210827905255, 90.48452257634333762, 74.90854212414863866 ) ) ;
#72076=DIRECTION ( 'NONE',  ( -0.000000000000000000, -0.000000000000000000, 1.000000000000000000 ) ) ;
#72077=CARTESIAN_POINT ( 'NONE',  ( 92.35000000039373447, 90.00002930740642171, 76.74344264317738862 ) ) ;
#72080=CARTESIAN_POINT ( 'NONE',  ( -97.30629616937501680, 88.66845928578038638, 81.44072916753380298 ) ) ;
#72083=AXIS2_PLACEMENT_3D ( 'NONE', #3655, #60056, #43866 ) ;
#72085=ORIENTED_EDGE ( 'NONE', *, *, #62121, .T. ) ;
#72087=LINE ( 'NONE', #37895, #25219 ) ;
#72092=CARTESIAN_POINT ( 'NONE',  ( 97.30629616937498838, -208.6684592857803011, 79.37697916753381833 ) ) ;
#72102=CARTESIAN_POINT ( 'NONE',  ( 93.84685191531251292, -211.9973110713294489, 77.20739583420048291 ) ) ;
#72107=DIRECTION ( 'NONE',  ( 1.000000000000000000, 0.000000000000000000, 0.000000000000000000 ) ) ;
#72113=CARTESIAN_POINT ( 'NONE',  ( 97.64999999999999147, -209.9999999999999716, 79.60187500173429953 ) ) ;
#72114=CARTESIAN_POINT ( 'NONE',  ( 97.64999999999997726, 88.47002178664753558, 85.81958333333331268 ) ) ;
#72119=ORIENTED_EDGE ( 'NONE', *, *, #47267, .T. ) ;
#72121=CARTESIAN_POINT ( 'NONE',  ( -97.30629616937501680, 91.33154071421968467, 85.30364583420048064 ) ) ;
#72122=CARTESIAN_POINT ( 'NONE',  ( 97.30629616937498838, 90.00000000000002842, 81.70531250086713726 ) ) ;
#72125=ADVANCED_FACE ( 'NONE', ( #50685 ), #39420, .F. ) ;
#72141=CARTESIAN_POINT ( 'NONE',  ( -97.30629616937495996, -209.9999999999999716, 78.21281250086714465 ) ) ;
#72144=EDGE_CURVE ( 'NONE', #15908, #61999, #44545, .T. ) ;
#72146=LINE ( 'NONE', #20656, #15310 ) ;
#72147=CARTESIAN_POINT ( 'NONE',  ( -96.32499999999996021, -207.7050326799711968, 89.33854166840096411 ) ) ;
#72152=CARTESIAN_POINT ( 'NONE',  ( 93.84685191531248449, 91.99731107132950569, 89.53697916753381492 ) ) ;
#72153=CYLINDRICAL_SURFACE ( 'NONE', #55626, 2.649999999999985700 ) ;
#72156=CARTESIAN_POINT ( 'NONE',  ( -97.65000000000001990, 89.99996562134467126, 88.80937619077336365 ) ) ;
#72164=DIRECTION ( 'NONE',  ( 1.000000000000000000, 0.000000000000000000, 0.000000000000000000 ) ) ;
#72168=CARTESIAN_POINT ( 'NONE',  ( -97.64999999999994884, -208.4700217866474645, 88.67708333333332860 ) ) ;
#72173=FILL_AREA_STYLE_COLOUR ( '', #1054 ) ;
#72185=CARTESIAN_POINT ( 'NONE',  ( 95.00000000000000000, -212.6630814284392557, 82.18156250086715886 ) ) ;
#72186=CARTESIAN_POINT ( 'NONE',  ( 95.00000000000000000, -212.6630814284392557, 84.88031250086713442 ) ) ;
#72188=CARTESIAN_POINT ( 'NONE',  ( 93.84685191531251292, -211.9973110713294489, 87.36739583420049371 ) ) ;
#72193=CARTESIAN_POINT ( 'NONE',  ( -93.84685191531254134, 91.99731107132950569, 77.52489583420047836 ) ) ;
#72196=EDGE_LOOP ( 'NONE', ( #67357, #22945 ) ) ;
#72206=AXIS2_PLACEMENT_3D ( 'NONE', #36855, #59802, #8286 ) ;
#72207=CARTESIAN_POINT ( 'NONE',  ( 97.65000000000000568, -211.5299782133524218, 81.45395833506763950 ) ) ;
#72209=EDGE_CURVE ( 'NONE', #52406, #58523, #41664, .T. ) ;
#72210=EDGE_LOOP ( 'NONE', ( #42540, #46059, #52919, #37404 ) ) ;
#72212=CARTESIAN_POINT ( 'NONE',  ( 97.30629616937498838, -208.6684592857803011, 77.31322916753380525 ) ) ;
#72217=ORIENTED_EDGE ( 'NONE', *, *, #8653, .F. ) ;
#72220=CARTESIAN_POINT ( 'NONE',  ( -92.69370383062504004, 90.00000000000004263, 78.68906250086715204 ) ) ;
#72223=CARTESIAN_POINT ( 'NONE',  ( 96.15314808468748708, 91.99731107132950569, 76.09614583420047040 ) ) ;
#72231=CARTESIAN_POINT ( 'NONE',  ( -92.69370383062498320, -208.6684592857803295, 77.94822916753381037 ) ) ;
#72236=EDGE_CURVE ( 'NONE', #47150, #66356, #74104, .T. ) ;
#72246=CARTESIAN_POINT ( 'NONE',  ( -93.84685191531254134, 91.99731107132950569, 86.25614583420048120 ) ) ;
#72259=CARTESIAN_POINT ( 'NONE',  ( -97.30629616937495996, -209.9999999999999716, 84.08656250086716000 ) ) ;
#72263=( BOUNDED_CURVE ( )  B_SPLINE_CURVE ( 2, ( #4407, #50239, #16791, #16412, #22051, #33700, #67545 ),
 .UNSPECIFIED., .F., .F. ) 
 B_SPLINE_CURVE_WITH_KNOTS ( ( 3, 2, 2, 3 ),
 ( 0.7831899741104385582, 0.7902457405827062464, 0.7973015061236232714, 0.8043570860693807223 ),
 .UNSPECIFIED. ) 
 CURVE ( )  GEOMETRIC_REPRESENTATION_ITEM ( )  RATIONAL_B_SPLINE_CURVE ( ( 1.000000000000000000, 0.8660254037844387076, 1.000000000000000000, 0.8660254037844387076, 1.000000000000000000, 0.8660289278579667016, 0.9999929520383388226 ) ) 
 REPRESENTATION_ITEM ( '' )  );
#72271=CARTESIAN_POINT ( 'NONE',  ( 97.65000000000000568, -208.4700217866474645, 79.57541666666666913 ) ) ;
#72277=CARTESIAN_POINT ( 'NONE',  ( -2.500000000000015543, -73.00000000000001421, -208.2999999999999261 ) ) ;
#72284=ADVANCED_FACE ( 'NONE', ( #64565 ), #58546, .F. ) ;
#72294=CYLINDRICAL_SURFACE ( 'NONE', #10691, 3.299999999999969624 ) ;
#72300=CARTESIAN_POINT ( 'NONE',  ( 97.30629616937498838, 91.33154071421968467, 76.20197916753382117 ) ) ;
#72306=CARTESIAN_POINT ( 'NONE',  ( 92.69370383062498320, 91.33154071421968467, 87.04989583420048405 ) ) ;
#72309=CARTESIAN_POINT ( 'NONE',  ( 97.30629616937498838, -209.9999999999999716, 88.69031250086715090 ) ) ;
#72318=CARTESIAN_POINT ( 'NONE',  ( -94.99999999999997158, -206.9400435732949575, 75.95062500173428077 ) ) ;
#72319=CARTESIAN_POINT ( 'NONE',  ( -93.84685191531254134, 91.99731107132950569, 87.68489583420048916 ) ) ;
#72321=CARTESIAN_POINT ( 'NONE',  ( 94.99999999999998579, 92.66308142843935514, 87.57906250086713840 ) ) ;
#72322=CARTESIAN_POINT ( 'NONE',  ( -93.84685191531254134, 91.99731107132950569, 86.89114583420047211 ) ) ;
#72329=CARTESIAN_POINT ( 'NONE',  ( 97.64999999999996305, -209.9999996502043018, 77.69687501385438111 ) ) ;
#72335=EDGE_LOOP ( 'NONE', ( #23507, #25959 ) ) ;
#72337=CARTESIAN_POINT ( 'NONE',  ( -97.65000000000001990, 91.52997821335253548, 82.96208333333333940 ) ) ;
#72340=CARTESIAN_POINT ( 'NONE',  ( 92.35000000000000853, -209.9999999999999716, 76.03000000000000114 ) ) ;
#72344=CARTESIAN_POINT ( 'NONE',  ( 97.64999999999999147, 90.00000000000002842, 84.60249999999999204 ) ) ;
#72346=CARTESIAN_POINT ( 'NONE',  ( -93.84685191531254134, 91.99731107132950569, 81.81114583420047381 ) ) ;
#72348=CARTESIAN_POINT ( 'NONE',  ( 92.34999999999999432, 90.00003216987884969, 82.45937388908920695 ) ) ;
#72349=CARTESIAN_POINT ( 'NONE',  ( -96.32500000000001705, 87.70503267997129626, 85.66083333333332916 ) ) ;
#72354=CARTESIAN_POINT ( 'NONE',  ( -97.64999999999996305, -209.9999999999999716, 86.18999999999999773 ) ) ;
#72359=CARTESIAN_POINT ( 'NONE',  ( 96.15314808468748708, 91.99731107132950569, 81.33489583420049485 ) ) ;
#72360=CARTESIAN_POINT ( 'NONE',  ( -92.69370383062498320, -211.3315407142195852, 83.08114583420048405 ) ) ;
#72364=CARTESIAN_POINT ( 'NONE',  ( -92.34999999999999432, -209.9999999999999716, 76.34749999999999659 ) ) ;
#72365=CYLINDRICAL_SURFACE ( 'NONE', #558, 2.649999999999985700 ) ;
#72368=CARTESIAN_POINT ( 'NONE',  ( 92.69370383062501162, -209.9999999999999716, 83.92781250086714806 ) ) ;
#72370=DIRECTION ( 'NONE',  ( -0.000000000000000000, -0.000000000000000000, 1.000000000000000000 ) ) ;
#72377=CARTESIAN_POINT ( 'NONE',  ( 93.84685191531251292, -211.9973110713294489, 77.20739583420048291 ) ) ;
#72380=FACE_OUTER_BOUND ( 'NONE', #42994, .T. ) ;
#72381=CARTESIAN_POINT ( 'NONE',  ( 97.30629616937498838, 88.66845928578037217, 88.16114583420048234 ) ) ;
#72383=CARTESIAN_POINT ( 'NONE',  ( 97.64999999999997726, -211.5299782133524502, 82.64458333333331552 ) ) ;
#72391=CARTESIAN_POINT ( 'NONE',  ( -92.69370383062502583, 88.66845928578038638, 83.71614583420050337 ) ) ;
#72394=( BOUNDED_CURVE ( )  B_SPLINE_CURVE ( 2, ( #74007, #27393, #44334, #10113, #5611, #67634, #39068 ),
 .UNSPECIFIED., .F., .F. ) 
 B_SPLINE_CURVE_WITH_KNOTS ( ( 3, 2, 2, 3 ),
 ( 0.5624999999999997780, 0.5694444444444440867, 0.5763888888888885065, 0.5833333333333329263 ),
 .UNSPECIFIED. ) 
 CURVE ( )  GEOMETRIC_REPRESENTATION_ITEM ( )  RATIONAL_B_SPLINE_CURVE ( ( 1.000000000000004219, 0.8660254037844343777, 1.000000000000000000, 0.8660254037844387076, 1.000000000000000000, 0.8660254037844472563, 0.9999999999999914513 ) ) 
 REPRESENTATION_ITEM ( '' )  );
#72399=CARTESIAN_POINT ( 'NONE',  ( -92.34999999999999432, -209.9999999999999716, 85.95187500173430806 ) ) ;
#72404=CARTESIAN_POINT ( 'NONE',  ( -93.67500000000003979, 87.70503267997129626, 83.30604166840096525 ) ) ;
#72406=CARTESIAN_POINT ( 'NONE',  ( 92.69370383062498320, 91.33154071421968467, 86.57364583420047666 ) ) ;
#72414=CARTESIAN_POINT ( 'NONE',  ( 92.35000000000000853, -209.9999999999999716, 77.93499999999998806 ) ) ;
#72425=CARTESIAN_POINT ( 'NONE',  ( -93.84685191531248449, -208.0026889286704943, 85.77989583420048803 ) ) ;
#72430=CARTESIAN_POINT ( 'NONE',  ( 97.64999999999324132, 90.00000598221777182, 82.14187520865721126 ) ) ;
#72431=CARTESIAN_POINT ( 'NONE',  ( 92.34999999999999432, -210.0000348885106405, 83.09437620840748195 ) ) ;
#72432=CARTESIAN_POINT ( 'NONE',  ( 92.69370383062498320, 88.66845928578035796, 76.99572916753380980 ) ) ;
#72438=CARTESIAN_POINT ( 'NONE',  ( -93.67499999999998295, -212.2949673200287179, 87.03666666666666174 ) ) ;
#72443=CARTESIAN_POINT ( 'NONE',  ( 93.67499999999998295, 92.29496732002878900, 89.25916666666667254 ) ) ;
#72445=CARTESIAN_POINT ( 'NONE',  ( -96.15314808468751551, 88.00268892867056536, 82.76364583420047438 ) ) ;
#72452=CARTESIAN_POINT ( 'NONE',  ( -97.64999999993855795, 90.00001182178863246, 76.10900611559313234 ) ) ;
#72453=CARTESIAN_POINT ( 'NONE',  ( 96.32499999999997442, 92.29496732002878900, 85.34333333333333371 ) ) ;
#72458=CARTESIAN_POINT ( 'NONE',  ( 97.30629616937498838, -211.3315407142195852, 77.36614583420048064 ) ) ;
#72460=ORIENTED_EDGE ( 'NONE', *, *, #8347, .T. ) ;
#72461=ORIENTED_EDGE ( 'NONE', *, *, #30308, .F. ) ;
#72464=CARTESIAN_POINT ( 'NONE',  ( -2.499999999999970690, 73.00000000000001421, -255.0000000000000000 ) ) ;
#72467=ADVANCED_FACE ( 'NONE', ( #72043 ), #19797, .F. ) ;
#72469=CARTESIAN_POINT ( 'NONE',  ( 95.00000000000000000, -212.6630814284392557, 77.89531250086714920 ) ) ;
#72480=CARTESIAN_POINT ( 'NONE',  ( 97.64999999999997726, -208.4700217866474645, 80.92479166840098515 ) ) ;
#72481=CARTESIAN_POINT ( 'NONE',  ( 92.34999999999999432, 91.52997821335252127, 84.86708333333334053 ) ) ;
#72483=ORIENTED_EDGE ( 'NONE', *, *, #25415, .T. ) ;
#72488=ORIENTED_EDGE ( 'NONE', *, *, #42306, .F. ) ;
#72490=( BOUNDED_CURVE ( )  B_SPLINE_CURVE ( 2, ( #51372, #51748, #40465, #295, #5541, #63059, #22823 ),
 .UNSPECIFIED., .F., .F. ) 
 B_SPLINE_CURVE_WITH_KNOTS ( ( 3, 2, 2, 3 ),
 ( 0.4791666666666668517, 0.4861111111111112160, 0.4930555555555556357, 0.5000000000000000000 ),
 .UNSPECIFIED. ) 
 CURVE ( )  GEOMETRIC_REPRESENTATION_ITEM ( )  RATIONAL_B_SPLINE_CURVE ( ( 0.9999999999999967804, 0.8660254037844419273, 1.000000000000000000, 0.8660254037844387076, 1.000000000000000000, 0.8660254037844387076, 1.000000000000000000 ) ) 
 REPRESENTATION_ITEM ( '' )  );
#72491=CARTESIAN_POINT ( 'NONE',  ( -92.69370383062505425, 88.66845928578038638, 83.71614583420048916 ) ) ;
#72492=CARTESIAN_POINT ( 'NONE',  ( 92.69370383062498320, 91.33154071421968467, 83.23989583420046756 ) ) ;
#72498=ORIENTED_EDGE ( 'NONE', *, *, #65899, .T. ) ;
#72500=CARTESIAN_POINT ( 'NONE',  ( 96.32499999999998863, 87.70503267997126784, 80.05166666666666231 ) ) ;
#72502=DIRECTION ( 'NONE',  ( -0.000000000000000000, -0.000000000000000000, 1.000000000000000000 ) ) ;
#72504=CARTESIAN_POINT ( 'NONE',  ( 93.67499999999999716, 87.70503267997126784, 88.28020833506764120 ) ) ;
#72506=FACE_OUTER_BOUND ( 'NONE', #4215, .T. ) ;
#72507=CARTESIAN_POINT ( 'NONE',  ( -92.69370383062498320, -208.6684592857803011, 80.48822916753383083 ) ) ;
#72515=AXIS2_PLACEMENT_3D ( 'NONE', #7908, #70673, #35727 ) ;
#72517=CARTESIAN_POINT ( 'NONE',  ( 94.99999999999998579, 92.66308142843932671, 88.84906250086713442 ) ) ;
#72525=LINE ( 'NONE', #38708, #60465 ) ;
#72527=AXIS2_PLACEMENT_3D ( 'NONE', #163, #63278, #45984 ) ;
#72530=CARTESIAN_POINT ( 'NONE',  ( -93.67499999999998295, -207.7050326799711968, 84.70833333333332860 ) ) ;
#72533=FACE_OUTER_BOUND ( 'NONE', #53261, .T. ) ;
#72540=VECTOR ( 'NONE', #28471, 1000.000000000000000 ) ;
#72545=ORIENTED_EDGE ( 'NONE', *, *, #47228, .F. ) ;
#72546=CIRCLE ( 'NONE', #7747, 23.50000000000000355 ) ;
#72547=CARTESIAN_POINT ( 'NONE',  ( 93.84685191531251292, -211.9973110713294489, 80.22364583420046813 ) ) ;
#72548=CARTESIAN_POINT ( 'NONE',  ( 97.30629616937498838, -211.3315407142195852, 84.35114583420050849 ) ) ;
#72549=EDGE_CURVE ( 'NONE', #15281, #48178, #44611, .T. ) ;
#72551=CARTESIAN_POINT ( 'NONE',  ( 93.84685191531251292, -211.9973110713294489, 84.82739583420048746 ) ) ;
#72552=ORIENTED_EDGE ( 'NONE', *, *, #27655, .F. ) ;
#72556=CARTESIAN_POINT ( 'NONE',  ( -92.69370383062504004, 90.00000000000004263, 76.78406250086715090 ) ) ;
#72567=EDGE_CURVE ( 'NONE', #64357, #47972, #72768, .T. ) ;
#72576=CARTESIAN_POINT ( 'NONE',  ( 97.30629616937498838, -209.9999999999999716, 74.72031250086713783 ) ) ;
#72577=DIRECTION ( 'NONE',  ( -1.000000000000000000, 3.061616997868382648E-16, 0.000000000000000000 ) ) ;
#72581=CARTESIAN_POINT ( 'NONE',  ( -97.64999999999992042, -211.5299782133524786, 84.33791666666667197 ) ) ;
#72583=CARTESIAN_POINT ( 'NONE',  ( -96.32500000000001705, 92.29496732002878900, 89.89416666666666345 ) ) ;
#72585=CARTESIAN_POINT ( 'NONE',  ( 96.15314808468748708, 91.99731107132950569, 78.00114583420048575 ) ) ;
#72587=CARTESIAN_POINT ( 'NONE',  ( -97.30629616937497417, -208.6684592857803011, 89.58989583420047609 ) ) ;
#72591=CARTESIAN_POINT ( 'NONE',  ( -96.15314808468747287, -208.0026889286704943, 79.37697916753380412 ) ) ;
#72599=CARTESIAN_POINT ( 'NONE',  ( -97.64999999999984936, -211.5299782133525071, 88.78291666666667936 ) ) ;
#72600=CARTESIAN_POINT ( 'NONE',  ( 97.64999999999999147, 89.99999990163419739, 80.23687499810812085 ) ) ;
#72601=CARTESIAN_POINT ( 'NONE',  ( -97.30629616937501680, 88.66845928578038638, 82.71072916753379900 ) ) ;
#72614=CARTESIAN_POINT ( 'NONE',  ( -96.15314808468745866, -211.9973110713294489, 84.19239583420049655 ) ) ;
#72628=AXIS2_PLACEMENT_3D ( 'NONE', #1389, #35914, #58865 ) ;
#72633=VERTEX_POINT ( 'NONE', #38962 ) ;
#72636=CARTESIAN_POINT ( 'NONE',  ( -92.35000000000000853, 91.52997821335250705, 77.67041666666666799 ) ) ;
#72643=VERTEX_POINT ( 'NONE', #22407 ) ;
#72647=EDGE_CURVE ( 'NONE', #51903, #44494, #20882, .T. ) ;
#72651=CARTESIAN_POINT ( 'NONE',  ( 92.69370383062498320, 90.00000000000002842, 75.83156250086716454 ) ) ;
#72659=CARTESIAN_POINT ( 'NONE',  ( 97.30629616937498838, 91.33154071421968467, 88.10822916753380696 ) ) ;
#72660=VERTEX_POINT ( 'NONE', #32560 ) ;
#72661=CARTESIAN_POINT ( 'NONE',  ( 97.30629616937498838, -211.3315407142195852, 85.46239583420047836 ) ) ;
#72664=CARTESIAN_POINT ( 'NONE',  ( -97.65000000000001990, 91.52997821335253548, 77.32645833506762756 ) ) ;
#72668=FACE_OUTER_BOUND ( 'NONE', #57976, .T. ) ;
#72670=CARTESIAN_POINT ( 'NONE',  ( -93.84685191531247028, -211.9973110713294489, 88.58447916753381435 ) ) ;
#72671=CARTESIAN_POINT ( 'NONE',  ( -97.30629616937501680, 90.00000000000004263, 89.16656250086715829 ) ) ;
#72673=CARTESIAN_POINT ( 'NONE',  ( 97.30629616937498838, 91.33154071421968467, 88.10822916753380696 ) ) ;
#72674=CARTESIAN_POINT ( 'NONE',  ( -93.84685191531254134, 91.99731107132950569, 87.52614583420047722 ) ) ;
#72676=CARTESIAN_POINT ( 'NONE',  ( 96.32499999999998863, -212.2949673200287179, 84.57604166840096127 ) ) ;
#72679=CARTESIAN_POINT ( 'NONE',  ( 94.99999999999998579, 93.05995642670504253, 82.30062500173427509 ) ) ;
#72681=CARTESIAN_POINT ( 'NONE',  ( -96.15314808468747287, -208.0026889286704943, 88.90197916753380980 ) ) ;
#72682=LINE ( 'NONE', #50883, #60205 ) ;
#72684=ORIENTED_EDGE ( 'NONE', *, *, #9518, .T. ) ;
#72687=CARTESIAN_POINT ( 'NONE',  ( -92.35000000000003695, 90.00000000000004263, 82.06250000000000000 ) ) ;
#72692=CARTESIAN_POINT ( 'NONE',  ( -97.64999999993855795, 90.00001182178863246, 76.10900611559313234 ) ) ;
#72693=( BOUNDED_CURVE ( )  B_SPLINE_CURVE ( 2, ( #52156, #57438, #40512, #63457, #16472, #40147, #51794, #67604, #28114, #67977, #61972 ),
 .UNSPECIFIED., .F., .F. ) 
 B_SPLINE_CURVE_WITH_KNOTS ( ( 3, 2, 2, 2, 2, 3 ),
 ( 0.4233457466706606609, 0.4233459324550212788, 0.4304016979959381928, 0.4374574635368551623, 0.4445132290777720763, 0.4445132602993024373 ),
 .UNSPECIFIED. ) 
 CURVE ( )  GEOMETRIC_REPRESENTATION_ITEM ( )  RATIONAL_B_SPLINE_CURVE ( ( 0.9999929448536319931, 0.9999964723339295203, 1.000000000000000000, 0.8660254037844387076, 1.000000000000000000, 0.8660254037844387076, 1.000000000000000000, 0.8660254037844387076, 1.000000000000000000, 0.9999994071668198981, 0.9999988143388863771 ) ) 
 REPRESENTATION_ITEM ( '' )  );
#72696=CARTESIAN_POINT ( 'NONE',  ( -92.69370383062502583, 88.66845928578038638, 82.28739583420048120 ) ) ;
#72707=( BOUNDED_CURVE ( )  B_SPLINE_CURVE ( 2, ( #55871, #56630, #4762, #28031, #16769, #16389, #68650 ),
 .UNSPECIFIED., .F., .F. ) 
 B_SPLINE_CURVE_WITH_KNOTS ( ( 3, 2, 2, 3 ),
 ( 0.2083333333333331483, 0.2152777777777775681, 0.2222222222222219323, 0.2291666666666663521 ),
 .UNSPECIFIED. ) 
 CURVE ( )  GEOMETRIC_REPRESENTATION_ITEM ( )  RATIONAL_B_SPLINE_CURVE ( ( 1.000000000000003775, 0.8660254037844349329, 1.000000000000000000, 0.8660254037844387076, 1.000000000000000000, 0.8660254037844445918, 0.9999999999999941158 ) ) 
 REPRESENTATION_ITEM ( '' )  );
#72708=VECTOR ( 'NONE', #19709, 1000.000000000000000 ) ;
#72709=CARTESIAN_POINT ( 'NONE',  ( 93.84685191531248449, 91.99731107132950569, 80.80572916753382628 ) ) ;
#72710=CARTESIAN_POINT ( 'NONE',  ( -94.99999999999997158, -212.6630814284392557, 83.61031250086715261 ) ) ;
#72712=ORIENTED_EDGE ( 'NONE', *, *, #36143, .T. ) ;
#72714=CARTESIAN_POINT ( 'NONE',  ( -97.65000000000003411, 90.00000928824094615, 86.90437468048608594 ) ) ;
#72715=CARTESIAN_POINT ( 'NONE',  ( -92.34999999999999432, -211.5299782133524502, 76.92958333333332632 ) ) ;
#72720=CARTESIAN_POINT ( 'NONE',  ( -93.84685191531254134, 91.99731107132950569, 77.52489583420047836 ) ) ;
#72721=CARTESIAN_POINT ( 'NONE',  ( 95.00000000000000000, -212.6630814284392557, 84.72156250086713669 ) ) ;
#72731=CARTESIAN_POINT ( 'NONE',  ( -97.64999999999996305, -209.9999999999999716, 83.65000000000000568 ) ) ;
#72740=CARTESIAN_POINT ( 'NONE',  ( -94.99999999999997158, -209.9999999999999716, 90.00000000000000000 ) ) ;
#72741=CARTESIAN_POINT ( 'NONE',  ( 97.30629616937498838, 88.66845928578037217, 87.52614583420049144 ) ) ;
#72743=CARTESIAN_POINT ( 'NONE',  ( 92.35000000000002274, -208.4700217866474645, 77.24708333333332178 ) ) ;
#72751=CARTESIAN_POINT ( 'NONE',  ( -92.34999999999999432, -208.4700217866474645, 77.03541666666666288 ) ) ;
#72756=CARTESIAN_POINT ( 'NONE',  ( -93.67499999999998295, -207.7050326799711968, 85.42270833506762528 ) ) ;
#72760=CARTESIAN_POINT ( 'NONE',  ( -96.32500000000001705, 87.70503267997129626, 81.29520833506762756 ) ) ;
#72762=CARTESIAN_POINT ( 'NONE',  ( 93.84685191531248449, 91.99731107132950569, 82.07572916753382231 ) ) ;
#72764=DIRECTION ( 'NONE',  ( 1.000000000000000000, 0.000000000000000000, 0.000000000000000000 ) ) ;
#72768=LINE ( 'NONE', #11127, #14457 ) ;
#72781=CARTESIAN_POINT ( 'NONE',  ( -92.69370383062498320, -208.6684592857803011, 85.09197916753380753 ) ) ;
#72783=CARTESIAN_POINT ( 'NONE',  ( 92.35000000000000853, -209.9999999999999716, 81.10999999999999943 ) ) ;
#72787=DIRECTION ( 'NONE',  ( -0.000000000000000000, -0.000000000000000000, 1.000000000000000000 ) ) ;
#72790=CARTESIAN_POINT ( 'NONE',  ( 92.69370383062498320, 91.33154071421968467, 78.79489583420047438 ) ) ;
#72797=EDGE_CURVE ( 'NONE', #50886, #58346, #24170, .T. ) ;
#72799=CARTESIAN_POINT ( 'NONE',  ( -100.0000000000000142, 95.00000000000002842, -90.00000000000000000 ) ) ;
#72801=CARTESIAN_POINT ( 'NONE',  ( -93.67499999999998295, -212.2949673200287179, 75.68604166840097491 ) ) ;
#72803=CARTESIAN_POINT ( 'NONE',  ( -92.69370383062504004, 90.00000000000004263, 83.61031250086713840 ) ) ;
#72807=DIRECTION ( 'NONE',  ( 0.000000000000000000, 0.000000000000000000, -1.000000000000000000 ) ) ;
#72808=ORIENTED_EDGE ( 'NONE', *, *, #7290, .T. ) ;
#72814=DIRECTION ( 'NONE',  ( -0.000000000000000000, -0.000000000000000000, 1.000000000000000000 ) ) ;
#72817=CARTESIAN_POINT ( 'NONE',  ( 93.84685191531249870, -208.0026889286704943, 78.90072916753382515 ) ) ;
#72825=CARTESIAN_POINT ( 'NONE',  ( -97.64999999999996305, -210.0000359324575925, 85.63437624451401575 ) ) ;
#72828=CARTESIAN_POINT ( 'NONE',  ( 95.00000000000000000, -207.3369185715606307, 76.94281250086714863 ) ) ;
#72836=LINE ( 'NONE', #60485, #16119 ) ;
#72839=CARTESIAN_POINT ( 'NONE',  ( 92.35000000000002274, -211.5299782133524502, 79.33729166840096525 ) ) ;
#72840=CARTESIAN_POINT ( 'NONE',  ( 94.99999999999998579, 86.94004357329500010, 81.90374999999998806 ) ) ;
#72845=CARTESIAN_POINT ( 'NONE',  ( -96.32499999999996021, -212.2949673200287179, 88.91520833506763211 ) ) ;
#72847=CARTESIAN_POINT ( 'NONE',  ( 94.99999999999998579, 93.05995642670504253, 84.20562500173429044 ) ) ;
#72848=CARTESIAN_POINT ( 'NONE',  ( -97.30629616937501680, 90.00000000000004263, 85.99156250086716113 ) ) ;
#72849=CARTESIAN_POINT ( 'NONE',  ( 92.69370383062498320, 90.00000000000002842, 78.21281250086714465 ) ) ;
#72855=CARTESIAN_POINT ( 'NONE',  ( -92.69370383062498320, -208.6684592857803011, 79.85322916753379729 ) ) ;
#72858=CARTESIAN_POINT ( 'NONE',  ( 92.34999999999999432, 90.00000000000002842, 79.83999999999998920 ) ) ;
#72860=CARTESIAN_POINT ( 'NONE',  ( -97.64995694994090059, -208.4699969316842783, 81.13645661577280066 ) ) ;
#72861=CARTESIAN_POINT ( 'NONE',  ( 94.99999999999998579, 93.05995642670504253, 89.28562500173430294 ) ) ;
#72863=CARTESIAN_POINT ( 'NONE',  ( -93.84685191531247028, -211.9973110713294489, 80.96447916753380980 ) ) ;
#72876=CARTESIAN_POINT ( 'NONE',  ( 96.32499999999998863, -207.7050326799711968, 82.24770833506762813 ) ) ;
#72877=CARTESIAN_POINT ( 'NONE',  ( 96.15314808468748708, 88.00268892867053694, 87.94947916753380923 ) ) ;
#72881=CARTESIAN_POINT ( 'NONE',  ( -95.00000000000002842, 86.94004357329504273, 86.98374999999998636 ) ) ;
#72886=CARTESIAN_POINT ( 'NONE',  ( -92.35000000000003695, 90.00000000000004263, 75.71250000000000568 ) ) ;
#72890=CYLINDRICAL_SURFACE ( 'NONE', #50282, 2.649999999999985700 ) ;
#72892=CARTESIAN_POINT ( 'NONE',  ( -93.67499999999998295, -207.7050326799711968, 85.97833333333332462 ) ) ;
#72895=CARTESIAN_POINT ( 'NONE',  ( -92.34999999999999432, -209.9999999999999716, 90.00000000000000000 ) ) ;
#72902=ADVANCED_FACE ( 'NONE', ( #21456 ), #26723, .F. ) ;
#72903=CARTESIAN_POINT ( 'NONE',  ( 92.69370383062501162, -209.9999999999999716, 75.03781250086713328 ) ) ;
#72904=ORIENTED_EDGE ( 'NONE', *, *, #14413, .F. ) ;
#72909=( BOUNDED_CURVE ( )  B_SPLINE_CURVE ( 2, ( #33399, #27778, #72147, #73628, #21013, #22142, #43965, #9002, #61259 ),
 .UNSPECIFIED., .F., .F. ) 
 B_SPLINE_CURVE_WITH_KNOTS ( ( 3, 2, 2, 2, 3 ),
 ( 0.000000000000000000, 0.007055765540917050167, 0.01411153108183410033, 0.02116729662275115137, 0.02116741234835334273 ),
 .UNSPECIFIED. ) 
 CURVE ( )  GEOMETRIC_REPRESENTATION_ITEM ( )  RATIONAL_B_SPLINE_CURVE ( ( 1.000000000000000000, 0.8660254037844387076, 1.000000000000000000, 0.8660254037844387076, 1.000000000000000000, 0.8660254037844387076, 1.000000000000000000, 0.9999978026068560011, 0.9999956052857933431 ) ) 
 REPRESENTATION_ITEM ( '' )  );
#72910=CARTESIAN_POINT ( 'NONE',  ( 92.69370383062501162, -208.6684592857803295, 78.79489583420047438 ) ) ;
#72911=CARTESIAN_POINT ( 'NONE',  ( 92.69370383062501162, -211.3315407142195852, 84.13947916753383538 ) ) ;
#72914=CARTESIAN_POINT ( 'NONE',  ( 92.69370383062501162, -209.9999999999999716, 84.72156250086715090 ) ) ;
#72926=CARTESIAN_POINT ( 'NONE',  ( 97.64999999999997726, -211.5299782133524502, 89.07395833506762983 ) ) ;
#72927=ORIENTED_EDGE ( 'NONE', *, *, #55153, .T. ) ;
#72929=ORIENTED_EDGE ( 'NONE', *, *, #2237, .F. ) ;
#72931=ORIENTED_EDGE ( 'NONE', *, *, #12454, .T. ) ;
#72935=CARTESIAN_POINT ( 'NONE',  ( 97.30629616937498838, -209.9999999999999716, 76.62531250086713897 ) ) ;
#72943=EDGE_CURVE ( 'NONE', #44177, #18340, #5680, .T. ) ;
#72949=CARTESIAN_POINT ( 'NONE',  ( -97.65000000000001990, 91.52997821335253548, 89.94708333333333883 ) ) ;
#72951=CARTESIAN_POINT ( 'NONE',  ( 94.99999999999998579, 92.66308142843935514, 78.68906250086713783 ) ) ;
#72953=VECTOR ( 'NONE', #61746, 1000.000000000000000 ) ;
#72954=VERTEX_POINT ( 'NONE', #26106 ) ;
#72961=CARTESIAN_POINT ( 'NONE',  ( -93.84685191531247028, -211.9973110713294489, 78.42447916753381776 ) ) ;
#72971=CARTESIAN_POINT ( 'NONE',  ( 93.09104985768162521, -208.4386293813703048, 74.88237134757146407 ) ) ;
#72972=CARTESIAN_POINT ( 'NONE',  ( -92.69370383062502583, 91.33154071421968467, 81.75822916753381264 ) ) ;
#72978=CARTESIAN_POINT ( 'NONE',  ( 2.499999999999979572, 90.00000000000000000, -280.0000000000000000 ) ) ;
#72985=CARTESIAN_POINT ( 'NONE',  ( -92.35000000000006537, 91.52997821335257811, 87.19541666666667368 ) ) ;
#72986=CARTESIAN_POINT ( 'NONE',  ( -96.15314808468745866, -211.9973110713294489, 80.38239583420048007 ) ) ;
#72988=CARTESIAN_POINT ( 'NONE',  ( -92.35000000045951651, -209.9999506483816560, 87.22187670868756015 ) ) ;
#72990=EDGE_CURVE ( 'NONE', #1800, #7004, #21021, .T. ) ;
#72996=LINE ( 'NONE', #58226, #52188 ) ;
#73001=CYLINDRICAL_SURFACE ( 'NONE', #63626, 2.649999999999985700 ) ;
#73004=CARTESIAN_POINT ( 'NONE',  ( -92.35000000000179909, 90.00000306648279036, 75.79187510780352000 ) ) ;
#73009=DIRECTION ( 'NONE',  ( 0.000000000000000000, -0.000000000000000000, 1.000000000000000000 ) ) ;
#73014=CARTESIAN_POINT ( 'NONE',  ( 92.35000000000000853, -209.9999999999999716, 81.74500000000000455 ) ) ;
#73016=ORIENTED_EDGE ( 'NONE', *, *, #15289, .F. ) ;
#73018=CARTESIAN_POINT ( 'NONE',  ( 2.500000000000034639, 90.00000000000000000, -90.00000000000000000 ) ) ;
#73021=EDGE_LOOP ( 'NONE', ( #14411, #6778, #33257, #2816 ) ) ;
#73022=CARTESIAN_POINT ( 'NONE',  ( 97.30629616937498838, 88.66845928578037217, 75.46114583420049371 ) ) ;
#73030=CARTESIAN_POINT ( 'NONE',  ( 97.30629616937498838, 90.00000000000002842, 88.05531250086713158 ) ) ;
#73032=CARTESIAN_POINT ( 'NONE',  ( 92.69370383062501162, -211.3315407142195852, 86.52072916753381548 ) ) ;
#73043=CARTESIAN_POINT ( 'NONE',  ( -96.15314808468745866, -211.9973110713294489, 89.11364583420048291 ) ) ;
#73045=CARTESIAN_POINT ( 'NONE',  ( -96.15314808468751551, 88.00268892867056536, 84.19239583420049655 ) ) ;
#73047=CARTESIAN_POINT ( 'NONE',  ( 92.69370383062498320, 90.00000000000002842, 88.37281250086715545 ) ) ;
#73048=CARTESIAN_POINT ( 'NONE',  ( -93.84685191531254134, 91.99731107132950569, 89.43114583420047836 ) ) ;
#73055=FACE_OUTER_BOUND ( 'NONE', #18962, .T. ) ;
#73060=CARTESIAN_POINT ( 'NONE',  ( 97.64999999999999147, 90.00000000000002842, 89.68250000000000455 ) ) ;
#73061=ORIENTED_EDGE ( 'NONE', *, *, #53786, .F. ) ;
#73066=CARTESIAN_POINT ( 'NONE',  ( -97.65000000000001990, 88.47002178664754979, 80.52791666666665549 ) ) ;
#73067=CARTESIAN_POINT ( 'NONE',  ( -97.64999999950686060, 89.99996796133669363, 83.73041644179562581 ) ) ;
#73076=CARTESIAN_POINT ( 'NONE',  ( -97.30629616937501680, 88.66845928578038638, 82.71072916753379900 ) ) ;
#73083=CARTESIAN_POINT ( 'NONE',  ( -92.34999999999999432, -209.9999999999999716, 79.52249999999999375 ) ) ;
#73089=CARTESIAN_POINT ( 'NONE',  ( 97.30629616937498838, 91.33154071421968467, 79.37697916753381833 ) ) ;
#73092=CARTESIAN_POINT ( 'NONE',  ( -94.99999999999997158, -207.3369185715606307, 83.92781250086716227 ) ) ;
#73094=EDGE_LOOP ( 'NONE', ( #72808, #2806, #145, #53357 ) ) ;
#73095=CARTESIAN_POINT ( 'NONE',  ( -94.99999999999997158, -206.9400435732949575, 77.77624999999999034 ) ) ;
#73096=CARTESIAN_POINT ( 'NONE',  ( 92.35000000000000853, -211.5299782133524218, 78.70229166840096013 ) ) ;
#73099=CARTESIAN_POINT ( 'NONE',  ( -96.15314808468752972, 91.99731107132950569, 78.90072916753382515 ) ) ;
#73100=CARTESIAN_POINT ( 'NONE',  ( 97.30629616937498838, -208.6684592857803011, 80.48822916753383083 ) ) ;
#73104=CARTESIAN_POINT ( 'NONE',  ( -97.64999999993850111, -209.9999881782113675, 76.10900611559516449 ) ) ;
#73110=ORIENTED_EDGE ( 'NONE', *, *, #16476, .F. ) ;
#73115=CARTESIAN_POINT ( 'NONE',  ( 97.30629616937498838, -209.9999999999999716, 76.14906250086716000 ) ) ;
#73120=CARTESIAN_POINT ( 'NONE',  ( -96.10855813661771663, 87.63060383671344766, 74.97612907457774156 ) ) ;
#73121=CARTESIAN_POINT ( 'NONE',  ( 96.15314808468748708, 88.00268892867053694, 86.20322916753382003 ) ) ;
#73123=CARTESIAN_POINT ( 'NONE',  ( 92.35000000000002274, -211.5299782133524502, 79.25791666666665947 ) ) ;
#73128=CARTESIAN_POINT ( 'NONE',  ( 96.32499999999998863, -207.7050326799711968, 89.15333333333333599 ) ) ;
#73130=CARTESIAN_POINT ( 'NONE',  ( -97.64999999999996305, -209.9999999999999716, 90.00000000000000000 ) ) ;
#73131=FACE_OUTER_BOUND ( 'NONE', #41884, .T. ) ;
#73135=DIRECTION ( 'NONE',  ( -0.000000000000000000, -0.000000000000000000, 1.000000000000000000 ) ) ;
#73137=CARTESIAN_POINT ( 'NONE',  ( -97.64999999999996305, -209.9999999999999716, 81.82437500173429612 ) ) ;
#73141=CARTESIAN_POINT ( 'NONE',  ( 92.34999999999999432, 90.00000000000002842, 81.18937500173430521 ) ) ;
#73142=CARTESIAN_POINT ( 'NONE',  ( -92.35000000000005116, 88.47002178664754979, 83.35895833506762642 ) ) ;
#73143=( BOUNDED_CURVE ( )  B_SPLINE_CURVE ( 2, ( #70637, #19150, #42099, #66057, #37483, #50213, #22029 ),
 .UNSPECIFIED., .F., .F. ) 
 B_SPLINE_CURVE_WITH_KNOTS ( ( 3, 2, 2, 3 ),
 ( 0.2328402629019979686, 0.2398960283900005153, 0.2469517939308828458, 0.2540073681283128160 ),
 .UNSPECIFIED. ) 
 CURVE ( )  GEOMETRIC_REPRESENTATION_ITEM ( )  RATIONAL_B_SPLINE_CURVE ( ( 1.000000000000000000, 0.8660254037844387076, 1.000000000000000000, 0.8660254037844387076, 1.000000000000000000, 0.8660290370063226106, 0.9999927337532890093 ) ) 
 REPRESENTATION_ITEM ( '' )  );
#73145=CARTESIAN_POINT ( 'NONE',  ( 93.84685191531248449, 91.99731107132950569, 83.98072916753382344 ) ) ;
#73156=CARTESIAN_POINT ( 'NONE',  ( 97.64999999999999147, -209.9999999999999716, 77.61749999999999261 ) ) ;
#73166=CARTESIAN_POINT ( 'NONE',  ( -97.30629616937495996, -209.9999999999999716, 79.64156250086715261 ) ) ;
#73168=CARTESIAN_POINT ( 'NONE',  ( 95.00000000000000000, -213.0599564267049857, 81.26874999999999716 ) ) ;
#73175=LINE ( 'NONE', #56270, #7108 ) ;
#73176=CARTESIAN_POINT ( 'NONE',  ( 95.00000000000000000, -206.9400435732949575, 82.93562500173430863 ) ) ;
#73177=CARTESIAN_POINT ( 'NONE',  ( 94.99999999999998579, 92.66308142843932671, 77.41906250086714181 ) ) ;
#73179=CARTESIAN_POINT ( 'NONE',  ( -89.99999999999998579, -204.9999999999999716, 90.00000000000000000 ) ) ;
#73181=VECTOR ( 'NONE', #35861, 1000.000000000000000 ) ;
#73187=CARTESIAN_POINT ( 'NONE',  ( 93.67500000000001137, -212.2949673200287179, 83.12083333333332291 ) ) ;
#73190=CARTESIAN_POINT ( 'NONE',  ( -92.35001786631356424, 88.47001147152658973, 78.27895762153875125 ) ) ;
#73192=CARTESIAN_POINT ( 'NONE',  ( -97.30629616937501680, 91.33154071421968467, 83.87489583420047268 ) ) ;
#73201=AXIS2_PLACEMENT_3D ( 'NONE', #48224, #42960, #60260 ) ;
#73203=CARTESIAN_POINT ( 'NONE',  ( 92.69370383062501162, -208.6684592857803011, 79.58864583420047722 ) ) ;
#73204=ORIENTED_EDGE ( 'NONE', *, *, #63596, .F. ) ;
#73210=CARTESIAN_POINT ( 'NONE',  ( 97.64999999999999147, -209.9999999999999716, 89.68250000000000455 ) ) ;
#73216=ORIENTED_EDGE ( 'NONE', *, *, #39498, .F. ) ;
#73225=CARTESIAN_POINT ( 'NONE',  ( 95.00000000000000000, -206.9400435732949575, 78.49062500173430124 ) ) ;
#73227=CARTESIAN_POINT ( 'NONE',  ( 97.64999999999999147, 90.00000000000002842, 82.69749999999999091 ) ) ;
#73231=CARTESIAN_POINT ( 'NONE',  ( 92.35004305005917047, 91.53000306831577859, 81.13645661577284329 ) ) ;
#73232=EDGE_LOOP ( 'NONE', ( #39573, #57333, #40045, #23302 ) ) ;
#73234=EDGE_CURVE ( 'NONE', #6931, #33091, #64596, .T. ) ;
#73235=CARTESIAN_POINT ( 'NONE',  ( -97.30629616937501680, 90.00000000000004263, 85.35656250086715602 ) ) ;
#73236=CARTESIAN_POINT ( 'NONE',  ( 97.30629616937498838, 90.00000000000002842, 79.16531250086714522 ) ) ;
#73243=CARTESIAN_POINT ( 'NONE',  ( 92.69370383062501162, -209.9999999999999716, 89.80156250086714920 ) ) ;
#73244=CARTESIAN_POINT ( 'NONE',  ( -96.15314808468745866, -211.9973110713294489, 81.49364583420047836 ) ) ;
#73247=FACE_OUTER_BOUND ( 'NONE', #53951, .T. ) ;
#73249=DIRECTION ( 'NONE',  ( -0.000000000000000000, -0.000000000000000000, 1.000000000000000000 ) ) ;
#73250=CARTESIAN_POINT ( 'NONE',  ( 93.67499999999998295, 92.29496732002878900, 88.06854166840095388 ) ) ;
#73251=VERTEX_POINT ( 'NONE', #46377 ) ;
#73252=CARTESIAN_POINT ( 'NONE',  ( -97.30629616937495996, -209.9999999999999716, 76.30781250086714351 ) ) ;
#73255=CARTESIAN_POINT ( 'NONE',  ( -99.99999999999998579, -124.0000000000000284, 39.99999999999996447 ) ) ;
#73265=CARTESIAN_POINT ( 'NONE',  ( 93.84685191531248449, 88.00268892867053694, 89.11364583420048291 ) ) ;
#73267=CARTESIAN_POINT ( 'NONE',  ( 93.67499999999999716, 87.70503267997126784, 81.29520833506762756 ) ) ;
#73272=CARTESIAN_POINT ( 'NONE',  ( 92.34999999999999432, 90.00000000000002842, 77.29999999999999716 ) ) ;
#73281=CARTESIAN_POINT ( 'NONE',  ( -97.64999999999994884, -211.5299782133524502, 85.60791666666665378 ) ) ;
#73285=DIRECTION ( 'NONE',  ( 0.000000000000000000, 0.000000000000000000, 1.000000000000000000 ) ) ;
#73287=CARTESIAN_POINT ( 'NONE',  ( 92.34999999999999432, 90.00000000000002842, 81.74500000000000455 ) ) ;
#73288=CARTESIAN_POINT ( 'NONE',  ( 97.30629616937498838, -209.9999999999999716, 74.72031250086713783 ) ) ;
#73289=ORIENTED_EDGE ( 'NONE', *, *, #63826, .F. ) ;
#73292=VERTEX_POINT ( 'NONE', #52374 ) ;
#73293=CARTESIAN_POINT ( 'NONE',  ( 97.30629616937498838, -209.9999999999999716, 77.26031250086714408 ) ) ;
#73295=CARTESIAN_POINT ( 'NONE',  ( 92.69370383062501162, -209.9999999999999716, 83.45156250086715488 ) ) ;
#73302=DIRECTION ( 'NONE',  ( -3.061616997868382648E-16, -1.000000000000000000, 0.000000000000000000 ) ) ;
#73304=ORIENTED_EDGE ( 'NONE', *, *, #47985, .T. ) ;
#73308=FACE_OUTER_BOUND ( 'NONE', #11625, .T. ) ;
#73317=EDGE_CURVE ( 'NONE', #32442, #21322, #28828, .T. ) ;
#73320=CARTESIAN_POINT ( 'NONE',  ( 95.00000000000000000, -207.3369185715606307, 76.78406250086712248 ) ) ;
#73323=EDGE_LOOP ( 'NONE', ( #193, #55386, #17749, #62846 ) ) ;
#73331=CARTESIAN_POINT ( 'NONE',  ( -93.67500000000003979, 87.70503267997129626, 89.57666666666666799 ) ) ;
#73332=ADVANCED_FACE ( 'NONE', ( #55983 ), #54602, .F. ) ;
#73334=CARTESIAN_POINT ( 'NONE',  ( 92.69370383062498320, 88.66845928578037217, 76.36072916753381890 ) ) ;
#73336=DIRECTION ( 'NONE',  ( 1.000000000000000000, 0.000000000000000000, 0.000000000000000000 ) ) ;
#73337=CARTESIAN_POINT ( 'NONE',  ( -93.84685191531247028, -211.9973110713294489, 88.58447916753381435 ) ) ;
#73338=VERTEX_POINT ( 'NONE', #7995 ) ;
#73342=CARTESIAN_POINT ( 'NONE',  ( -97.30629616937497417, -211.3315407142195852, 78.26572916753380582 ) ) ;
#73343=CARTESIAN_POINT ( 'NONE',  ( -97.64999999999996305, -209.9999999999999716, 83.65000000000000568 ) ) ;
#73349=VERTEX_POINT ( 'NONE', #14377 ) ;
#73350=CYLINDRICAL_SURFACE ( 'NONE', #25256, 2.649999999999985700 ) ;
#73352=CARTESIAN_POINT ( 'NONE',  ( 93.86969025972541658, -207.8557763824826168, 74.86230178910948041 ) ) ;
#73353=CARTESIAN_POINT ( 'NONE',  ( -96.15314808468751551, 88.00268892867056536, 80.22364583420046813 ) ) ;
#73362=CARTESIAN_POINT ( 'NONE',  ( -2.499999999999965361, 90.00000000000000000, -310.0000000000000000 ) ) ;
#73365=CARTESIAN_POINT ( 'NONE',  ( 97.64999999999997726, -210.0000085086476531, 88.49187470744953998 ) ) ;
#73366=CARTESIAN_POINT ( 'NONE',  ( -97.30629616937497417, -211.3315407142195852, 79.05947916753382287 ) ) ;
#73368=( BOUNDED_CURVE ( )  B_SPLINE_CURVE ( 2, ( #46241, #62053, #73682, #45135, #16549, #34212, #21819 ),
 .UNSPECIFIED., .F., .F. ) 
 B_SPLINE_CURVE_WITH_KNOTS ( ( 3, 2, 2, 3 ),
 ( 0.2499999999999995837, 0.2569444444444442532, 0.2638888888888890061, 0.2708333333333337034 ),
 .UNSPECIFIED. ) 
 CURVE ( )  GEOMETRIC_REPRESENTATION_ITEM ( )  RATIONAL_B_SPLINE_CURVE ( ( 1.000000000000007994, 0.8660254037844307140, 1.000000000000000000, 0.8660254037844387076, 1.000000000000000000, 0.8660254037844311581, 1.000000000000007550 ) ) 
 REPRESENTATION_ITEM ( '' )  );
#73385=EDGE_CURVE ( 'NONE', #70635, #27457, #26019, .T. ) ;
#73392=CARTESIAN_POINT ( 'NONE',  ( -92.35000000010064980, -209.9999769027738239, 83.41187580057901130 ) ) ;
#73394=CARTESIAN_POINT ( 'NONE',  ( 96.32499999999998863, -212.2949673200287179, 81.95666666666666345 ) ) ;
#73402=ORIENTED_EDGE ( 'NONE', *, *, #30225, .F. ) ;
#73403=CARTESIAN_POINT ( 'NONE',  ( 94.99999999999998579, 92.66308142843935514, 77.57781250086715374 ) ) ;
#73407=ORIENTED_EDGE ( 'NONE', *, *, #4457, .T. ) ;
#73410=ORIENTED_EDGE ( 'NONE', *, *, #67815, .T. ) ;
#73411=CARTESIAN_POINT ( 'NONE',  ( -92.35000000000003695, 90.00000000000004263, 89.68250000000000455 ) ) ;
#73412=VECTOR ( 'NONE', #49512, 1000.000000000000000 ) ;
#73413=ORIENTED_EDGE ( 'NONE', *, *, #68089, .T. ) ;
#73414=CARTESIAN_POINT ( 'NONE',  ( 92.69370383062501162, -209.9999999999999716, 86.46781250086714010 ) ) ;
#73422=CARTESIAN_POINT ( 'NONE',  ( 92.34999999999999432, 90.00000929204269084, 84.99937468035462018 ) ) ;
#73423=CARTESIAN_POINT ( 'NONE',  ( -93.84685191531247028, -211.9973110713294489, 86.67947916753381321 ) ) ;
#73425=CARTESIAN_POINT ( 'NONE',  ( -95.00000000000002842, 87.33691857156074434, 85.51531250086713953 ) ) ;
#73428=ORIENTED_EDGE ( 'NONE', *, *, #24022, .F. ) ;
#73429=CARTESIAN_POINT ( 'NONE',  ( 92.69370383062498320, 88.66845928578037217, 89.06072916753379332 ) ) ;
#73430=CARTESIAN_POINT ( 'NONE',  ( -97.30629616937501680, 88.66845928578038638, 85.88572916753382458 ) ) ;
#73436=CARTESIAN_POINT ( 'NONE',  ( -96.15314808468745866, -211.9973110713294489, 88.47864583420047779 ) ) ;
#73437=CARTESIAN_POINT ( 'NONE',  ( 96.32499999999998863, -207.7050326799711968, 82.16833333333332234 ) ) ;
#73445=CARTESIAN_POINT ( 'NONE',  ( -93.67500000000003979, 87.70503267997129626, 80.68666666666665321 ) ) ;
#73447=CARTESIAN_POINT ( 'NONE',  ( 93.67500000000001137, -207.7050326799711968, 75.92416666666666458 ) ) ;
#73449=CARTESIAN_POINT ( 'NONE',  ( -94.99999999999997158, -213.0599564267049857, 76.90312500173429555 ) ) ;
#73454=CARTESIAN_POINT ( 'NONE',  ( -96.15314808468751551, 88.00268892867056536, 80.22364583420046813 ) ) ;
#73455=LINE ( 'NONE', #50900, #48753 ) ;
#73459=CARTESIAN_POINT ( 'NONE',  ( 2.500000000000043965, 65.00000000000000000, -290.0000000000000568 ) ) ;
#73460=CARTESIAN_POINT ( 'NONE',  ( -97.30629616937497417, -211.3315407142195852, 87.94947916753382344 ) ) ;
#73463=CARTESIAN_POINT ( 'NONE',  ( 92.69370383062498320, 88.66845928578035796, 80.32947916753381890 ) ) ;
#73464=CARTESIAN_POINT ( 'NONE',  ( -93.84685191531248449, -208.0026889286704943, 80.06489583420048461 ) ) ;
#73465=CARTESIAN_POINT ( 'NONE',  ( -92.35000000000003695, 89.99999988321006583, 84.68187499741277691 ) ) ;
#73470=CARTESIAN_POINT ( 'NONE',  ( 92.34999999999999432, 91.52997821335252127, 85.58145833506763722 ) ) ;
#73473=CARTESIAN_POINT ( 'NONE',  ( -97.30629616937501680, 88.66845928578038638, 78.42447916753380355 ) ) ;
#73474=CARTESIAN_POINT ( 'NONE',  ( 95.00000000000000000, -207.3369185715606307, 79.95906250086713385 ) ) ;
#73481=CARTESIAN_POINT ( 'NONE',  ( -97.64999999999994884, -210.0000065184970026, 88.17437522718661569 ) ) ;
#73493=CARTESIAN_POINT ( 'NONE',  ( 96.32499999999998863, -212.2949673200287179, 83.86166666666666458 ) ) ;
#73494=CARTESIAN_POINT ( 'NONE',  ( 96.15314808468748708, 88.00268892867053694, 88.10822916753382117 ) ) ;
#73495=ADVANCED_FACE ( 'NONE', ( #23269 ), #46201, .F. ) ;
#73497=CARTESIAN_POINT ( 'NONE',  ( 92.35000000000002274, -208.4700217866474645, 77.88208333333332689 ) ) ;
#73498=EDGE_LOOP ( 'NONE', ( #35961, #32884, #41777, #10155 ) ) ;
#73506=DIRECTION ( 'NONE',  ( -0.000000000000000000, -0.000000000000000000, 1.000000000000000000 ) ) ;
#73509=CARTESIAN_POINT ( 'NONE',  ( -92.34999999999999432, -208.4700217866474645, 83.46479166840096298 ) ) ;
#73510=EDGE_CURVE ( 'NONE', #70258, #70635, #15689, .T. ) ;
#73515=CARTESIAN_POINT ( 'NONE',  ( 92.34999999999999432, 88.47002178664753558, 82.51229166840094820 ) ) ;
#73516=CARTESIAN_POINT ( 'NONE',  ( -93.67500000000003979, 92.29496732002878900, 83.51770833506763836 ) ) ;
#73519=CARTESIAN_POINT ( 'NONE',  ( 97.30629616937498838, 91.33154071421968467, 84.45697916753383083 ) ) ;
#73520=CARTESIAN_POINT ( 'NONE',  ( -97.65000000000001990, 90.00000000000004263, 76.03000000000000114 ) ) ;
#73531=ORIENTED_EDGE ( 'NONE', *, *, #11857, .T. ) ;
#73532=AXIS2_PLACEMENT_3D ( 'NONE', #34161, #46192, #11584 ) ;
#73537=CARTESIAN_POINT ( 'NONE',  ( -93.84685191531248449, -208.0026889286704943, 81.96989583420048575 ) ) ;
#73540=ORIENTED_EDGE ( 'NONE', *, *, #21266, .T. ) ;
#73550=DIRECTION ( 'NONE',  ( 1.000000000000000000, 0.000000000000000000, 0.000000000000000000 ) ) ;
#73553=CARTESIAN_POINT ( 'NONE',  ( 92.35000000007822507, -209.9999869687480611, 79.28395951162927702 ) ) ;
#73559=CARTESIAN_POINT ( 'NONE',  ( -93.84685191531254134, 91.99731107132950569, 79.27114583420046756 ) ) ;
#73561=DIRECTION ( 'NONE',  ( -0.000000000000000000, -0.000000000000000000, 1.000000000000000000 ) ) ;
#73569=CARTESIAN_POINT ( 'NONE',  ( 95.00000000000000000, -207.3369185715606307, 75.67281250086716682 ) ) ;
#73571=ORIENTED_EDGE ( 'NONE', *, *, #34143, .T. ) ;
#73577=( BOUNDED_CURVE ( )  B_SPLINE_CURVE ( 2, ( #4214, #21468, #39153, #56069, #44054, #44429, #9832 ),
 .UNSPECIFIED., .F., .F. ) 
 B_SPLINE_CURVE_WITH_KNOTS ( ( 3, 2, 2, 3 ),
 ( 0.3749999999999998335, 0.3819444444444441977, 0.3888888888888886730, 0.3958333333333330373 ),
 .UNSPECIFIED. ) 
 CURVE ( )  GEOMETRIC_REPRESENTATION_ITEM ( )  RATIONAL_B_SPLINE_CURVE ( ( 1.000000000000003109, 0.8660254037844354880, 1.000000000000000000, 0.8660254037844387076, 1.000000000000000000, 0.8660254037844440367, 0.9999999999999946709 ) ) 
 REPRESENTATION_ITEM ( '' )  );
#73582=EDGE_CURVE ( 'NONE', #65117, #35350, #46376, .T. ) ;
#73583=CARTESIAN_POINT ( 'NONE',  ( 95.00000000000000000, -213.0599564267049857, 89.52375000000000682 ) ) ;
#73592=CARTESIAN_POINT ( 'NONE',  ( 2.499999999999988454, -65.00000000000000000, -290.0000000000000568 ) ) ;
#73593=ORIENTED_EDGE ( 'NONE', *, *, #73317, .F. ) ;
#73595=CARTESIAN_POINT ( 'NONE',  ( 97.64999999999997726, -211.5299782133524502, 80.18395833506764347 ) ) ;
#73596=CARTESIAN_POINT ( 'NONE',  ( 93.67499999999999716, 87.70503267997126784, 81.21583333333333599 ) ) ;
#73600=ADVANCED_FACE ( 'NONE', ( #51832 ), #10489, .F. ) ;
#73605=CARTESIAN_POINT ( 'NONE',  ( -92.69370383062505425, 88.66845928578038638, 84.98614583420047097 ) ) ;
#73606=CARTESIAN_POINT ( 'NONE',  ( 94.99999999999998579, 92.66308142843935514, 78.05406250086714692 ) ) ;
#73607=ORIENTED_EDGE ( 'NONE', *, *, #5446, .T. ) ;
#73614=CARTESIAN_POINT ( 'NONE',  ( -92.69370383062498320, -208.6684592857803011, 76.04322916753380923 ) ) ;
#73622=ORIENTED_EDGE ( 'NONE', *, *, #55991, .T. ) ;
#73623=CARTESIAN_POINT ( 'NONE',  ( -96.15314808468747287, -208.0026889286704943, 74.93197916753379673 ) ) ;
#73628=CARTESIAN_POINT ( 'NONE',  ( -94.99999999999997158, -206.9400435732949575, 89.28562500173430294 ) ) ;
#73632=CARTESIAN_POINT ( 'NONE',  ( 96.15314808468748708, 91.99731107132950569, 85.62114583420046188 ) ) ;
#73642=CARTESIAN_POINT ( 'NONE',  ( 97.64999999999999147, 90.00000000000002842, 78.88750000000000284 ) ) ;
#73646=CARTESIAN_POINT ( 'NONE',  ( -92.69370383062505425, 88.66845928578038638, 88.63739583420047552 ) ) ;
#73651=CARTESIAN_POINT ( 'NONE',  ( -96.32499999999996021, -212.2949673200287179, 85.66083333333332916 ) ) ;
#73653=EDGE_CURVE ( 'NONE', #45691, #35608, #51643, .T. ) ;
#73660=CARTESIAN_POINT ( 'NONE',  ( 97.30629616937498838, -211.3315407142195852, 85.62114583420047609 ) ) ;
#73661=ORIENTED_EDGE ( 'NONE', *, *, #69027, .T. ) ;
#73662=EDGE_LOOP ( 'NONE', ( #67430, #39340, #64214 ) ) ;
#73666=CARTESIAN_POINT ( 'NONE',  ( 96.15314808468748708, -208.0026889286704943, 76.73114583420047552 ) ) ;
#73668=VERTEX_POINT ( 'NONE', #6709 ) ;
#73669=ADVANCED_FACE ( 'NONE', ( #64232 ), #1483, .F. ) ;
#73670=CARTESIAN_POINT ( 'NONE',  ( 95.00000000000000000, -212.6630814284392557, 81.70531250086715147 ) ) ;
#73680=DIRECTION ( 'NONE',  ( -0.000000000000000000, -0.000000000000000000, 1.000000000000000000 ) ) ;
#73681=EDGE_LOOP ( 'NONE', ( #30486, #38910, #23207, #18116 ) ) ;
#73682=CARTESIAN_POINT ( 'NONE',  ( 93.67499999999998295, 92.29496732002878900, 86.08416666666666117 ) ) ;
#73683=CARTESIAN_POINT ( 'NONE',  ( 92.35000000000002274, -208.4700217866474645, 89.39145833506763950 ) ) ;
#73695=CARTESIAN_POINT ( 'NONE',  ( 97.30629616937498838, -208.6684592857803011, 76.04322916753380923 ) ) ;
#73698=CARTESIAN_POINT ( 'NONE',  ( -97.64999999999996305, -209.9999999999999716, 90.00000000000000000 ) ) ;
#73702=CARTESIAN_POINT ( 'NONE',  ( 96.32499999999998863, -212.2949673200287179, 76.24166666666666003 ) ) ;
#73703=CARTESIAN_POINT ( 'NONE',  ( -97.65000000000004832, -208.4700217866474929, 88.67708333333332860 ) ) ;
#73704=CARTESIAN_POINT ( 'NONE',  ( -93.84685191531254134, 91.99731107132950569, 76.88989583420048746 ) ) ;
#73706=CARTESIAN_POINT ( 'NONE',  ( 93.84685191531248449, 88.00268892867053694, 75.77864583420047495 ) ) ;
#73708=CARTESIAN_POINT ( 'NONE',  ( -92.69370383062498320, -208.6684592857803011, 84.93322916753379559 ) ) ;
#73711=CARTESIAN_POINT ( 'NONE',  ( -90.00000000000002842, 95.00000000000002842, 90.00000000000000000 ) ) ;
#73713=CARTESIAN_POINT ( 'NONE',  ( -92.69370383062498320, -211.3315407142195852, 79.11239583420046984 ) ) ;
#73721=CARTESIAN_POINT ( 'NONE',  ( 92.50303120605396145, -209.7556371990021944, 74.91343443312142369 ) ) ;
#73722=CARTESIAN_POINT ( 'NONE',  ( -97.30629616937501680, 91.33154071421968467, 81.96989583420048575 ) ) ;
#73724=CARTESIAN_POINT ( 'NONE',  ( 97.64999999999999147, 90.00000000000002842, 75.71250000000000568 ) ) ;
#73726=DIRECTION ( 'NONE',  ( -1.000000000000000000, 0.000000000000000000, 0.000000000000000000 ) ) ;
#73727=EDGE_CURVE ( 'NONE', #28568, #23400, #59327, .T. ) ;
#73734=CARTESIAN_POINT ( 'NONE',  ( -96.32500000000001705, 92.29496732002878900, 87.35416666666665719 ) ) ;
#73735=CARTESIAN_POINT ( 'NONE',  ( -92.69370383062498320, -209.9999999999999716, 80.59406250086715318 ) ) ;
#73743=CARTESIAN_POINT ( 'NONE',  ( -92.35000000000003695, 89.99999997928479445, 80.87187500099602744 ) ) ;
#73758=CARTESIAN_POINT ( 'NONE',  ( 96.15314808468750130, -211.9973110713294489, 87.94947916753380923 ) ) ;
#73764=CARTESIAN_POINT ( 'NONE',  ( -92.34999999999999432, -210.0000001167898631, 84.68187499741277691 ) ) ;
#73768=CARTESIAN_POINT ( 'NONE',  ( 92.35000000000003695, -211.5299782133524218, 81.79791666666665151 ) ) ;
#73775=CARTESIAN_POINT ( 'NONE',  ( 97.64999999999997726, 91.52997821335252127, 87.19541666666667368 ) ) ;
#73776=CYLINDRICAL_SURFACE ( 'NONE', #4840, 2.649999999999985700 ) ;
#73781=CARTESIAN_POINT ( 'NONE',  ( 96.15314808468748708, 88.00268892867053694, 89.21947916753380525 ) ) ;
#73783=CARTESIAN_POINT ( 'NONE',  ( 93.84685191531251292, -211.9973110713294489, 85.93864583420048575 ) ) ;
#73788=CARTESIAN_POINT ( 'NONE',  ( -93.67500000000003979, 92.29496732002878900, 77.80270833506763495 ) ) ;
#73790=CYLINDRICAL_SURFACE ( 'NONE', #18012, 2.649999999999999467 ) ;
#73792=CARTESIAN_POINT ( 'NONE',  ( -97.30629616937497417, -208.6684592857803011, 86.41489583420047893 ) ) ;
#73793=CARTESIAN_POINT ( 'NONE',  ( -95.00000000000002842, 87.33691857156074434, 84.88031250086714863 ) ) ;
#73794=EDGE_LOOP ( 'NONE', ( #29157, #43664, #60672, #35601 ) ) ;
#73795=CARTESIAN_POINT ( 'NONE',  ( 94.99999999999998579, 92.66308142843935514, 83.13406250086714522 ) ) ;
#73796=CARTESIAN_POINT ( 'NONE',  ( -97.30629616937501680, 90.00000000000004263, 85.83281250086714920 ) ) ;
#73800=CARTESIAN_POINT ( 'NONE',  ( -93.67499999999998295, -212.2949673200287179, 80.76604166840097321 ) ) ;
#73804=CARTESIAN_POINT ( 'NONE',  ( -93.84685191531248449, -208.0026889286704943, 88.79614583420047325 ) ) ;
#73812=CARTESIAN_POINT ( 'NONE',  ( -92.35000000000005116, 88.47002178664754979, 80.10458333333332348 ) ) ;
#73818=CARTESIAN_POINT ( 'NONE',  ( 97.64999999954044085, 90.00004935162768049, 87.22187670868791542 ) ) ;
#73821=( BOUNDED_CURVE ( )  B_SPLINE_CURVE ( 2, ( #67177, #32946, #48767, #21677, #37871, #61547, #49140, #54783, #10026 ),
 .UNSPECIFIED., .F., .F. ) 
 B_SPLINE_CURVE_WITH_KNOTS ( ( 3, 2, 2, 2, 3 ),
 ( 0.8678591737257297378, 0.8749149270737099915, 0.8819706926146264614, 0.8890264581555429313, 0.8890265259402125864 ),
 .UNSPECIFIED. ) 
 CURVE ( )  GEOMETRIC_REPRESENTATION_ITEM ( )  RATIONAL_B_SPLINE_CURVE ( ( 1.000000000000000000, 0.8660254037844387076, 1.000000000000000000, 0.8660254037844387076, 1.000000000000000000, 0.8660254037844387076, 1.000000000000000000, 0.9999987129073806269, 0.9999974258394913607 ) ) 
 REPRESENTATION_ITEM ( '' )  );
#73823=CARTESIAN_POINT ( 'NONE',  ( -92.69370383062502583, 88.66845928578038638, 78.47739583420047893 ) ) ;
#73825=EDGE_CURVE ( 'NONE', #42474, #18479, #15681, .T. ) ;
#73827=DIRECTION ( 'NONE',  ( -0.000000000000000000, -0.000000000000000000, 1.000000000000000000 ) ) ;
#73832=CARTESIAN_POINT ( 'NONE',  ( -93.84685191531248449, -208.0026889286704943, 89.58989583420049030 ) ) ;
#73835=CARTESIAN_POINT ( 'NONE',  ( 92.69370383062498320, 90.00000000000002842, 78.37156250086715659 ) ) ;
#73836=CARTESIAN_POINT ( 'NONE',  ( -94.99999999999997158, -212.6630814284392557, 81.07031250086716057 ) ) ;
#73840=CARTESIAN_POINT ( 'NONE',  ( -97.64999999999994884, -211.5299782133524502, 76.08291666666666231 ) ) ;
#73843=CARTESIAN_POINT ( 'NONE',  ( -93.84685191531254134, 91.99731107132950569, 79.42989583420049371 ) ) ;
#73844=CARTESIAN_POINT ( 'NONE',  ( 96.15314808468750130, -211.9973110713294489, 79.05947916753380866 ) ) ;
#73853=ORIENTED_EDGE ( 'NONE', *, *, #29761, .T. ) ;
#73861=ORIENTED_EDGE ( 'NONE', *, *, #24676, .T. ) ;
#73862=CARTESIAN_POINT ( 'NONE',  ( 93.84685191531249870, -208.0026889286704943, 75.09072916753380866 ) ) ;
#73867=CARTESIAN_POINT ( 'NONE',  ( 94.99999999999998579, 92.66308142843935514, 87.73781250086715033 ) ) ;
#73869=CARTESIAN_POINT ( 'NONE',  ( 97.64999999999999147, -209.9999999999999716, 79.52249999999999375 ) ) ;
#73872=ORIENTED_EDGE ( 'NONE', *, *, #8249, .T. ) ;
#73873=EDGE_LOOP ( 'NONE', ( #15030, #14351, #49652, #40523 ) ) ;
#73874=ORIENTED_EDGE ( 'NONE', *, *, #36655, .T. ) ;
#73879=CYLINDRICAL_SURFACE ( 'NONE', #65245, 2.649999999999985700 ) ;
#73884=CARTESIAN_POINT ( 'NONE',  ( -92.34999999999999432, -211.5299782133524502, 83.99395833506763154 ) ) ;
#73888=CARTESIAN_POINT ( 'NONE',  ( 97.64999999999997726, 88.47002178664753558, 83.35895833506762642 ) ) ;
#73889=CARTESIAN_POINT ( 'NONE',  ( -95.00000000000002842, 93.05995642670501411, 80.39562500173431658 ) ) ;
#73891=CARTESIAN_POINT ( 'NONE',  ( 94.99999999999998579, 87.33691857156068750, 84.24531250086715772 ) ) ;
#73892=FACE_OUTER_BOUND ( 'NONE', #36526, .T. ) ;
#73897=CARTESIAN_POINT ( 'NONE',  ( 92.34999999999999432, 90.00000000000002842, 90.00000000000000000 ) ) ;
#73906=CARTESIAN_POINT ( 'NONE',  ( 100.0010000000000474, -65.00000000000002842, -290.0000000000000568 ) ) ;
#73910=CYLINDRICAL_SURFACE ( 'NONE', #58125, 23.50000000000000355 ) ;
#73911=CARTESIAN_POINT ( 'NONE',  ( -92.69370383062498320, -211.3315407142195852, 81.17614583420048291 ) ) ;
#73913=CARTESIAN_POINT ( 'NONE',  ( -97.30629616937501680, 91.33154071421968467, 89.58989583420047609 ) ) ;
#73916=DIRECTION ( 'NONE',  ( -0.000000000000000000, -0.000000000000000000, 1.000000000000000000 ) ) ;
#73923=DIRECTION ( 'NONE',  ( -0.000000000000000000, -0.000000000000000000, -1.000000000000000000 ) ) ;
#73924=CARTESIAN_POINT ( 'NONE',  ( -99.99999999999998579, -116.0000000000000000, -40.00000000000002132 ) ) ;
#73931=CARTESIAN_POINT ( 'NONE',  ( 94.99999999999998579, 92.66308142843932671, 89.64281250086715147 ) ) ;
#73932=CARTESIAN_POINT ( 'NONE',  ( -94.99999999999997158, -212.6630814284392557, 89.32531250086715602 ) ) ;
#73936=CARTESIAN_POINT ( 'NONE',  ( -97.30629616937501680, 91.33154071421968467, 80.06489583420047040 ) ) ;
#73947=CARTESIAN_POINT ( 'NONE',  ( 96.15314808468748708, -208.0026889286704943, 74.98489583420048632 ) ) ;
#73949=VERTEX_POINT ( 'NONE', #34442 ) ;
#73950=CARTESIAN_POINT ( 'NONE',  ( 97.30629616937498838, -209.7238243954290056, 74.79348190356851944 ) ) ;
#73956=CARTESIAN_POINT ( 'NONE',  ( 95.00000000000000000, -213.0599564267049857, 88.25374999999999659 ) ) ;
#73959=DIRECTION ( 'NONE',  ( -4.476705744456277943E-17, 1.000000000000000000, -0.000000000000000000 ) ) ;
#73960=ORIENTED_EDGE ( 'NONE', *, *, #40658, .F. ) ;
#73968=CARTESIAN_POINT ( 'NONE',  ( 95.00000000000000000, -213.0599564267049857, 77.53812500173428646 ) ) ;
#73969=CARTESIAN_POINT ( 'NONE',  ( 94.99999999999998579, 86.94004357329500010, 80.63375000000000625 ) ) ;
#73977=CARTESIAN_POINT ( 'NONE',  ( 96.32499999999998863, -212.2949673200287179, 88.38604166840097776 ) ) ;
#73978=CARTESIAN_POINT ( 'NONE',  ( -95.00000000000002842, 87.33691857156074434, 80.43531250086715545 ) ) ;
#73979=CARTESIAN_POINT ( 'NONE',  ( 97.30629616937498838, 90.00000000000002842, 77.26031250086714408 ) ) ;
#73988=CARTESIAN_POINT ( 'NONE',  ( -92.69370383062498320, -208.6684592857803011, 77.94822916753381037 ) ) ;
#73997=ORIENTED_EDGE ( 'NONE', *, *, #52053, .F. ) ;
#73998=CARTESIAN_POINT ( 'NONE',  ( -92.69370383062498320, -209.9999999999999716, 76.62531250086713897 ) ) ;
#73999=ORIENTED_EDGE ( 'NONE', *, *, #21831, .T. ) ;
#74007=CARTESIAN_POINT ( 'NONE',  ( -92.35000000000003695, 90.00000000000004263, 81.42749999999999488 ) ) ;
#74009=CARTESIAN_POINT ( 'NONE',  ( 92.69370383062498320, 88.66845928578035796, 83.34572916753381833 ) ) ;
#74011=LINE ( 'NONE', #16887, #62610 ) ;
#74024=VECTOR ( 'NONE', #397, 1000.000000000000000 ) ;
#74025=CARTESIAN_POINT ( 'NONE',  ( -97.64999999999994884, -211.5299782133524502, 84.33791666666667197 ) ) ;
#74027=CARTESIAN_POINT ( 'NONE',  ( 96.32499999999998863, 87.70503267997126784, 85.76666666666665151 ) ) ;
#74031=( BOUNDED_CURVE ( )  B_SPLINE_CURVE ( 2, ( #73060, #68932, #23075, #44522, #74187, #56915, #22704 ),
 .UNSPECIFIED., .F., .F. ) 
 B_SPLINE_CURVE_WITH_KNOTS ( ( 3, 2, 2, 3 ),
 ( 0.02083333333333322115, 0.02777777777777762705, 0.03472222222222204335, 0.04166666666666644231 ),
 .UNSPECIFIED. ) 
 CURVE ( )  GEOMETRIC_REPRESENTATION_ITEM ( )  RATIONAL_B_SPLINE_CURVE ( ( 1.000000000000002220, 0.8660254037844365982, 1.000000000000000000, 0.8660254037844387076, 1.000000000000000000, 0.8660254037844430375, 0.9999999999999956701 ) ) 
 REPRESENTATION_ITEM ( '' )  );
#74037=CARTESIAN_POINT ( 'NONE',  ( 93.84685191531251292, -211.9973110713294489, 86.09739583420049769 ) ) ;
#74044=CARTESIAN_POINT ( 'NONE',  ( 97.30629616937498838, -211.3315407142195852, 77.20739583420046870 ) ) ;
#74046=CARTESIAN_POINT ( 'NONE',  ( 93.84685191531251292, -211.9973110713294489, 83.55739583420049144 ) ) ;
#74048=CARTESIAN_POINT ( 'NONE',  ( 92.35000000009272014, 90.00001381026685010, 80.55392363656929433 ) ) ;
#74051=CARTESIAN_POINT ( 'NONE',  ( -97.30629616937501680, 90.00000000000004263, 75.19656250086714522 ) ) ;
#74056=CARTESIAN_POINT ( 'NONE',  ( 97.64999999999997726, -208.4700217866474645, 88.54479166840097548 ) ) ;
#74057=VERTEX_POINT ( 'NONE', #39357 ) ;
#74059=EDGE_CURVE ( 'NONE', #19568, #28732, #34825, .T. ) ;
#74060=ORIENTED_EDGE ( 'NONE', *, *, #24447, .T. ) ;
#74071=ADVANCED_FACE ( 'NONE', ( #67554 ), #27309, .F. ) ;
#74079=CARTESIAN_POINT ( 'NONE',  ( -92.69370383062502583, 88.66845928578038638, 75.46114583420049371 ) ) ;
#74080=VERTEX_POINT ( 'NONE', #45002 ) ;
#74082=CARTESIAN_POINT ( 'NONE',  ( 92.69370383062498320, 90.00000000000002842, 75.67281250086713840 ) ) ;
#74084=FACE_OUTER_BOUND ( 'NONE', #68187, .T. ) ;
#74085=CARTESIAN_POINT ( 'NONE',  ( -93.84685191531248449, -208.0026889286704943, 86.89114583420047211 ) ) ;
#74091=CARTESIAN_POINT ( 'NONE',  ( -92.69370383062498320, -209.9999999999999716, 76.62531250086713897 ) ) ;
#74092=EDGE_CURVE ( 'NONE', #9907, #70250, #13772, .T. ) ;
#74096=CARTESIAN_POINT ( 'NONE',  ( -95.00000000000002842, 86.94004357329504273, 85.15812500173429100 ) ) ;
#74100=CARTESIAN_POINT ( 'NONE',  ( -93.84685191531254134, 91.99731107132950569, 81.81114583420047381 ) ) ;
#74104=B_SPLINE_CURVE_WITH_KNOTS ( 'NONE', 3,
 ( #34889, #63841, #63469, #36353, #69462, #11941 ),
 .UNSPECIFIED., .F., .F.,
 ( 4, 2, 4 ),
 ( 0.000000000000000000, 0.0008269033587273426789, 0.001653806717454685358 ),
 .UNSPECIFIED. ) ;
#74113=CARTESIAN_POINT ( 'NONE',  ( -97.64996763243314604, 91.52999690077599837, 87.48645704240065868 ) ) ;
#74114=CARTESIAN_POINT ( 'NONE',  ( -92.69370383062498320, -211.3315407142195852, 80.54114583420049200 ) ) ;
#74117=ORIENTED_EDGE ( 'NONE', *, *, #50647, .F. ) ;
#74129=ORIENTED_EDGE ( 'NONE', *, *, #18099, .F. ) ;
#74133=CARTESIAN_POINT ( 'NONE',  ( 96.15314808468750130, -211.9973110713294489, 89.21947916753380525 ) ) ;
#74134=CARTESIAN_POINT ( 'NONE',  ( -97.64999999950680376, -210.0000320386661485, 83.73041644189096644 ) ) ;
#74135=ORIENTED_EDGE ( 'NONE', *, *, #24228, .F. ) ;
#74146=CARTESIAN_POINT ( 'NONE',  ( 7.103376864691351012E-17, -120.0000000000000000, -85.59999999999999432 ) ) ;
#74149=ORIENTED_EDGE ( 'NONE', *, *, #55222, .T. ) ;
#74150=CARTESIAN_POINT ( 'NONE',  ( 92.34999999999999432, 88.47002178664753558, 89.41791666666667027 ) ) ;
#74151=CARTESIAN_POINT ( 'NONE',  ( 92.34999999999999432, 90.00000000000002842, 77.93499999999998806 ) ) ;
#74153=EDGE_LOOP ( 'NONE', ( #72545, #5315 ) ) ;
#74157=CARTESIAN_POINT ( 'NONE',  ( 96.15314808468748708, 91.99731107132950569, 83.71614583420047495 ) ) ;
#74159=CARTESIAN_POINT ( 'NONE',  ( 97.30629616937498838, -211.3315407142195852, 84.19239583420046813 ) ) ;
#74162=ADVANCED_FACE ( 'NONE', ( #13361 ), #1759, .F. ) ;
#74164=CARTESIAN_POINT ( 'NONE',  ( -97.64999999996642543, 89.99999234487438571, 78.01464417100932280 ) ) ;
#74170=CARTESIAN_POINT ( 'NONE',  ( -94.99999999999997158, -207.3369185715606307, 86.30906250086715659 ) ) ;
#74171=CARTESIAN_POINT ( 'NONE',  ( -97.30629616937501680, 88.66845928578038638, 85.40947916753380298 ) ) ;
#74173=CARTESIAN_POINT ( 'NONE',  ( 94.99999999999998579, 92.66308142843935514, 85.67406250086715147 ) ) ;
#74174=CARTESIAN_POINT ( 'NONE',  ( -92.69370383062502583, 88.66845928578038638, 84.82739583420045903 ) ) ;
#74187=CARTESIAN_POINT ( 'NONE',  ( 93.67499999999999716, 87.70503267997126784, 89.47083333333333144 ) ) ;
#74188=ORIENTED_EDGE ( 'NONE', *, *, #20410, .T. ) ;
#74194=CARTESIAN_POINT ( 'NONE',  ( -97.65000000000001990, 91.52997821335253548, 79.15208333333332291 ) ) ;
#74198=CARTESIAN_POINT ( 'NONE',  ( -97.64999999999996305, -209.9999999999999716, 90.00000000000000000 ) ) ;
#74199=DIRECTION ( 'NONE',  ( -0.000000000000000000, -0.000000000000000000, 1.000000000000000000 ) ) ;
#74202=CARTESIAN_POINT ( 'NONE',  ( -96.15314808468751551, 88.00268892867056536, 77.68364583420047609 ) ) ;
#74214=CARTESIAN_POINT ( 'NONE',  ( 92.69370383062498320, 90.00000000000002842, 77.10156250086714635 ) ) ;
#74215=CARTESIAN_POINT ( 'NONE',  ( -97.30629616937497417, -208.6684592857803295, 79.58864583420049144 ) ) ;
#74219=CARTESIAN_POINT ( 'NONE',  ( -92.34999999999999432, -208.4700217866474645, 75.13041666666666174 ) ) ;
#74221=CARTESIAN_POINT ( 'NONE',  ( -95.00000000000002842, 87.33691857156074434, 77.89531250086714920 ) ) ;
#74222=CARTESIAN_POINT ( 'NONE',  ( 92.69370383062501162, -208.6684592857803011, 81.33489583420048064 ) ) ;
#74235=ORIENTED_EDGE ( 'NONE', *, *, #9435, .T. ) ;
#74237=VERTEX_POINT ( 'NONE', #30641 ) ;
#74240=CARTESIAN_POINT ( 'NONE',  ( 93.84685191531248449, 88.00268892867053694, 82.92239583420048632 ) ) ;
#74241=CARTESIAN_POINT ( 'NONE',  ( 97.64999999999999147, -209.9999999999999716, 77.61749999999999261 ) ) ;
#74242=ORIENTED_EDGE ( 'NONE', *, *, #67817, .F. ) ;
#74252=DIRECTION ( 'NONE',  ( -0.000000000000000000, -0.000000000000000000, 1.000000000000000000 ) ) ;
#74253=FACE_OUTER_BOUND ( 'NONE', #71211, .T. ) ;
#74254=CARTESIAN_POINT ( 'NONE',  ( 92.35000000049298308, -210.0000320324309939, 85.63541623677062375 ) ) ;
#74257=CARTESIAN_POINT ( 'NONE',  ( -97.64999999950680376, -210.0000320386661485, 83.73041644189096644 ) ) ;
#74261=CARTESIAN_POINT ( 'NONE',  ( -92.34999999999999432, -208.4700217866474645, 82.82979166840095786 ) ) ;
#74265=CARTESIAN_POINT ( 'NONE',  ( 97.64999999999997726, 88.47002178664753558, 78.27895833506762813 ) ) ;
#74266=CARTESIAN_POINT ( 'NONE',  ( -92.35000000000005116, 88.47002178664754979, 79.54895833506762415 ) ) ;
#74267=( BOUNDED_CURVE ( )  B_SPLINE_CURVE ( 2, ( #31386, #55440, #49785, #54335, #37426, #49427, #2862 ),
 .UNSPECIFIED., .F., .F. ) 
 B_SPLINE_CURVE_WITH_KNOTS ( ( 3, 2, 2, 3 ),
 ( 0.5926843883797353607, 0.5997400709749997061, 0.6067958365158828693, 0.6138516023186938453 ),
 .UNSPECIFIED. ) 
 CURVE ( )  GEOMETRIC_REPRESENTATION_ITEM ( )  RATIONAL_B_SPLINE_CURVE ( ( 0.9999968501007930888, 0.8660269787525570750, 1.000000000000000000, 0.8660254037844387076, 1.000000000000000000, 0.8660254037844387076, 1.000000000000000000 ) ) 
 REPRESENTATION_ITEM ( '' )  );
#74268=ADVANCED_FACE ( 'NONE', ( #6620 ), #47579, .F. ) ;
#74270=CARTESIAN_POINT ( 'NONE',  ( 92.69370383062498320, 90.00000000000002842, 83.45156250086715488 ) ) ;
#74284=EDGE_CURVE ( 'NONE', #45691, #24219, #42682, .T. ) ;
#74288=CARTESIAN_POINT ( 'NONE',  ( -92.69370383062498320, -209.9999999999999716, 81.86406250086714920 ) ) ;
#74295=EDGE_CURVE ( 'NONE', #53104, #58523, #55065, .T. ) ;
#74299=CARTESIAN_POINT ( 'NONE',  ( 92.69370383062498320, 90.00000000000002842, 75.67281250086713840 ) ) ;
#74303=CARTESIAN_POINT ( 'NONE',  ( -97.65000000000003411, -208.4700217866475214, 79.15208333333333712 ) ) ;
#74304=CARTESIAN_POINT ( 'NONE',  ( -92.34999999999999432, -209.9999999999999716, 90.00000000000000000 ) ) ;
#74306=CARTESIAN_POINT ( 'NONE',  ( 97.30629616937498838, 88.66845928578035796, 86.25614583420048120 ) ) ;
#74308=CARTESIAN_POINT ( 'NONE',  ( -94.99999999999997158, -212.6630814284392557, 88.69031250086716511 ) ) ;
#74311=VERTEX_POINT ( 'NONE', #43447 ) ;
#74313=CARTESIAN_POINT ( 'NONE',  ( -97.30629616937501680, 90.00000000000004263, 79.48281250086714067 ) ) ;
#74323=CARTESIAN_POINT ( 'NONE',  ( 93.84685191531251292, -211.9973110713294489, 75.30239583420048177 ) ) ;
#74329=CARTESIAN_POINT ( 'NONE',  ( 96.15314808468748708, -208.0026889286704943, 85.77989583420048803 ) ) ;
#74335=AXIS2_PLACEMENT_3D ( 'NONE', #44418, #27474, #73336 ) ;
#74337=CARTESIAN_POINT ( 'NONE',  ( 96.32499999999998863, -212.2949673200287179, 88.94166666666666288 ) ) ;
ENDSEC;
END-ISO-10303-21;
